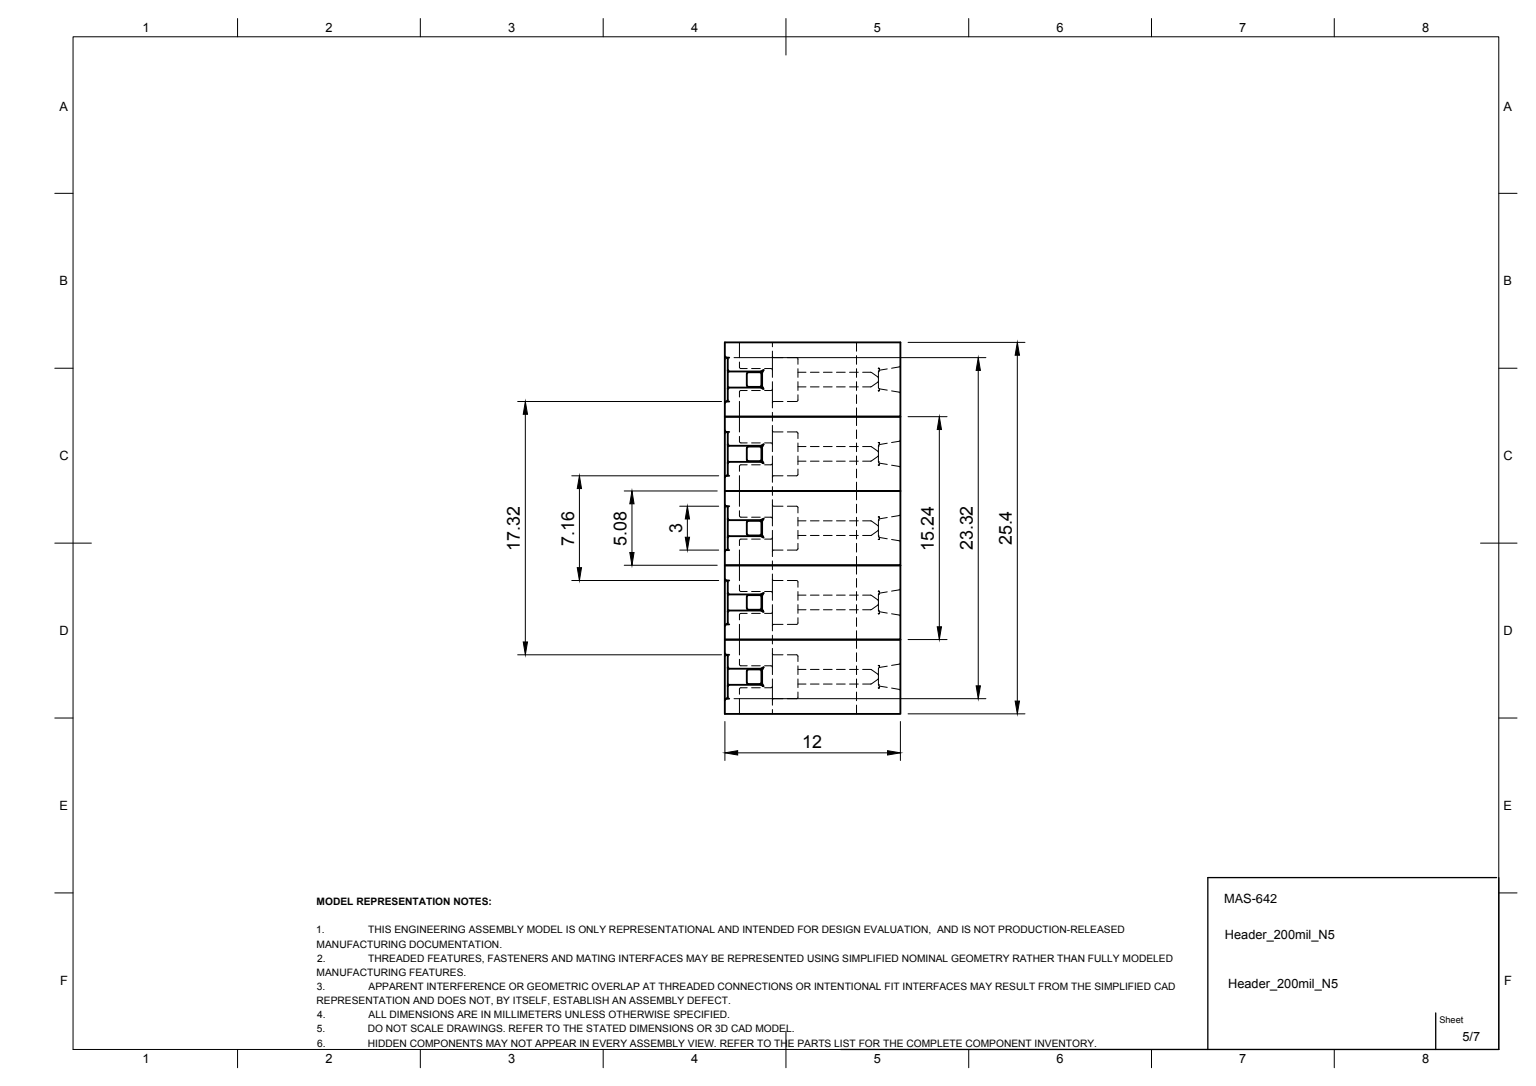
ISO-10303-21;
HEADER;
FILE_DESCRIPTION((''),'2;1');
FILE_NAME('Header_200mil_N5.step','2026-10-09T09:51:33-07:00',(''),(''),'','','');
FILE_SCHEMA (('AUTOMOTIVE_DESIGN { 1 0 10303 214 3 1 1 }'));
ENDSEC;
DATA;
#10=MECHANICAL_DESIGN_GEOMETRIC_PRESENTATION_REPRESENTATION('',(#482,#483,#484,#485,#486,#487,#488,#489,#490,#491,#492,#493,#494,#495,#496,#497,#498,#499,#500,#501,#502,#503,#504,#505,#506,#507,#508,#509,#510,#511,#512,#513,#514,#515,#516,#517,#518,#519,#520,#521,#522,#523,#524,#525,#526,#527,#528,#529,#530,#531,#532,#533,#534,#535,#536,#537,#538,#539,#540,#541,#542,#543,#544,#545,#546,#547,#548,#549,#550,#551,#552,#553,#554,#555,#556,#557,#558,#559,#560,#561,#562,#563,#564,#565,#566,#567,#568,#569,#570,#571,#572,#573,#574,#575,#576,#577,#578,#579,#580,#581,#582,#583,#584,#585,#586,#587,#588,#589,#590,#591,#592,#593,#594,#595,#596,#597,#598,#599,#600,#601,#602,#603,#604,#605,#606,#607,#608,#609,#610,#611,#612,#613,#614,#615,#616,#617,#618,#619,#620,#621,#622,#623,#624,#625,#626,#627,#628,#629,#630,#631,#632,#633,#634,#635,#636,#637,#638,#639,#640,#641,#642,#643,#644,#645,#646,#647,#648,#649,#650,#651,#652,#653,#654,#655,#656,#657,#658,#659,#660,#661,#662,#663,#664,#665,#666,#667,#668,#669,#670,#671,#672,#673,#674,#675,#676,#677,#678,#679,#680,#681,#682,#683,#684,#685,#686,#687,#688,#689,#690,#691,#692,#693,#694,#695,#696,#697,#698,#699,#700,#701,#702,#703,#704,#705,#706,#707,#708,#709,#710,#711,#712,#713,#714,#715,#716,#717,#718,#719,#720,#721,#722,#723,#724,#725,#726,#727,#728,#729,#730,#731,#732,#733,#734,#735,#736,#737,#738,#739,#740,#741,#742,#743,#744,#745,#746,#747,#748,#749,#750,#751,#752,#753,#754,#755,#756,#757,#758,#759,#760,#761,#762,#763,#764,#765,#766,#767,#768,#769,#770,#771,#772,#773,#774,#775,#776,#777,#778,#779,#780,#781,#782,#783,#784,#785,#786,#787,#788,#789,#790,#791,#792,#793,#794,#795,#796,#797,#798,#799,#800,#801,#802,#803,#804,#805,#806,#807,#808,#809,#810,#811,#812,#813,#814,#815,#816,#817,#818,#819,#820,#821,#822,#823,#824,#825,#826,#827,#828,#829,#830,#831,#832,#833,#834,#835,#836,#837,#838,#839,#840,#841,#842,#843,#844,#845,#846,#847,#848,#849,#850,#851,#852,#853,#854,#855,#856,#857,#858,#859,#860,#861,#862,#863,#864,#865,#866,#867,#868,#869,#870,#871,#872,#873,#874,#875,#876,#877,#878,#879,#880,#881,#882,#883,#884,#885,#886,#887,#888,#889,#890,#891,#892,#893,#894,#895,#896,#897,#898,#899,#900,#901,#902,#903,#904,#905,#906,#907,#908,#909,#910,#911,#912,#913,#914,#915,#916,#917,#918,#919,#920,#921,#922,#923,#924,#925,#926,#927,#928,#929,#930,#931,#932,#933,#934,#935,#936,#937,#938,#939,#940,#941,#942,#943,#944,#945,#946,#947,#948,#949,#950,#951,#952,#953,#954,#955,#956,#957,#958,#959,#960,#961,#962,#963,#964,#965,#966,#967,#968,#969,#970,#971,#972,#973,#974,#975,#976,#977,#978,#979,#980,#981,#982,#983,#984,#985,#986,#987,#988,#989,#990,#991,#992,#993,#994,#995,#996,#997,#998,#999,#1000,#1001,#1002,#1003,#1004,#1005,#1006,#1007,#1008,#1009,#1010,#1011,#1012,#1013,#1014,#1015,#1016,#1017,#1018,#1019,#1020,#1021,#1022,#1023,#1024,#1025,#1026,#1027,#1028,#1029,#1030,#1031,#1032,#1033,#1034,#1035,#1036,#1037,#1038,#1039,#1040,#1041,#1042,#1043,#1044,#1045,#1046,#1047,#1048,#1049,#1050,#1051,#1052,#1053,#1054,#1055,#1056,#1057,#1058,#1059,#1060,#1061,#1062,#1063,#1064,#1065,#1066,#1067,#1068,#1069,#1070,#1071,#1072,#1073,#1074,#1075,#1076,#1077,#1078,#1079,#1080,#1081,#1082,#1083,#1084,#1085,#1086,#1087,#1088,#1089,#1090,#1091,#1092,#1093,#1094,#1095,#1096,#1097,#1098,#1099,#1100,#1101,#1102,#1103,#1104,#1105,#1106,#1107,#1108,#1109,#1110,#1111,#1112,#1113,#1114,#1115,#1116,#1117,#1118,#1119,#1120,#1121,#1122,#1123,#1124,#1125,#1126,#1127,#1128,#1129,#1130,#1131,#1132,#1133,#1134,#1135,#1136,#1137,#1138,#1139,#1140,#1141,#1142,#1143,#1144,#1145,#1146,#1147,#1148,#1149,#1150,#1151,#1152,#1153,#1154,#1155,#1156,#1157,#1158,#1159,#1160,#1161,#1162,#1163,#1164,#1165,#1166,#1167,#1168,#1169,#1170,#1171,#1172,#1173,#1174,#1175,#1176,#1177,#1178,#1179,#1180,#1181,#1182,#1183,#1184,#1185,#1186,#1187,#1188,#1189,#1190,#1191,#1192,#1193,#1194,#1195,#1196,#1197,#1198,#1199,#1200,#1201,#1202,#1203,#1204,#1205,#1206,#1207,#1208,#1209,#1210,#1211,#1212,#1213,#1214,#1215,#1216,#1217,#1218,#1219,#1220,#1221,#1222,#1223,#1224,#1225,#1226,#1227,#1228,#1229,#1230,#1231,#1232,#1233,#1234,#1235,#1236,#1237,#1238,#1239,#1240,#1241,#1242,#1243,#1244,#1245,#1246,#1247,#1248,#1249,#1250,#1251,#1252,#1253,#1254,#1255,#1256,#1257,#1258,#1259,#1260,#1261,#1262,#1263,#1264,#1265,#1266,#1267,#1268,#1269,#1270,#1271,#1272,#1273,#1274,#1275,#1276,#1277,#1278,#1279,#1280,#1281,#1282,#1283,#1284,#1285,#1286,#1287,#1288,#1289,#1290,#1291,#1292,#1293,#1294,#1295,#1296,#1297,#1298,#1299,#1300,#1301,#1302,#1303,#1304,#1305,#1306,#1307,#1308,#1309,#1310,#1311,#1312,#1313,#1314,#1315,#1316,#1317,#1318,#1319,#1320,#1321,#1322,#1323,#1324,#1325,#1326,#1327,#1328,#1329,#1330,#1331,#1332,#1333,#1334,#1335,#1336,#1337,#1338,#1339,#1340,#1341,#1342,#1343,#1344,#1345,#1346,#1347,#1348,#1349,#1350,#1351,#1352,#1353,#1354,#1355,#1356,#1357,#1358,#1359,#1360,#1361,#1362,#1363,#1364,#1365,#1366,#1367,#1368,#1369,#1370,#1371,#1372,#1373,#1374,#1375,#1376,#1377,#1378,#1379,#1380,#1381,#1382,#1383,#1384,#1385,#1386,#1387,#1388,#1389,#1390,#1391,#1392,#1393,#1394,#1395,#1396,#1397,#1398,#1399,#1400,#1401,#1402,#1403,#1404,#1405,#1406,#1407,#1408,#1409,#1410,#1411,#1412,#1413,#1414,#1415,#1416,#1417,#1418,#1419,#1420,#1421,#1422,#1423,#1424,#1425,#1426,#1427,#1428,#1429,#1430,#1431,#1432,#1433,#1434,#1435,#1436,#1437,#1438,#1439,#1440,#1441,#1442,#1443,#1444,#1445,#1446,#1447,#1448,#1449,#1450,#1451,#1452,#1453,#1454,#1455,#1456,#1457,#1458,#1459,#1460,#1461,#1462,#1463,#1464,#1465,#1466,#1467,#1468,#1469,#1470,#1471,#1472,#1473,#1474,#1475,#1476,#1477,#1478,#1479,#1480,#1481,#1482,#1483,#1484,#1485,#1486,#1487,#1488,#1489,#1490,#1491,#1492,#1493,#1494,#1495,#1496,#1497,#1498,#1499,#1500,#1501,#1502,#1503,#1504,#1505,#1506,#1507,#1508,#1509,#1510,#1511,#1512,#1513,#1514,#1515,#1516,#1517,#1518,#1519,#1520,#1521,#1522,#1523,#1524,#1525,#1526,#1527,#1528,#1529,#1530,#1531,#1532,#1533,#1534,#1535,#1536,#1537,#1538,#1539,#1540,#1541,#1542,#1543,#1544,#1545,#1546,#1547,#1548,#1549,#1550,#1551,#1552,#1553,#1554,#1555,#1556,#1557,#1558,#1559,#1560,#1561,#1562,#1563,#1564,#1565,#1566,#1567,#1568,#1569,#1570,#1571,#1572,#1573,#1574,#1575,#1576,#1577,#1578,#1579,#1580,#1581,#1582,#1583,#1584,#1585,#1586,#1587,#1588,#1589,#1590,#1591,#1592,#1593,#1594,#1595,#1596,#1597,#1598,#1599,#1600,#1601,#1602,#1603,#1604,#1605,#1606,#1607,#1608,#1609,#1610,#1611,#1612,#1613,#1614,#1615,#1616,#1617,#1618,#1619,#1620,#1621,#1622,#1623,#1624,#1625,#1626,#1627,#1628,#1629,#1630,#1631,#1632,#1633,#1634,#1635,#1636,#1637,#1638,#1639,#1640,#1641,#1642,#1643,#1644,#1645,#1646,#1647,#1648,#1649,#1650,#1651,#1652,#1653,#1654,#1655,#1656,#1657,#1658,#1659,#1660,#1661,#1662,#1663,#1664,#1665,#1666,#1667,#1668,#1669,#1670,#1671,#1672,#1673,#1674,#1675,#1676,#1677,#1678,#1679,#1680,#1681,#1682,#1683,#1684,#1685,#1686,#1687,#1688,#1689,#1690,#1691,#1692,#1693,#1694,#1695,#1696,#1697,#1698,#1699,#1700,#1701,#1702,#1703,#1704,#1705,#1706,#1707,#1708,#1709,#1710,#1711,#1712,#1713,#1714,#1715,#1716,#1717,#1718,#1719,#1720,#1721,#1722,#1723,#1724,#1725,#1726,#1727,#1728,#1729,#1730,#1731,#1732,#1733,#1734,#1735,#1736,#1737,#1738,#1739,#1740,#1741,#1742,#1743,#1744,#1745,#1746,#1747,#1748,#1749,#1750,#1751,#1752,#1753,#1754,#1755,#1756,#1757,#1758,#1759,#1760,#1761,#1762,#1763,#1764,#1765,#1766,#1767,#1768,#1769,#1770,#1771,#1772,#1773,#1774,#1775,#1776,#1777,#1778,#1779,#1780,#1781,#1782,#1783,#1784,#1785,#1786,#1787,#1788,#1789,#1790,#1791,#1792,#1793,#1794,#1795,#1796,#1797,#1798,#1799,#1800,#1801,#1802,#1803,#1804,#1805,#1806,#1807,#1808,#1809,#1810,#1811,#1812,#1813,#1814,#1815,#1816,#1817,#1818,#1819,#1820,#1821,#1822,#1823,#1824,#1825,#1826,#1827,#1828,#1829,#1830,#1831,#1832,#1833,#1834,#1835,#1836,#1837,#1838,#1839,#1840,#1841,#1842,#1843,#1844,#1845,#1846,#1847,#1848,#1849,#1850,#1851,#1852,#1853,#1854,#1855,#1856,#1857,#1858,#1859,#1860,#1861,#1862,#1863,#1864,#1865,#1866,#1867,#1868,#1869,#1870,#1871,#1872,#1873,#1874,#1875,#1876,#1877,#1878,#1879,#1880,#1881,#1882,#1883,#1884,#1885,#1886,#1887,#1888,#1889,#1890,#1891,#1892,#1893,#1894,#1895,#1896,#1897,#1898,#1899,#1900,#1901,#1902,#1903,#1904,#1905,#1906,#1907,#1908,#1909,#1910,#1911,#1912,#1913,#1914,#1915,#1916,#1917,#1918,#1919,#1920,#1921,#1922,#1923,#1924,#1925,#1926,#1927,#1928,#1929,#1930,#1931),#126571);
#75=B_SPLINE_CURVE_WITH_KNOTS('',3,(#101199,#101200,#101201,#101202,#101203,
#101204,#101205,#101206,#101207,#101208),.UNSPECIFIED.,.F.,.F.,(4,3,3,4),
(3.9738238267564E-15,3.94729529730257E-5,7.90727202189652E-5,0.000103003463696664),
 .UNSPECIFIED.) ;
#76=B_SPLINE_CURVE_WITH_KNOTS('',3,(#101215,#101216,#101217,#101218,#101219,
#101220,#101221),.UNSPECIFIED.,.F.,.F.,(4,3,4),(0.000158223357507089,0.000179871364136711,
0.000191820073778124),.UNSPECIFIED.) ;
#77=B_SPLINE_CURVE_WITH_KNOTS('',3,(#101236,#101237,#101238,#101239,#101240,
#101241,#101242,#101243,#101244,#101245,#101246,#101247,#101248,#101249,
#101250,#101251),.UNSPECIFIED.,.F.,.F.,(4,3,3,3,3,4),(2.2541451328491E-8,
3.71181381094363E-5,7.40234349159883E-5,0.000126639028433409,0.000171180683285943,
0.000173579731706481),.UNSPECIFIED.) ;
#78=B_SPLINE_CURVE_WITH_KNOTS('',3,(#101307,#101308,#101309,#101310,#101311,
#101312),.UNSPECIFIED.,.F.,.F.,(4,2,4),(0.,0.000162685424844482,0.000325370849688964),
 .UNSPECIFIED.) ;
#79=B_SPLINE_CURVE_WITH_KNOTS('',3,(#101315,#101316,#101317,#101318,#101319,
#101320),.UNSPECIFIED.,.F.,.F.,(4,2,4),(0.,0.000163438694679258,0.000326877389358517),
 .UNSPECIFIED.) ;
#80=B_SPLINE_CURVE_WITH_KNOTS('',3,(#101331,#101332,#101333,#101334,#101335,
#101336),.UNSPECIFIED.,.F.,.F.,(4,2,4),(-0.00501427184001373,-0.00354643693242479,
0.),.UNSPECIFIED.) ;
#81=B_SPLINE_CURVE_WITH_KNOTS('',3,(#101349,#101350,#101351,#101352,#101353,
#101354,#101355,#101356,#101357,#101358,#101359,#101360,#101361,#101362,
#101363,#101364,#101365,#101366,#101367,#101368,#101369,#101370,#101371,
#101372,#101373,#101374,#101375,#101376),.UNSPECIFIED.,.F.,.F.,(4,3,3,3,
3,3,3,3,3,4),(5.23810621123106E-9,5.84794260518929E-6,8.4966204178186E-6,
1.21937803558207E-5,1.76033670138093E-5,1.93092034273016E-5,2.55871453405733E-5,
3.03154216363468E-5,3.6851966035102E-5,3.92146766969322E-5),
 .UNSPECIFIED.) ;
#82=B_SPLINE_CURVE_WITH_KNOTS('',3,(#101378,#101379,#101380,#101381,#101382,
#101383,#101384,#101385,#101386,#101387),.UNSPECIFIED.,.F.,.F.,(4,3,3,4),
(0.000144469795965456,0.000165397602015579,0.000173816468562374,0.000175865847906018),
 .UNSPECIFIED.) ;
#83=B_SPLINE_CURVE_WITH_KNOTS('',3,(#101405,#101406,#101407,#101408,#101409,
#101410,#101411),.UNSPECIFIED.,.F.,.F.,(4,3,4),(-2.05331166616804E-6,2.04386714305399E-5,
3.16299855932264E-5),.UNSPECIFIED.) ;
#84=B_SPLINE_CURVE_WITH_KNOTS('',3,(#101413,#101414,#101415,#101416,#101417,
#101418,#101419,#101420,#101421,#101422,#101423,#101424),.UNSPECIFIED.,
 .F.,.F.,(4,2,2,2,2,4),(9.00279448284787E-9,0.00183032786992351,0.0060774656661988,
0.0169681634641076,0.0216775195638031,0.0254454420779839),.UNSPECIFIED.) ;
#85=B_SPLINE_CURVE_WITH_KNOTS('',3,(#101583,#101584,#101585,#101586,#101587,
#101588,#101589,#101590,#101591,#101592,#101593,#101594,#101595,#101596,
#101597,#101598,#101599,#101600,#101601,#101602,#101603,#101604,#101605,
#101606,#101607,#101608,#101609,#101610,#101611,#101612,#101613,#101614,
#101615,#101616,#101617,#101618,#101619,#101620,#101621,#101622),
 .UNSPECIFIED.,.F.,.F.,(4,3,3,3,3,3,3,3,3,3,3,3,3,4),(3.25260651745651E-19,
5.07173230207635E-5,0.000104017413485144,0.000124506719166644,0.000125249568192437,
0.000156566023859648,0.000186760078749966,0.000187880030991792,0.000203537318084802,
0.000211366035547456,0.000217886758541627,0.000219194644848635,0.000234851354133261,
0.000249013438333288),.UNSPECIFIED.) ;
#86=B_SPLINE_CURVE_WITH_KNOTS('',3,(#101628,#101629,#101630,#101631,#101632,
#101633,#101634,#101635,#101636,#101637,#101638,#101639,#101640,#101641,
#101642,#101643,#101644,#101645,#101646,#101647,#101648,#101649,#101650,
#101651,#101652,#101653,#101654,#101655,#101656,#101657,#101658,#101659,
#101660,#101661,#101662,#101663,#101664,#101665,#101666,#101667),
 .UNSPECIFIED.,.F.,.F.,(4,3,3,3,3,3,3,3,3,3,3,3,3,4),(0.,1.43115567092604E-5,
3.01335133960367E-5,3.14552036774737E-5,3.8044751729729E-5,4.5956122251847E-5,
6.17788922892814E-5,6.29104073549473E-5,9.3421096696511E-5,0.000125066393795497,
0.000125820814709898,0.000179837268175291,0.000231469985683482,0.0002516416294198),
 .UNSPECIFIED.) ;
#87=B_SPLINE_CURVE_WITH_KNOTS('',3,(#101672,#101673,#101674,#101675,#101676,
#101677,#101678),.UNSPECIFIED.,.F.,.F.,(4,3,4),(-2.04939766627081E-6,0.,
2.93835791072158E-5),.UNSPECIFIED.) ;
#88=B_SPLINE_CURVE_WITH_KNOTS('',3,(#101693,#101694,#101695,#101696,#101697,
#101698,#101699,#101700,#101701,#101702,#101703,#101704,#101705,#101706),
 .UNSPECIFIED.,.F.,.F.,(4,2,2,2,2,2,4),(1.44901762830932E-6,0.00056162152378578,
0.00112173034328052,0.00210338619166554,0.00384452539466144,0.00473112295119629,
0.00541108585516142),.UNSPECIFIED.) ;
#89=B_SPLINE_CURVE_WITH_KNOTS('',3,(#101715,#101716,#101717,#101718,#101719,
#101720,#101721,#101722,#101723,#101724,#101725,#101726,#101727,#101728,
#101729,#101730,#101731,#101732,#101733,#101734,#101735,#101736,#101737,
#101738,#101739,#101740,#101741,#101742,#101743,#101744,#101745,#101746,
#101747,#101748),.UNSPECIFIED.,.F.,.F.,(4,2,2,2,2,2,2,2,2,2,2,2,2,2,2,2,
4),(0.,1.67528894171223E-5,3.36326639087882E-5,3.53285003632596E-5,3.67766442981684E-5,
4.45936877500603E-5,5.25629171992643E-5,5.37833548713901E-5,5.51649664472508E-5,
7.22376444474067E-5,7.35532885963332E-5,0.000109240736296583,0.000146228640920627,
0.000147106577192663,0.000203359192947108,0.000258123601946057,0.000294213154385318),
 .UNSPECIFIED.) ;
#90=B_SPLINE_CURVE_WITH_KNOTS('',3,(#101752,#101753,#101754,#101755,#101756,
#101757,#101758,#101759,#101760,#101761,#101762,#101763,#101764,#101765,
#101766,#101767,#101768,#101769,#101770,#101771,#101772,#101773,#101774,
#101775,#101776,#101777,#101778,#101779,#101780,#101781,#101782,#101783,
#101784,#101785,#101786,#101787,#101788,#101789,#101790,#101791,#101792,
#101793,#101794,#101795,#101796,#101797,#101798,#101799,#101800,#101801,
#101802,#101803),.UNSPECIFIED.,.F.,.F.,(4,3,3,3,3,3,3,3,3,3,3,3,3,3,3,3,
3,4),(0.,5.28180786082966E-5,0.000107888430275573,0.000143209193858987,
0.000144078242180707,0.000180086811859616,0.000214813790788481,0.00021545817026355,
0.000216102549738619,0.000232714940020855,0.000234106492510809,0.000238605983992194,
0.000240855729732887,0.00024310547547358,0.00025061608925323,0.000252108710851783,
0.000270124214172477,0.000286418387717979),.UNSPECIFIED.) ;
#91=B_SPLINE_CURVE_WITH_KNOTS('',3,(#101948,#101949,#101950,#101951,#101952,
#101953,#101954,#101955),.UNSPECIFIED.,.F.,.F.,(4,2,2,4),(-0.0473604779370388,
-0.0461995546884435,-0.0447198409510953,-0.0410407833884838),
 .UNSPECIFIED.) ;
#92=B_SPLINE_CURVE_WITH_KNOTS('',3,(#101963,#101964,#101965,#101966,#101967,
#101968,#101969,#101970),.UNSPECIFIED.,.F.,.F.,(4,2,2,4),(-0.0536801724855785,
-0.0500011149229822,-0.048521401185634,-0.0473604779370388),
 .UNSPECIFIED.) ;
#93=B_SPLINE_CURVE_WITH_KNOTS('',3,(#102424,#102425,#102426,#102427,#102428,
#102429,#102430,#102431,#102432,#102433,#102434,#102435,#102436,#102437),
 .UNSPECIFIED.,.F.,.F.,(4,2,2,2,2,2,4),(4.71238898038469,4.8817580624518,
5.06763701998932,5.24337922965563,5.26451333208247,5.44874090582915,5.49822830854824),
 .UNSPECIFIED.) ;
#94=B_SPLINE_CURVE_WITH_KNOTS('',3,(#102442,#102443,#102444,#102445,#102446,
#102447,#102448,#102449,#102450,#102451,#102452,#102453,#102454,#102455),
 .UNSPECIFIED.,.F.,.F.,(4,2,2,2,2,2,4),(0.784956998631334,0.96694169431193,
1.1431172121296,1.16348181627596,1.34745079132871,1.51752882030683,1.5707963267949),
 .UNSPECIFIED.) ;
#95=B_SPLINE_CURVE_WITH_KNOTS('',3,(#102461,#102462,#102463,#102464,#102465,
#102466,#102467,#102468,#102469,#102470,#102471,#102472,#102473,#102474),
 .UNSPECIFIED.,.F.,.F.,(4,2,2,2,2,2,4),(0.784956998631337,0.966941694311871,
1.14311721213079,1.16348181627588,1.34745079132852,1.51752882030658,1.5707963267949),
 .UNSPECIFIED.) ;
#96=B_SPLINE_CURVE_WITH_KNOTS('',3,(#102476,#102477,#102478,#102479,#102480,
#102481,#102482,#102483,#102484,#102485,#102486,#102487,#102488,#102489),
 .UNSPECIFIED.,.F.,.F.,(4,2,2,2,2,2,4),(4.71238898038469,4.88175806245191,
5.06763701998937,5.24337922965534,5.2645133320825,5.44874090582923,5.49822830854825),
 .UNSPECIFIED.) ;
#97=B_SPLINE_CURVE_WITH_KNOTS('',3,(#102493,#102494,#102495,#102496,#102497,
#102498,#102499,#102500,#102501,#102502,#102503,#102504,#102505,#102506),
 .UNSPECIFIED.,.F.,.F.,(4,2,2,2,2,2,4),(4.71238898038469,4.88175806245175,
5.06763701998915,5.24337922965918,5.26451333208223,5.44874090582892,5.49822830854824),
 .UNSPECIFIED.) ;
#98=B_SPLINE_CURVE_WITH_KNOTS('',3,(#102510,#102511,#102512,#102513,#102514,
#102515,#102516,#102517,#102518,#102519,#102520,#102521,#102522,#102523),
 .UNSPECIFIED.,.F.,.F.,(4,2,2,2,2,2,4),(0.784956998631348,0.96694169431196,
1.14311721213076,1.16348181627594,1.34745079132846,1.51752882030657,1.5707963267949),
 .UNSPECIFIED.) ;
#99=B_SPLINE_CURVE_WITH_KNOTS('',3,(#102538,#102539,#102540,#102541,#102542,
#102543,#102544,#102545,#102546,#102547,#102548,#102549,#102550,#102551),
 .UNSPECIFIED.,.F.,.F.,(4,2,2,2,2,2,4),(0.784956998631344,0.966941694311673,
1.14311721213023,1.16348181627565,1.34745079132822,1.51752882030641,1.5707963267949),
 .UNSPECIFIED.) ;
#100=B_SPLINE_CURVE_WITH_KNOTS('',3,(#102555,#102556,#102557,#102558,#102559,
#102560,#102561,#102562,#102563,#102564,#102565,#102566,#102567,#102568),
 .UNSPECIFIED.,.F.,.F.,(4,2,2,2,2,2,4),(4.71238898038469,4.88175806245189,
5.06763701998948,5.24337922965067,5.26451333208267,5.44874090582925,5.49822830854823),
 .UNSPECIFIED.) ;
#101=B_SPLINE_CURVE_WITH_KNOTS('',3,(#102673,#102674,#102675,#102676,#102677,
#102678,#102679,#102680,#102681,#102682,#102683,#102684,#102685,#102686,
#102687,#102688),.UNSPECIFIED.,.F.,.F.,(4,3,3,3,3,4),(0.,3.26760986414936E-5,
6.60604127813368E-5,0.00010113572426573,0.000138237800333083,0.000166242991827322),
 .UNSPECIFIED.) ;
#102=B_SPLINE_CURVE_WITH_KNOTS('',3,(#102750,#102751,#102752,#102753,#102754,
#102755,#102756,#102757,#102758,#102759,#102760,#102761,#102762,#102763,
#102764,#102765),.UNSPECIFIED.,.F.,.F.,(4,3,3,3,3,4),(0.,1.86901632150157E-5,
5.38940239621533E-5,9.13255451816924E-5,0.000129775966053829,0.000168373497604197),
 .UNSPECIFIED.) ;
#103=B_SPLINE_CURVE_WITH_KNOTS('',3,(#102770,#102771,#102772,#102773,#102774,
#102775,#102776,#102777,#102778,#102779),.UNSPECIFIED.,.F.,.F.,(4,2,2,2,
4),(0.0288531015810606,0.0296205843579712,0.0328031056820271,0.0376042554622301,
0.0407130021445681),.UNSPECIFIED.) ;
#104=B_SPLINE_CURVE_WITH_KNOTS('',3,(#102784,#102785,#102786,#102787,#102788,
#102789),.UNSPECIFIED.,.F.,.F.,(4,2,4),(0.0637474840427468,0.0675088661505087,
0.0720284409664136),.UNSPECIFIED.) ;
#105=B_SPLINE_CURVE_WITH_KNOTS('',3,(#102795,#102796,#102797,#102798,#102799,
#102800,#102801,#102802,#102803,#102804),.UNSPECIFIED.,.F.,.F.,(4,2,2,2,
4),(0.0767275662247105,0.0771734766312244,0.0818220866843324,0.0868722195343171,
0.0892832637334449),.UNSPECIFIED.) ;
#106=B_SPLINE_CURVE_WITH_KNOTS('',3,(#102839,#102840,#102841,#102842,#102843,
#102844),.UNSPECIFIED.,.F.,.F.,(4,2,4),(0.171679973604307,0.178707475947415,
0.186889989698882),.UNSPECIFIED.) ;
#107=B_SPLINE_CURVE_WITH_KNOTS('',3,(#102884,#102885,#102886,#102887,#102888,
#102889,#102890,#102891,#102892,#102893,#102894,#102895,#102896,#102897,
#102898,#102899,#102900,#102901,#102902,#102903,#102904,#102905,#102906,
#102907,#102908,#102909,#102910,#102911,#102912,#102913),.UNSPECIFIED.,
 .F.,.F.,(4,2,2,2,2,2,2,2,2,2,2,2,2,2,4),(2.36970964942748,2.55498029688293,
2.73514427897862,2.74569929646372,2.92071305421519,2.93943382978511,3.11857096683926,
3.13197658032397,3.25399179664489,3.45054278261474,3.62794535800311,3.64606212534864,
3.82474099483969,3.83698255062518,3.9134742131524),.UNSPECIFIED.) ;
#108=B_SPLINE_CURVE_WITH_KNOTS('',3,(#102924,#102925,#102926,#102927,#102928,
#102929,#102930,#102931,#102932,#102933,#102934,#102935,#102936,#102937,
#102938,#102939,#102940,#102941,#102942,#102943,#102944,#102945,#102946,
#102947,#102948,#102949),.UNSPECIFIED.,.F.,.F.,(4,2,2,2,2,2,2,2,2,2,2,2,
4),(2.70344464881052,2.89144352771273,3.06851986332525,3.0808108907457,
3.26996664970825,3.35940092938491,3.54587543017999,3.72254345721242,3.73903833379419,
3.91570024693591,3.93052100184837,4.1173551198632,4.22222897897866),
 .UNSPECIFIED.) ;
#109=B_SPLINE_CURVE_WITH_KNOTS('',3,(#103107,#103108,#103109,#103110,#103111,
#103112,#103113,#103114,#103115,#103116,#103117,#103118,#103119,#103120,
#103121,#103122,#103123,#103124,#103125),.UNSPECIFIED.,.F.,.F.,(4,3,3,3,
3,3,4),(2.81004151652491E-8,3.99307614181575E-5,8.00540716903473E-5,0.000126830846822484,
0.000175618195186419,0.00021519314047228,0.000245220898756747),
 .UNSPECIFIED.) ;
#110=B_SPLINE_CURVE_WITH_KNOTS('',3,(#103148,#103149,#103150,#103151,#103152,
#103153,#103154,#103155,#103156,#103157,#103158,#103159,#103160,#103161,
#103162,#103163,#103164,#103165,#103166,#103167,#103168,#103169,#103170,
#103171,#103172,#103173,#103174,#103175,#103176,#103177,#103178,#103179,
#103180,#103181,#103182,#103183,#103184,#103185,#103186,#103187,#103188,
#103189,#103190,#103191,#103192,#103193,#103194,#103195,#103196,#103197,
#103198,#103199,#103200,#103201,#103202,#103203,#103204,#103205,#103206,
#103207,#103208,#103209,#103210,#103211,#103212,#103213,#103214,#103215,
#103216,#103217,#103218,#103219,#103220,#103221,#103222,#103223,#103224,
#103225,#103226),.UNSPECIFIED.,.F.,.F.,(4,3,3,3,3,3,3,3,3,3,3,3,3,3,3,3,
3,3,3,3,3,3,3,3,3,3,4),(0.000152038190190966,0.00015489284140843,0.000155160464960067,
0.000160456565729287,0.000163456795060822,0.000166580092246913,0.000167751328691697,
0.000168007536663994,0.000168255738137156,0.000169267315291243,0.000175949983805187,
0.000178959298271468,0.000180334649023636,0.000187987241670312,0.000191981216408558,
0.000193065528939082,0.000193839174265184,0.000198143816207852,0.000212206269476803,
0.000226582370019584,0.000228143757087806,0.000228729277238389,0.000232827918292472,
0.000249109432819239,0.000250176797440921,0.000265881325829883,0.00026752567658937),
 .UNSPECIFIED.) ;
#111=B_SPLINE_CURVE_WITH_KNOTS('',3,(#103228,#103229,#103230,#103231,#103232,
#103233,#103234,#103235,#103236,#103237),.UNSPECIFIED.,.F.,.F.,(4,3,3,4),
(0.000130631741230592,0.000139067346352972,0.000143554831048516,0.000152038189371529),
 .UNSPECIFIED.) ;
#112=B_SPLINE_CURVE_WITH_KNOTS('',3,(#103239,#103240,#103241,#103242,#103243,
#103244,#103245,#103246,#103247,#103248,#103249,#103250,#103251,#103252,
#103253,#103254,#103255,#103256,#103257),.UNSPECIFIED.,.F.,.F.,(4,3,3,3,
3,3,4),(0.000104137230127885,0.000110259474166351,0.000116844366893157,
0.000120664217590229,0.000125429508057305,0.000130430624030388,0.000130630877722849),
 .UNSPECIFIED.) ;
#113=B_SPLINE_CURVE_WITH_KNOTS('',3,(#103258,#103259,#103260,#103261,#103262,
#103263,#103264,#103265,#103266,#103267,#103268,#103269,#103270,#103271,
#103272,#103273,#103274,#103275,#103276,#103277,#103278,#103279,#103280,
#103281,#103282,#103283,#103284,#103285,#103286,#103287,#103288,#103289,
#103290,#103291,#103292,#103293,#103294,#103295,#103296,#103297,#103298,
#103299,#103300),.UNSPECIFIED.,.F.,.F.,(4,3,3,3,3,3,3,3,3,3,3,3,3,3,4),
(0.,4.7842153196409E-6,1.59977421330766E-5,1.7596526576931E-5,2.63603667654262E-5,
3.75047088104424E-5,4.29655082836412E-5,5.34507806651091E-5,6.17416442239024E-5,
6.3936053046577E-5,7.32944438956243E-5,8.49065978095127E-5,9.46209320477897E-5,
9.66050857869699E-5,0.000104137229466899),.UNSPECIFIED.) ;
#114=B_SPLINE_CURVE_WITH_KNOTS('',3,(#103370,#103371,#103372,#103373,#103374,
#103375,#103376,#103377,#103378,#103379,#103380,#103381,#103382,#103383,
#103384,#103385,#103386,#103387,#103388,#103389,#103390,#103391,#103392,
#103393,#103394,#103395,#103396,#103397,#103398,#103399,#103400,#103401,
#103402,#103403),.UNSPECIFIED.,.F.,.F.,(4,3,3,3,3,3,3,3,3,3,3,4),(0.000173579735006479,
0.000179152672590571,0.000187122196212527,0.000190349677855674,0.000201571576239331,
0.000207505544696437,0.000209082158340111,0.000218112358783822,0.000219837174422831,
0.000228512621317844,0.000240802935331578,0.000245138123631296),
 .UNSPECIFIED.) ;
#115=B_SPLINE_CURVE_WITH_KNOTS('',3,(#103465,#103466,#103467,#103468,#103469,
#103470,#103471,#103472,#103473,#103474,#103475,#103476,#103477,#103478,
#103479,#103480),.UNSPECIFIED.,.F.,.F.,(4,3,3,3,3,4),(0.00014982626823882,
0.000156541783273878,0.000187447062839771,0.000218157419331145,0.000251253590119498,
0.000263630362845943),.UNSPECIFIED.) ;
#116=B_SPLINE_CURVE_WITH_KNOTS('',3,(#103482,#103483,#103484,#103485),
 .UNSPECIFIED.,.F.,.F.,(4,4),(0.000128945525003041,0.00014982626823882),
 .UNSPECIFIED.) ;
#117=B_SPLINE_CURVE_WITH_KNOTS('',3,(#103486,#103487,#103488,#103489,#103490,
#103491,#103492,#103493,#103494,#103495,#103496,#103497,#103498,#103499,
#103500,#103501),.UNSPECIFIED.,.F.,.F.,(4,3,3,3,3,4),(0.000107977862661221,
0.000113849696954279,0.000116758640899991,0.000123355930725603,0.00012864932133829,
0.000128945525003041),.UNSPECIFIED.) ;
#118=B_SPLINE_CURVE_WITH_KNOTS('',3,(#103711,#103712,#103713,#103714,#103715,
#103716,#103717,#103718,#103719,#103720),.UNSPECIFIED.,.F.,.F.,(4,3,3,4),
(3.97263228028543E-15,3.94729529730253E-5,7.90727202189645E-5,0.000103003463696544),
 .UNSPECIFIED.) ;
#119=B_SPLINE_CURVE_WITH_KNOTS('',3,(#103727,#103728,#103729,#103730,#103731,
#103732,#103733),.UNSPECIFIED.,.F.,.F.,(4,3,4),(0.000158223357507079,0.000179871364137041,
0.000191820073778125),.UNSPECIFIED.) ;
#120=B_SPLINE_CURVE_WITH_KNOTS('',3,(#103748,#103749,#103750,#103751,#103752,
#103753,#103754,#103755,#103756,#103757,#103758,#103759,#103760,#103761,
#103762,#103763),.UNSPECIFIED.,.F.,.F.,(4,3,3,3,3,4),(2.25414513312457E-8,
3.71181381094367E-5,7.40234349159884E-5,0.00012663902843341,0.000171180683285944,
0.000173579731706483),.UNSPECIFIED.) ;
#121=B_SPLINE_CURVE_WITH_KNOTS('',3,(#103819,#103820,#103821,#103822,#103823,
#103824),.UNSPECIFIED.,.F.,.F.,(4,2,4),(0.,0.000162685424844482,0.000325370849688964),
 .UNSPECIFIED.) ;
#122=B_SPLINE_CURVE_WITH_KNOTS('',3,(#103827,#103828,#103829,#103830,#103831,
#103832),.UNSPECIFIED.,.F.,.F.,(4,2,4),(0.,0.000163438694679258,0.000326877389358517),
 .UNSPECIFIED.) ;
#123=B_SPLINE_CURVE_WITH_KNOTS('',3,(#103843,#103844,#103845,#103846,#103847,
#103848),.UNSPECIFIED.,.F.,.F.,(4,2,4),(-0.00501427184001364,-0.00354643693242477,
0.),.UNSPECIFIED.) ;
#124=B_SPLINE_CURVE_WITH_KNOTS('',3,(#103861,#103862,#103863,#103864,#103865,
#103866,#103867,#103868,#103869,#103870,#103871,#103872,#103873,#103874,
#103875,#103876,#103877,#103878,#103879,#103880,#103881,#103882,#103883,
#103884,#103885,#103886,#103887,#103888),.UNSPECIFIED.,.F.,.F.,(4,3,3,3,
3,3,3,3,3,4),(5.23810620682237E-9,5.84794260519337E-6,8.49662041781855E-6,
1.2193780355802E-5,1.76033670137239E-5,1.93092034273018E-5,2.55871453405539E-5,
3.03154216363478E-5,3.68519660351436E-5,3.92146766969337E-5),
 .UNSPECIFIED.) ;
#125=B_SPLINE_CURVE_WITH_KNOTS('',3,(#103890,#103891,#103892,#103893,#103894,
#103895,#103896,#103897,#103898,#103899),.UNSPECIFIED.,.F.,.F.,(4,3,3,4),
(0.000144469795965455,0.000165397602015561,0.000173816468562373,0.000175865847906015),
 .UNSPECIFIED.) ;
#126=B_SPLINE_CURVE_WITH_KNOTS('',3,(#103917,#103918,#103919,#103920,#103921,
#103922,#103923),.UNSPECIFIED.,.F.,.F.,(4,3,4),(-2.05331166616703E-6,2.04386714305792E-5,
3.1629985593224E-5),.UNSPECIFIED.) ;
#127=B_SPLINE_CURVE_WITH_KNOTS('',3,(#103925,#103926,#103927,#103928,#103929,
#103930,#103931,#103932,#103933,#103934,#103935,#103936),.UNSPECIFIED.,
 .F.,.F.,(4,2,2,2,2,4),(9.00279511935952E-9,0.00183032787015945,0.00607746566495241,
0.016968163415124,0.0216775194921712,0.025445441987748),.UNSPECIFIED.) ;
#128=B_SPLINE_CURVE_WITH_KNOTS('',3,(#104095,#104096,#104097,#104098,#104099,
#104100,#104101,#104102,#104103,#104104,#104105,#104106,#104107,#104108,
#104109,#104110,#104111,#104112,#104113,#104114,#104115,#104116,#104117,
#104118,#104119,#104120,#104121,#104122,#104123,#104124,#104125,#104126,
#104127,#104128,#104129,#104130,#104131,#104132,#104133,#104134),
 .UNSPECIFIED.,.F.,.F.,(4,3,3,3,3,3,3,3,3,3,3,3,3,4),(0.,5.0717323021306E-5,
0.000104017413486267,0.000124506719166654,0.000125249568192443,0.000156566023859662,
0.000186760078749982,0.000187880030991811,0.000203537318084821,0.000211366035547473,
0.000217886758541643,0.000219194644848652,0.000234851354133276,0.000249013438333305),
 .UNSPECIFIED.) ;
#129=B_SPLINE_CURVE_WITH_KNOTS('',3,(#104140,#104141,#104142,#104143,#104144,
#104145,#104146,#104147,#104148,#104149,#104150,#104151,#104152,#104153,
#104154,#104155,#104156,#104157,#104158,#104159,#104160,#104161,#104162,
#104163,#104164,#104165,#104166,#104167,#104168,#104169,#104170,#104171,
#104172,#104173,#104174,#104175,#104176,#104177,#104178,#104179),
 .UNSPECIFIED.,.F.,.F.,(4,3,3,3,3,3,3,3,3,3,3,3,3,4),(0.,1.43115567092614E-5,
3.01335133960405E-5,3.14552036774747E-5,3.80447517297348E-5,4.59561222518546E-5,
6.17788922892857E-5,6.29104073549493E-5,9.34210966965139E-5,0.000125066393795497,
0.000125820814709899,0.00017983726817215,0.000231469985677585,0.0002516416294198),
 .UNSPECIFIED.) ;
#130=B_SPLINE_CURVE_WITH_KNOTS('',3,(#104184,#104185,#104186,#104187,#104188,
#104189,#104190),.UNSPECIFIED.,.F.,.F.,(4,3,4),(-2.04939766627066E-6,0.,
2.9383579107217E-5),.UNSPECIFIED.) ;
#131=B_SPLINE_CURVE_WITH_KNOTS('',3,(#104205,#104206,#104207,#104208,#104209,
#104210,#104211,#104212,#104213,#104214,#104215,#104216,#104217,#104218),
 .UNSPECIFIED.,.F.,.F.,(4,2,2,2,2,2,4),(1.44901762819747E-6,0.000561621523735244,
0.00112173034317294,0.00210338619144832,0.00384452539459816,0.00473112295166382,
0.00541108585598296),.UNSPECIFIED.) ;
#132=B_SPLINE_CURVE_WITH_KNOTS('',3,(#104227,#104228,#104229,#104230,#104231,
#104232,#104233,#104234,#104235,#104236,#104237,#104238,#104239,#104240,
#104241,#104242,#104243,#104244,#104245,#104246,#104247,#104248,#104249,
#104250,#104251,#104252,#104253,#104254,#104255,#104256,#104257,#104258,
#104259,#104260),.UNSPECIFIED.,.F.,.F.,(4,2,2,2,2,2,2,2,2,2,2,2,2,2,2,2,
4),(0.,1.67528894171568E-5,3.36326639087595E-5,3.532850036333E-5,3.67766442982351E-5,
4.45936877501458E-5,5.2562917199235E-5,5.37833548714877E-5,5.51649664473517E-5,
7.22376444475302E-5,7.35532885964682E-5,0.000109240736296779,0.000146228640920914,
0.000147106577192946,0.0002033591929484,0.000258123601948835,0.000294213154385907),
 .UNSPECIFIED.) ;
#133=B_SPLINE_CURVE_WITH_KNOTS('',3,(#104264,#104265,#104266,#104267,#104268,
#104269,#104270,#104271,#104272,#104273,#104274,#104275,#104276,#104277,
#104278,#104279,#104280,#104281,#104282,#104283,#104284,#104285,#104286,
#104287,#104288,#104289,#104290,#104291,#104292,#104293,#104294,#104295,
#104296,#104297,#104298,#104299,#104300,#104301,#104302,#104303,#104304,
#104305,#104306,#104307,#104308,#104309,#104310,#104311,#104312,#104313,
#104314,#104315),.UNSPECIFIED.,.F.,.F.,(4,3,3,3,3,3,3,3,3,3,3,3,3,3,3,3,
3,4),(0.,5.28180786102637E-5,0.00010788843028001,0.000143209193858987,0.000144078242180701,
0.000180086811859617,0.000214813790788482,0.000215458170263551,0.00021610254973862,
0.000232714940020857,0.00023410649251081,0.000238605983992196,0.000240855729732889,
0.000243105475473582,0.000250616089253232,0.000252108710851784,0.000270124214172475,
0.00028641838771798),.UNSPECIFIED.) ;
#134=B_SPLINE_CURVE_WITH_KNOTS('',3,(#104460,#104461,#104462,#104463,#104464,
#104465,#104466,#104467),.UNSPECIFIED.,.F.,.F.,(4,2,2,4),(-0.0473604779370388,
-0.0461995546884436,-0.0447198409510954,-0.0410407833884838),
 .UNSPECIFIED.) ;
#135=B_SPLINE_CURVE_WITH_KNOTS('',3,(#104475,#104476,#104477,#104478,#104479,
#104480,#104481,#104482),.UNSPECIFIED.,.F.,.F.,(4,2,2,4),(-0.0536801724855784,
-0.0500011149229823,-0.048521401185634,-0.0473604779370388),
 .UNSPECIFIED.) ;
#136=B_SPLINE_CURVE_WITH_KNOTS('',3,(#104936,#104937,#104938,#104939,#104940,
#104941,#104942,#104943,#104944,#104945,#104946,#104947,#104948,#104949),
 .UNSPECIFIED.,.F.,.F.,(4,2,2,2,2,2,4),(4.71238898038469,4.88175806245194,
5.06763701998947,5.24337922965538,5.26451333208261,5.4487409058292,5.49822830854821),
 .UNSPECIFIED.) ;
#137=B_SPLINE_CURVE_WITH_KNOTS('',3,(#104954,#104955,#104956,#104957,#104958,
#104959,#104960,#104961,#104962,#104963,#104964,#104965,#104966,#104967),
 .UNSPECIFIED.,.F.,.F.,(4,2,2,2,2,2,4),(0.78495699863134,0.966941694312354,
1.14311721213096,1.16348181627614,1.34745079132807,1.51752882030578,1.5707963267949),
 .UNSPECIFIED.) ;
#138=B_SPLINE_CURVE_WITH_KNOTS('',3,(#104973,#104974,#104975,#104976,#104977,
#104978,#104979,#104980,#104981,#104982,#104983,#104984,#104985,#104986),
 .UNSPECIFIED.,.F.,.F.,(4,2,2,2,2,2,4),(0.784956998631338,0.966941694312111,
1.14311721213157,1.16348181627597,1.34745079132821,1.51752882030615,1.5707963267949),
 .UNSPECIFIED.) ;
#139=B_SPLINE_CURVE_WITH_KNOTS('',3,(#104988,#104989,#104990,#104991,#104992,
#104993,#104994,#104995,#104996,#104997,#104998,#104999,#105000,#105001),
 .UNSPECIFIED.,.F.,.F.,(4,2,2,2,2,2,4),(4.71238898038469,4.88175806245166,
5.06763701998869,5.24337922965497,5.26451333208185,5.44874090582888,5.49822830854824),
 .UNSPECIFIED.) ;
#140=B_SPLINE_CURVE_WITH_KNOTS('',3,(#105005,#105006,#105007,#105008,#105009,
#105010,#105011,#105012,#105013,#105014,#105015,#105016,#105017,#105018),
 .UNSPECIFIED.,.F.,.F.,(4,2,2,2,2,2,4),(4.71238898038469,4.88175806245182,
5.06763701998925,5.24337922964886,5.26451333208237,5.44874090582905,5.49822830854823),
 .UNSPECIFIED.) ;
#141=B_SPLINE_CURVE_WITH_KNOTS('',3,(#105022,#105023,#105024,#105025,#105026,
#105027,#105028,#105029,#105030,#105031,#105032,#105033,#105034,#105035),
 .UNSPECIFIED.,.F.,.F.,(4,2,2,2,2,2,4),(0.784956998631348,0.966941694311913,
1.14311721213295,1.16348181627588,1.34745079132843,1.51752882030647,1.5707963267949),
 .UNSPECIFIED.) ;
#142=B_SPLINE_CURVE_WITH_KNOTS('',3,(#105050,#105051,#105052,#105053,#105054,
#105055,#105056,#105057,#105058,#105059,#105060,#105061,#105062,#105063),
 .UNSPECIFIED.,.F.,.F.,(4,2,2,2,2,2,4),(0.784956998631365,0.966941694311873,
1.14311721213002,1.16348181627585,1.34745079132852,1.51752882030655,1.5707963267949),
 .UNSPECIFIED.) ;
#143=B_SPLINE_CURVE_WITH_KNOTS('',3,(#105067,#105068,#105069,#105070,#105071,
#105072,#105073,#105074,#105075,#105076,#105077,#105078,#105079,#105080),
 .UNSPECIFIED.,.F.,.F.,(4,2,2,2,2,2,4),(4.71238898038469,4.88175806245151,
5.06763701998819,5.24337922965584,5.26451333208124,5.4487409058285,5.49822830854824),
 .UNSPECIFIED.) ;
#144=B_SPLINE_CURVE_WITH_KNOTS('',3,(#105185,#105186,#105187,#105188,#105189,
#105190,#105191,#105192,#105193,#105194,#105195,#105196,#105197,#105198,
#105199,#105200),.UNSPECIFIED.,.F.,.F.,(4,3,3,3,3,4),(0.,3.26760986414935E-5,
6.60604127813367E-5,0.00010113572426573,0.000138237800333083,0.000166242991827323),
 .UNSPECIFIED.) ;
#145=B_SPLINE_CURVE_WITH_KNOTS('',3,(#105262,#105263,#105264,#105265,#105266,
#105267,#105268,#105269,#105270,#105271,#105272,#105273,#105274,#105275,
#105276,#105277),.UNSPECIFIED.,.F.,.F.,(4,3,3,3,3,4),(0.,1.86901632150157E-5,
5.38940239621529E-5,9.13255451816918E-5,0.000129775966053829,0.000168373497604196),
 .UNSPECIFIED.) ;
#146=B_SPLINE_CURVE_WITH_KNOTS('',3,(#105282,#105283,#105284,#105285,#105286,
#105287,#105288,#105289,#105290,#105291),.UNSPECIFIED.,.F.,.F.,(4,2,2,2,
4),(0.0288531015801791,0.0296205843570608,0.0328031056810013,0.0376042554610398,
0.0407130021432729),.UNSPECIFIED.) ;
#147=B_SPLINE_CURVE_WITH_KNOTS('',3,(#105296,#105297,#105298,#105299,#105300,
#105301),.UNSPECIFIED.,.F.,.F.,(4,2,4),(0.063747484019213,0.0675088661241108,
0.0720284409363993),.UNSPECIFIED.) ;
#148=B_SPLINE_CURVE_WITH_KNOTS('',3,(#105307,#105308,#105309,#105310,#105311,
#105312,#105313,#105314,#105315,#105316),.UNSPECIFIED.,.F.,.F.,(4,2,2,2,
4),(0.0767275662235905,0.0771734766300911,0.0818220866830681,0.0868722195329092,
0.0892832637319672),.UNSPECIFIED.) ;
#149=B_SPLINE_CURVE_WITH_KNOTS('',3,(#105351,#105352,#105353,#105354,#105355,
#105356),.UNSPECIFIED.,.F.,.F.,(4,2,4),(0.171679973604201,0.178707475947309,
0.186889989698777),.UNSPECIFIED.) ;
#150=B_SPLINE_CURVE_WITH_KNOTS('',3,(#105396,#105397,#105398,#105399,#105400,
#105401,#105402,#105403,#105404,#105405,#105406,#105407,#105408,#105409,
#105410,#105411,#105412,#105413,#105414,#105415,#105416,#105417,#105418,
#105419,#105420,#105421,#105422,#105423,#105424,#105425),.UNSPECIFIED.,
 .F.,.F.,(4,2,2,2,2,2,2,2,2,2,2,2,2,2,4),(2.36970964942748,2.55498029688299,
2.73514427896706,2.74569929646378,2.92071305421126,2.93943382978513,3.11857096684179,
3.13197658032393,3.25399179664495,3.45054278261475,3.62794535799811,3.64606212534864,
3.82474099483732,3.83698255062522,3.91347421315246),.UNSPECIFIED.) ;
#151=B_SPLINE_CURVE_WITH_KNOTS('',3,(#105436,#105437,#105438,#105439,#105440,
#105441,#105442,#105443,#105444,#105445,#105446,#105447,#105448,#105449,
#105450,#105451,#105452,#105453,#105454,#105455,#105456,#105457,#105458,
#105459,#105460,#105461),.UNSPECIFIED.,.F.,.F.,(4,2,2,2,2,2,2,2,2,2,2,2,
4),(2.70344464881055,2.89144352771225,3.06851986332573,3.08081089074492,
3.26996664970766,3.35940092938473,3.5458754301802,3.72254345721718,3.73903833379462,
3.91570024693468,3.93052100184901,4.11735511986399,4.22222897897866),
 .UNSPECIFIED.) ;
#152=B_SPLINE_CURVE_WITH_KNOTS('',3,(#105619,#105620,#105621,#105622,#105623,
#105624,#105625,#105626,#105627,#105628,#105629,#105630,#105631,#105632,
#105633,#105634,#105635,#105636,#105637),.UNSPECIFIED.,.F.,.F.,(4,3,3,3,
3,3,4),(2.81004151703333E-8,3.99307614181576E-5,8.00540716903473E-5,0.000126830846822484,
0.00017561819518642,0.00021519314047228,0.000245220898756746),
 .UNSPECIFIED.) ;
#153=B_SPLINE_CURVE_WITH_KNOTS('',3,(#105660,#105661,#105662,#105663,#105664,
#105665,#105666,#105667,#105668,#105669,#105670,#105671,#105672,#105673,
#105674,#105675,#105676,#105677,#105678,#105679,#105680,#105681,#105682,
#105683,#105684,#105685,#105686,#105687,#105688,#105689,#105690,#105691,
#105692,#105693,#105694,#105695,#105696,#105697,#105698,#105699,#105700,
#105701,#105702,#105703,#105704,#105705,#105706,#105707,#105708,#105709,
#105710,#105711,#105712,#105713,#105714,#105715,#105716,#105717,#105718,
#105719,#105720,#105721,#105722,#105723,#105724,#105725,#105726,#105727,
#105728,#105729,#105730,#105731,#105732,#105733,#105734,#105735,#105736,
#105737,#105738),.UNSPECIFIED.,.F.,.F.,(4,3,3,3,3,3,3,3,3,3,3,3,3,3,3,3,
3,3,3,3,3,3,3,3,3,3,4),(0.000152038190191021,0.000154892841408471,0.000155160464960107,
0.000160456565729371,0.000163456795060821,0.000166580092246908,0.00016775132869169,
0.000168007536663986,0.000168255738137148,0.000169267315291303,0.000175949983805168,
0.000178959298271447,0.000180334649023613,0.000187987241670282,0.00019198121640859,
0.000193065528939067,0.00019383917426517,0.000198143816207851,0.000212206269476815,
0.000226582370019607,0.000228143757087823,0.000228729277238404,0.000232827918292471,
0.00024910943281953,0.00025017679744092,0.000265881325830107,0.000267525676589369),
 .UNSPECIFIED.) ;
#154=B_SPLINE_CURVE_WITH_KNOTS('',3,(#105740,#105741,#105742,#105743,#105744,
#105745,#105746,#105747,#105748,#105749),.UNSPECIFIED.,.F.,.F.,(4,3,3,4),
(0.000130631741230759,0.000139067346352796,0.000143554831048674,0.000152038189371587),
 .UNSPECIFIED.) ;
#155=B_SPLINE_CURVE_WITH_KNOTS('',3,(#105751,#105752,#105753,#105754,#105755,
#105756,#105757,#105758,#105759,#105760,#105761,#105762,#105763,#105764,
#105765,#105766,#105767,#105768,#105769),.UNSPECIFIED.,.F.,.F.,(4,3,3,3,
3,3,4),(0.000104137230127934,0.000110259474166471,0.000116844366893148,
0.000120664217590266,0.000125429508057305,0.000130430624030549,0.000130630877723017),
 .UNSPECIFIED.) ;
#156=B_SPLINE_CURVE_WITH_KNOTS('',3,(#105770,#105771,#105772,#105773,#105774,
#105775,#105776,#105777,#105778,#105779,#105780,#105781,#105782,#105783,
#105784,#105785,#105786,#105787,#105788,#105789,#105790,#105791,#105792,
#105793,#105794,#105795,#105796,#105797,#105798,#105799,#105800,#105801,
#105802,#105803,#105804,#105805,#105806,#105807,#105808,#105809,#105810,
#105811,#105812),.UNSPECIFIED.,.F.,.F.,(4,3,3,3,3,3,3,3,3,3,3,3,3,3,4),
(0.,4.78421531964037E-6,1.59977421331184E-5,1.75965265774506E-5,2.6360366765448E-5,
3.75047088104788E-5,4.29655082836413E-5,5.3450780665109E-5,6.17416442237089E-5,
6.39360530465768E-5,7.32944438958948E-5,8.49065978095123E-5,9.46209320474951E-5,
9.66050857869684E-5,0.000104137229466949),.UNSPECIFIED.) ;
#157=B_SPLINE_CURVE_WITH_KNOTS('',3,(#105882,#105883,#105884,#105885,#105886,
#105887,#105888,#105889,#105890,#105891,#105892,#105893,#105894,#105895,
#105896,#105897,#105898,#105899,#105900,#105901,#105902,#105903,#105904,
#105905,#105906,#105907,#105908,#105909,#105910,#105911,#105912,#105913,
#105914,#105915),.UNSPECIFIED.,.F.,.F.,(4,3,3,3,3,3,3,3,3,3,3,4),(0.000173579735006482,
0.000179152672590559,0.000187122196212438,0.000190349677855741,0.000201571576239487,
0.000207505544696553,0.000209082158340111,0.000218112358783938,0.000219837174422809,
0.000228512621317814,0.000240802935332003,0.000245138123631297),
 .UNSPECIFIED.) ;
#158=B_SPLINE_CURVE_WITH_KNOTS('',3,(#105977,#105978,#105979,#105980,#105981,
#105982,#105983,#105984,#105985,#105986,#105987,#105988,#105989,#105990,
#105991,#105992),.UNSPECIFIED.,.F.,.F.,(4,3,3,3,3,4),(0.000149826268238821,
0.000156541783273878,0.000187447062839771,0.000218157419331144,0.000251253590119497,
0.000263630362845938),.UNSPECIFIED.) ;
#159=B_SPLINE_CURVE_WITH_KNOTS('',3,(#105994,#105995,#105996,#105997),
 .UNSPECIFIED.,.F.,.F.,(4,4),(0.000128945525003057,0.000149826268238821),
 .UNSPECIFIED.) ;
#160=B_SPLINE_CURVE_WITH_KNOTS('',3,(#105998,#105999,#106000,#106001,#106002,
#106003,#106004,#106005,#106006,#106007,#106008,#106009,#106010,#106011,
#106012,#106013),.UNSPECIFIED.,.F.,.F.,(4,3,3,3,3,4),(0.000107977862661221,
0.000113849696954291,0.00011675864089999,0.000123355930725607,0.000128649321338309,
0.000128945525003057),.UNSPECIFIED.) ;
#161=B_SPLINE_CURVE_WITH_KNOTS('',3,(#106223,#106224,#106225,#106226,#106227,
#106228,#106229,#106230,#106231,#106232),.UNSPECIFIED.,.F.,.F.,(4,3,3,4),
(3.97436543900202E-15,3.94729529730262E-5,7.90727202189655E-5,0.000103003463696588),
 .UNSPECIFIED.) ;
#162=B_SPLINE_CURVE_WITH_KNOTS('',3,(#106239,#106240,#106241,#106242,#106243,
#106244,#106245),.UNSPECIFIED.,.F.,.F.,(4,3,4),(0.000158223357507084,0.000179871364136752,
0.000191820073778124),.UNSPECIFIED.) ;
#163=B_SPLINE_CURVE_WITH_KNOTS('',3,(#106260,#106261,#106262,#106263,#106264,
#106265,#106266,#106267,#106268,#106269,#106270,#106271,#106272,#106273,
#106274,#106275),.UNSPECIFIED.,.F.,.F.,(4,3,3,3,3,4),(2.25414513257385E-8,
3.7118138109435E-5,7.40234349159874E-5,0.000126639028433408,0.000171180683285943,
0.000173579731706481),.UNSPECIFIED.) ;
#164=B_SPLINE_CURVE_WITH_KNOTS('',3,(#106331,#106332,#106333,#106334,#106335,
#106336),.UNSPECIFIED.,.F.,.F.,(4,2,4),(0.,0.000162685424844482,0.000325370849688964),
 .UNSPECIFIED.) ;
#165=B_SPLINE_CURVE_WITH_KNOTS('',3,(#106339,#106340,#106341,#106342,#106343,
#106344),.UNSPECIFIED.,.F.,.F.,(4,2,4),(0.,0.000163438694679259,0.000326877389358518),
 .UNSPECIFIED.) ;
#166=B_SPLINE_CURVE_WITH_KNOTS('',3,(#106355,#106356,#106357,#106358,#106359,
#106360),.UNSPECIFIED.,.F.,.F.,(4,2,4),(-0.00501427184001376,-0.00354643693242498,
0.),.UNSPECIFIED.) ;
#167=B_SPLINE_CURVE_WITH_KNOTS('',3,(#106373,#106374,#106375,#106376,#106377,
#106378,#106379,#106380,#106381,#106382,#106383,#106384,#106385,#106386,
#106387,#106388,#106389,#106390,#106391,#106392,#106393,#106394,#106395,
#106396,#106397,#106398,#106399,#106400),.UNSPECIFIED.,.F.,.F.,(4,3,3,3,
3,3,3,3,3,4),(5.2381062129225E-9,5.84794260519105E-6,8.49662041781866E-6,
1.21937803558578E-5,1.76033670137842E-5,1.93092034273014E-5,2.55871453405162E-5,
3.0315421636347E-5,3.68519660350372E-5,3.92146766969318E-5),
 .UNSPECIFIED.) ;
#168=B_SPLINE_CURVE_WITH_KNOTS('',3,(#106402,#106403,#106404,#106405,#106406,
#106407,#106408,#106409,#106410,#106411),.UNSPECIFIED.,.F.,.F.,(4,3,3,4),
(0.000144469795965457,0.000165397602015722,0.000173816468562375,0.000175865847906017),
 .UNSPECIFIED.) ;
#169=B_SPLINE_CURVE_WITH_KNOTS('',3,(#106429,#106430,#106431,#106432,#106433,
#106434,#106435),.UNSPECIFIED.,.F.,.F.,(4,3,4),(-2.05331166617142E-6,2.04386714309068E-5,
3.1629985593225E-5),.UNSPECIFIED.) ;
#170=B_SPLINE_CURVE_WITH_KNOTS('',3,(#106437,#106438,#106439,#106440,#106441,
#106442,#106443,#106444,#106445,#106446,#106447,#106448),.UNSPECIFIED.,
 .F.,.F.,(4,2,2,2,2,4),(9.00279624299152E-9,0.00183032786957268,0.006077465667517,
0.0169681635237984,0.0216775196496615,0.0254454421850849),.UNSPECIFIED.) ;
#171=B_SPLINE_CURVE_WITH_KNOTS('',3,(#106607,#106608,#106609,#106610,#106611,
#106612,#106613,#106614,#106615,#106616,#106617,#106618,#106619,#106620,
#106621,#106622,#106623,#106624,#106625,#106626,#106627,#106628,#106629,
#106630,#106631,#106632,#106633,#106634,#106635,#106636,#106637,#106638,
#106639,#106640,#106641,#106642,#106643,#106644,#106645,#106646),
 .UNSPECIFIED.,.F.,.F.,(4,3,3,3,3,3,3,3,3,3,3,3,3,4),(0.,5.07173230218452E-5,
0.00010401741348744,0.000124506719166651,0.000125249568192438,0.000156566023859653,
0.000186760078749975,0.000187880030991798,0.000203537318084809,0.000211366035547463,
0.000217886758541637,0.000219194644848643,0.000234851354133269,0.000249013438333299),
 .UNSPECIFIED.) ;
#172=B_SPLINE_CURVE_WITH_KNOTS('',3,(#106652,#106653,#106654,#106655,#106656,
#106657,#106658,#106659,#106660,#106661,#106662,#106663,#106664,#106665,
#106666,#106667,#106668,#106669,#106670,#106671,#106672,#106673,#106674,
#106675,#106676,#106677,#106678,#106679,#106680,#106681,#106682,#106683,
#106684,#106685,#106686,#106687,#106688,#106689,#106690,#106691),
 .UNSPECIFIED.,.F.,.F.,(4,3,3,3,3,3,3,3,3,3,3,3,3,4),(0.,1.4311556709258E-5,
3.01335133960352E-5,3.14552036774726E-5,3.80447517297281E-5,4.59561222518464E-5,
6.17788922892798E-5,6.29104073549452E-5,9.34210966965093E-5,0.000125066393795483,
0.000125820814709883,0.000179837268173055,0.000231469985679291,0.000251641629419759),
 .UNSPECIFIED.) ;
#173=B_SPLINE_CURVE_WITH_KNOTS('',3,(#106696,#106697,#106698,#106699,#106700,
#106701,#106702),.UNSPECIFIED.,.F.,.F.,(4,3,4),(-2.04939766627128E-6,0.,
2.93835791072157E-5),.UNSPECIFIED.) ;
#174=B_SPLINE_CURVE_WITH_KNOTS('',3,(#106717,#106718,#106719,#106720,#106721,
#106722,#106723,#106724,#106725,#106726,#106727,#106728,#106729,#106730),
 .UNSPECIFIED.,.F.,.F.,(4,2,2,2,2,2,4),(1.44901762686856E-6,0.000561621523786212,
0.00112173034325288,0.00210338619152427,0.00384452539434926,0.00473112295079285,
0.00541108585487423),.UNSPECIFIED.) ;
#175=B_SPLINE_CURVE_WITH_KNOTS('',3,(#106739,#106740,#106741,#106742,#106743,
#106744,#106745,#106746,#106747,#106748,#106749,#106750,#106751,#106752,
#106753,#106754,#106755,#106756,#106757,#106758,#106759,#106760,#106761,
#106762,#106763,#106764,#106765,#106766,#106767,#106768,#106769,#106770,
#106771,#106772),.UNSPECIFIED.,.F.,.F.,(4,2,2,2,2,2,2,2,2,2,2,2,2,2,2,2,
4),(0.,1.6752889417125E-5,3.36326639084849E-5,3.53285003632986E-5,3.67766442982582E-5,
4.4593687750131E-5,5.25629171995868E-5,5.37833548715131E-5,5.51649664473856E-5,
7.22376444476005E-5,7.35532885965131E-5,0.000109240736296885,0.000146228640921016,
0.000147106577193024,0.000203359192940443,0.000258123601934358,0.000294213154386043),
 .UNSPECIFIED.) ;
#176=B_SPLINE_CURVE_WITH_KNOTS('',3,(#106776,#106777,#106778,#106779,#106780,
#106781,#106782,#106783,#106784,#106785,#106786,#106787,#106788,#106789,
#106790,#106791,#106792,#106793,#106794,#106795,#106796,#106797,#106798,
#106799,#106800,#106801,#106802,#106803,#106804,#106805,#106806,#106807,
#106808,#106809,#106810,#106811,#106812,#106813,#106814,#106815,#106816,
#106817,#106818,#106819,#106820,#106821,#106822,#106823,#106824,#106825,
#106826,#106827),.UNSPECIFIED.,.F.,.F.,(4,3,3,3,3,3,3,3,3,3,3,3,3,3,3,3,
3,4),(0.,5.28180786064093E-5,0.000107888430271973,0.000143209193858987,
0.00014407824218072,0.000180086811859619,0.00021481379078848,0.00021545817026355,
0.00021610254973862,0.000232714940020853,0.000234106492510808,0.000238605983992193,
0.000240855729732885,0.000243105475473578,0.000250616089253225,0.000252108710851782,
0.000270124214172477,0.000286418387717971),.UNSPECIFIED.) ;
#177=B_SPLINE_CURVE_WITH_KNOTS('',3,(#106972,#106973,#106974,#106975,#106976,
#106977,#106978,#106979),.UNSPECIFIED.,.F.,.F.,(4,2,2,4),(-0.0473604779370388,
-0.0461995546884437,-0.0447198409510955,-0.0410407833884838),
 .UNSPECIFIED.) ;
#178=B_SPLINE_CURVE_WITH_KNOTS('',3,(#106987,#106988,#106989,#106990,#106991,
#106992,#106993,#106994),.UNSPECIFIED.,.F.,.F.,(4,2,2,4),(-0.0536801724855783,
-0.0500011149229821,-0.0485214011856339,-0.0473604779370387),
 .UNSPECIFIED.) ;
#179=B_SPLINE_CURVE_WITH_KNOTS('',3,(#107448,#107449,#107450,#107451,#107452,
#107453,#107454,#107455,#107456,#107457,#107458,#107459,#107460,#107461),
 .UNSPECIFIED.,.F.,.F.,(4,2,2,2,2,2,4),(4.71238898038469,4.88175806245169,
5.06763701998897,5.24337922960769,5.26451333208202,5.44874090582883,5.49822830854825),
 .UNSPECIFIED.) ;
#180=B_SPLINE_CURVE_WITH_KNOTS('',3,(#107466,#107467,#107468,#107469,#107470,
#107471,#107472,#107473,#107474,#107475,#107476,#107477,#107478,#107479),
 .UNSPECIFIED.,.F.,.F.,(4,2,2,2,2,2,4),(0.784956998631304,0.966941694312144,
1.14311721221009,1.16348181627612,1.34745079132841,1.51752882030647,1.5707963267949),
 .UNSPECIFIED.) ;
#181=B_SPLINE_CURVE_WITH_KNOTS('',3,(#107485,#107486,#107487,#107488,#107489,
#107490,#107491,#107492,#107493,#107494,#107495,#107496,#107497,#107498),
 .UNSPECIFIED.,.F.,.F.,(4,2,2,2,2,2,4),(0.784956998631347,0.966941694312202,
1.1431172121312,1.16348181627609,1.34745079132826,1.51752882030624,1.5707963267949),
 .UNSPECIFIED.) ;
#182=B_SPLINE_CURVE_WITH_KNOTS('',3,(#107500,#107501,#107502,#107503,#107504,
#107505,#107506,#107507,#107508,#107509,#107510,#107511,#107512,#107513),
 .UNSPECIFIED.,.F.,.F.,(4,2,2,2,2,2,4),(4.71238898038469,4.88175806245171,
5.06763701998877,5.24337922965479,5.26451333208194,5.44874090582893,5.49822830854826),
 .UNSPECIFIED.) ;
#183=B_SPLINE_CURVE_WITH_KNOTS('',3,(#107517,#107518,#107519,#107520,#107521,
#107522,#107523,#107524,#107525,#107526,#107527,#107528,#107529,#107530),
 .UNSPECIFIED.,.F.,.F.,(4,2,2,2,2,2,4),(4.71238898038469,4.88175806245169,
5.06763701998911,5.2433792296566,5.26451333208232,5.44874090582905,5.49822830854824),
 .UNSPECIFIED.) ;
#184=B_SPLINE_CURVE_WITH_KNOTS('',3,(#107534,#107535,#107536,#107537,#107538,
#107539,#107540,#107541,#107542,#107543,#107544,#107545,#107546,#107547),
 .UNSPECIFIED.,.F.,.F.,(4,2,2,2,2,2,4),(0.784956998631345,0.966941694311759,
1.14311721212769,1.16348181627571,1.34745079132821,1.5175288203063,1.5707963267949),
 .UNSPECIFIED.) ;
#185=B_SPLINE_CURVE_WITH_KNOTS('',3,(#107562,#107563,#107564,#107565,#107566,
#107567,#107568,#107569,#107570,#107571,#107572,#107573,#107574,#107575),
 .UNSPECIFIED.,.F.,.F.,(4,2,2,2,2,2,4),(0.784956998631335,0.966941694312017,
1.14311721212471,1.16348181627591,1.34745079132842,1.5175288203063,1.5707963267949),
 .UNSPECIFIED.) ;
#186=B_SPLINE_CURVE_WITH_KNOTS('',3,(#107579,#107580,#107581,#107582,#107583,
#107584,#107585,#107586,#107587,#107588,#107589,#107590,#107591,#107592),
 .UNSPECIFIED.,.F.,.F.,(4,2,2,2,2,2,4),(4.71238898038469,4.88175806245169,
5.06763701998889,5.24337922965042,5.26451333208206,5.44874090582913,5.49822830854829),
 .UNSPECIFIED.) ;
#187=B_SPLINE_CURVE_WITH_KNOTS('',3,(#107697,#107698,#107699,#107700,#107701,
#107702,#107703,#107704,#107705,#107706,#107707,#107708,#107709,#107710,
#107711,#107712),.UNSPECIFIED.,.F.,.F.,(4,3,3,3,3,4),(0.,3.26760986414935E-5,
6.60604127813372E-5,0.00010113572426573,0.000138237800333083,0.000166242991827321),
 .UNSPECIFIED.) ;
#188=B_SPLINE_CURVE_WITH_KNOTS('',3,(#107774,#107775,#107776,#107777,#107778,
#107779,#107780,#107781,#107782,#107783,#107784,#107785,#107786,#107787,
#107788,#107789),.UNSPECIFIED.,.F.,.F.,(4,3,3,3,3,4),(0.,1.86901632150156E-5,
5.38940239621536E-5,9.1325545181693E-5,0.00012977596605383,0.000168373497604197),
 .UNSPECIFIED.) ;
#189=B_SPLINE_CURVE_WITH_KNOTS('',3,(#107794,#107795,#107796,#107797,#107798,
#107799,#107800,#107801,#107802,#107803),.UNSPECIFIED.,.F.,.F.,(4,2,2,2,
4),(0.0288531015833118,0.0296205843603292,0.0328031056847702,0.0376042554655217,
0.0407130021481444),.UNSPECIFIED.) ;
#190=B_SPLINE_CURVE_WITH_KNOTS('',3,(#107808,#107809,#107810,#107811,#107812,
#107813),.UNSPECIFIED.,.F.,.F.,(4,2,4),(0.0637474840407795,0.0675088661482764,
0.0720284409638634),.UNSPECIFIED.) ;
#191=B_SPLINE_CURVE_WITH_KNOTS('',3,(#107819,#107820,#107821,#107822,#107823,
#107824,#107825,#107826,#107827,#107828),.UNSPECIFIED.,.F.,.F.,(4,2,2,2,
4),(0.0767275662236361,0.0771734766301334,0.0818220866832597,0.0868722195332896,
0.0892832637324438),.UNSPECIFIED.) ;
#192=B_SPLINE_CURVE_WITH_KNOTS('',3,(#107863,#107864,#107865,#107866,#107867,
#107868),.UNSPECIFIED.,.F.,.F.,(4,2,4),(0.171679973605268,0.17870747594849,
0.186889989700107),.UNSPECIFIED.) ;
#193=B_SPLINE_CURVE_WITH_KNOTS('',3,(#107908,#107909,#107910,#107911,#107912,
#107913,#107914,#107915,#107916,#107917,#107918,#107919,#107920,#107921,
#107922,#107923,#107924,#107925,#107926,#107927,#107928,#107929,#107930,
#107931,#107932,#107933,#107934,#107935,#107936,#107937),.UNSPECIFIED.,
 .F.,.F.,(4,2,2,2,2,2,2,2,2,2,2,2,2,2,4),(2.36970964942748,2.55498029688296,
2.73514427897508,2.74569929646384,2.92071305423067,2.9394338297853,3.11857096686515,
3.13197658032419,3.25399179664505,3.450542782615,3.62794535799348,3.64606212534887,
3.82474099482299,3.83698255062533,3.9134742131517),.UNSPECIFIED.) ;
#194=B_SPLINE_CURVE_WITH_KNOTS('',3,(#107948,#107949,#107950,#107951,#107952,
#107953,#107954,#107955,#107956,#107957,#107958,#107959,#107960,#107961,
#107962,#107963,#107964,#107965,#107966,#107967,#107968,#107969,#107970,
#107971,#107972,#107973),.UNSPECIFIED.,.F.,.F.,(4,2,2,2,2,2,2,2,2,2,2,2,
4),(2.70344464881042,2.89144352771213,3.06851986339517,3.0808108907447,
3.26996664970742,3.35940092938473,3.54587543017995,3.72254345721779,3.73903833379426,
3.91570024691714,3.93052100184844,4.11735511986315,4.22222897897866),
 .UNSPECIFIED.) ;
#195=B_SPLINE_CURVE_WITH_KNOTS('',3,(#108131,#108132,#108133,#108134,#108135,
#108136,#108137,#108138,#108139,#108140,#108141,#108142,#108143,#108144,
#108145,#108146,#108147,#108148,#108149),.UNSPECIFIED.,.F.,.F.,(4,3,3,3,
3,3,4),(2.81004151523444E-8,3.99307614181576E-5,8.00540716903464E-5,0.000126830846822483,
0.000175618195186419,0.000215193140472279,0.00024522089875675),
 .UNSPECIFIED.) ;
#196=B_SPLINE_CURVE_WITH_KNOTS('',3,(#108172,#108173,#108174,#108175,#108176,
#108177,#108178,#108179,#108180,#108181,#108182,#108183,#108184,#108185,
#108186,#108187,#108188,#108189,#108190,#108191,#108192,#108193,#108194,
#108195,#108196,#108197,#108198,#108199,#108200,#108201,#108202,#108203,
#108204,#108205,#108206,#108207,#108208,#108209,#108210,#108211,#108212,
#108213,#108214,#108215,#108216,#108217,#108218,#108219,#108220,#108221,
#108222,#108223,#108224,#108225,#108226,#108227,#108228,#108229,#108230,
#108231,#108232,#108233,#108234,#108235,#108236,#108237,#108238,#108239,
#108240,#108241,#108242,#108243,#108244,#108245,#108246,#108247,#108248,
#108249,#108250),.UNSPECIFIED.,.F.,.F.,(4,3,3,3,3,3,3,3,3,3,3,3,3,3,3,3,
3,3,3,3,3,3,3,3,3,3,4),(0.000152038190191199,0.000154892841408555,0.000155160464960188,
0.000160456565729593,0.000163456795060823,0.000166580092246912,0.000167751328691695,
0.000168007536663992,0.000168255738137154,0.000169267315291292,0.000175949983805179,
0.000178959298271457,0.000180334649023622,0.000187987241670289,0.000191981216408587,
0.000193065528939071,0.000193839174265175,0.000198143816207854,0.000212206269476809,
0.000226582370019589,0.00022814375708781,0.000228729277238393,0.000232827918292474,
0.000249109432810095,0.000250176797440924,0.000265881325831287,0.000267525676589373),
 .UNSPECIFIED.) ;
#197=B_SPLINE_CURVE_WITH_KNOTS('',3,(#108252,#108253,#108254,#108255,#108256,
#108257,#108258,#108259,#108260,#108261),.UNSPECIFIED.,.F.,.F.,(4,3,3,4),
(0.000130631741230765,0.000139067346353096,0.000143554831048713,0.000152038189371763),
 .UNSPECIFIED.) ;
#198=B_SPLINE_CURVE_WITH_KNOTS('',3,(#108263,#108264,#108265,#108266,#108267,
#108268,#108269,#108270,#108271,#108272,#108273,#108274,#108275,#108276,
#108277,#108278,#108279,#108280,#108281),.UNSPECIFIED.,.F.,.F.,(4,3,3,3,
3,3,4),(0.000104137230128489,0.000110259474166938,0.000116844366893606,
0.00012066421759078,0.000125429508057306,0.000130430624030732,0.000130630877723054),
 .UNSPECIFIED.) ;
#199=B_SPLINE_CURVE_WITH_KNOTS('',3,(#108282,#108283,#108284,#108285,#108286,
#108287,#108288,#108289,#108290,#108291,#108292,#108293,#108294,#108295,
#108296,#108297,#108298,#108299,#108300,#108301,#108302,#108303,#108304,
#108305,#108306,#108307,#108308,#108309,#108310,#108311,#108312,#108313,
#108314,#108315,#108316,#108317,#108318,#108319,#108320,#108321,#108322,
#108323,#108324),.UNSPECIFIED.,.F.,.F.,(4,3,3,3,3,3,3,3,3,3,3,3,3,3,4),
(0.,4.78421531964207E-6,1.5997742133728E-5,1.75965265776594E-5,2.63603667652772E-5,
3.75047088100453E-5,4.29655082836422E-5,5.34507806651101E-5,6.17416442235669E-5,
6.39360530465779E-5,7.32944438965259E-5,8.49065978095135E-5,9.46209320476381E-5,
9.66050857869696E-5,0.000104137229467517),.UNSPECIFIED.) ;
#200=B_SPLINE_CURVE_WITH_KNOTS('',3,(#108394,#108395,#108396,#108397,#108398,
#108399,#108400,#108401,#108402,#108403,#108404,#108405,#108406,#108407,
#108408,#108409,#108410,#108411,#108412,#108413,#108414,#108415,#108416,
#108417,#108418,#108419,#108420,#108421,#108422,#108423,#108424,#108425,
#108426,#108427),.UNSPECIFIED.,.F.,.F.,(4,3,3,3,3,3,3,3,3,3,3,4),(0.00017357973500648,
0.000179152672590604,0.000187122196212524,0.000190349677855844,0.000201571576239683,
0.000207505544696743,0.00020908215834011,0.000218112358783795,0.000219837174422841,
0.000228512621317681,0.00024080293533128,0.000245138123631291),
 .UNSPECIFIED.) ;
#201=B_SPLINE_CURVE_WITH_KNOTS('',3,(#108489,#108490,#108491,#108492,#108493,
#108494,#108495,#108496,#108497,#108498,#108499,#108500,#108501,#108502,
#108503,#108504),.UNSPECIFIED.,.F.,.F.,(4,3,3,3,3,4),(0.000149826268238863,
0.000156541783273878,0.000187447062839773,0.000218157419331147,0.0002512535901195,
0.000263630362845944),.UNSPECIFIED.) ;
#202=B_SPLINE_CURVE_WITH_KNOTS('',3,(#108506,#108507,#108508,#108509),
 .UNSPECIFIED.,.F.,.F.,(4,4),(0.00012894552500308,0.000149826268238863),
 .UNSPECIFIED.) ;
#203=B_SPLINE_CURVE_WITH_KNOTS('',3,(#108510,#108511,#108512,#108513,#108514,
#108515,#108516,#108517,#108518,#108519,#108520,#108521,#108522,#108523,
#108524,#108525),.UNSPECIFIED.,.F.,.F.,(4,3,3,3,3,4),(0.000107977862661225,
0.000113849696954203,0.00011675864089999,0.000123355930725642,0.000128649321338296,
0.00012894552500308),.UNSPECIFIED.) ;
#204=B_SPLINE_CURVE_WITH_KNOTS('',3,(#108735,#108736,#108737,#108738,#108739,
#108740,#108741,#108742,#108743,#108744),.UNSPECIFIED.,.F.,.F.,(4,3,3,4),
(3.97436543900202E-15,3.94729529730262E-5,7.90727202189655E-5,0.000103003463696568),
 .UNSPECIFIED.) ;
#205=B_SPLINE_CURVE_WITH_KNOTS('',3,(#108751,#108752,#108753,#108754,#108755,
#108756,#108757),.UNSPECIFIED.,.F.,.F.,(4,3,4),(0.000158223357507064,0.000179871364136604,
0.000191820073778122),.UNSPECIFIED.) ;
#206=B_SPLINE_CURVE_WITH_KNOTS('',3,(#108772,#108773,#108774,#108775,#108776,
#108777,#108778,#108779,#108780,#108781,#108782,#108783,#108784,#108785,
#108786,#108787),.UNSPECIFIED.,.F.,.F.,(4,3,3,3,3,4),(2.25414513247713E-8,
3.7118138109435E-5,7.40234349159874E-5,0.000126639028433408,0.000171180683285943,
0.000173579731706481),.UNSPECIFIED.) ;
#207=B_SPLINE_CURVE_WITH_KNOTS('',3,(#108843,#108844,#108845,#108846,#108847,
#108848),.UNSPECIFIED.,.F.,.F.,(4,2,4),(0.,0.000162685424844483,0.000325370849688965),
 .UNSPECIFIED.) ;
#208=B_SPLINE_CURVE_WITH_KNOTS('',3,(#108851,#108852,#108853,#108854,#108855,
#108856),.UNSPECIFIED.,.F.,.F.,(4,2,4),(0.,0.000163438694679259,0.000326877389358518),
 .UNSPECIFIED.) ;
#209=B_SPLINE_CURVE_WITH_KNOTS('',3,(#108867,#108868,#108869,#108870,#108871,
#108872),.UNSPECIFIED.,.F.,.F.,(4,2,4),(-0.00501427184001376,-0.00354643693242498,
0.),.UNSPECIFIED.) ;
#210=B_SPLINE_CURVE_WITH_KNOTS('',3,(#108885,#108886,#108887,#108888,#108889,
#108890,#108891,#108892,#108893,#108894,#108895,#108896,#108897,#108898,
#108899,#108900,#108901,#108902,#108903,#108904,#108905,#108906,#108907,
#108908,#108909,#108910,#108911,#108912),.UNSPECIFIED.,.F.,.F.,(4,3,3,3,
3,3,3,3,3,4),(5.23810621265401E-9,5.84794260519711E-6,8.49662041781891E-6,
1.21937803558104E-5,1.76033670136906E-5,1.93092034273021E-5,2.55871453406251E-5,
3.0315421636348E-5,3.68519660352467E-5,3.92146766969314E-5),
 .UNSPECIFIED.) ;
#211=B_SPLINE_CURVE_WITH_KNOTS('',3,(#108914,#108915,#108916,#108917,#108918,
#108919,#108920,#108921,#108922,#108923),.UNSPECIFIED.,.F.,.F.,(4,3,3,4),
(0.000144469795965455,0.000165397602015376,0.000173816468562374,0.000175865847906018),
 .UNSPECIFIED.) ;
#212=B_SPLINE_CURVE_WITH_KNOTS('',3,(#108941,#108942,#108943,#108944,#108945,
#108946,#108947),.UNSPECIFIED.,.F.,.F.,(4,3,4),(-2.05331166616594E-6,2.04386714314149E-5,
3.16299855932266E-5),.UNSPECIFIED.) ;
#213=B_SPLINE_CURVE_WITH_KNOTS('',3,(#108949,#108950,#108951,#108952,#108953,
#108954,#108955,#108956,#108957,#108958,#108959,#108960),.UNSPECIFIED.,
 .F.,.F.,(4,2,2,2,2,4),(9.00279528345874E-9,0.00183032786964776,0.00607746566718187,
0.0169681635075991,0.0216775196267783,0.0254454421566977),.UNSPECIFIED.) ;
#214=B_SPLINE_CURVE_WITH_KNOTS('',3,(#109119,#109120,#109121,#109122,#109123,
#109124,#109125,#109126,#109127,#109128,#109129,#109130,#109131,#109132,
#109133,#109134,#109135,#109136,#109137,#109138,#109139,#109140,#109141,
#109142,#109143,#109144,#109145,#109146,#109147,#109148,#109149,#109150,
#109151,#109152,#109153,#109154,#109155,#109156,#109157,#109158),
 .UNSPECIFIED.,.F.,.F.,(4,3,3,3,3,3,3,3,3,3,3,3,3,4),(0.,5.0717323028302E-5,
0.00010401741350107,0.00012450671916665,0.000125249568192411,0.000156566023859649,
0.000186760078749971,0.000187880030991799,0.000203537318084808,0.000211366035547462,
0.000217886758541633,0.000219194644848641,0.000234851354133266,0.000249013438333296),
 .UNSPECIFIED.) ;
#215=B_SPLINE_CURVE_WITH_KNOTS('',3,(#109164,#109165,#109166,#109167,#109168,
#109169,#109170,#109171,#109172,#109173,#109174,#109175,#109176,#109177,
#109178,#109179,#109180,#109181,#109182,#109183,#109184,#109185,#109186,
#109187,#109188,#109189,#109190,#109191,#109192,#109193,#109194,#109195,
#109196,#109197,#109198,#109199,#109200,#109201,#109202,#109203),
 .UNSPECIFIED.,.F.,.F.,(4,3,3,3,3,3,3,3,3,3,3,3,3,4),(0.,1.43115567092591E-5,
3.01335133960395E-5,3.14552036774756E-5,3.80447517297363E-5,4.59561222518582E-5,
6.17788922892867E-5,6.29104073549512E-5,9.34210966965043E-5,0.00012506639379551,
0.00012582081470991,0.000179837268177068,0.000231469985686737,0.00025164162941983),
 .UNSPECIFIED.) ;
#216=B_SPLINE_CURVE_WITH_KNOTS('',3,(#109208,#109209,#109210,#109211,#109212,
#109213,#109214),.UNSPECIFIED.,.F.,.F.,(4,3,4),(-2.04939766627128E-6,0.,
2.93835791072157E-5),.UNSPECIFIED.) ;
#217=B_SPLINE_CURVE_WITH_KNOTS('',3,(#109229,#109230,#109231,#109232,#109233,
#109234,#109235,#109236,#109237,#109238,#109239,#109240,#109241,#109242),
 .UNSPECIFIED.,.F.,.F.,(4,2,2,2,2,2,4),(1.44901763072086E-6,0.000561621523748031,
0.00112173034319911,0.00210338619150003,0.00384452539461507,0.00473112295159275,
0.00541108585601945),.UNSPECIFIED.) ;
#218=B_SPLINE_CURVE_WITH_KNOTS('',3,(#109251,#109252,#109253,#109254,#109255,
#109256,#109257,#109258,#109259,#109260,#109261,#109262,#109263,#109264,
#109265,#109266,#109267,#109268,#109269,#109270,#109271,#109272,#109273,
#109274,#109275,#109276,#109277,#109278,#109279,#109280,#109281,#109282,
#109283,#109284),.UNSPECIFIED.,.F.,.F.,(4,2,2,2,2,2,2,2,2,2,2,2,2,2,2,2,
4),(0.,1.67528894171495E-5,3.36326639089867E-5,3.5328500363345E-5,3.67766442982523E-5,
4.45936877501694E-5,5.25629171990832E-5,5.37833548715101E-5,5.51649664473801E-5,
7.22376444475638E-5,7.35532885965079E-5,0.00010924073629687,0.000146228640921011,
0.000147106577193012,0.000203359192943554,0.000258123601940488,0.00029421315438602),
 .UNSPECIFIED.) ;
#219=B_SPLINE_CURVE_WITH_KNOTS('',3,(#109288,#109289,#109290,#109291,#109292,
#109293,#109294,#109295,#109296,#109297,#109298,#109299,#109300,#109301,
#109302,#109303,#109304,#109305,#109306,#109307,#109308,#109309,#109310,
#109311,#109312,#109313,#109314,#109315,#109316,#109317,#109318,#109319,
#109320,#109321,#109322,#109323,#109324,#109325,#109326,#109327,#109328,
#109329,#109330,#109331,#109332,#109333,#109334,#109335,#109336,#109337,
#109338,#109339),.UNSPECIFIED.,.F.,.F.,(4,3,3,3,3,3,3,3,3,3,3,3,3,3,3,3,
3,4),(0.,5.28180786069338E-5,0.00010788843027313,0.000143209193858996,0.000144078242180727,
0.000180086811859628,0.000214813790788495,0.000215458170263561,0.000216102549738628,
0.000232714940020866,0.000234106492510818,0.000238605983992203,0.000240855729732896,
0.000243105475473589,0.000250616089253237,0.000252108710851791,0.000270124214172479,
0.000286418387717971),.UNSPECIFIED.) ;
#220=B_SPLINE_CURVE_WITH_KNOTS('',3,(#109484,#109485,#109486,#109487,#109488,
#109489,#109490,#109491),.UNSPECIFIED.,.F.,.F.,(4,2,2,4),(-0.0473604779370388,
-0.0461995546884437,-0.0447198409510955,-0.0410407833884838),
 .UNSPECIFIED.) ;
#221=B_SPLINE_CURVE_WITH_KNOTS('',3,(#109499,#109500,#109501,#109502,#109503,
#109504,#109505,#109506),.UNSPECIFIED.,.F.,.F.,(4,2,2,4),(-0.0536801724855779,
-0.0500011149229821,-0.048521401185634,-0.0473604779370388),
 .UNSPECIFIED.) ;
#222=B_SPLINE_CURVE_WITH_KNOTS('',3,(#109960,#109961,#109962,#109963,#109964,
#109965,#109966,#109967,#109968,#109969,#109970,#109971,#109972,#109973),
 .UNSPECIFIED.,.F.,.F.,(4,2,2,2,2,2,4),(4.71238898038469,4.88175806245107,
5.06763701998695,5.2433792296077,5.26451333207962,5.44874090582719,5.49822830854814),
 .UNSPECIFIED.) ;
#223=B_SPLINE_CURVE_WITH_KNOTS('',3,(#109978,#109979,#109980,#109981,#109982,
#109983,#109984,#109985,#109986,#109987,#109988,#109989,#109990,#109991),
 .UNSPECIFIED.,.F.,.F.,(4,2,2,2,2,2,4),(0.784956998631454,0.966941694311884,
1.1431172121161,1.16348181627568,1.34745079132797,1.51752882030577,1.5707963267949),
 .UNSPECIFIED.) ;
#224=B_SPLINE_CURVE_WITH_KNOTS('',3,(#109997,#109998,#109999,#110000,#110001,
#110002,#110003,#110004,#110005,#110006,#110007,#110008,#110009,#110010),
 .UNSPECIFIED.,.F.,.F.,(4,2,2,2,2,2,4),(0.78495699863135,0.966941694311801,
1.14311721212949,1.16348181627581,1.34745079132849,1.51752882030664,1.5707963267949),
 .UNSPECIFIED.) ;
#225=B_SPLINE_CURVE_WITH_KNOTS('',3,(#110012,#110013,#110014,#110015,#110016,
#110017,#110018,#110019,#110020,#110021,#110022,#110023,#110024,#110025),
 .UNSPECIFIED.,.F.,.F.,(4,2,2,2,2,2,4),(4.71238898038469,4.8817580624516,
5.06763701998866,5.24337922965485,5.26451333208181,5.44874090582897,5.49822830854826),
 .UNSPECIFIED.) ;
#226=B_SPLINE_CURVE_WITH_KNOTS('',3,(#110029,#110030,#110031,#110032,#110033,
#110034,#110035,#110036,#110037,#110038,#110039,#110040,#110041,#110042),
 .UNSPECIFIED.,.F.,.F.,(4,2,2,2,2,2,4),(4.71238898038469,4.88175806245179,
5.06763701998917,5.24337922965321,5.26451333208237,5.44874090582905,5.49822830854822),
 .UNSPECIFIED.) ;
#227=B_SPLINE_CURVE_WITH_KNOTS('',3,(#110046,#110047,#110048,#110049,#110050,
#110051,#110052,#110053,#110054,#110055,#110056,#110057,#110058,#110059),
 .UNSPECIFIED.,.F.,.F.,(4,2,2,2,2,2,4),(0.784956998631211,0.966941694311843,
1.14311721213428,1.16348181627569,1.3474507913286,1.51752882030718,1.5707963267949),
 .UNSPECIFIED.) ;
#228=B_SPLINE_CURVE_WITH_KNOTS('',3,(#110074,#110075,#110076,#110077,#110078,
#110079,#110080,#110081,#110082,#110083,#110084,#110085,#110086,#110087),
 .UNSPECIFIED.,.F.,.F.,(4,2,2,2,2,2,4),(0.784956998631298,0.966941694311769,
1.14311721211431,1.1634818162758,1.3474507913284,1.51752882030656,1.5707963267949),
 .UNSPECIFIED.) ;
#229=B_SPLINE_CURVE_WITH_KNOTS('',3,(#110091,#110092,#110093,#110094,#110095,
#110096,#110097,#110098,#110099,#110100,#110101,#110102,#110103,#110104),
 .UNSPECIFIED.,.F.,.F.,(4,2,2,2,2,2,4),(4.71238898038469,4.88175806245195,
5.06763701998927,5.24337922961088,5.26451333208257,5.44874090582964,5.49822830854831),
 .UNSPECIFIED.) ;
#230=B_SPLINE_CURVE_WITH_KNOTS('',3,(#110209,#110210,#110211,#110212,#110213,
#110214,#110215,#110216,#110217,#110218,#110219,#110220,#110221,#110222,
#110223,#110224),.UNSPECIFIED.,.F.,.F.,(4,3,3,3,3,4),(0.,3.26760986414938E-5,
6.60604127813367E-5,0.000101135724265729,0.00013823780033308,0.00016624299182732),
 .UNSPECIFIED.) ;
#231=B_SPLINE_CURVE_WITH_KNOTS('',3,(#110286,#110287,#110288,#110289,#110290,
#110291,#110292,#110293,#110294,#110295,#110296,#110297,#110298,#110299,
#110300,#110301),.UNSPECIFIED.,.F.,.F.,(4,3,3,3,3,4),(0.,1.86901632150156E-5,
5.38940239621536E-5,9.1325545181693E-5,0.00012977596605383,0.000168373497604197),
 .UNSPECIFIED.) ;
#232=B_SPLINE_CURVE_WITH_KNOTS('',3,(#110306,#110307,#110308,#110309,#110310,
#110311,#110312,#110313,#110314,#110315),.UNSPECIFIED.,.F.,.F.,(4,2,2,2,
4),(0.0288531015809221,0.0296205843578462,0.0328031056819848,0.0376042554623528,
0.0407130021448623),.UNSPECIFIED.) ;
#233=B_SPLINE_CURVE_WITH_KNOTS('',3,(#110320,#110321,#110322,#110323,#110324,
#110325),.UNSPECIFIED.,.F.,.F.,(4,2,4),(0.0637474840407795,0.0675088661482764,
0.0720284409638635),.UNSPECIFIED.) ;
#234=B_SPLINE_CURVE_WITH_KNOTS('',3,(#110331,#110332,#110333,#110334,#110335,
#110336,#110337,#110338,#110339,#110340),.UNSPECIFIED.,.F.,.F.,(4,2,2,2,
4),(0.0767275662269652,0.0771734766335448,0.0818220866869972,0.0868722195372896,
0.0892832637365362),.UNSPECIFIED.) ;
#235=B_SPLINE_CURVE_WITH_KNOTS('',3,(#110375,#110376,#110377,#110378,#110379,
#110380),.UNSPECIFIED.,.F.,.F.,(4,2,4),(0.171679973605596,0.178707475948804,
0.186889989700405),.UNSPECIFIED.) ;
#236=B_SPLINE_CURVE_WITH_KNOTS('',3,(#110420,#110421,#110422,#110423,#110424,
#110425,#110426,#110427,#110428,#110429,#110430,#110431,#110432,#110433,
#110434,#110435,#110436,#110437,#110438,#110439,#110440,#110441,#110442,
#110443,#110444,#110445,#110446,#110447,#110448,#110449),.UNSPECIFIED.,
 .F.,.F.,(4,2,2,2,2,2,2,2,2,2,2,2,2,2,4),(2.36970964942748,2.55498029688329,
2.73514427898821,2.74569929646429,2.92071305420847,2.93943382978577,3.11857096685307,
3.13197658032462,3.25399179664507,3.45054278261492,3.62794535799599,3.64606212534882,
3.82474099482791,3.83698255062549,3.91347421315166),.UNSPECIFIED.) ;
#237=B_SPLINE_CURVE_WITH_KNOTS('',3,(#110460,#110461,#110462,#110463,#110464,
#110465,#110466,#110467,#110468,#110469,#110470,#110471,#110472,#110473,
#110474,#110475,#110476,#110477,#110478,#110479,#110480,#110481,#110482,
#110483,#110484,#110485),.UNSPECIFIED.,.F.,.F.,(4,2,2,2,2,2,2,2,2,2,2,2,
4),(2.70344464880683,2.89144352771223,3.06851986340401,3.08081089074483,
3.26996664970738,3.35940092938476,3.54587543017967,3.72254345722124,3.73903833379381,
3.9157002469173,3.93052100184786,4.11735511986238,4.22222897897867),
 .UNSPECIFIED.) ;
#238=B_SPLINE_CURVE_WITH_KNOTS('',3,(#110643,#110644,#110645,#110646,#110647,
#110648,#110649,#110650,#110651,#110652,#110653,#110654,#110655,#110656,
#110657,#110658,#110659,#110660,#110661),.UNSPECIFIED.,.F.,.F.,(4,3,3,3,
3,3,4),(2.81004151507315E-8,3.99307614181576E-5,8.00540716903477E-5,0.000126830846822483,
0.000175618195186418,0.000215193140472276,0.00024522089875673),
 .UNSPECIFIED.) ;
#239=B_SPLINE_CURVE_WITH_KNOTS('',3,(#110684,#110685,#110686,#110687,#110688,
#110689,#110690,#110691,#110692,#110693,#110694,#110695,#110696,#110697,
#110698,#110699,#110700,#110701,#110702,#110703,#110704,#110705,#110706,
#110707,#110708,#110709,#110710,#110711,#110712,#110713,#110714,#110715,
#110716,#110717,#110718,#110719,#110720,#110721,#110722,#110723,#110724,
#110725,#110726,#110727,#110728,#110729,#110730,#110731,#110732,#110733,
#110734,#110735,#110736,#110737,#110738,#110739,#110740,#110741,#110742,
#110743,#110744,#110745,#110746,#110747,#110748,#110749,#110750,#110751,
#110752,#110753,#110754,#110755,#110756,#110757,#110758,#110759,#110760,
#110761,#110762),.UNSPECIFIED.,.F.,.F.,(4,3,3,3,3,3,3,3,3,3,3,3,3,3,3,3,
3,3,3,3,3,3,3,3,3,3,4),(0.000152038190190988,0.000154892841408446,0.000155160464960082,
0.000160456565729206,0.000163456795060818,0.0001665800922469,0.000167751328691681,
0.000168007536663977,0.000168255738137138,0.000169267315291294,0.000175949983805147,
0.000178959298271426,0.000180334649023592,0.000187987241670261,0.000191981216408588,
0.000193065528939054,0.000193839174265159,0.000198143816207847,0.000212206269476804,
0.000226582370019588,0.000228143757087808,0.000228729277238391,0.000232827918292468,
0.000249109432820284,0.000250176797440916,0.000265881325831968,0.000267525676589363),
 .UNSPECIFIED.) ;
#240=B_SPLINE_CURVE_WITH_KNOTS('',3,(#110764,#110765,#110766,#110767,#110768,
#110769,#110770,#110771,#110772,#110773),.UNSPECIFIED.,.F.,.F.,(4,3,3,4),
(0.00013063174123083,0.000139067346351189,0.000143554831048705,0.00015203818937155),
 .UNSPECIFIED.) ;
#241=B_SPLINE_CURVE_WITH_KNOTS('',3,(#110775,#110776,#110777,#110778,#110779,
#110780,#110781,#110782,#110783,#110784,#110785,#110786,#110787,#110788,
#110789,#110790,#110791,#110792,#110793),.UNSPECIFIED.,.F.,.F.,(4,3,3,3,
3,3,4),(0.000104137230128263,0.000110259474166881,0.000116844366893684,
0.000120664217590594,0.000125429508057303,0.000130430624030584,0.000130630877723054),
 .UNSPECIFIED.) ;
#242=B_SPLINE_CURVE_WITH_KNOTS('',3,(#110794,#110795,#110796,#110797,#110798,
#110799,#110800,#110801,#110802,#110803,#110804,#110805,#110806,#110807,
#110808,#110809,#110810,#110811,#110812,#110813,#110814,#110815,#110816,
#110817,#110818,#110819,#110820,#110821,#110822,#110823,#110824,#110825,
#110826,#110827,#110828,#110829,#110830,#110831,#110832,#110833,#110834,
#110835,#110836),.UNSPECIFIED.,.F.,.F.,(4,3,3,3,3,3,3,3,3,3,3,3,3,3,4),
(0.,4.78421531964037E-6,1.59977421339088E-5,1.75965265776683E-5,2.63603667652888E-5,
3.75047088100213E-5,4.29655082836385E-5,5.3450780665107E-5,6.17416442233874E-5,
6.39360530465754E-5,7.32944438965348E-5,8.49065978095124E-5,9.46209320470023E-5,
9.66050857869651E-5,0.00010413722946728),.UNSPECIFIED.) ;
#243=B_SPLINE_CURVE_WITH_KNOTS('',3,(#110906,#110907,#110908,#110909,#110910,
#110911,#110912,#110913,#110914,#110915,#110916,#110917,#110918,#110919,
#110920,#110921,#110922,#110923,#110924,#110925,#110926,#110927,#110928,
#110929,#110930,#110931,#110932,#110933,#110934,#110935,#110936,#110937,
#110938,#110939),.UNSPECIFIED.,.F.,.F.,(4,3,3,3,3,3,3,3,3,3,3,4),(0.000173579735006458,
0.000179152672590563,0.00018712219621297,0.000190349677855919,0.000201571576238784,
0.000207505544696865,0.00020908215834011,0.000218112358783792,0.000219837174422847,
0.000228512621317669,0.00024080293533235,0.000245138123631364),
 .UNSPECIFIED.) ;
#244=B_SPLINE_CURVE_WITH_KNOTS('',3,(#111001,#111002,#111003,#111004,#111005,
#111006,#111007,#111008,#111009,#111010,#111011,#111012,#111013,#111014,
#111015,#111016),.UNSPECIFIED.,.F.,.F.,(4,3,3,3,3,4),(0.000149826268238874,
0.000156541783273878,0.000187447062839771,0.000218157419331147,0.0002512535901195,
0.000263630362845938),.UNSPECIFIED.) ;
#245=B_SPLINE_CURVE_WITH_KNOTS('',3,(#111018,#111019,#111020,#111021),
 .UNSPECIFIED.,.F.,.F.,(4,4),(0.00012894552500308,0.000149826268238874),
 .UNSPECIFIED.) ;
#246=B_SPLINE_CURVE_WITH_KNOTS('',3,(#111022,#111023,#111024,#111025,#111026,
#111027,#111028,#111029,#111030,#111031,#111032,#111033,#111034,#111035,
#111036,#111037),.UNSPECIFIED.,.F.,.F.,(4,3,3,3,3,4),(0.000107977862661226,
0.000113849696954328,0.00011675864089999,0.000123355930725867,0.000128649321338313,
0.00012894552500308),.UNSPECIFIED.) ;
#247=B_SPLINE_CURVE_WITH_KNOTS('',3,(#111247,#111248,#111249,#111250,#111251,
#111252,#111253,#111254,#111255,#111256),.UNSPECIFIED.,.F.,.F.,(4,3,3,4),
(3.97263228028543E-15,3.94729529730244E-5,7.90727202189635E-5,0.00010300346369627),
 .UNSPECIFIED.) ;
#248=B_SPLINE_CURVE_WITH_KNOTS('',3,(#111263,#111264,#111265,#111266,#111267,
#111268,#111269),.UNSPECIFIED.,.F.,.F.,(4,3,4),(0.00015822335750707,0.000179871364136697,
0.000191820073778123),.UNSPECIFIED.) ;
#249=B_SPLINE_CURVE_WITH_KNOTS('',3,(#111284,#111285,#111286,#111287,#111288,
#111289,#111290,#111291,#111292,#111293,#111294,#111295,#111296,#111297,
#111298,#111299),.UNSPECIFIED.,.F.,.F.,(4,3,3,3,3,4),(2.25414513468041E-8,
3.71181381094367E-5,7.40234349159894E-5,0.000126639028433412,0.000171180683285944,
0.000173579731706482),.UNSPECIFIED.) ;
#250=B_SPLINE_CURVE_WITH_KNOTS('',3,(#111355,#111356,#111357,#111358,#111359,
#111360),.UNSPECIFIED.,.F.,.F.,(4,2,4),(0.,0.000162685424844483,0.000325370849688965),
 .UNSPECIFIED.) ;
#251=B_SPLINE_CURVE_WITH_KNOTS('',3,(#111363,#111364,#111365,#111366,#111367,
#111368),.UNSPECIFIED.,.F.,.F.,(4,2,4),(0.,0.000163438694679257,0.000326877389358514),
 .UNSPECIFIED.) ;
#252=B_SPLINE_CURVE_WITH_KNOTS('',3,(#111379,#111380,#111381,#111382,#111383,
#111384),.UNSPECIFIED.,.F.,.F.,(4,2,4),(-0.00501427184001352,-0.00354643693242498,
0.),.UNSPECIFIED.) ;
#253=B_SPLINE_CURVE_WITH_KNOTS('',3,(#111397,#111398,#111399,#111400,#111401,
#111402,#111403,#111404,#111405,#111406,#111407,#111408,#111409,#111410,
#111411,#111412,#111413,#111414,#111415,#111416,#111417,#111418,#111419,
#111420,#111421,#111422,#111423,#111424),.UNSPECIFIED.,.F.,.F.,(4,3,3,3,
3,3,3,3,3,4),(5.2381062116969E-9,5.84794260526809E-6,8.49662041781891E-6,
1.21937803558058E-5,1.7603367013667E-5,1.93092034273021E-5,2.55871453405969E-5,
3.0315421636348E-5,3.68519660351865E-5,3.92146766969307E-5),
 .UNSPECIFIED.) ;
#254=B_SPLINE_CURVE_WITH_KNOTS('',3,(#111426,#111427,#111428,#111429,#111430,
#111431,#111432,#111433,#111434,#111435),.UNSPECIFIED.,.F.,.F.,(4,3,3,4),
(0.000144469795965455,0.000165397602015043,0.000173816468562374,0.000175865847906018),
 .UNSPECIFIED.) ;
#255=B_SPLINE_CURVE_WITH_KNOTS('',3,(#111453,#111454,#111455,#111456,#111457,
#111458,#111459),.UNSPECIFIED.,.F.,.F.,(4,3,4),(-2.05331166616455E-6,2.04386714311757E-5,
3.16299855932218E-5),.UNSPECIFIED.) ;
#256=B_SPLINE_CURVE_WITH_KNOTS('',3,(#111461,#111462,#111463,#111464,#111465,
#111466,#111467,#111468,#111469,#111470,#111471,#111472),.UNSPECIFIED.,
 .F.,.F.,(4,2,2,2,2,4),(9.00279523814192E-9,0.00183032786984177,0.0060774656662359,
0.0169681634717373,0.0216775195756215,0.0254454420933995),.UNSPECIFIED.) ;
#257=B_SPLINE_CURVE_WITH_KNOTS('',3,(#111631,#111632,#111633,#111634,#111635,
#111636,#111637,#111638,#111639,#111640,#111641,#111642,#111643,#111644,
#111645,#111646,#111647,#111648,#111649,#111650,#111651,#111652,#111653,
#111654,#111655,#111656,#111657,#111658,#111659,#111660,#111661,#111662,
#111663,#111664,#111665,#111666,#111667,#111668,#111669,#111670),
 .UNSPECIFIED.,.F.,.F.,(4,3,3,3,3,3,3,3,3,3,3,3,3,4),(0.,5.0717323028292E-5,
0.000104017413501046,0.00012450671916665,0.00012524956819241,0.000156566023859647,
0.000186760078749971,0.000187880030991795,0.000203537318084806,0.00021136603554746,
0.000217886758541633,0.00021919464484864,0.000234851354133265,0.000249013438333296),
 .UNSPECIFIED.) ;
#258=B_SPLINE_CURVE_WITH_KNOTS('',3,(#111676,#111677,#111678,#111679,#111680,
#111681,#111682,#111683,#111684,#111685,#111686,#111687,#111688,#111689,
#111690,#111691,#111692,#111693,#111694,#111695,#111696,#111697,#111698,
#111699,#111700,#111701,#111702,#111703,#111704,#111705,#111706,#111707,
#111708,#111709,#111710,#111711,#111712,#111713,#111714,#111715),
 .UNSPECIFIED.,.F.,.F.,(4,3,3,3,3,3,3,3,3,3,3,3,3,4),(0.,1.43115567092639E-5,
3.01335133960425E-5,3.14552036774813E-5,3.80447517297347E-5,4.59561222518525E-5,
6.17788922892923E-5,6.29104073549626E-5,9.34210966965285E-5,0.000125066393795525,
0.000125820814709921,0.000179837268182647,0.000231469985696588,0.000251641629419827),
 .UNSPECIFIED.) ;
#259=B_SPLINE_CURVE_WITH_KNOTS('',3,(#111720,#111721,#111722,#111723,#111724,
#111725,#111726),.UNSPECIFIED.,.F.,.F.,(4,3,4),(-2.04939766627003E-6,0.,
2.93835791072157E-5),.UNSPECIFIED.) ;
#260=B_SPLINE_CURVE_WITH_KNOTS('',3,(#111741,#111742,#111743,#111744,#111745,
#111746,#111747,#111748,#111749,#111750,#111751,#111752,#111753,#111754),
 .UNSPECIFIED.,.F.,.F.,(4,2,2,2,2,2,4),(1.44901763004144E-6,0.000561621523804037,
0.00112173034329354,0.00210338619163598,0.00384452539442495,0.00473112295062459,
0.00541108585437911),.UNSPECIFIED.) ;
#261=B_SPLINE_CURVE_WITH_KNOTS('',3,(#111763,#111764,#111765,#111766,#111767,
#111768,#111769,#111770,#111771,#111772,#111773,#111774,#111775,#111776,
#111777,#111778,#111779,#111780,#111781,#111782,#111783,#111784,#111785,
#111786,#111787,#111788,#111789,#111790,#111791,#111792,#111793,#111794,
#111795,#111796),.UNSPECIFIED.,.F.,.F.,(4,2,2,2,2,2,2,2,2,2,2,2,2,2,2,2,
4),(0.,1.67528894171673E-5,3.36326639087995E-5,3.53285003633486E-5,3.67766442982523E-5,
4.45936877501694E-5,5.25629171991637E-5,5.37833548715111E-5,5.51649664473801E-5,
7.22376444475639E-5,7.35532885965079E-5,0.000109240736296815,0.000146228640920945,
0.000147106577193012,0.000203359192945594,0.000258123601943362,0.00029421315438602),
 .UNSPECIFIED.) ;
#262=B_SPLINE_CURVE_WITH_KNOTS('',3,(#111800,#111801,#111802,#111803,#111804,
#111805,#111806,#111807,#111808,#111809,#111810,#111811,#111812,#111813,
#111814,#111815,#111816,#111817,#111818,#111819,#111820,#111821,#111822,
#111823,#111824,#111825,#111826,#111827,#111828,#111829,#111830,#111831,
#111832,#111833,#111834,#111835,#111836,#111837,#111838,#111839,#111840,
#111841,#111842,#111843,#111844,#111845,#111846,#111847,#111848,#111849,
#111850,#111851),.UNSPECIFIED.,.F.,.F.,(4,3,3,3,3,3,3,3,3,3,3,3,3,3,3,3,
3,4),(0.,5.28180786157377E-5,0.000107888430292485,0.000143209193859038,
0.000144078242180733,0.000180086811859676,0.000214813790788553,0.000215458170263625,
0.000216102549738696,0.000232714940020933,0.000234106492510888,0.000238605983992275,
0.000240855729732968,0.000243105475473661,0.000250616089253313,0.000252108710851866,
0.000270124214172563,0.000286418387718064),.UNSPECIFIED.) ;
#263=B_SPLINE_CURVE_WITH_KNOTS('',3,(#111996,#111997,#111998,#111999,#112000,
#112001,#112002,#112003),.UNSPECIFIED.,.F.,.F.,(4,2,2,4),(-0.0473604779370388,
-0.0461995546884436,-0.0447198409510952,-0.0410407833884837),
 .UNSPECIFIED.) ;
#264=B_SPLINE_CURVE_WITH_KNOTS('',3,(#112011,#112012,#112013,#112014,#112015,
#112016,#112017,#112018),.UNSPECIFIED.,.F.,.F.,(4,2,2,4),(-0.0536801724855783,
-0.0500011149229823,-0.0485214011856339,-0.0473604779370388),
 .UNSPECIFIED.) ;
#265=B_SPLINE_CURVE_WITH_KNOTS('',3,(#112472,#112473,#112474,#112475,#112476,
#112477,#112478,#112479,#112480,#112481,#112482,#112483,#112484,#112485),
 .UNSPECIFIED.,.F.,.F.,(4,2,2,2,2,2,4),(4.71238898038469,4.88175806245101,
5.06763701998682,5.24337922961327,5.2645133320796,5.44874090582723,5.49822830854813),
 .UNSPECIFIED.) ;
#266=B_SPLINE_CURVE_WITH_KNOTS('',3,(#112490,#112491,#112492,#112493,#112494,
#112495,#112496,#112497,#112498,#112499,#112500,#112501,#112502,#112503),
 .UNSPECIFIED.,.F.,.F.,(4,2,2,2,2,2,4),(0.78495699863145,0.966941694311798,
1.1431172121153,1.16348181627562,1.34745079132799,1.51752882030591,1.5707963267949),
 .UNSPECIFIED.) ;
#267=B_SPLINE_CURVE_WITH_KNOTS('',3,(#112509,#112510,#112511,#112512,#112513,
#112514,#112515,#112516,#112517,#112518,#112519,#112520,#112521,#112522),
 .UNSPECIFIED.,.F.,.F.,(4,2,2,2,2,2,4),(0.784956998631343,0.966941694311655,
1.14311721212998,1.16348181627563,1.34745079132838,1.51752882030652,1.5707963267949),
 .UNSPECIFIED.) ;
#268=B_SPLINE_CURVE_WITH_KNOTS('',3,(#112524,#112525,#112526,#112527,#112528,
#112529,#112530,#112531,#112532,#112533,#112534,#112535,#112536,#112537),
 .UNSPECIFIED.,.F.,.F.,(4,2,2,2,2,2,4),(4.71238898038469,4.88175806245179,
5.06763701998934,5.2433792296541,5.26451333208252,5.44874090582906,5.49822830854823),
 .UNSPECIFIED.) ;
#269=B_SPLINE_CURVE_WITH_KNOTS('',3,(#112541,#112542,#112543,#112544,#112545,
#112546,#112547,#112548,#112549,#112550,#112551,#112552,#112553,#112554),
 .UNSPECIFIED.,.F.,.F.,(4,2,2,2,2,2,4),(4.71238898038469,4.88175806245174,
5.06763701998914,5.24337922964868,5.26451333208227,5.44874090582901,5.49822830854825),
 .UNSPECIFIED.) ;
#270=B_SPLINE_CURVE_WITH_KNOTS('',3,(#112558,#112559,#112560,#112561,#112562,
#112563,#112564,#112565,#112566,#112567,#112568,#112569,#112570,#112571),
 .UNSPECIFIED.,.F.,.F.,(4,2,2,2,2,2,4),(0.784956998631379,0.966941694311961,
1.14311721212408,1.1634818162759,1.34745079132852,1.5175288203065,1.5707963267949),
 .UNSPECIFIED.) ;
#271=B_SPLINE_CURVE_WITH_KNOTS('',3,(#112586,#112587,#112588,#112589,#112590,
#112591,#112592,#112593,#112594,#112595,#112596,#112597,#112598,#112599),
 .UNSPECIFIED.,.F.,.F.,(4,2,2,2,2,2,4),(0.784956998631469,0.966941694312593,
1.14311721209935,1.16348181627602,1.34745079132695,1.51752882030426,1.5707963267949),
 .UNSPECIFIED.) ;
#272=B_SPLINE_CURVE_WITH_KNOTS('',3,(#112603,#112604,#112605,#112606,#112607,
#112608,#112609,#112610,#112611,#112612,#112613,#112614,#112615,#112616),
 .UNSPECIFIED.,.F.,.F.,(4,2,2,2,2,2,4),(4.71238898038469,4.88175806245153,
5.06763701998872,5.24337922961216,5.2645133320817,5.44874090582829,5.49822830854814),
 .UNSPECIFIED.) ;
#273=B_SPLINE_CURVE_WITH_KNOTS('',3,(#112721,#112722,#112723,#112724,#112725,
#112726,#112727,#112728,#112729,#112730,#112731,#112732,#112733,#112734,
#112735,#112736),.UNSPECIFIED.,.F.,.F.,(4,3,3,3,3,4),(0.,3.26760986414938E-5,
6.60604127813367E-5,0.000101135724265729,0.00013823780033308,0.00016624299182732),
 .UNSPECIFIED.) ;
#274=B_SPLINE_CURVE_WITH_KNOTS('',3,(#112798,#112799,#112800,#112801,#112802,
#112803,#112804,#112805,#112806,#112807,#112808,#112809,#112810,#112811,
#112812,#112813),.UNSPECIFIED.,.F.,.F.,(4,3,3,3,3,4),(0.,1.86901632150156E-5,
5.38940239621527E-5,9.13255451816914E-5,0.000129775966053829,0.000168373497604197),
 .UNSPECIFIED.) ;
#275=B_SPLINE_CURVE_WITH_KNOTS('',3,(#112818,#112819,#112820,#112821,#112822,
#112823,#112824,#112825,#112826,#112827),.UNSPECIFIED.,.F.,.F.,(4,2,2,2,
4),(0.0288531015839766,0.0296205843610201,0.032803105685514,0.0376042554662768,
0.0407130021489537),.UNSPECIFIED.) ;
#276=B_SPLINE_CURVE_WITH_KNOTS('',3,(#112832,#112833,#112834,#112835,#112836,
#112837),.UNSPECIFIED.,.F.,.F.,(4,2,4),(0.0637474840140125,0.0675088661184123,
0.0720284409301188),.UNSPECIFIED.) ;
#277=B_SPLINE_CURVE_WITH_KNOTS('',3,(#112843,#112844,#112845,#112846,#112847,
#112848,#112849,#112850,#112851,#112852),.UNSPECIFIED.,.F.,.F.,(4,2,2,2,
4),(0.0767275662203977,0.0771734766269397,0.0818220866796455,0.0868722195290685,
0.0892832637278774),.UNSPECIFIED.) ;
#278=B_SPLINE_CURVE_WITH_KNOTS('',3,(#112887,#112888,#112889,#112890,#112891,
#112892),.UNSPECIFIED.,.F.,.F.,(4,2,4),(0.171679973607292,0.178707475950603,
0.186889989702311),.UNSPECIFIED.) ;
#279=B_SPLINE_CURVE_WITH_KNOTS('',3,(#112932,#112933,#112934,#112935,#112936,
#112937,#112938,#112939,#112940,#112941,#112942,#112943,#112944,#112945,
#112946,#112947,#112948,#112949,#112950,#112951,#112952,#112953,#112954,
#112955,#112956,#112957,#112958,#112959,#112960,#112961),.UNSPECIFIED.,
 .F.,.F.,(4,2,2,2,2,2,2,2,2,2,2,2,2,2,4),(2.36970964942748,2.55498029688324,
2.73514427898934,2.74569929646418,2.92071305420845,2.93943382978562,3.11857096684871,
3.13197658032441,3.25399179664502,3.4505427826148,3.6279453579965,3.64606212534862,
3.82474099481916,3.83698255062526,3.91347421315172),.UNSPECIFIED.) ;
#280=B_SPLINE_CURVE_WITH_KNOTS('',3,(#112972,#112973,#112974,#112975,#112976,
#112977,#112978,#112979,#112980,#112981,#112982,#112983,#112984,#112985,
#112986,#112987,#112988,#112989,#112990,#112991,#112992,#112993,#112994,
#112995,#112996,#112997),.UNSPECIFIED.,.F.,.F.,(4,2,2,2,2,2,2,2,2,2,2,2,
4),(2.70344464881048,2.89144352771225,3.06851986339127,3.08081089074493,
3.2699666497075,3.35940092938474,3.54587543017978,3.72254345722052,3.73903833379394,
3.91570024691754,3.93052100184793,4.11735511986242,4.22222897897867),
 .UNSPECIFIED.) ;
#281=B_SPLINE_CURVE_WITH_KNOTS('',3,(#113155,#113156,#113157,#113158,#113159,
#113160,#113161,#113162,#113163,#113164,#113165,#113166,#113167,#113168,
#113169,#113170,#113171,#113172,#113173),.UNSPECIFIED.,.F.,.F.,(4,3,3,3,
3,3,4),(2.8100415148163E-8,3.99307614181576E-5,8.00540716903477E-5,0.000126830846822483,
0.000175618195186418,0.000215193140472276,0.00024522089875673),
 .UNSPECIFIED.) ;
#282=B_SPLINE_CURVE_WITH_KNOTS('',3,(#113196,#113197,#113198,#113199,#113200,
#113201,#113202,#113203,#113204,#113205,#113206,#113207,#113208,#113209,
#113210,#113211,#113212,#113213,#113214,#113215,#113216,#113217,#113218,
#113219,#113220,#113221,#113222,#113223,#113224,#113225,#113226,#113227,
#113228,#113229,#113230,#113231,#113232,#113233,#113234,#113235,#113236,
#113237,#113238,#113239,#113240,#113241,#113242,#113243,#113244,#113245,
#113246,#113247,#113248,#113249,#113250,#113251,#113252,#113253,#113254,
#113255,#113256,#113257,#113258,#113259,#113260,#113261,#113262,#113263,
#113264,#113265,#113266,#113267,#113268,#113269,#113270,#113271,#113272,
#113273,#113274),.UNSPECIFIED.,.F.,.F.,(4,3,3,3,3,3,3,3,3,3,3,3,3,3,3,3,
3,3,3,3,3,3,3,3,3,3,4),(0.000152038190190979,0.000154892841408439,0.000155160464960076,
0.00016045656572911,0.000163456795060818,0.000166580092246901,0.000167751328691683,
0.000168007536663979,0.00016825573813714,0.0001692673152913,0.000175949983805152,
0.000178959298271428,0.000180334649023594,0.000187987241670257,0.000191981216408588,
0.000193065528939052,0.000193839174265157,0.000198143816207847,0.000212206269476822,
0.000226582370019626,0.000228143757087837,0.000228729277238415,0.000232827918292468,
0.000249109432822923,0.000250176797440916,0.000265881325831446,0.000267525676589363),
 .UNSPECIFIED.) ;
#283=B_SPLINE_CURVE_WITH_KNOTS('',3,(#113276,#113277,#113278,#113279,#113280,
#113281,#113282,#113283,#113284,#113285),.UNSPECIFIED.,.F.,.F.,(4,3,3,4),
(0.000130631741230824,0.000139067346351537,0.000143554831048706,0.000152038189371535),
 .UNSPECIFIED.) ;
#284=B_SPLINE_CURVE_WITH_KNOTS('',3,(#113287,#113288,#113289,#113290,#113291,
#113292,#113293,#113294,#113295,#113296,#113297,#113298,#113299,#113300,
#113301,#113302,#113303,#113304,#113305),.UNSPECIFIED.,.F.,.F.,(4,3,3,3,
3,3,4),(0.000104137230128253,0.00011025947416687,0.000116844366893704,0.000120664217590573,
0.000125429508057303,0.00013043062403061,0.000130630877723054),
 .UNSPECIFIED.) ;
#285=B_SPLINE_CURVE_WITH_KNOTS('',3,(#113306,#113307,#113308,#113309,#113310,
#113311,#113312,#113313,#113314,#113315,#113316,#113317,#113318,#113319,
#113320,#113321,#113322,#113323,#113324,#113325,#113326,#113327,#113328,
#113329,#113330,#113331,#113332,#113333,#113334,#113335,#113336,#113337,
#113338,#113339,#113340,#113341,#113342,#113343,#113344,#113345,#113346,
#113347,#113348),.UNSPECIFIED.,.F.,.F.,(4,3,3,3,3,3,3,3,3,3,3,3,3,3,4),
(0.,4.78421531964037E-6,1.5997742133367E-5,1.75965265776407E-5,2.63603667654138E-5,
3.75047088105756E-5,4.29655082836385E-5,5.3450780665107E-5,6.17416442233547E-5,
6.39360530465754E-5,7.32944438965254E-5,8.49065978095124E-5,9.4620932046832E-5,
9.6605085786969E-5,0.000104137229467266),.UNSPECIFIED.) ;
#286=B_SPLINE_CURVE_WITH_KNOTS('',3,(#113418,#113419,#113420,#113421,#113422,
#113423,#113424,#113425,#113426,#113427,#113428,#113429,#113430,#113431,
#113432,#113433,#113434,#113435,#113436,#113437,#113438,#113439,#113440,
#113441,#113442,#113443,#113444,#113445,#113446,#113447,#113448,#113449,
#113450,#113451),.UNSPECIFIED.,.F.,.F.,(4,3,3,3,3,3,3,3,3,3,3,4),(0.00017357973500646,
0.000179152672590516,0.000187122196212348,0.000190349677855926,0.00020157157623905,
0.000207505544696952,0.000209082158340111,0.000218112358784159,0.00021983717442272,
0.000228512621317903,0.000240802935335257,0.000245138123631368),
 .UNSPECIFIED.) ;
#287=B_SPLINE_CURVE_WITH_KNOTS('',3,(#113513,#113514,#113515,#113516,#113517,
#113518,#113519,#113520,#113521,#113522,#113523,#113524,#113525,#113526,
#113527,#113528),.UNSPECIFIED.,.F.,.F.,(4,3,3,3,3,4),(0.00014982626823866,
0.000156541783273877,0.000187447062839769,0.000218157419331144,0.000251253590119498,
0.000263630362845952),.UNSPECIFIED.) ;
#288=B_SPLINE_CURVE_WITH_KNOTS('',3,(#113530,#113531,#113532,#113533),
 .UNSPECIFIED.,.F.,.F.,(4,4),(0.000128945525002973,0.00014982626823866),
 .UNSPECIFIED.) ;
#289=B_SPLINE_CURVE_WITH_KNOTS('',3,(#113534,#113535,#113536,#113537,#113538,
#113539,#113540,#113541,#113542,#113543,#113544,#113545,#113546,#113547,
#113548,#113549),.UNSPECIFIED.,.F.,.F.,(4,3,3,3,3,4),(0.000107977862661223,
0.000113849696953733,0.000116758640899989,0.000123355930725824,0.000128649321338145,
0.000128945525002973),.UNSPECIFIED.) ;
#377=(
BOUNDED_SURFACE()
B_SPLINE_SURFACE(3,2,((#101185,#101186,#101187),(#101188,#101189,#101190),
(#101191,#101192,#101193),(#101194,#101195,#101196)),.UNSPECIFIED.,.F.,
 .F.,.F.)
B_SPLINE_SURFACE_WITH_KNOTS((4,4),(3,3),(-8.88178419700125E-16,1.00173611575494),
(0.800638603120404,1.),.UNSPECIFIED.)
GEOMETRIC_REPRESENTATION_ITEM()
RATIONAL_B_SPLINE_SURFACE(((0.931056261594764,0.956944532691445,1.),(0.931106613485821,
0.956975977522396,1.),(0.926966069646249,0.954390201728277,1.),(0.920044734228405,
0.950067817452233,1.)))
REPRESENTATION_ITEM('')
SURFACE()
) ;
#378=(
BOUNDED_SURFACE()
B_SPLINE_SURFACE(3,2,((#101222,#101223,#101224),(#101225,#101226,#101227),
(#101228,#101229,#101230),(#101231,#101232,#101233)),.UNSPECIFIED.,.F.,
 .F.,.F.)
B_SPLINE_SURFACE_WITH_KNOTS((4,4),(3,3),(1.8295911660693E-15,1.08063632538888),
(0.,1.),.UNSPECIFIED.)
GEOMETRIC_REPRESENTATION_ITEM()
RATIONAL_B_SPLINE_SURFACE(((1.,0.821344978643199,1.),(1.,0.821618737292292,
1.),(1.,0.799663084581839,1.),(1.,0.763019982472727,1.)))
REPRESENTATION_ITEM('')
SURFACE()
) ;
#379=(
BOUNDED_SURFACE()
B_SPLINE_SURFACE(3,2,((#102700,#102701,#102702),(#102703,#102704,#102705),
(#102706,#102707,#102708),(#102709,#102710,#102711),(#102712,#102713,#102714),
(#102715,#102716,#102717)),.UNSPECIFIED.,.F.,.F.,.F.)
B_SPLINE_SURFACE_WITH_KNOTS((4,2,4),(3,3),(9.07204043127161E-5,0.000289236237441534,
0.000487752070570359),(-0.000844756555527479,1.00064307855265),
 .UNSPECIFIED.)
GEOMETRIC_REPRESENTATION_ITEM()
RATIONAL_B_SPLINE_SURFACE(((1.0006785336953,0.598126578821808,1.00051643581316),
(1.00070177595156,0.584360946986066,1.00053412562517),(1.00066498743049,
0.606149590529446,1.00050612567481),(1.00056632625581,0.664583392836326,
1.00043103409964),(1.00050548323107,0.700618735924288,1.0003847261312),
(1.00047271456519,0.720026550084155,1.00035978571524)))
REPRESENTATION_ITEM('')
SURFACE()
) ;
#380=(
BOUNDED_SURFACE()
B_SPLINE_SURFACE(3,2,((#102732,#102733,#102734),(#102735,#102736,#102737),
(#102738,#102739,#102740),(#102741,#102742,#102743),(#102744,#102745,#102746),
(#102747,#102748,#102749)),.UNSPECIFIED.,.F.,.F.,.F.)
B_SPLINE_SURFACE_WITH_KNOTS((4,2,4),(3,3),(0.000107162911540598,0.000298022515767418,
0.000488882119994237),(-0.000759939855646165,1.00062534339576),
 .UNSPECIFIED.)
GEOMETRIC_REPRESENTATION_ITEM()
RATIONAL_B_SPLINE_SURFACE(((1.000428625731,0.717810580914592,1.00035266240945),
(1.00045905072597,0.697780025035142,1.00037769532571),(1.00051114946329,
0.663480375353458,1.00042056084894),(1.00059665225219,0.607188882365371,
1.00049091038087),(1.00062840114513,0.586286726926422,1.0005170325669),
(1.00061268510755,0.596633514797481,1.00050410180871)))
REPRESENTATION_ITEM('')
SURFACE()
) ;
#381=(
BOUNDED_SURFACE()
B_SPLINE_SURFACE(3,2,((#102979,#102980,#102981),(#102982,#102983,#102984),
(#102985,#102986,#102987),(#102988,#102989,#102990),(#102991,#102992,#102993),
(#102994,#102995,#102996),(#102997,#102998,#102999),(#103000,#103001,#103002)),
 .UNSPECIFIED.,.F.,.F.,.F.)
B_SPLINE_SURFACE_WITH_KNOTS((4,2,2,4),(3,3),(6.28318530717959,6.67588438887831,
7.06858347057703,7.85398163397448),(0.,1.),.UNSPECIFIED.)
GEOMETRIC_REPRESENTATION_ITEM()
RATIONAL_B_SPLINE_SURFACE(((1.,0.707106781186548,1.),(1.,0.706675310150437,
1.),(1.,0.726552333979981,1.),(1.,0.787677905717223,1.),(1.,0.828238301901761,
1.),(1.,0.941599607549792,1.),(1.,1.00267605951746,1.),(1.,1.,1.)))
REPRESENTATION_ITEM('')
SURFACE()
) ;
#382=(
BOUNDED_SURFACE()
B_SPLINE_SURFACE(3,2,((#103010,#103011,#103012),(#103013,#103014,#103015),
(#103016,#103017,#103018),(#103019,#103020,#103021),(#103022,#103023,#103024),
(#103025,#103026,#103027),(#103028,#103029,#103030),(#103031,#103032,#103033)),
 .UNSPECIFIED.,.F.,.F.,.F.)
B_SPLINE_SURFACE_WITH_KNOTS((4,2,2,4),(3,3),(4.71238898038469,5.49778714378214,
5.89048622548086,6.28318530717959),(0.,1.),.UNSPECIFIED.)
GEOMETRIC_REPRESENTATION_ITEM()
RATIONAL_B_SPLINE_SURFACE(((1.,1.,1.),(1.,1.00267605951745,1.),(1.,0.941599607549811,
1.),(1.,0.828238301901754,1.),(1.,0.787677905717215,1.),(1.,0.72655233397999,
1.),(1.,0.706675310150431,1.),(1.,0.707106781186547,1.)))
REPRESENTATION_ITEM('')
SURFACE()
) ;
#383=(
BOUNDED_SURFACE()
B_SPLINE_SURFACE(3,2,((#103034,#103035,#103036),(#103037,#103038,#103039),
(#103040,#103041,#103042),(#103043,#103044,#103045),(#103046,#103047,#103048),
(#103049,#103050,#103051),(#103052,#103053,#103054),(#103055,#103056,#103057)),
 .UNSPECIFIED.,.F.,.F.,.F.)
B_SPLINE_SURFACE_WITH_KNOTS((4,2,2,4),(3,3),(4.71238898038469,5.49778714378214,
5.89048622548086,6.28318530717959),(0.,1.),.UNSPECIFIED.)
GEOMETRIC_REPRESENTATION_ITEM()
RATIONAL_B_SPLINE_SURFACE(((1.,1.,1.),(1.,1.00267605951745,1.),(1.,0.941599607549811,
1.),(1.,0.828238301901754,1.),(1.,0.787677905717212,1.),(1.,0.726552333979993,
1.),(1.,0.706675310150429,1.),(1.,0.707106781186548,1.)))
REPRESENTATION_ITEM('')
SURFACE()
) ;
#384=(
BOUNDED_SURFACE()
B_SPLINE_SURFACE(3,2,((#103065,#103066,#103067),(#103068,#103069,#103070),
(#103071,#103072,#103073),(#103074,#103075,#103076),(#103077,#103078,#103079),
(#103080,#103081,#103082),(#103083,#103084,#103085),(#103086,#103087,#103088)),
 .UNSPECIFIED.,.F.,.F.,.F.)
B_SPLINE_SURFACE_WITH_KNOTS((4,2,2,4),(3,3),(6.28318530717959,6.67588438887831,
7.06858347057703,7.85398163397448),(0.,1.),.UNSPECIFIED.)
GEOMETRIC_REPRESENTATION_ITEM()
RATIONAL_B_SPLINE_SURFACE(((1.,0.707106781186548,1.),(1.,0.70667531015044,
1.),(1.,0.726552333979978,1.),(1.,0.787677905717225,1.),(1.,0.828238301901761,
1.),(1.,0.941599607549792,1.),(1.,1.00267605951746,1.),(1.,1.,1.)))
REPRESENTATION_ITEM('')
SURFACE()
) ;
#385=(
BOUNDED_SURFACE()
B_SPLINE_SURFACE(3,2,((#103089,#103090,#103091),(#103092,#103093,#103094),
(#103095,#103096,#103097),(#103098,#103099,#103100),(#103101,#103102,#103103),
(#103104,#103105,#103106)),.UNSPECIFIED.,.F.,.F.,.F.)
B_SPLINE_SURFACE_WITH_KNOTS((4,2,4),(3,3),(2.06095632820092,2.9281173096476,
3.79527829109429),(0.,1.),.UNSPECIFIED.)
GEOMETRIC_REPRESENTATION_ITEM()
RATIONAL_B_SPLINE_SURFACE(((1.,0.763019982472727,1.),(1.,0.792403856906193,
1.),(1.,0.812400188579439,1.),(1.,0.825457041220947,1.),(1.,0.818529518851321,
1.),(1.,0.799131938862213,1.)))
REPRESENTATION_ITEM('')
SURFACE()
) ;
#386=(
BOUNDED_SURFACE()
B_SPLINE_SURFACE(3,2,((#103129,#103130,#103131),(#103132,#103133,#103134),
(#103135,#103136,#103137),(#103138,#103139,#103140),(#103141,#103142,#103143),
(#103144,#103145,#103146)),.UNSPECIFIED.,.F.,.F.,.F.)
B_SPLINE_SURFACE_WITH_KNOTS((4,2,4),(3,3),(2.13522523980987,3.02435044878099,
3.9134756577521),(0.,1.),.UNSPECIFIED.)
GEOMETRIC_REPRESENTATION_ITEM()
RATIONAL_B_SPLINE_SURFACE(((1.,0.749240327740277,1.),(1.,0.768579562596357,
1.),(1.,0.780993049743008,1.),(1.,0.78606840104594,1.),(1.,0.778729916329032,
1.),(1.,0.763019982472727,1.)))
REPRESENTATION_ITEM('')
SURFACE()
) ;
#387=(
BOUNDED_SURFACE()
B_SPLINE_SURFACE(3,2,((#103303,#103304,#103305),(#103306,#103307,#103308),
(#103309,#103310,#103311),(#103312,#103313,#103314),(#103315,#103316,#103317),
(#103318,#103319,#103320),(#103321,#103322,#103323),(#103324,#103325,#103326),
(#103327,#103328,#103329),(#103330,#103331,#103332),(#103333,#103334,#103335),
(#103336,#103337,#103338),(#103339,#103340,#103341),(#103342,#103343,#103344),
(#103345,#103346,#103347),(#103348,#103349,#103350),(#103351,#103352,#103353),
(#103354,#103355,#103356)),.UNSPECIFIED.,.F.,.F.,.F.)
B_SPLINE_SURFACE_WITH_KNOTS((4,2,2,2,2,2,2,2,4),(3,3),(-2.88136898045006E-5,
0.000144068449022501,0.000180085561278126,0.000216102673533752,0.000234111229661564,
0.000243115507725471,0.000252119785789377,0.00027012834191719,0.000315232069289129),
(-0.00230043332376221,1.00649231299482),.UNSPECIFIED.)
GEOMETRIC_REPRESENTATION_ITEM()
RATIONAL_B_SPLINE_SURFACE(((1.00137797387137,0.698547958833496,1.00390520040674),
(1.00130996746141,0.713425360736485,1.00371246913268),(1.0013392130407,
0.707027460342999,1.00379535158098),(1.00112343332548,0.754232445100877,
1.00318382835174),(1.00107694244916,0.76440300773299,1.00305207245063),
(1.00092854904644,0.796866246024035,1.00263152312912),(1.00083723042777,
0.816843536281347,1.00237272467569),(1.0005249519753,0.885159038384459,
1.00148772245255),(1.0003623858312,0.920722772198159,1.00102700735102),
(1.00013066612431,0.97141486445937,1.00037030992561),(1.00008161134638,
0.982146318257361,1.00023128788558),(1.00010185218186,0.977718337948078,
1.00028865074315),(1.00015066464696,0.967039893643917,1.00042698606469),
(1.00027150756266,0.94060372939002,1.00076945685705),(1.00035349548867,
0.922667665317858,1.00100181197542),(1.00060974665136,0.866608956479207,
1.0017280319463),(1.00075148156369,0.8356023608425,1.00212971099755),(1.00085165739564,
0.813687424976079,1.00241361093774)))
REPRESENTATION_ITEM('')
SURFACE()
) ;
#388=(
BOUNDED_SURFACE()
B_SPLINE_SURFACE(3,2,((#103358,#103359,#103360),(#103361,#103362,#103363),
(#103364,#103365,#103366),(#103367,#103368,#103369)),.UNSPECIFIED.,.F.,
 .F.,.F.)
B_SPLINE_SURFACE_WITH_KNOTS((4,4),(3,3),(5.63598348762742,6.28318530717959),
(0.792338840560963,1.),.UNSPECIFIED.)
GEOMETRIC_REPRESENTATION_ITEM()
RATIONAL_B_SPLINE_SURFACE(((0.934040253948343,0.958376553896462,1.),(0.938725627259265,
0.961333226642434,1.),(0.941220250254381,0.962907441402214,1.),(0.941208919370365,
0.962900291125441,1.)))
REPRESENTATION_ITEM('')
SURFACE()
) ;
#389=(
BOUNDED_SURFACE()
B_SPLINE_SURFACE(3,2,((#103410,#103411,#103412),(#103413,#103414,#103415),
(#103416,#103417,#103418),(#103419,#103420,#103421),(#103422,#103423,#103424),
(#103425,#103426,#103427),(#103428,#103429,#103430),(#103431,#103432,#103433),
(#103434,#103435,#103436),(#103437,#103438,#103439),(#103440,#103441,#103442),
(#103443,#103444,#103445),(#103446,#103447,#103448),(#103449,#103450,#103451),
(#103452,#103453,#103454),(#103455,#103456,#103457),(#103458,#103459,#103460),
(#103461,#103462,#103463)),.UNSPECIFIED.,.F.,.F.,.F.)
B_SPLINE_SURFACE_WITH_KNOTS((4,2,2,2,2,2,2,2,4),(3,3),(-3.19743590576754E-5,
0.000144068449022546,0.000180085561278183,0.000216102673533819,0.000234111229661638,
0.000243115507725547,0.000252119785789456,0.000270128341917274,0.000288136898045092),
(-0.00668341897260021,1.00019683226132),.UNSPECIFIED.)
GEOMETRIC_REPRESENTATION_ITEM()
RATIONAL_B_SPLINE_SURFACE(((1.00403209003396,0.698291475893957,1.00011798325541),
(1.00381915098312,0.714225030505444,1.00011175243164),(1.00391733895236,
0.706877935813784,1.00011462551636),(1.00327816898458,0.754704999695385,
1.0000959227213),(1.00314250899891,0.764856006670135,1.00009195316541),
(1.00270949829923,0.797256825605574,1.00007928281045),(1.00244303133882,
0.817195704120572,1.00007148570295),(1.0015318054439,0.885379851192721,
1.00004482226126),(1.0010574388042,0.920875204110099,1.00003094178738),
(1.00038128265054,0.971469827113991,1.00001115673707),(1.00023814122158,
0.98218064678933,1.00000696826617),(1.00029720380908,0.97776118046934,1.00000869650048),
(1.00043963817124,0.967103268362387,1.00001286428185),(1.0007922567818,
0.940717934784036,1.00002318227853),(1.00103149685957,0.922816357646008,
1.00003018269841),(1.00145821870303,0.890886113898632,1.00004266903473),
(1.00165232267982,0.87636192821199,1.00004834872414),(1.00182713963607,
0.863280929173223,1.00005346405476)))
REPRESENTATION_ITEM('')
SURFACE()
) ;
#390=(
BOUNDED_SURFACE()
B_SPLINE_SURFACE(3,2,((#103502,#103503,#103504),(#103505,#103506,#103507),
(#103508,#103509,#103510),(#103511,#103512,#103513)),.UNSPECIFIED.,.F.,
 .F.,.F.)
B_SPLINE_SURFACE_WITH_KNOTS((4,4),(3,3),(5.51130230301728,6.28318530717959),
(0.,1.),.UNSPECIFIED.)
GEOMETRIC_REPRESENTATION_ITEM()
RATIONAL_B_SPLINE_SURFACE(((1.,0.763019982472727,1.),(1.,0.776565014072566,
1.),(1.,0.78408875836913,1.),(1.,0.784033077704815,1.)))
REPRESENTATION_ITEM('')
SURFACE()
) ;
#391=(
BOUNDED_SURFACE()
B_SPLINE_SURFACE(3,2,((#103518,#103519,#103520),(#103521,#103522,#103523),
(#103524,#103525,#103526),(#103527,#103528,#103529)),.UNSPECIFIED.,.F.,
 .F.,.F.)
B_SPLINE_SURFACE_WITH_KNOTS((4,4),(3,3),(0.0051446850272488,0.00657473287039649),
(0.,1.),.UNSPECIFIED.)
GEOMETRIC_REPRESENTATION_ITEM()
RATIONAL_B_SPLINE_SURFACE(((1.,0.943476662524758,1.),(1.,0.944945702024752,
1.),(1.,0.946300916277096,1.),(1.,0.947565352018496,1.)))
REPRESENTATION_ITEM('')
SURFACE()
) ;
#392=(
BOUNDED_SURFACE()
B_SPLINE_SURFACE(3,2,((#103568,#103569,#103570),(#103571,#103572,#103573),
(#103574,#103575,#103576),(#103577,#103578,#103579)),.UNSPECIFIED.,.F.,
 .F.,.F.)
B_SPLINE_SURFACE_WITH_KNOTS((4,4),(3,3),(0.0051446850272488,0.00657473287039648),
(0.,1.),.UNSPECIFIED.)
GEOMETRIC_REPRESENTATION_ITEM()
RATIONAL_B_SPLINE_SURFACE(((1.,0.943476662524758,1.),(1.,0.944945702024752,
1.),(1.,0.946300916277096,1.),(1.,0.947565352018496,1.)))
REPRESENTATION_ITEM('')
SURFACE()
) ;
#393=(
BOUNDED_SURFACE()
B_SPLINE_SURFACE(3,2,((#103584,#103585,#103586),(#103587,#103588,#103589),
(#103590,#103591,#103592),(#103593,#103594,#103595),(#103596,#103597,#103598),
(#103599,#103600,#103601),(#103602,#103603,#103604),(#103605,#103606,#103607),
(#103608,#103609,#103610),(#103611,#103612,#103613),(#103614,#103615,#103616),
(#103617,#103618,#103619),(#103620,#103621,#103622),(#103623,#103624,#103625),
(#103626,#103627,#103628),(#103629,#103630,#103631),(#103632,#103633,#103634),
(#103635,#103636,#103637)),.UNSPECIFIED.,.F.,.F.,.F.)
B_SPLINE_SURFACE_WITH_KNOTS((4,2,2,2,2,2,2,2,4),(3,3),(-2.77591379149742E-5,
0.000125253167969377,0.000156566459961721,0.000187879751954065,0.000203536397950237,
0.000211364720948323,0.000219193043946409,0.000234849689942581,0.000250506335938753),
(0.,1.00287807885248),.UNSPECIFIED.)
GEOMETRIC_REPRESENTATION_ITEM()
RATIONAL_B_SPLINE_SURFACE(((1.,0.698587265144072,1.00173497923611),(1.,
0.713937574732587,1.0016466204333),(1.,0.719549163949171,1.00161431924079),
(1.,0.771808112009009,1.00131350849427),(1.,0.782482243723509,1.00125206650876),
(1.,0.810804881627976,1.00108903693836),(1.,0.827824808964379,1.00099106755248),
(1.,0.868687526094284,1.00075585530843),(1.,0.885097717150239,1.00066139566074),
(1.,0.918597380148661,1.00046856631746),(1.,0.931968622959475,1.00039159933513),
(1.,0.95574199467466,1.00025475605836),(1.,0.963776461019218,1.00020850840301),
(1.,0.96542172890934,1.00019903798156),(1.,0.949947468785993,1.0002881102632),
(1.,0.927474619202833,1.00041746752948),(1.,0.916335140210118,1.00048158812731),
(1.,0.906010523700252,1.00054101824819)))
REPRESENTATION_ITEM('')
SURFACE()
) ;
#394=(
BOUNDED_SURFACE()
B_SPLINE_SURFACE(3,2,((#103641,#103642,#103643),(#103644,#103645,#103646),
(#103647,#103648,#103649),(#103650,#103651,#103652),(#103653,#103654,#103655),
(#103656,#103657,#103658),(#103659,#103660,#103661),(#103662,#103663,#103664),
(#103665,#103666,#103667),(#103668,#103669,#103670),(#103671,#103672,#103673),
(#103674,#103675,#103676),(#103677,#103678,#103679),(#103680,#103681,#103682),
(#103683,#103684,#103685),(#103686,#103687,#103688),(#103689,#103690,#103691),
(#103692,#103693,#103694)),.UNSPECIFIED.,.F.,.F.,.F.)
B_SPLINE_SURFACE_WITH_KNOTS((4,2,2,2,2,2,2,2,4),(3,3),(-2.79610875103897E-5,
0.000125253167969368,0.00015656645996171,0.000187879751954052,0.000203536397950223,
0.000211364720948308,0.000219193043946394,0.000234849689942565,0.000253195388096685),
(-0.00314610977262661,1.),.UNSPECIFIED.)
GEOMETRIC_REPRESENTATION_ITEM()
RATIONAL_B_SPLINE_SURFACE(((1.00189744483735,0.698445862592737,1.),(1.00180054146108,
0.713846370407001,1.),(1.0017654902188,0.719416939270283,1.),(1.001436217201,
0.771747125052562,1.),(1.00136903527044,0.782424109553829,1.),(1.00119077538533,
0.810754317015262,1.),(1.00108365364399,0.82777879312693,1.),(1.00082646773902,
0.868652431296543,1.),(1.0007231836176,0.885067008168521,1.),(1.00051234004796,
0.918575624344433,1.),(1.00042818276659,0.931950440776527,1.),(1.00027855551348,
0.955730166204014,1.),(1.00022798737599,0.963766779853875,1.),(1.00021763222242,
0.965412487461153,1.),(1.00031502568701,0.949934091660457,1.),(1.00046861400988,
0.92552484754986,1.),(1.00055064362451,0.912488173602249,1.),(1.00062456604608,
0.900739946914071,0.999999999999999)))
REPRESENTATION_ITEM('')
SURFACE()
) ;
#395=(
BOUNDED_SURFACE()
B_SPLINE_SURFACE(3,2,((#103697,#103698,#103699),(#103700,#103701,#103702),
(#103703,#103704,#103705),(#103706,#103707,#103708)),.UNSPECIFIED.,.F.,
 .F.,.F.)
B_SPLINE_SURFACE_WITH_KNOTS((4,4),(3,3),(-1.77635683940025E-15,1.00173611575493),
(0.800638603120394,1.),.UNSPECIFIED.)
GEOMETRIC_REPRESENTATION_ITEM()
RATIONAL_B_SPLINE_SURFACE(((0.931056261594762,0.956944532691443,1.),(0.931106613485818,
0.956975977522394,1.),(0.926966069646246,0.954390201728275,1.),(0.920044734228402,
0.95006781745223,1.)))
REPRESENTATION_ITEM('')
SURFACE()
) ;
#396=(
BOUNDED_SURFACE()
B_SPLINE_SURFACE(3,2,((#103734,#103735,#103736),(#103737,#103738,#103739),
(#103740,#103741,#103742),(#103743,#103744,#103745)),.UNSPECIFIED.,.F.,
 .F.,.F.)
B_SPLINE_SURFACE_WITH_KNOTS((4,4),(3,3),(3.32036915323687E-15,1.08063632538888),
(0.,1.),.UNSPECIFIED.)
GEOMETRIC_REPRESENTATION_ITEM()
RATIONAL_B_SPLINE_SURFACE(((1.,0.821344978643199,1.),(1.,0.821618737292291,
1.),(1.,0.79966308458184,1.),(1.,0.763019982472727,1.)))
REPRESENTATION_ITEM('')
SURFACE()
) ;
#397=(
BOUNDED_SURFACE()
B_SPLINE_SURFACE(3,2,((#105212,#105213,#105214),(#105215,#105216,#105217),
(#105218,#105219,#105220),(#105221,#105222,#105223),(#105224,#105225,#105226),
(#105227,#105228,#105229)),.UNSPECIFIED.,.F.,.F.,.F.)
B_SPLINE_SURFACE_WITH_KNOTS((4,2,4),(3,3),(9.07204043127111E-5,0.000289236237441535,
0.000487752070570357),(-0.000844756555506173,1.00064307855256),
 .UNSPECIFIED.)
GEOMETRIC_REPRESENTATION_ITEM()
RATIONAL_B_SPLINE_SURFACE(((1.00067853369529,0.598126578821862,1.00051643581309),
(1.00070177595154,0.5843609469861,1.00053412562509),(1.00066498743048,0.606149590529492,
1.00050612567475),(1.0005663262558,0.664583392836358,1.00043103409958),
(1.00050548323105,0.700618735924326,1.00038472613115),(1.00047271456518,
0.720026550084179,1.00035978571519)))
REPRESENTATION_ITEM('')
SURFACE()
) ;
#398=(
BOUNDED_SURFACE()
B_SPLINE_SURFACE(3,2,((#105244,#105245,#105246),(#105247,#105248,#105249),
(#105250,#105251,#105252),(#105253,#105254,#105255),(#105256,#105257,#105258),
(#105259,#105260,#105261)),.UNSPECIFIED.,.F.,.F.,.F.)
B_SPLINE_SURFACE_WITH_KNOTS((4,2,4),(3,3),(0.000107162911540596,0.000298022515767417,
0.000488882119994237),(-0.00075993985561925,1.00062534339583),
 .UNSPECIFIED.)
GEOMETRIC_REPRESENTATION_ITEM()
RATIONAL_B_SPLINE_SURFACE(((1.00042862573099,0.717810580914598,1.00035266240949),
(1.00045905072595,0.697780025035093,1.00037769532575),(1.00051114946327,
0.663480375353471,1.00042056084899),(1.00059665225217,0.607188882365325,
1.00049091038093),(1.0006284011451,0.586286726926441,1.00051703256696),
(1.00061268510753,0.596633514797444,1.00050410180877)))
REPRESENTATION_ITEM('')
SURFACE()
) ;
#399=(
BOUNDED_SURFACE()
B_SPLINE_SURFACE(3,2,((#105491,#105492,#105493),(#105494,#105495,#105496),
(#105497,#105498,#105499),(#105500,#105501,#105502),(#105503,#105504,#105505),
(#105506,#105507,#105508),(#105509,#105510,#105511),(#105512,#105513,#105514)),
 .UNSPECIFIED.,.F.,.F.,.F.)
B_SPLINE_SURFACE_WITH_KNOTS((4,2,2,4),(3,3),(6.28318530717959,6.67588438887831,
7.06858347057703,7.85398163397448),(0.,1.),.UNSPECIFIED.)
GEOMETRIC_REPRESENTATION_ITEM()
RATIONAL_B_SPLINE_SURFACE(((1.,0.707106781186548,1.),(1.,0.706675310150414,
1.),(1.,0.726552333980012,1.),(1.,0.787677905717191,1.),(1.,0.828238301901766,
1.),(1.,0.941599607549786,1.),(1.,1.00267605951747,1.),(1.,1.,1.)))
REPRESENTATION_ITEM('')
SURFACE()
) ;
#400=(
BOUNDED_SURFACE()
B_SPLINE_SURFACE(3,2,((#105522,#105523,#105524),(#105525,#105526,#105527),
(#105528,#105529,#105530),(#105531,#105532,#105533),(#105534,#105535,#105536),
(#105537,#105538,#105539),(#105540,#105541,#105542),(#105543,#105544,#105545)),
 .UNSPECIFIED.,.F.,.F.,.F.)
B_SPLINE_SURFACE_WITH_KNOTS((4,2,2,4),(3,3),(4.71238898038469,5.49778714378214,
5.89048622548086,6.28318530717959),(0.,1.),.UNSPECIFIED.)
GEOMETRIC_REPRESENTATION_ITEM()
RATIONAL_B_SPLINE_SURFACE(((1.,1.,1.),(1.,1.00267605951742,1.),(1.,0.941599607549841,
1.),(1.,0.82823830190174,1.),(1.,0.787677905717214,1.),(1.,0.726552333979992,
1.),(1.,0.706675310150431,1.),(1.,0.707106781186548,1.)))
REPRESENTATION_ITEM('')
SURFACE()
) ;
#401=(
BOUNDED_SURFACE()
B_SPLINE_SURFACE(3,2,((#105546,#105547,#105548),(#105549,#105550,#105551),
(#105552,#105553,#105554),(#105555,#105556,#105557),(#105558,#105559,#105560),
(#105561,#105562,#105563),(#105564,#105565,#105566),(#105567,#105568,#105569)),
 .UNSPECIFIED.,.F.,.F.,.F.)
B_SPLINE_SURFACE_WITH_KNOTS((4,2,2,4),(3,3),(4.71238898038469,5.49778714378214,
5.89048622548086,6.28318530717959),(0.,1.),.UNSPECIFIED.)
GEOMETRIC_REPRESENTATION_ITEM()
RATIONAL_B_SPLINE_SURFACE(((1.,1.,1.),(1.,1.00267605951742,1.),(1.,0.94159960754984,
1.),(1.,0.828238301901739,1.),(1.,0.787677905717214,1.),(1.,0.726552333979992,
1.),(1.,0.70667531015043,1.),(1.,0.707106781186548,1.)))
REPRESENTATION_ITEM('')
SURFACE()
) ;
#402=(
BOUNDED_SURFACE()
B_SPLINE_SURFACE(3,2,((#105577,#105578,#105579),(#105580,#105581,#105582),
(#105583,#105584,#105585),(#105586,#105587,#105588),(#105589,#105590,#105591),
(#105592,#105593,#105594),(#105595,#105596,#105597),(#105598,#105599,#105600)),
 .UNSPECIFIED.,.F.,.F.,.F.)
B_SPLINE_SURFACE_WITH_KNOTS((4,2,2,4),(3,3),(6.28318530717959,6.67588438887831,
7.06858347057703,7.85398163397448),(0.,1.),.UNSPECIFIED.)
GEOMETRIC_REPRESENTATION_ITEM()
RATIONAL_B_SPLINE_SURFACE(((1.,0.707106781186548,1.),(1.,0.706675310150437,
1.),(1.,0.726552333979981,1.),(1.,0.787677905717222,1.),(1.,0.828238301901765,
1.),(1.,0.941599607549785,1.),(1.,1.00267605951747,1.),(1.,1.,1.)))
REPRESENTATION_ITEM('')
SURFACE()
) ;
#403=(
BOUNDED_SURFACE()
B_SPLINE_SURFACE(3,2,((#105601,#105602,#105603),(#105604,#105605,#105606),
(#105607,#105608,#105609),(#105610,#105611,#105612),(#105613,#105614,#105615),
(#105616,#105617,#105618)),.UNSPECIFIED.,.F.,.F.,.F.)
B_SPLINE_SURFACE_WITH_KNOTS((4,2,4),(3,3),(2.06095632820092,2.9281173096476,
3.79527829109429),(0.,1.),.UNSPECIFIED.)
GEOMETRIC_REPRESENTATION_ITEM()
RATIONAL_B_SPLINE_SURFACE(((1.,0.763019982472727,1.),(1.,0.792403856906172,
1.),(1.,0.812400188579468,1.),(1.,0.825457041220918,1.),(1.,0.818529518851342,
1.),(1.,0.799131938862213,1.)))
REPRESENTATION_ITEM('')
SURFACE()
) ;
#404=(
BOUNDED_SURFACE()
B_SPLINE_SURFACE(3,2,((#105641,#105642,#105643),(#105644,#105645,#105646),
(#105647,#105648,#105649),(#105650,#105651,#105652),(#105653,#105654,#105655),
(#105656,#105657,#105658)),.UNSPECIFIED.,.F.,.F.,.F.)
B_SPLINE_SURFACE_WITH_KNOTS((4,2,4),(3,3),(2.13522523980988,3.02435044878099,
3.9134756577521),(0.,1.),.UNSPECIFIED.)
GEOMETRIC_REPRESENTATION_ITEM()
RATIONAL_B_SPLINE_SURFACE(((1.,0.749240327740277,1.),(1.,0.76857956259632,
1.),(1.,0.780993049743057,1.),(1.,0.786068401045891,1.),(1.,0.778729916329069,
1.),(1.,0.763019982472727,1.)))
REPRESENTATION_ITEM('')
SURFACE()
) ;
#405=(
BOUNDED_SURFACE()
B_SPLINE_SURFACE(3,2,((#105815,#105816,#105817),(#105818,#105819,#105820),
(#105821,#105822,#105823),(#105824,#105825,#105826),(#105827,#105828,#105829),
(#105830,#105831,#105832),(#105833,#105834,#105835),(#105836,#105837,#105838),
(#105839,#105840,#105841),(#105842,#105843,#105844),(#105845,#105846,#105847),
(#105848,#105849,#105850),(#105851,#105852,#105853),(#105854,#105855,#105856),
(#105857,#105858,#105859),(#105860,#105861,#105862),(#105863,#105864,#105865),
(#105866,#105867,#105868)),.UNSPECIFIED.,.F.,.F.,.F.)
B_SPLINE_SURFACE_WITH_KNOTS((4,2,2,2,2,2,2,2,4),(3,3),(-2.88136898044879E-5,
0.000144068449022439,0.000180085561278049,0.000216102673533659,0.000234111229661463,
0.000243115507725366,0.000252119785789268,0.000270128341917073,0.000315232069288994),
(-0.00230043332309208,1.00649231299495),.UNSPECIFIED.)
GEOMETRIC_REPRESENTATION_ITEM()
RATIONAL_B_SPLINE_SURFACE(((1.00137797387097,0.698547958833687,1.00390520040681),
(1.00130996746102,0.71342536073659,1.00371246913275),(1.00133921304031,
0.707027460343199,1.00379535158106),(1.00112343332516,0.754232445100949,
1.0031838283518),(1.00107694244884,0.764403007733067,1.00305207245068),
(1.00092854904617,0.796866246023982,1.00263152312917),(1.00083723042752,
0.81684353628167,1.00237272467573),(1.00052495197515,0.885159038383876,
1.00148772245259),(1.0003623858311,0.920722772198335,1.00102700735104),
(1.00013066612427,0.971414864458886,1.00037030992563),(1.00008161134636,
0.98214631825728,1.00023128788558),(1.00010185218183,0.977718337948346,
1.00028865074315),(1.00015066464691,0.967039893644153,1.00042698606469),
(1.00027150756258,0.940603729390226,1.00076945685706),(1.00035349548857,
0.922667665318029,1.00100181197544),(1.00060974665118,0.866608956479267,
1.00172803194633),(1.00075148156347,0.835602360842649,1.00212971099759),
(1.0008516573954,0.813687424975539,1.0024136109378)))
REPRESENTATION_ITEM('')
SURFACE()
) ;
#406=(
BOUNDED_SURFACE()
B_SPLINE_SURFACE(3,2,((#105870,#105871,#105872),(#105873,#105874,#105875),
(#105876,#105877,#105878),(#105879,#105880,#105881)),.UNSPECIFIED.,.F.,
 .F.,.F.)
B_SPLINE_SURFACE_WITH_KNOTS((4,4),(3,3),(5.63598348762742,6.28318530717959),
(0.792338840560958,1.),.UNSPECIFIED.)
GEOMETRIC_REPRESENTATION_ITEM()
RATIONAL_B_SPLINE_SURFACE(((0.934040253948341,0.958376553896461,1.),(0.938725627259263,
0.961333226642432,1.),(0.94122025025438,0.962907441402213,1.),(0.941208919370364,
0.96290029112544,1.)))
REPRESENTATION_ITEM('')
SURFACE()
) ;
#407=(
BOUNDED_SURFACE()
B_SPLINE_SURFACE(3,2,((#105922,#105923,#105924),(#105925,#105926,#105927),
(#105928,#105929,#105930),(#105931,#105932,#105933),(#105934,#105935,#105936),
(#105937,#105938,#105939),(#105940,#105941,#105942),(#105943,#105944,#105945),
(#105946,#105947,#105948),(#105949,#105950,#105951),(#105952,#105953,#105954),
(#105955,#105956,#105957),(#105958,#105959,#105960),(#105961,#105962,#105963),
(#105964,#105965,#105966),(#105967,#105968,#105969),(#105970,#105971,#105972),
(#105973,#105974,#105975)),.UNSPECIFIED.,.F.,.F.,.F.)
B_SPLINE_SURFACE_WITH_KNOTS((4,2,2,2,2,2,2,2,4),(3,3),(-3.19743590576624E-5,
0.000144068449022547,0.000180085561278184,0.000216102673533821,0.000234111229661639,
0.000243115507725548,0.000252119785789458,0.000270128341917276,0.000288136898045094),
(-0.0066834189723838,1.00019683226129),.UNSPECIFIED.)
GEOMETRIC_REPRESENTATION_ITEM()
RATIONAL_B_SPLINE_SURFACE(((1.00403209003383,0.698291475894096,1.00011798325539),
(1.003819150983,0.714225030505405,1.00011175243162),(1.00391733895223,0.706877935813939,
1.00011462551634),(1.00327816898448,0.75470499969543,1.00009592272129),
(1.00314250899881,0.764856006670175,1.0000919531654),(1.00270949829915,
0.797256825605654,1.00007928281044),(1.00244303133874,0.817195704120573,
1.00007148570294),(1.00153180544385,0.885379851192701,1.00004482226125),
(1.00105743880416,0.920875204110361,1.00003094178737),(1.00038128265052,
0.971469827114154,1.00001115673707),(1.00023814122157,0.982180646789333,
1.00000696826617),(1.00029720380907,0.977761180469344,1.00000869650048),
(1.00043963817123,0.967103268362389,1.00001286428185),(1.00079225678177,
0.940717934784047,1.00002318227853),(1.00103149685954,0.922816357646006,
1.0000301826984),(1.00145821870299,0.890886113898669,1.00004266903472),
(1.00165232267976,0.876361928212014,1.00004834872413),(1.00182713963601,
0.863280929173256,1.00005346405475)))
REPRESENTATION_ITEM('')
SURFACE()
) ;
#408=(
BOUNDED_SURFACE()
B_SPLINE_SURFACE(3,2,((#106014,#106015,#106016),(#106017,#106018,#106019),
(#106020,#106021,#106022),(#106023,#106024,#106025)),.UNSPECIFIED.,.F.,
 .F.,.F.)
B_SPLINE_SURFACE_WITH_KNOTS((4,4),(3,3),(5.51130230301728,6.28318530717958),
(0.,1.),.UNSPECIFIED.)
GEOMETRIC_REPRESENTATION_ITEM()
RATIONAL_B_SPLINE_SURFACE(((1.,0.763019982472727,1.),(1.,0.776565014072565,
1.),(1.,0.784088758369132,1.),(1.,0.784033077704815,1.)))
REPRESENTATION_ITEM('')
SURFACE()
) ;
#409=(
BOUNDED_SURFACE()
B_SPLINE_SURFACE(3,2,((#106030,#106031,#106032),(#106033,#106034,#106035),
(#106036,#106037,#106038),(#106039,#106040,#106041)),.UNSPECIFIED.,.F.,
 .F.,.F.)
B_SPLINE_SURFACE_WITH_KNOTS((4,4),(3,3),(0.0051446850272488,0.00657473287039649),
(0.,1.),.UNSPECIFIED.)
GEOMETRIC_REPRESENTATION_ITEM()
RATIONAL_B_SPLINE_SURFACE(((1.,0.943476662524758,1.),(1.,0.944945702024752,
1.),(1.,0.946300916277095,1.),(1.,0.947565352018496,1.)))
REPRESENTATION_ITEM('')
SURFACE()
) ;
#410=(
BOUNDED_SURFACE()
B_SPLINE_SURFACE(3,2,((#106080,#106081,#106082),(#106083,#106084,#106085),
(#106086,#106087,#106088),(#106089,#106090,#106091)),.UNSPECIFIED.,.F.,
 .F.,.F.)
B_SPLINE_SURFACE_WITH_KNOTS((4,4),(3,3),(0.0051446850272488,0.00657473287039648),
(0.,1.),.UNSPECIFIED.)
GEOMETRIC_REPRESENTATION_ITEM()
RATIONAL_B_SPLINE_SURFACE(((1.,0.943476662524758,1.),(1.,0.944945702024752,
1.),(1.,0.946300916277093,1.),(1.,0.947565352018496,1.)))
REPRESENTATION_ITEM('')
SURFACE()
) ;
#411=(
BOUNDED_SURFACE()
B_SPLINE_SURFACE(3,2,((#106096,#106097,#106098),(#106099,#106100,#106101),
(#106102,#106103,#106104),(#106105,#106106,#106107),(#106108,#106109,#106110),
(#106111,#106112,#106113),(#106114,#106115,#106116),(#106117,#106118,#106119),
(#106120,#106121,#106122),(#106123,#106124,#106125),(#106126,#106127,#106128),
(#106129,#106130,#106131),(#106132,#106133,#106134),(#106135,#106136,#106137),
(#106138,#106139,#106140),(#106141,#106142,#106143),(#106144,#106145,#106146),
(#106147,#106148,#106149)),.UNSPECIFIED.,.F.,.F.,.F.)
B_SPLINE_SURFACE_WITH_KNOTS((4,2,2,2,2,2,2,2,4),(3,3),(-2.77591379149735E-5,
0.000125253167969377,0.000156566459961721,0.000187879751954065,0.000203536397950237,
0.000211364720948323,0.000219193043946409,0.000234849689942581,0.000250506335938753),
(0.,1.00287807885233),.UNSPECIFIED.)
GEOMETRIC_REPRESENTATION_ITEM()
RATIONAL_B_SPLINE_SURFACE(((1.,0.698587265144123,1.00173497923602),(1.,
0.713937574732621,1.00164662043321),(1.,0.719549163949218,1.00161431924071),
(1.,0.771808112009042,1.0013135084942),(1.,0.782482243723491,1.00125206650869),
(1.,0.810804881628056,1.0010890369383),(1.,0.82782480896442,1.00099106755243),
(1.,0.868687526094324,1.00075585530839),(1.,0.885097717150333,1.00066139566071),
(1.,0.918597380148702,1.00046856631744),(1.,0.931968622959456,1.00039159933511),
(1.,0.955741994674696,1.00025475605835),(1.,0.963776461019225,1.00020850840299),
(1.,0.965421728909339,1.00019903798155),(1.,0.949947468785964,1.00028811026319),
(1.,0.927474619202864,1.00041746752946),(1.,0.91633514021013,1.00048158812729),
(1.,0.906010523700257,1.00054101824816)))
REPRESENTATION_ITEM('')
SURFACE()
) ;
#412=(
BOUNDED_SURFACE()
B_SPLINE_SURFACE(3,2,((#106153,#106154,#106155),(#106156,#106157,#106158),
(#106159,#106160,#106161),(#106162,#106163,#106164),(#106165,#106166,#106167),
(#106168,#106169,#106170),(#106171,#106172,#106173),(#106174,#106175,#106176),
(#106177,#106178,#106179),(#106180,#106181,#106182),(#106183,#106184,#106185),
(#106186,#106187,#106188),(#106189,#106190,#106191),(#106192,#106193,#106194),
(#106195,#106196,#106197),(#106198,#106199,#106200),(#106201,#106202,#106203),
(#106204,#106205,#106206)),.UNSPECIFIED.,.F.,.F.,.F.)
B_SPLINE_SURFACE_WITH_KNOTS((4,2,2,2,2,2,2,2,4),(3,3),(-2.79610875103821E-5,
0.000125253167969377,0.000156566459961721,0.000187879751954065,0.000203536397950237,
0.000211364720948323,0.000219193043946409,0.000234849689942581,0.00025319538809668),
(-0.00314610977277591,1.),.UNSPECIFIED.)
GEOMETRIC_REPRESENTATION_ITEM()
RATIONAL_B_SPLINE_SURFACE(((1.00189744483744,0.698445862592552,0.999999999999999),
(1.00180054146116,0.713846370407211,1.),(1.00176549021887,0.719416939270069,
1.),(1.00143621720107,0.771747125052571,1.),(1.00136903527051,0.782424109553791,
1.),(1.00119077538539,0.810754317015272,1.),(1.00108365364405,0.827778793126799,
1.),(1.00082646773906,0.868652431296628,1.),(1.00072318361763,0.885067008168634,
1.),(1.00051234004798,0.918575624344512,1.),(1.00042818276661,0.931950440776572,
1.),(1.00027855551349,0.955730166204094,1.),(1.000227987376,0.96376677985388,
1.),(1.00021763222243,0.965412487461141,1.),(1.00031502568702,0.949934091660348,
1.),(1.0004686140099,0.925524847549937,1.),(1.00055064362453,0.912488173602174,
1.),(1.00062456604613,0.90073994691414,1.)))
REPRESENTATION_ITEM('')
SURFACE()
) ;
#413=(
BOUNDED_SURFACE()
B_SPLINE_SURFACE(3,2,((#106209,#106210,#106211),(#106212,#106213,#106214),
(#106215,#106216,#106217),(#106218,#106219,#106220)),.UNSPECIFIED.,.F.,
 .F.,.F.)
B_SPLINE_SURFACE_WITH_KNOTS((4,4),(3,3),(-1.77635683940025E-15,1.00173611575494),
(0.800638603120415,1.),.UNSPECIFIED.)
GEOMETRIC_REPRESENTATION_ITEM()
RATIONAL_B_SPLINE_SURFACE(((0.931056261594767,0.956944532691447,1.),(0.931106613485823,
0.956975977522398,1.),(0.926966069646252,0.95439020172828,1.),(0.920044734228408,
0.950067817452235,1.)))
REPRESENTATION_ITEM('')
SURFACE()
) ;
#414=(
BOUNDED_SURFACE()
B_SPLINE_SURFACE(3,2,((#106246,#106247,#106248),(#106249,#106250,#106251),
(#106252,#106253,#106254),(#106255,#106256,#106257)),.UNSPECIFIED.,.F.,
 .F.,.F.)
B_SPLINE_SURFACE_WITH_KNOTS((4,4),(3,3),(-8.88178419700125E-16,1.08063632538888),
(0.,1.),.UNSPECIFIED.)
GEOMETRIC_REPRESENTATION_ITEM()
RATIONAL_B_SPLINE_SURFACE(((1.,0.821344978643199,1.),(1.,0.821618737292292,
1.),(1.,0.799663084581839,1.),(1.,0.763019982472728,1.)))
REPRESENTATION_ITEM('')
SURFACE()
) ;
#415=(
BOUNDED_SURFACE()
B_SPLINE_SURFACE(3,2,((#107724,#107725,#107726),(#107727,#107728,#107729),
(#107730,#107731,#107732),(#107733,#107734,#107735),(#107736,#107737,#107738),
(#107739,#107740,#107741)),.UNSPECIFIED.,.F.,.F.,.F.)
B_SPLINE_SURFACE_WITH_KNOTS((4,2,4),(3,3),(9.07204043127126E-5,0.000289236237441534,
0.000487752070570335),(-0.000844756556539755,1.00064307855249),
 .UNSPECIFIED.)
GEOMETRIC_REPRESENTATION_ITEM()
RATIONAL_B_SPLINE_SURFACE(((1.00067853369612,0.598126578821559,1.00051643581304),
(1.0007017759524,0.584360946985556,1.00053412562504),(1.00066498743129,
0.60614959052921,1.00050612567469),(1.00056632625649,0.664583392835936,
1.00043103409954),(1.00050548323167,0.700618735924161,1.00038472613111),
(1.00047271456577,0.720026550083823,1.00035978571515)))
REPRESENTATION_ITEM('')
SURFACE()
) ;
#416=(
BOUNDED_SURFACE()
B_SPLINE_SURFACE(3,2,((#107756,#107757,#107758),(#107759,#107760,#107761),
(#107762,#107763,#107764),(#107765,#107766,#107767),(#107768,#107769,#107770),
(#107771,#107772,#107773)),.UNSPECIFIED.,.F.,.F.,.F.)
B_SPLINE_SURFACE_WITH_KNOTS((4,2,4),(3,3),(0.000107162911540598,0.000298022515767418,
0.000488882119994237),(-0.000759939855667643,1.00062534339582),
 .UNSPECIFIED.)
GEOMETRIC_REPRESENTATION_ITEM()
RATIONAL_B_SPLINE_SURFACE(((1.00042862573101,0.717810580914495,1.00035266240948),
(1.00045905072598,0.697780025035261,1.00037769532575),(1.0005111494633,
0.663480375353317,1.00042056084899),(1.00059665225221,0.607188882365452,
1.00049091038093),(1.00062840114514,0.586286726926244,1.00051703256695),
(1.00061268510756,0.596633514797517,1.00050410180877)))
REPRESENTATION_ITEM('')
SURFACE()
) ;
#417=(
BOUNDED_SURFACE()
B_SPLINE_SURFACE(3,2,((#108003,#108004,#108005),(#108006,#108007,#108008),
(#108009,#108010,#108011),(#108012,#108013,#108014),(#108015,#108016,#108017),
(#108018,#108019,#108020),(#108021,#108022,#108023),(#108024,#108025,#108026)),
 .UNSPECIFIED.,.F.,.F.,.F.)
B_SPLINE_SURFACE_WITH_KNOTS((4,2,2,4),(3,3),(6.28318530717959,6.67588438887831,
7.06858347057703,7.85398163397448),(0.,1.),.UNSPECIFIED.)
GEOMETRIC_REPRESENTATION_ITEM()
RATIONAL_B_SPLINE_SURFACE(((1.,0.707106781186548,1.),(1.,0.706675310150441,
1.),(1.,0.726552333979978,1.),(1.,0.787677905717226,1.),(1.,0.828238301901708,
1.),(1.,0.941599607549899,1.),(1.,1.00267605951738,1.),(1.,1.,1.)))
REPRESENTATION_ITEM('')
SURFACE()
) ;
#418=(
BOUNDED_SURFACE()
B_SPLINE_SURFACE(3,2,((#108034,#108035,#108036),(#108037,#108038,#108039),
(#108040,#108041,#108042),(#108043,#108044,#108045),(#108046,#108047,#108048),
(#108049,#108050,#108051),(#108052,#108053,#108054),(#108055,#108056,#108057)),
 .UNSPECIFIED.,.F.,.F.,.F.)
B_SPLINE_SURFACE_WITH_KNOTS((4,2,2,4),(3,3),(4.71238898038469,5.49778714378214,
5.89048622548086,6.28318530717959),(0.,1.),.UNSPECIFIED.)
GEOMETRIC_REPRESENTATION_ITEM()
RATIONAL_B_SPLINE_SURFACE(((1.,1.,1.),(1.,1.0026760595174,1.),(1.,0.94159960754987,
1.),(1.,0.828238301901727,1.),(1.,0.787677905717214,1.),(1.,0.726552333979982,
1.),(1.,0.706675310150449,1.),(1.,0.707106781186548,1.)))
REPRESENTATION_ITEM('')
SURFACE()
) ;
#419=(
BOUNDED_SURFACE()
B_SPLINE_SURFACE(3,2,((#108058,#108059,#108060),(#108061,#108062,#108063),
(#108064,#108065,#108066),(#108067,#108068,#108069),(#108070,#108071,#108072),
(#108073,#108074,#108075),(#108076,#108077,#108078),(#108079,#108080,#108081)),
 .UNSPECIFIED.,.F.,.F.,.F.)
B_SPLINE_SURFACE_WITH_KNOTS((4,2,2,4),(3,3),(4.71238898038469,5.49778714378214,
5.89048622548086,6.28318530717959),(0.,1.),.UNSPECIFIED.)
GEOMETRIC_REPRESENTATION_ITEM()
RATIONAL_B_SPLINE_SURFACE(((1.,1.,1.),(1.,1.00267605951745,1.),(1.,0.941599607549811,
1.),(1.,0.828238301901754,1.),(1.,0.787677905717219,1.),(1.,0.726552333979987,
1.),(1.,0.706675310150434,1.),(1.,0.707106781186548,1.)))
REPRESENTATION_ITEM('')
SURFACE()
) ;
#420=(
BOUNDED_SURFACE()
B_SPLINE_SURFACE(3,2,((#108089,#108090,#108091),(#108092,#108093,#108094),
(#108095,#108096,#108097),(#108098,#108099,#108100),(#108101,#108102,#108103),
(#108104,#108105,#108106),(#108107,#108108,#108109),(#108110,#108111,#108112)),
 .UNSPECIFIED.,.F.,.F.,.F.)
B_SPLINE_SURFACE_WITH_KNOTS((4,2,2,4),(3,3),(6.28318530717959,6.67588438887831,
7.06858347057703,7.85398163397448),(0.,1.),.UNSPECIFIED.)
GEOMETRIC_REPRESENTATION_ITEM()
RATIONAL_B_SPLINE_SURFACE(((1.,0.707106781186548,1.),(1.,0.70667531015044,
1.),(1.,0.726552333979978,1.),(1.,0.787677905717226,1.),(1.,0.828238301901736,
1.),(1.,0.941599607549842,1.),(1.,1.00267605951742,1.),(1.,1.,1.)))
REPRESENTATION_ITEM('')
SURFACE()
) ;
#421=(
BOUNDED_SURFACE()
B_SPLINE_SURFACE(3,2,((#108113,#108114,#108115),(#108116,#108117,#108118),
(#108119,#108120,#108121),(#108122,#108123,#108124),(#108125,#108126,#108127),
(#108128,#108129,#108130)),.UNSPECIFIED.,.F.,.F.,.F.)
B_SPLINE_SURFACE_WITH_KNOTS((4,2,4),(3,3),(2.06095632820092,2.9281173096476,
3.79527829109429),(0.,1.),.UNSPECIFIED.)
GEOMETRIC_REPRESENTATION_ITEM()
RATIONAL_B_SPLINE_SURFACE(((1.,0.763019982472728,1.),(1.,0.792403856906196,
1.),(1.,0.812400188579439,1.),(1.,0.825457041220947,1.),(1.,0.818529518851322,
1.),(1.,0.799131938862213,1.)))
REPRESENTATION_ITEM('')
SURFACE()
) ;
#422=(
BOUNDED_SURFACE()
B_SPLINE_SURFACE(3,2,((#108153,#108154,#108155),(#108156,#108157,#108158),
(#108159,#108160,#108161),(#108162,#108163,#108164),(#108165,#108166,#108167),
(#108168,#108169,#108170)),.UNSPECIFIED.,.F.,.F.,.F.)
B_SPLINE_SURFACE_WITH_KNOTS((4,2,4),(3,3),(2.13522523980986,3.02435044878098,
3.91347565775211),(0.,1.),.UNSPECIFIED.)
GEOMETRIC_REPRESENTATION_ITEM()
RATIONAL_B_SPLINE_SURFACE(((1.,0.749240327740271,1.),(1.,0.768579562596362,
1.),(1.,0.780993049743008,1.),(1.,0.78606840104594,1.),(1.,0.778729916329028,
1.),(1.,0.763019982472728,1.)))
REPRESENTATION_ITEM('')
SURFACE()
) ;
#423=(
BOUNDED_SURFACE()
B_SPLINE_SURFACE(3,2,((#108327,#108328,#108329),(#108330,#108331,#108332),
(#108333,#108334,#108335),(#108336,#108337,#108338),(#108339,#108340,#108341),
(#108342,#108343,#108344),(#108345,#108346,#108347),(#108348,#108349,#108350),
(#108351,#108352,#108353),(#108354,#108355,#108356),(#108357,#108358,#108359),
(#108360,#108361,#108362),(#108363,#108364,#108365),(#108366,#108367,#108368),
(#108369,#108370,#108371),(#108372,#108373,#108374),(#108375,#108376,#108377),
(#108378,#108379,#108380)),.UNSPECIFIED.,.F.,.F.,.F.)
B_SPLINE_SURFACE_WITH_KNOTS((4,2,2,2,2,2,2,2,4),(3,3),(-2.88136898044851E-5,
0.000144068449022425,0.000180085561278031,0.000216102673533637,0.00023411122966144,
0.000243115507725342,0.000252119785789243,0.000270128341917046,0.000315232069288961),
(-0.00230043332275091,1.00649231299441),.UNSPECIFIED.)
GEOMETRIC_REPRESENTATION_ITEM()
RATIONAL_B_SPLINE_SURFACE(((1.00137797387076,0.698547958833899,1.00390520040649),
(1.00130996746083,0.713425360736938,1.00371246913244),(1.00133921304011,
0.70702746034338,1.00379535158075),(1.00112343332499,0.754232445101169,
1.00318382835154),(1.00107694244868,0.764403007733155,1.00305207245044),
(1.00092854904603,0.796866246024235,1.00263152312896),(1.0008372304274,
0.816843536281796,1.00237272467553),(1.00052495197507,0.885159038383831,
1.00148772245247),(1.00036238583105,0.920722772197686,1.00102700735096),
(1.00013066612426,0.97141486445809,1.0003703099256),(1.00008161134635,0.982146318257279,
1.00023128788556),(1.00010185218181,0.977718337948419,1.00028865074314),
(1.00015066464689,0.967039893644228,1.00042698606465),(1.00027150756254,
0.940603729390326,1.00076945685699),(1.00035349548852,0.922667665318131,
1.00100181197535),(1.00060974665109,0.866608956479371,1.00172803194619),
(1.00075148156336,0.835602360842761,1.00212971099741),(1.00085165739527,
0.813687424975854,1.00241361093759)))
REPRESENTATION_ITEM('')
SURFACE()
) ;
#424=(
BOUNDED_SURFACE()
B_SPLINE_SURFACE(3,2,((#108382,#108383,#108384),(#108385,#108386,#108387),
(#108388,#108389,#108390),(#108391,#108392,#108393)),.UNSPECIFIED.,.F.,
 .F.,.F.)
B_SPLINE_SURFACE_WITH_KNOTS((4,4),(3,3),(5.63598348762741,6.28318530717959),
(0.792338840560947,1.),.UNSPECIFIED.)
GEOMETRIC_REPRESENTATION_ITEM()
RATIONAL_B_SPLINE_SURFACE(((0.934040253948337,0.958376553896458,1.),(0.938725627259263,
0.961333226642432,1.),(0.941220250254377,0.96290744140221,1.),(0.941208919370362,
0.962900291125438,1.)))
REPRESENTATION_ITEM('')
SURFACE()
) ;
#425=(
BOUNDED_SURFACE()
B_SPLINE_SURFACE(3,2,((#108434,#108435,#108436),(#108437,#108438,#108439),
(#108440,#108441,#108442),(#108443,#108444,#108445),(#108446,#108447,#108448),
(#108449,#108450,#108451),(#108452,#108453,#108454),(#108455,#108456,#108457),
(#108458,#108459,#108460),(#108461,#108462,#108463),(#108464,#108465,#108466),
(#108467,#108468,#108469),(#108470,#108471,#108472),(#108473,#108474,#108475),
(#108476,#108477,#108478),(#108479,#108480,#108481),(#108482,#108483,#108484),
(#108485,#108486,#108487)),.UNSPECIFIED.,.F.,.F.,.F.)
B_SPLINE_SURFACE_WITH_KNOTS((4,2,2,2,2,2,2,2,4),(3,3),(-3.19743590576725E-5,
0.000144068449022543,0.000180085561278178,0.000216102673533814,0.000234111229661632,
0.000243115507725541,0.00025211978578945,0.000270128341917267,0.000288136898045085),
(-0.0066834189729316,1.00019683226125),.UNSPECIFIED.)
GEOMETRIC_REPRESENTATION_ITEM()
RATIONAL_B_SPLINE_SURFACE(((1.00403209003416,0.69829147589393,1.00011798325537),
(1.00381915098331,0.714225030505279,1.0001117524316),(1.00391733895256,
0.706877935813777,1.00011462551633),(1.00327816898475,0.754704999695305,
1.00009592272127),(1.00314250899907,0.764856006670041,1.00009195316538),
(1.00270949829937,0.797256825605557,1.00007928281042),(1.00244303133896,
0.817195704119684,1.00007148570292),(1.00153180544397,0.885379851193009,
1.00004482226124),(1.00105743880425,0.920875204110236,1.00003094178737),
(1.00038128265055,0.971469827114243,1.00001115673706),(1.00023814122159,
0.982180646789321,1.00000696826617),(1.0002972038091,0.977761180469343,
1.00000869650048),(1.00043963817126,0.967103268362385,1.00001286428185),
(1.00079225678184,0.940717934784041,1.00002318227853),(1.00103149685962,
0.922816357645972,1.0000301826984),(1.00145821870311,0.890886113898623,
1.00004266903471),(1.0016523226799,0.876361928211943,1.00004834872412),
(1.00182713963616,0.863280929173184,1.00005346405474)))
REPRESENTATION_ITEM('')
SURFACE()
) ;
#426=(
BOUNDED_SURFACE()
B_SPLINE_SURFACE(3,2,((#108526,#108527,#108528),(#108529,#108530,#108531),
(#108532,#108533,#108534),(#108535,#108536,#108537)),.UNSPECIFIED.,.F.,
 .F.,.F.)
B_SPLINE_SURFACE_WITH_KNOTS((4,4),(3,3),(5.51130230301727,6.28318530717958),
(0.,1.),.UNSPECIFIED.)
GEOMETRIC_REPRESENTATION_ITEM()
RATIONAL_B_SPLINE_SURFACE(((1.,0.763019982472728,1.),(1.,0.776565014072567,
1.),(1.,0.78408875836913,1.),(1.,0.784033077704815,1.)))
REPRESENTATION_ITEM('')
SURFACE()
) ;
#427=(
BOUNDED_SURFACE()
B_SPLINE_SURFACE(3,2,((#108542,#108543,#108544),(#108545,#108546,#108547),
(#108548,#108549,#108550),(#108551,#108552,#108553)),.UNSPECIFIED.,.F.,
 .F.,.F.)
B_SPLINE_SURFACE_WITH_KNOTS((4,4),(3,3),(0.0051446850272488,0.00657473287039649),
(0.,1.),.UNSPECIFIED.)
GEOMETRIC_REPRESENTATION_ITEM()
RATIONAL_B_SPLINE_SURFACE(((1.,0.943476662524758,1.),(1.,0.94494570202475,
1.),(1.,0.946300916277098,1.),(1.,0.947565352018496,1.)))
REPRESENTATION_ITEM('')
SURFACE()
) ;
#428=(
BOUNDED_SURFACE()
B_SPLINE_SURFACE(3,2,((#108592,#108593,#108594),(#108595,#108596,#108597),
(#108598,#108599,#108600),(#108601,#108602,#108603)),.UNSPECIFIED.,.F.,
 .F.,.F.)
B_SPLINE_SURFACE_WITH_KNOTS((4,4),(3,3),(0.0051446850272488,0.00657473287039648),
(0.,1.),.UNSPECIFIED.)
GEOMETRIC_REPRESENTATION_ITEM()
RATIONAL_B_SPLINE_SURFACE(((1.,0.943476662524758,1.),(1.,0.944945702024751,
1.),(1.,0.946300916277097,1.),(1.,0.947565352018496,1.)))
REPRESENTATION_ITEM('')
SURFACE()
) ;
#429=(
BOUNDED_SURFACE()
B_SPLINE_SURFACE(3,2,((#108608,#108609,#108610),(#108611,#108612,#108613),
(#108614,#108615,#108616),(#108617,#108618,#108619),(#108620,#108621,#108622),
(#108623,#108624,#108625),(#108626,#108627,#108628),(#108629,#108630,#108631),
(#108632,#108633,#108634),(#108635,#108636,#108637),(#108638,#108639,#108640),
(#108641,#108642,#108643),(#108644,#108645,#108646),(#108647,#108648,#108649),
(#108650,#108651,#108652),(#108653,#108654,#108655),(#108656,#108657,#108658),
(#108659,#108660,#108661)),.UNSPECIFIED.,.F.,.F.,.F.)
B_SPLINE_SURFACE_WITH_KNOTS((4,2,2,2,2,2,2,2,4),(3,3),(-2.77591379149846E-5,
0.00012525316796938,0.000156566459961724,0.000187879751954069,0.000203536397950241,
0.000211364720948327,0.000219193043946413,0.000234849689942586,0.000250506335938758),
(0.,1.00287807885244),.UNSPECIFIED.)
GEOMETRIC_REPRESENTATION_ITEM()
RATIONAL_B_SPLINE_SURFACE(((1.,0.6985872651442,1.00173497923609),(1.,0.713937574732387,
1.00164662043327),(1.,0.719549163949333,1.00161431924077),(1.,0.771808112008987,
1.00131350849425),(1.,0.78248224372348,1.00125206650874),(1.,0.810804881628055,
1.00108903693834),(1.,0.82782480896445,1.00099106755247),(1.,0.868687526094294,
1.00075585530842),(1.,0.885097717150226,1.00066139566073),(1.,0.918597380148776,
1.00046856631745),(1.,0.931968622959474,1.00039159933513),(1.,0.955741994674726,
1.00025475605836),(1.,0.963776461019231,1.000208508403),(1.,0.965421728909319,
1.00019903798156),(1.,0.949947468785985,1.0002881102632),(1.,0.92747461920283,
1.00041746752947),(1.,0.916335140210132,1.00048158812731),(1.,0.906010523700246,
1.00054101824818)))
REPRESENTATION_ITEM('')
SURFACE()
) ;
#430=(
BOUNDED_SURFACE()
B_SPLINE_SURFACE(3,2,((#108665,#108666,#108667),(#108668,#108669,#108670),
(#108671,#108672,#108673),(#108674,#108675,#108676),(#108677,#108678,#108679),
(#108680,#108681,#108682),(#108683,#108684,#108685),(#108686,#108687,#108688),
(#108689,#108690,#108691),(#108692,#108693,#108694),(#108695,#108696,#108697),
(#108698,#108699,#108700),(#108701,#108702,#108703),(#108704,#108705,#108706),
(#108707,#108708,#108709),(#108710,#108711,#108712),(#108713,#108714,#108715),
(#108716,#108717,#108718)),.UNSPECIFIED.,.F.,.F.,.F.)
B_SPLINE_SURFACE_WITH_KNOTS((4,2,2,2,2,2,2,2,4),(3,3),(-2.79610875103729E-5,
0.000125253167969372,0.000156566459961715,0.000187879751954059,0.00020353639795023,
0.000211364720948316,0.000219193043946402,0.000234849689942574,0.000253195388096673),
(-0.00314610977265889,1.),.UNSPECIFIED.)
GEOMETRIC_REPRESENTATION_ITEM()
RATIONAL_B_SPLINE_SURFACE(((1.00189744483737,0.698445862592838,0.999999999999999),
(1.00180054146109,0.713846370406803,1.),(1.0017654902188,0.719416939270416,
1.),(1.00143621720102,0.771747125052534,1.),(1.00136903527045,0.782424109553835,
1.),(1.00119077538534,0.810754317015274,1.),(1.00108365364401,0.827778793126865,
1.),(1.00082646773903,0.868652431296584,1.),(1.0007231836176,0.885067008168485,
1.),(1.00051234004796,0.91857562434451,1.),(1.0004281827666,0.931950440776612,
1.),(1.00027855551348,0.955730166203988,1.),(1.00022798737599,0.963766779853886,
1.),(1.00021763222242,0.965412487461145,1.),(1.00031502568701,0.949934091660368,
1.),(1.00046861400989,0.925524847549974,1.),(1.00055064362451,0.912488173602136,
1.),(1.00062456604611,0.900739946914172,1.)))
REPRESENTATION_ITEM('')
SURFACE()
) ;
#431=(
BOUNDED_SURFACE()
B_SPLINE_SURFACE(3,2,((#108721,#108722,#108723),(#108724,#108725,#108726),
(#108727,#108728,#108729),(#108730,#108731,#108732)),.UNSPECIFIED.,.F.,
 .F.,.F.)
B_SPLINE_SURFACE_WITH_KNOTS((4,4),(3,3),(-1.77635683940025E-15,1.00173611575494),
(0.800638603120396,1.),.UNSPECIFIED.)
GEOMETRIC_REPRESENTATION_ITEM()
RATIONAL_B_SPLINE_SURFACE(((0.931056261594762,0.956944532691443,1.),(0.931106613485818,
0.956975977522394,1.),(0.926966069646247,0.954390201728275,1.),(0.920044734228403,
0.950067817452231,1.)))
REPRESENTATION_ITEM('')
SURFACE()
) ;
#432=(
BOUNDED_SURFACE()
B_SPLINE_SURFACE(3,2,((#108758,#108759,#108760),(#108761,#108762,#108763),
(#108764,#108765,#108766),(#108767,#108768,#108769)),.UNSPECIFIED.,.F.,
 .F.,.F.)
B_SPLINE_SURFACE_WITH_KNOTS((4,4),(3,3),(-8.88178419700125E-16,1.08063632538888),
(0.,1.),.UNSPECIFIED.)
GEOMETRIC_REPRESENTATION_ITEM()
RATIONAL_B_SPLINE_SURFACE(((1.,0.8213449786432,1.),(1.,0.821618737292288,
1.),(1.,0.799663084581846,1.),(1.,0.763019982472728,1.)))
REPRESENTATION_ITEM('')
SURFACE()
) ;
#433=(
BOUNDED_SURFACE()
B_SPLINE_SURFACE(3,2,((#110236,#110237,#110238),(#110239,#110240,#110241),
(#110242,#110243,#110244),(#110245,#110246,#110247),(#110248,#110249,#110250),
(#110251,#110252,#110253)),.UNSPECIFIED.,.F.,.F.,.F.)
B_SPLINE_SURFACE_WITH_KNOTS((4,2,4),(3,3),(9.07204043127176E-5,0.000289236237441533,
0.000487752070570311),(-0.000844756555347329,1.00064307855269),
 .UNSPECIFIED.)
GEOMETRIC_REPRESENTATION_ITEM()
RATIONAL_B_SPLINE_SURFACE(((1.00067853369516,0.598126578821866,1.0005164358132),
(1.00070177595141,0.584360946986094,1.0005341256252),(1.00066498743035,
0.606149590529527,1.00050612567485),(1.00056632625569,0.66458339283634,
1.00043103409967),(1.00050548323096,0.700618735924348,1.00038472613123),
(1.00047271456509,0.720026550084158,1.00035978571527)))
REPRESENTATION_ITEM('')
SURFACE()
) ;
#434=(
BOUNDED_SURFACE()
B_SPLINE_SURFACE(3,2,((#110268,#110269,#110270),(#110271,#110272,#110273),
(#110274,#110275,#110276),(#110277,#110278,#110279),(#110280,#110281,#110282),
(#110283,#110284,#110285)),.UNSPECIFIED.,.F.,.F.,.F.)
B_SPLINE_SURFACE_WITH_KNOTS((4,2,4),(3,3),(0.000107162911540598,0.000298022515767418,
0.000488882119994237),(-0.00075993985566105,1.00062534339582),
 .UNSPECIFIED.)
GEOMETRIC_REPRESENTATION_ITEM()
RATIONAL_B_SPLINE_SURFACE(((1.00042862573101,0.717810580914573,1.00035266240948),
(1.00045905072598,0.697780025035115,1.00037769532575),(1.0005111494633,
0.663480375353433,1.00042056084899),(1.0005966522522,0.607188882365342,
1.00049091038092),(1.00062840114514,0.586286726926399,1.00051703256695),
(1.00061268510756,0.596633514797443,1.00050410180877)))
REPRESENTATION_ITEM('')
SURFACE()
) ;
#435=(
BOUNDED_SURFACE()
B_SPLINE_SURFACE(3,2,((#110515,#110516,#110517),(#110518,#110519,#110520),
(#110521,#110522,#110523),(#110524,#110525,#110526),(#110527,#110528,#110529),
(#110530,#110531,#110532),(#110533,#110534,#110535),(#110536,#110537,#110538)),
 .UNSPECIFIED.,.F.,.F.,.F.)
B_SPLINE_SURFACE_WITH_KNOTS((4,2,2,4),(3,3),(6.28318530717959,6.67588438887831,
7.06858347057703,7.85398163397448),(0.,1.),.UNSPECIFIED.)
GEOMETRIC_REPRESENTATION_ITEM()
RATIONAL_B_SPLINE_SURFACE(((1.,0.707106781186548,1.),(1.,0.706675310150436,
1.),(1.,0.726552333979984,1.),(1.,0.787677905717219,1.),(1.,0.828238301901734,
1.),(1.,0.94159960754984,1.),(1.,1.00267605951742,1.),(1.,1.,1.)))
REPRESENTATION_ITEM('')
SURFACE()
) ;
#436=(
BOUNDED_SURFACE()
B_SPLINE_SURFACE(3,2,((#110546,#110547,#110548),(#110549,#110550,#110551),
(#110552,#110553,#110554),(#110555,#110556,#110557),(#110558,#110559,#110560),
(#110561,#110562,#110563),(#110564,#110565,#110566),(#110567,#110568,#110569)),
 .UNSPECIFIED.,.F.,.F.,.F.)
B_SPLINE_SURFACE_WITH_KNOTS((4,2,2,4),(3,3),(4.71238898038469,5.49778714378214,
5.89048622548086,6.28318530717959),(0.,1.),.UNSPECIFIED.)
GEOMETRIC_REPRESENTATION_ITEM()
RATIONAL_B_SPLINE_SURFACE(((1.,1.,1.),(1.,1.0026760595174,1.),(1.,0.94159960754987,
1.),(1.,0.828238301901727,1.),(1.,0.787677905717213,1.),(1.,0.726552333979991,
1.),(1.,0.706675310150431,1.),(1.,0.707106781186548,1.)))
REPRESENTATION_ITEM('')
SURFACE()
) ;
#437=(
BOUNDED_SURFACE()
B_SPLINE_SURFACE(3,2,((#110570,#110571,#110572),(#110573,#110574,#110575),
(#110576,#110577,#110578),(#110579,#110580,#110581),(#110582,#110583,#110584),
(#110585,#110586,#110587),(#110588,#110589,#110590),(#110591,#110592,#110593)),
 .UNSPECIFIED.,.F.,.F.,.F.)
B_SPLINE_SURFACE_WITH_KNOTS((4,2,2,4),(3,3),(4.71238898038469,5.49778714378214,
5.89048622548086,6.28318530717959),(0.,1.),.UNSPECIFIED.)
GEOMETRIC_REPRESENTATION_ITEM()
RATIONAL_B_SPLINE_SURFACE(((1.,1.,1.),(1.,1.00267605951744,1.),(1.,0.941599607549825,
1.),(1.,0.828238301901746,1.),(1.,0.787677905717283,1.),(1.,0.726552333979923,
1.),(1.,0.706675310150477,1.),(1.,0.707106781186554,1.)))
REPRESENTATION_ITEM('')
SURFACE()
) ;
#438=(
BOUNDED_SURFACE()
B_SPLINE_SURFACE(3,2,((#110601,#110602,#110603),(#110604,#110605,#110606),
(#110607,#110608,#110609),(#110610,#110611,#110612),(#110613,#110614,#110615),
(#110616,#110617,#110618),(#110619,#110620,#110621),(#110622,#110623,#110624)),
 .UNSPECIFIED.,.F.,.F.,.F.)
B_SPLINE_SURFACE_WITH_KNOTS((4,2,2,4),(3,3),(6.28318530717959,6.67588438887831,
7.06858347057703,7.85398163397448),(0.,1.),.UNSPECIFIED.)
GEOMETRIC_REPRESENTATION_ITEM()
RATIONAL_B_SPLINE_SURFACE(((1.,0.707106781186548,1.),(1.,0.706675310150428,
1.),(1.,0.726552333979983,1.),(1.,0.78767790571723,1.),(1.,0.828238301901763,
1.),(1.,0.941599607549783,1.),(1.,1.00267605951747,1.),(1.,1.,1.)))
REPRESENTATION_ITEM('')
SURFACE()
) ;
#439=(
BOUNDED_SURFACE()
B_SPLINE_SURFACE(3,2,((#110625,#110626,#110627),(#110628,#110629,#110630),
(#110631,#110632,#110633),(#110634,#110635,#110636),(#110637,#110638,#110639),
(#110640,#110641,#110642)),.UNSPECIFIED.,.F.,.F.,.F.)
B_SPLINE_SURFACE_WITH_KNOTS((4,2,4),(3,3),(2.06095632820092,2.92811730964759,
3.79527829109427),(0.,1.),.UNSPECIFIED.)
GEOMETRIC_REPRESENTATION_ITEM()
RATIONAL_B_SPLINE_SURFACE(((1.,0.763019982472728,1.),(1.,0.792403856906218,
1.),(1.,0.812400188579406,1.),(1.,0.825457041220978,1.),(1.,0.818529518851298,
1.),(1.,0.799131938862213,1.)))
REPRESENTATION_ITEM('')
SURFACE()
) ;
#440=(
BOUNDED_SURFACE()
B_SPLINE_SURFACE(3,2,((#110665,#110666,#110667),(#110668,#110669,#110670),
(#110671,#110672,#110673),(#110674,#110675,#110676),(#110677,#110678,#110679),
(#110680,#110681,#110682)),.UNSPECIFIED.,.F.,.F.,.F.)
B_SPLINE_SURFACE_WITH_KNOTS((4,2,4),(3,3),(2.13522523980989,3.02435044878099,
3.9134756577521),(0.,1.),.UNSPECIFIED.)
GEOMETRIC_REPRESENTATION_ITEM()
RATIONAL_B_SPLINE_SURFACE(((1.,0.749240327740279,1.),(1.,0.768579562596332,
1.),(1.,0.780993049743038,1.),(1.,0.78606840104591,1.),(1.,0.778729916329054,
1.),(1.,0.763019982472728,1.)))
REPRESENTATION_ITEM('')
SURFACE()
) ;
#441=(
BOUNDED_SURFACE()
B_SPLINE_SURFACE(3,2,((#110839,#110840,#110841),(#110842,#110843,#110844),
(#110845,#110846,#110847),(#110848,#110849,#110850),(#110851,#110852,#110853),
(#110854,#110855,#110856),(#110857,#110858,#110859),(#110860,#110861,#110862),
(#110863,#110864,#110865),(#110866,#110867,#110868),(#110869,#110870,#110871),
(#110872,#110873,#110874),(#110875,#110876,#110877),(#110878,#110879,#110880),
(#110881,#110882,#110883),(#110884,#110885,#110886),(#110887,#110888,#110889),
(#110890,#110891,#110892)),.UNSPECIFIED.,.F.,.F.,.F.)
B_SPLINE_SURFACE_WITH_KNOTS((4,2,2,2,2,2,2,2,4),(3,3),(-2.88136898044833E-5,
0.000144068449022426,0.000180085561278032,0.000216102673533639,0.000234111229661442,
0.000243115507725343,0.000252119785789245,0.000270128341917048,0.000315232069288965),
(-0.00230043332394133,1.00649231299454),.UNSPECIFIED.)
GEOMETRIC_REPRESENTATION_ITEM()
RATIONAL_B_SPLINE_SURFACE(((1.00137797387148,0.69854795883355,1.00390520040657),
(1.00130996746151,0.71342536073646,1.00371246913252),(1.00133921304081,
0.707027460343067,1.00379535158082),(1.00112343332557,0.754232445100828,
1.0031838283516),(1.00107694244924,0.764403007732966,1.0030520724505),(1.00092854904651,
0.796866246023831,1.00263152312901),(1.00083723042783,0.816843536281475,
1.00237272467558),(1.00052495197535,0.885159038383718,1.0014877224525),
(1.00036238583123,0.920722772198033,1.00102700735098),(1.00013066612433,
0.971414864457831,1.00037030992562),(1.00008161134639,0.982146318257256,
1.00023128788557),(1.00010185218186,0.977718337948391,1.00028865074313),
(1.00015066464697,0.96703989364419,1.00042698606466),(1.00027150756269,
0.940603729390218,1.00076945685701),(1.0003534954887,0.922667665318,1.00100181197537),
(1.00060974665141,0.866608956479275,1.00172803194623),(1.00075148156375,
0.835602360842203,1.00212971099746),(1.00085165739571,0.813687424976644,
1.00241361093764)))
REPRESENTATION_ITEM('')
SURFACE()
) ;
#442=(
BOUNDED_SURFACE()
B_SPLINE_SURFACE(3,2,((#110894,#110895,#110896),(#110897,#110898,#110899),
(#110900,#110901,#110902),(#110903,#110904,#110905)),.UNSPECIFIED.,.F.,
 .F.,.F.)
B_SPLINE_SURFACE_WITH_KNOTS((4,4),(3,3),(5.63598348762741,6.28318530717959),
(0.792338840560962,1.),.UNSPECIFIED.)
GEOMETRIC_REPRESENTATION_ITEM()
RATIONAL_B_SPLINE_SURFACE(((0.934040253948341,0.958376553896461,1.),(0.938725627259267,
0.961333226642435,1.),(0.941220250254379,0.962907441402212,1.),(0.941208919370365,
0.962900291125441,1.)))
REPRESENTATION_ITEM('')
SURFACE()
) ;
#443=(
BOUNDED_SURFACE()
B_SPLINE_SURFACE(3,2,((#110946,#110947,#110948),(#110949,#110950,#110951),
(#110952,#110953,#110954),(#110955,#110956,#110957),(#110958,#110959,#110960),
(#110961,#110962,#110963),(#110964,#110965,#110966),(#110967,#110968,#110969),
(#110970,#110971,#110972),(#110973,#110974,#110975),(#110976,#110977,#110978),
(#110979,#110980,#110981),(#110982,#110983,#110984),(#110985,#110986,#110987),
(#110988,#110989,#110990),(#110991,#110992,#110993),(#110994,#110995,#110996),
(#110997,#110998,#110999)),.UNSPECIFIED.,.F.,.F.,.F.)
B_SPLINE_SURFACE_WITH_KNOTS((4,2,2,2,2,2,2,2,4),(3,3),(-3.1974359057668E-5,
0.000144068449022543,0.000180085561278178,0.000216102673533814,0.000234111229661632,
0.000243115507725541,0.00025211978578945,0.000270128341917267,0.000288136898045085),
(-0.00668341897303802,1.00019683226125),.UNSPECIFIED.)
GEOMETRIC_REPRESENTATION_ITEM()
RATIONAL_B_SPLINE_SURFACE(((1.00403209003423,0.698291475893822,1.00011798325538),
(1.00381915098337,0.714225030505383,1.00011175243161),(1.00391733895262,
0.706877935813645,1.00011462551632),(1.0032781689848,0.754704999695298,
1.00009592272127),(1.00314250899912,0.764856006669979,1.00009195316538),
(1.00270949829941,0.79725682560557,1.00007928281042),(1.00244303133899,
0.817195704119653,1.00007148570293),(1.001531805444,0.885379851193002,1.00004482226125),
(1.00105743880427,0.920875204110228,1.00003094178737),(1.00038128265056,
0.971469827114239,1.00001115673706),(1.0002381412216,0.982180646789319,
1.00000696826617),(1.0002972038091,0.97776118046934,1.00000869650048),(1.00043963817127,
0.967103268362382,1.00001286428185),(1.00079225678185,0.940717934784034,
1.00002318227853),(1.00103149685964,0.922816357645954,1.0000301826984),
(1.00145821870313,0.890886113898608,1.00004266903471),(1.00165232267993,
0.876361928211933,1.00004834872412),(1.00182713963619,0.863280929173169,
1.00005346405474)))
REPRESENTATION_ITEM('')
SURFACE()
) ;
#444=(
BOUNDED_SURFACE()
B_SPLINE_SURFACE(3,2,((#111038,#111039,#111040),(#111041,#111042,#111043),
(#111044,#111045,#111046),(#111047,#111048,#111049)),.UNSPECIFIED.,.F.,
 .F.,.F.)
B_SPLINE_SURFACE_WITH_KNOTS((4,4),(3,3),(5.51130230301728,6.28318530717958),
(0.,1.),.UNSPECIFIED.)
GEOMETRIC_REPRESENTATION_ITEM()
RATIONAL_B_SPLINE_SURFACE(((1.,0.763019982472728,1.),(1.,0.776565014072563,
1.),(1.,0.78408875836913,1.),(1.,0.784033077704815,1.)))
REPRESENTATION_ITEM('')
SURFACE()
) ;
#445=(
BOUNDED_SURFACE()
B_SPLINE_SURFACE(3,2,((#111054,#111055,#111056),(#111057,#111058,#111059),
(#111060,#111061,#111062),(#111063,#111064,#111065)),.UNSPECIFIED.,.F.,
 .F.,.F.)
B_SPLINE_SURFACE_WITH_KNOTS((4,4),(3,3),(0.0051446850272488,0.00657473287039649),
(0.,1.),.UNSPECIFIED.)
GEOMETRIC_REPRESENTATION_ITEM()
RATIONAL_B_SPLINE_SURFACE(((1.,0.943476662524758,1.),(1.,0.944945702024748,
1.),(1.,0.946300916277099,1.),(1.,0.947565352018495,1.)))
REPRESENTATION_ITEM('')
SURFACE()
) ;
#446=(
BOUNDED_SURFACE()
B_SPLINE_SURFACE(3,2,((#111104,#111105,#111106),(#111107,#111108,#111109),
(#111110,#111111,#111112),(#111113,#111114,#111115)),.UNSPECIFIED.,.F.,
 .F.,.F.)
B_SPLINE_SURFACE_WITH_KNOTS((4,4),(3,3),(0.0051446850272488,0.00657473287039648),
(0.,1.),.UNSPECIFIED.)
GEOMETRIC_REPRESENTATION_ITEM()
RATIONAL_B_SPLINE_SURFACE(((1.,0.943476662524758,1.),(1.,0.944945702024752,
1.),(1.,0.946300916277091,1.),(1.,0.947565352018496,1.)))
REPRESENTATION_ITEM('')
SURFACE()
) ;
#447=(
BOUNDED_SURFACE()
B_SPLINE_SURFACE(3,2,((#111120,#111121,#111122),(#111123,#111124,#111125),
(#111126,#111127,#111128),(#111129,#111130,#111131),(#111132,#111133,#111134),
(#111135,#111136,#111137),(#111138,#111139,#111140),(#111141,#111142,#111143),
(#111144,#111145,#111146),(#111147,#111148,#111149),(#111150,#111151,#111152),
(#111153,#111154,#111155),(#111156,#111157,#111158),(#111159,#111160,#111161),
(#111162,#111163,#111164),(#111165,#111166,#111167),(#111168,#111169,#111170),
(#111171,#111172,#111173)),.UNSPECIFIED.,.F.,.F.,.F.)
B_SPLINE_SURFACE_WITH_KNOTS((4,2,2,2,2,2,2,2,4),(3,3),(-2.77591379148802E-5,
0.000125253167969374,0.000156566459961717,0.000187879751954061,0.000203536397950232,
0.000211364720948318,0.000219193043946404,0.000234849689942576,0.000250506335938747),
(0.,1.00287807885236),.UNSPECIFIED.)
GEOMETRIC_REPRESENTATION_ITEM()
RATIONAL_B_SPLINE_SURFACE(((1.,0.698587265144137,1.00173497923604),(1.,
0.713937574732619,1.00164662043323),(1.,0.719549163949235,1.00161431924073),
(1.,0.771808112009033,1.00131350849422),(1.,0.782482243723513,1.00125206650871),
(1.,0.810804881628019,1.00108903693831),(1.,0.827824808964515,1.00099106755244),
(1.,0.868687526094263,1.0007558553084),(1.,0.885097717150305,1.00066139566072),
(1.,0.918597380148718,1.00046856631744),(1.,0.931968622959399,1.00039159933512),
(1.,0.955741994674697,1.00025475605835),(1.,0.963776461019228,1.000208508403),
(1.,0.965421728909335,1.00019903798155),(1.,0.949947468785963,1.00028811026319),
(1.,0.927474619202861,1.00041746752946),(1.,0.916335140210129,1.00048158812729),
(1.,0.906010523700251,1.00054101824817)))
REPRESENTATION_ITEM('')
SURFACE()
) ;
#448=(
BOUNDED_SURFACE()
B_SPLINE_SURFACE(3,2,((#111177,#111178,#111179),(#111180,#111181,#111182),
(#111183,#111184,#111185),(#111186,#111187,#111188),(#111189,#111190,#111191),
(#111192,#111193,#111194),(#111195,#111196,#111197),(#111198,#111199,#111200),
(#111201,#111202,#111203),(#111204,#111205,#111206),(#111207,#111208,#111209),
(#111210,#111211,#111212),(#111213,#111214,#111215),(#111216,#111217,#111218),
(#111219,#111220,#111221),(#111222,#111223,#111224),(#111225,#111226,#111227),
(#111228,#111229,#111230)),.UNSPECIFIED.,.F.,.F.,.F.)
B_SPLINE_SURFACE_WITH_KNOTS((4,2,2,2,2,2,2,2,4),(3,3),(-2.7961087510372E-5,
0.000125253167969371,0.000156566459961714,0.000187879751954057,0.000203536397950228,
0.000211364720948314,0.000219193043946399,0.000234849689942571,0.000253195388096718),
(-0.00314610977256982,1.),.UNSPECIFIED.)
GEOMETRIC_REPRESENTATION_ITEM()
RATIONAL_B_SPLINE_SURFACE(((1.00189744483732,0.698445862592752,0.999999999999999),
(1.00180054146104,0.713846370407033,1.),(1.00176549021876,0.71941693927029,
1.),(1.00143621720098,0.771747125052584,1.),(1.00136903527042,0.78242410955385,
1.),(1.00119077538531,0.810754317015277,1.),(1.00108365364397,0.827778793126865,
1.),(1.000826467739,0.868652431296581,1.),(1.00072318361758,0.885067008168526,
1.),(1.00051234004795,0.9185756243445,1.),(1.00042818276658,0.931950440776531,
1.),(1.00027855551347,0.95573016620407,1.),(1.00022798737599,0.963766779853886,
1.),(1.00021763222241,0.965412487461147,1.),(1.000315025687,0.949934091660343,
1.),(1.00046861400987,0.925524847549985,1.),(1.0005506436245,0.912488173602062,
1.),(1.00062456604607,0.900739946914099,1.)))
REPRESENTATION_ITEM('')
SURFACE()
) ;
#449=(
BOUNDED_SURFACE()
B_SPLINE_SURFACE(3,2,((#111233,#111234,#111235),(#111236,#111237,#111238),
(#111239,#111240,#111241),(#111242,#111243,#111244)),.UNSPECIFIED.,.F.,
 .F.,.F.)
B_SPLINE_SURFACE_WITH_KNOTS((4,4),(3,3),(-1.77635683940025E-15,1.00173611575493),
(0.800638603120408,1.),.UNSPECIFIED.)
GEOMETRIC_REPRESENTATION_ITEM()
RATIONAL_B_SPLINE_SURFACE(((0.931056261594765,0.956944532691446,1.),(0.931106613485821,
0.956975977522397,1.),(0.92696606964625,0.954390201728278,1.),(0.920044734228406,
0.950067817452234,1.)))
REPRESENTATION_ITEM('')
SURFACE()
) ;
#450=(
BOUNDED_SURFACE()
B_SPLINE_SURFACE(3,2,((#111270,#111271,#111272),(#111273,#111274,#111275),
(#111276,#111277,#111278),(#111279,#111280,#111281)),.UNSPECIFIED.,.F.,
 .F.,.F.)
B_SPLINE_SURFACE_WITH_KNOTS((4,4),(3,3),(7.18283939271647E-15,1.08063632538888),
(0.,1.),.UNSPECIFIED.)
GEOMETRIC_REPRESENTATION_ITEM()
RATIONAL_B_SPLINE_SURFACE(((1.,0.821344978643199,1.),(1.,0.821618737292293,
1.),(1.,0.799663084581839,1.),(1.,0.763019982472728,1.)))
REPRESENTATION_ITEM('')
SURFACE()
) ;
#451=(
BOUNDED_SURFACE()
B_SPLINE_SURFACE(3,2,((#112748,#112749,#112750),(#112751,#112752,#112753),
(#112754,#112755,#112756),(#112757,#112758,#112759),(#112760,#112761,#112762),
(#112763,#112764,#112765)),.UNSPECIFIED.,.F.,.F.,.F.)
B_SPLINE_SURFACE_WITH_KNOTS((4,2,4),(3,3),(9.07204043127144E-5,0.000289236237441533,
0.000487752070570316),(-0.000844756555295823,1.00064307855252),
 .UNSPECIFIED.)
GEOMETRIC_REPRESENTATION_ITEM()
RATIONAL_B_SPLINE_SURFACE(((1.00067853369511,0.598126578822019,1.00051643581306),
(1.00070177595137,0.58436094698614,1.00053412562506),(1.0006649874303,0.606149590529623,
1.00050612567471),(1.00056632625566,0.664583392836423,1.00043103409956),
(1.00050548323092,0.700618735924398,1.00038472613112),(1.00047271456507,
0.720026550084235,1.00035978571517)))
REPRESENTATION_ITEM('')
SURFACE()
) ;
#452=(
BOUNDED_SURFACE()
B_SPLINE_SURFACE(3,2,((#112780,#112781,#112782),(#112783,#112784,#112785),
(#112786,#112787,#112788),(#112789,#112790,#112791),(#112792,#112793,#112794),
(#112795,#112796,#112797)),.UNSPECIFIED.,.F.,.F.,.F.)
B_SPLINE_SURFACE_WITH_KNOTS((4,2,4),(3,3),(0.000107162911540599,0.000298022515767417,
0.000488882119994238),(-0.000759939855676642,1.00062534339577),
 .UNSPECIFIED.)
GEOMETRIC_REPRESENTATION_ITEM()
RATIONAL_B_SPLINE_SURFACE(((1.00042862573102,0.717810580914605,1.00035266240945),
(1.00045905072599,0.697780025035077,1.00037769532572),(1.00051114946331,
0.663480375353483,1.00042056084895),(1.00059665225221,0.607188882365318,
1.00049091038088),(1.00062840114515,0.586286726926443,1.00051703256691),
(1.00061268510757,0.596633514797456,1.00050410180872)))
REPRESENTATION_ITEM('')
SURFACE()
) ;
#453=(
BOUNDED_SURFACE()
B_SPLINE_SURFACE(3,2,((#113027,#113028,#113029),(#113030,#113031,#113032),
(#113033,#113034,#113035),(#113036,#113037,#113038),(#113039,#113040,#113041),
(#113042,#113043,#113044),(#113045,#113046,#113047),(#113048,#113049,#113050)),
 .UNSPECIFIED.,.F.,.F.,.F.)
B_SPLINE_SURFACE_WITH_KNOTS((4,2,2,4),(3,3),(6.28318530717959,6.67588438887831,
7.06858347057703,7.85398163397448),(0.,1.),.UNSPECIFIED.)
GEOMETRIC_REPRESENTATION_ITEM()
RATIONAL_B_SPLINE_SURFACE(((1.,0.707106781186548,1.),(1.,0.706675310150436,
1.),(1.,0.726552333979984,1.),(1.,0.787677905717219,1.),(1.,0.828238301901734,
1.),(1.,0.94159960754984,1.),(1.,1.00267605951742,1.),(1.,1.,1.)))
REPRESENTATION_ITEM('')
SURFACE()
) ;
#454=(
BOUNDED_SURFACE()
B_SPLINE_SURFACE(3,2,((#113058,#113059,#113060),(#113061,#113062,#113063),
(#113064,#113065,#113066),(#113067,#113068,#113069),(#113070,#113071,#113072),
(#113073,#113074,#113075),(#113076,#113077,#113078),(#113079,#113080,#113081)),
 .UNSPECIFIED.,.F.,.F.,.F.)
B_SPLINE_SURFACE_WITH_KNOTS((4,2,2,4),(3,3),(4.71238898038469,5.49778714378214,
5.89048622548086,6.28318530717959),(0.,1.),.UNSPECIFIED.)
GEOMETRIC_REPRESENTATION_ITEM()
RATIONAL_B_SPLINE_SURFACE(((1.,1.,1.),(1.,1.0026760595174,1.),(1.,0.94159960754987,
1.),(1.,0.828238301901727,1.),(1.,0.787677905717213,1.),(1.,0.726552333979991,
1.),(1.,0.706675310150431,1.),(1.,0.707106781186548,1.)))
REPRESENTATION_ITEM('')
SURFACE()
) ;
#455=(
BOUNDED_SURFACE()
B_SPLINE_SURFACE(3,2,((#113082,#113083,#113084),(#113085,#113086,#113087),
(#113088,#113089,#113090),(#113091,#113092,#113093),(#113094,#113095,#113096),
(#113097,#113098,#113099),(#113100,#113101,#113102),(#113103,#113104,#113105)),
 .UNSPECIFIED.,.F.,.F.,.F.)
B_SPLINE_SURFACE_WITH_KNOTS((4,2,2,4),(3,3),(4.71238898038469,5.49778714378214,
5.89048622548086,6.28318530717959),(0.,1.),.UNSPECIFIED.)
GEOMETRIC_REPRESENTATION_ITEM()
RATIONAL_B_SPLINE_SURFACE(((1.,1.,1.),(1.,1.0026760595174,1.),(1.,0.94159960754987,
1.),(1.,0.828238301901727,1.),(1.,0.787677905717213,1.),(1.,0.726552333979991,
1.),(1.,0.706675310150431,1.),(1.,0.707106781186548,1.)))
REPRESENTATION_ITEM('')
SURFACE()
) ;
#456=(
BOUNDED_SURFACE()
B_SPLINE_SURFACE(3,2,((#113113,#113114,#113115),(#113116,#113117,#113118),
(#113119,#113120,#113121),(#113122,#113123,#113124),(#113125,#113126,#113127),
(#113128,#113129,#113130),(#113131,#113132,#113133),(#113134,#113135,#113136)),
 .UNSPECIFIED.,.F.,.F.,.F.)
B_SPLINE_SURFACE_WITH_KNOTS((4,2,2,4),(3,3),(6.28318530717959,6.67588438887831,
7.06858347057703,7.85398163397448),(0.,1.),.UNSPECIFIED.)
GEOMETRIC_REPRESENTATION_ITEM()
RATIONAL_B_SPLINE_SURFACE(((1.,0.707106781186548,1.),(1.,0.706675310150436,
1.),(1.,0.726552333979984,1.),(1.,0.787677905717219,1.),(1.,0.828238301901734,
1.),(1.,0.94159960754984,1.),(1.,1.00267605951742,1.),(1.,1.,1.)))
REPRESENTATION_ITEM('')
SURFACE()
) ;
#457=(
BOUNDED_SURFACE()
B_SPLINE_SURFACE(3,2,((#113137,#113138,#113139),(#113140,#113141,#113142),
(#113143,#113144,#113145),(#113146,#113147,#113148),(#113149,#113150,#113151),
(#113152,#113153,#113154)),.UNSPECIFIED.,.F.,.F.,.F.)
B_SPLINE_SURFACE_WITH_KNOTS((4,2,4),(3,3),(2.06095632820092,2.92811730964759,
3.79527829109427),(0.,1.),.UNSPECIFIED.)
GEOMETRIC_REPRESENTATION_ITEM()
RATIONAL_B_SPLINE_SURFACE(((1.,0.763019982472728,1.),(1.,0.792403856906318,
1.),(1.,0.812400188579283,1.),(1.,0.825457041221101,1.),(1.,0.818529518851208,
1.),(1.,0.799131938862211,1.)))
REPRESENTATION_ITEM('')
SURFACE()
) ;
#458=(
BOUNDED_SURFACE()
B_SPLINE_SURFACE(3,2,((#113177,#113178,#113179),(#113180,#113181,#113182),
(#113183,#113184,#113185),(#113186,#113187,#113188),(#113189,#113190,#113191),
(#113192,#113193,#113194)),.UNSPECIFIED.,.F.,.F.,.F.)
B_SPLINE_SURFACE_WITH_KNOTS((4,2,4),(3,3),(2.13522523980989,3.02435044878099,
3.9134756577521),(0.,1.),.UNSPECIFIED.)
GEOMETRIC_REPRESENTATION_ITEM()
RATIONAL_B_SPLINE_SURFACE(((1.,0.749240327740277,1.),(1.,0.768579562596332,
1.),(1.,0.780993049743038,1.),(1.,0.78606840104591,1.),(1.,0.778729916329044,
1.),(1.,0.763019982472728,1.)))
REPRESENTATION_ITEM('')
SURFACE()
) ;
#459=(
BOUNDED_SURFACE()
B_SPLINE_SURFACE(3,2,((#113351,#113352,#113353),(#113354,#113355,#113356),
(#113357,#113358,#113359),(#113360,#113361,#113362),(#113363,#113364,#113365),
(#113366,#113367,#113368),(#113369,#113370,#113371),(#113372,#113373,#113374),
(#113375,#113376,#113377),(#113378,#113379,#113380),(#113381,#113382,#113383),
(#113384,#113385,#113386),(#113387,#113388,#113389),(#113390,#113391,#113392),
(#113393,#113394,#113395),(#113396,#113397,#113398),(#113399,#113400,#113401),
(#113402,#113403,#113404)),.UNSPECIFIED.,.F.,.F.,.F.)
B_SPLINE_SURFACE_WITH_KNOTS((4,2,2,2,2,2,2,2,4),(3,3),(-2.88136898044833E-5,
0.000144068449022426,0.000180085561278032,0.000216102673533639,0.000234111229661442,
0.000243115507725343,0.000252119785789245,0.000270128341917048,0.000315232069288961),
(-0.00230043332395591,1.00649231299463),.UNSPECIFIED.)
GEOMETRIC_REPRESENTATION_ITEM()
RATIONAL_B_SPLINE_SURFACE(((1.00137797387149,0.698547958833521,1.00390520040663),
(1.00130996746152,0.713425360736431,1.00371246913257),(1.00133921304082,
0.707027460343038,1.00379535158087),(1.00112343332558,0.754232445100804,
1.00318382835165),(1.00107694244925,0.764403007732903,1.00305207245053),
(1.00092854904652,0.79686624602385,1.00263152312904),(1.00083723042784,
0.816843536281434,1.00237272467562),(1.00052495197535,0.885159038383718,
1.00148772245252),(1.00036238583123,0.920722772198024,1.00102700735099),
(1.00013066612433,0.971414864457828,1.00037030992562),(1.00008161134639,
0.982146318257254,1.00023128788557),(1.00010185218186,0.977718337948389,
1.00028865074314),(1.00015066464697,0.967039893644187,1.00042698606467),
(1.00027150756269,0.940603729390212,1.00076945685701),(1.0003534954887,
0.922667665317993,1.00100181197539),(1.00060974665141,0.866608956479265,
1.00172803194625),(1.00075148156376,0.835602360842176,1.00212971099749),
(1.00085165739571,0.813687424976746,1.00241361093766)))
REPRESENTATION_ITEM('')
SURFACE()
) ;
#460=(
BOUNDED_SURFACE()
B_SPLINE_SURFACE(3,2,((#113406,#113407,#113408),(#113409,#113410,#113411),
(#113412,#113413,#113414),(#113415,#113416,#113417)),.UNSPECIFIED.,.F.,
 .F.,.F.)
B_SPLINE_SURFACE_WITH_KNOTS((4,4),(3,3),(5.63598348762743,6.28318530717959),
(0.792338840560947,1.),.UNSPECIFIED.)
GEOMETRIC_REPRESENTATION_ITEM()
RATIONAL_B_SPLINE_SURFACE(((0.934040253948338,0.958376553896459,1.),(0.938725627259262,
0.961333226642431,1.),(0.941220250254377,0.962907441402211,1.),(0.941208919370362,
0.962900291125438,1.)))
REPRESENTATION_ITEM('')
SURFACE()
) ;
#461=(
BOUNDED_SURFACE()
B_SPLINE_SURFACE(3,2,((#113458,#113459,#113460),(#113461,#113462,#113463),
(#113464,#113465,#113466),(#113467,#113468,#113469),(#113470,#113471,#113472),
(#113473,#113474,#113475),(#113476,#113477,#113478),(#113479,#113480,#113481),
(#113482,#113483,#113484),(#113485,#113486,#113487),(#113488,#113489,#113490),
(#113491,#113492,#113493),(#113494,#113495,#113496),(#113497,#113498,#113499),
(#113500,#113501,#113502),(#113503,#113504,#113505),(#113506,#113507,#113508),
(#113509,#113510,#113511)),.UNSPECIFIED.,.F.,.F.,.F.)
B_SPLINE_SURFACE_WITH_KNOTS((4,2,2,2,2,2,2,2,4),(3,3),(-3.19743590575723E-5,
0.000144068449022591,0.000180085561278238,0.000216102673533885,0.000234111229661708,
0.00024311550772562,0.000252119785789532,0.000270128341917355,0.000288136898045179),
(-0.0066834189728382,1.00019683226058),.UNSPECIFIED.)
GEOMETRIC_REPRESENTATION_ITEM()
RATIONAL_B_SPLINE_SURFACE(((1.00403209003411,0.69829147589406,1.00011798325497),
(1.00381915098325,0.714225030505723,1.00011175243122),(1.0039173389525,
0.706877935813847,1.00011462551593),(1.0032781689847,0.754704999695571,
1.00009592272094),(1.00314250899902,0.764856006670268,1.00009195316507),
(1.00270949829933,0.797256825605796,1.00007928281015),(1.00244303133891,
0.817195704120733,1.00007148570268),(1.00153180544395,0.885379851192955,
1.00004482226109),(1.00105743880421,0.920875204111829,1.00003094178726),
(1.00038128265055,0.971469827113733,1.00001115673703),(1.00023814122159,
0.982180646789395,1.00000696826614),(1.00029720380909,0.977761180469183,
1.00000869650045),(1.00043963817126,0.967103268362262,1.0000128642818),
(1.00079225678183,0.940717934783944,1.00002318227845),(1.00103149685961,
0.922816357645932,1.00003018269829),(1.00145821870309,0.890886113898687,
1.00004266903457),(1.00165232267988,0.876361928212012,1.00004834872396),
(1.00182713963613,0.863280929173305,1.00005346405456)))
REPRESENTATION_ITEM('')
SURFACE()
) ;
#462=(
BOUNDED_SURFACE()
B_SPLINE_SURFACE(3,2,((#113550,#113551,#113552),(#113553,#113554,#113555),
(#113556,#113557,#113558),(#113559,#113560,#113561)),.UNSPECIFIED.,.F.,
 .F.,.F.)
B_SPLINE_SURFACE_WITH_KNOTS((4,4),(3,3),(5.51130230301728,6.28318530717958),
(0.,1.),.UNSPECIFIED.)
GEOMETRIC_REPRESENTATION_ITEM()
RATIONAL_B_SPLINE_SURFACE(((1.,0.763019982472728,1.),(1.,0.776565014072567,
1.),(1.,0.784088758369131,1.),(1.,0.784033077704815,1.)))
REPRESENTATION_ITEM('')
SURFACE()
) ;
#463=(
BOUNDED_SURFACE()
B_SPLINE_SURFACE(3,2,((#113566,#113567,#113568),(#113569,#113570,#113571),
(#113572,#113573,#113574),(#113575,#113576,#113577)),.UNSPECIFIED.,.F.,
 .F.,.F.)
B_SPLINE_SURFACE_WITH_KNOTS((4,4),(3,3),(0.0051446850272488,0.00657473287039649),
(0.,1.),.UNSPECIFIED.)
GEOMETRIC_REPRESENTATION_ITEM()
RATIONAL_B_SPLINE_SURFACE(((1.,0.943476662524759,1.),(1.,0.944945702024751,
1.),(1.,0.946300916277093,1.),(1.,0.947565352018496,1.)))
REPRESENTATION_ITEM('')
SURFACE()
) ;
#464=(
BOUNDED_SURFACE()
B_SPLINE_SURFACE(3,2,((#113616,#113617,#113618),(#113619,#113620,#113621),
(#113622,#113623,#113624),(#113625,#113626,#113627)),.UNSPECIFIED.,.F.,
 .F.,.F.)
B_SPLINE_SURFACE_WITH_KNOTS((4,4),(3,3),(0.0051446850272488,0.00657473287039648),
(0.,1.),.UNSPECIFIED.)
GEOMETRIC_REPRESENTATION_ITEM()
RATIONAL_B_SPLINE_SURFACE(((1.,0.94347666252476,1.),(1.,0.94494570202475,
1.),(1.,0.946300916277093,1.),(1.,0.947565352018496,1.)))
REPRESENTATION_ITEM('')
SURFACE()
) ;
#465=(
BOUNDED_SURFACE()
B_SPLINE_SURFACE(3,2,((#113632,#113633,#113634),(#113635,#113636,#113637),
(#113638,#113639,#113640),(#113641,#113642,#113643),(#113644,#113645,#113646),
(#113647,#113648,#113649),(#113650,#113651,#113652),(#113653,#113654,#113655),
(#113656,#113657,#113658),(#113659,#113660,#113661),(#113662,#113663,#113664),
(#113665,#113666,#113667),(#113668,#113669,#113670),(#113671,#113672,#113673),
(#113674,#113675,#113676),(#113677,#113678,#113679),(#113680,#113681,#113682),
(#113683,#113684,#113685)),.UNSPECIFIED.,.F.,.F.,.F.)
B_SPLINE_SURFACE_WITH_KNOTS((4,2,2,2,2,2,2,2,4),(3,3),(-2.77591379149701E-5,
0.000125253167969375,0.000156566459961718,0.000187879751954062,0.000203536397950234,
0.00021136472094832,0.000219193043946406,0.000234849689942578,0.00025050633593875),
(0.,1.00287807885242),.UNSPECIFIED.)
GEOMETRIC_REPRESENTATION_ITEM()
RATIONAL_B_SPLINE_SURFACE(((1.,0.698587265143979,1.00173497923608),(1.,
0.713937574732811,1.00164662043326),(1.,0.719549163949031,1.00161431924076),
(1.,0.771808112009055,1.00131350849424),(1.,0.782482243723506,1.00125206650873),
(1.,0.810804881628005,1.00108903693833),(1.,0.827824808964385,1.00099106755246),
(1.,0.868687526094324,1.00075585530841),(1.,0.885097717150309,1.00066139566073),
(1.,0.91859738014868,1.00046856631745),(1.,0.931968622959436,1.00039159933512),
(1.,0.955741994674629,1.00025475605835),(1.,0.963776461019212,1.000208508403),
(1.,0.965421728909353,1.00019903798156),(1.,0.949947468785925,1.00028811026319),
(1.,0.927474619202907,1.00041746752947),(1.,0.916335140210081,1.0004815881273),
(1.,0.906010523700247,1.00054101824818)))
REPRESENTATION_ITEM('')
SURFACE()
) ;
#466=(
BOUNDED_SURFACE()
B_SPLINE_SURFACE(3,2,((#113689,#113690,#113691),(#113692,#113693,#113694),
(#113695,#113696,#113697),(#113698,#113699,#113700),(#113701,#113702,#113703),
(#113704,#113705,#113706),(#113707,#113708,#113709),(#113710,#113711,#113712),
(#113713,#113714,#113715),(#113716,#113717,#113718),(#113719,#113720,#113721),
(#113722,#113723,#113724),(#113725,#113726,#113727),(#113728,#113729,#113730),
(#113731,#113732,#113733),(#113734,#113735,#113736),(#113737,#113738,#113739),
(#113740,#113741,#113742)),.UNSPECIFIED.,.F.,.F.,.F.)
B_SPLINE_SURFACE_WITH_KNOTS((4,2,2,2,2,2,2,2,4),(3,3),(-2.79610875104704E-5,
0.000125253167969371,0.000156566459961714,0.000187879751954057,0.000203536397950228,
0.000211364720948314,0.000219193043946399,0.000234849689942571,0.000253195388096719),
(-0.00314610977255892,1.),.UNSPECIFIED.)
GEOMETRIC_REPRESENTATION_ITEM()
RATIONAL_B_SPLINE_SURFACE(((1.00189744483731,0.698445862592619,1.),(1.00180054146103,
0.713846370407217,1.),(1.00176549021876,0.719416939270132,1.),(1.00143621720097,
0.771747125052614,1.),(1.00136903527041,0.782424109553879,1.),(1.00119077538531,
0.810754317015252,1.),(1.00108365364397,0.827778793126867,1.),(1.000826467739,
0.868652431296582,1.),(1.00072318361758,0.885067008168527,1.),(1.00051234004795,
0.918575624344501,1.),(1.00042818276658,0.931950440776532,1.),(1.00027855551347,
0.955730166204071,1.),(1.00022798737599,0.963766779853886,1.),(1.00021763222241,
0.965412487461148,1.),(1.000315025687,0.949934091660343,1.),(1.00046861400987,
0.925524847549986,1.),(1.0005506436245,0.912488173602064,1.),(1.00062456604607,
0.900739946914099,1.)))
REPRESENTATION_ITEM('')
SURFACE()
) ;
#470=SHAPE_REPRESENTATION_RELATIONSHIP('SRR','None',#126600,#476) ;
#476=ADVANCED_BREP_SHAPE_REPRESENTATION('',(#4173,#4174,#4175,#4176,#4177),
#126566) ;
#482=STYLED_ITEM('',(#126640),#63895) ;
#483=STYLED_ITEM('',(#126640),#63896) ;
#484=STYLED_ITEM('',(#126640),#63897) ;
#485=STYLED_ITEM('',(#126640),#63898) ;
#486=STYLED_ITEM('',(#126640),#63899) ;
#487=STYLED_ITEM('',(#126640),#63900) ;
#488=STYLED_ITEM('',(#126640),#63901) ;
#489=STYLED_ITEM('',(#126640),#63902) ;
#490=STYLED_ITEM('',(#126640),#63903) ;
#491=STYLED_ITEM('',(#126640),#63904) ;
#492=STYLED_ITEM('',(#126640),#63905) ;
#493=STYLED_ITEM('',(#126640),#63906) ;
#494=STYLED_ITEM('',(#126640),#63907) ;
#495=STYLED_ITEM('',(#126640),#63908) ;
#496=STYLED_ITEM('',(#126640),#63909) ;
#497=STYLED_ITEM('',(#126640),#63910) ;
#498=STYLED_ITEM('',(#126640),#63911) ;
#499=STYLED_ITEM('',(#126640),#63912) ;
#500=STYLED_ITEM('',(#126640),#63913) ;
#501=STYLED_ITEM('',(#126640),#63914) ;
#502=STYLED_ITEM('',(#126640),#63915) ;
#503=STYLED_ITEM('',(#126640),#63916) ;
#504=STYLED_ITEM('',(#126640),#63917) ;
#505=STYLED_ITEM('',(#126640),#63918) ;
#506=STYLED_ITEM('',(#126640),#63919) ;
#507=STYLED_ITEM('',(#126640),#63920) ;
#508=STYLED_ITEM('',(#126640),#63921) ;
#509=STYLED_ITEM('',(#126640),#63922) ;
#510=STYLED_ITEM('',(#126640),#63923) ;
#511=STYLED_ITEM('',(#126640),#63924) ;
#512=STYLED_ITEM('',(#126640),#63925) ;
#513=STYLED_ITEM('',(#126640),#63926) ;
#514=STYLED_ITEM('',(#126640),#63927) ;
#515=STYLED_ITEM('',(#126640),#63928) ;
#516=STYLED_ITEM('',(#126640),#63929) ;
#517=STYLED_ITEM('',(#126640),#63930) ;
#518=STYLED_ITEM('',(#126640),#63931) ;
#519=STYLED_ITEM('',(#126640),#63932) ;
#520=STYLED_ITEM('',(#126640),#63933) ;
#521=STYLED_ITEM('',(#126640),#63934) ;
#522=STYLED_ITEM('',(#126640),#63935) ;
#523=STYLED_ITEM('',(#126640),#63936) ;
#524=STYLED_ITEM('',(#126640),#63937) ;
#525=STYLED_ITEM('',(#126640),#63938) ;
#526=STYLED_ITEM('',(#126640),#63939) ;
#527=STYLED_ITEM('',(#126640),#63940) ;
#528=STYLED_ITEM('',(#126640),#63941) ;
#529=STYLED_ITEM('',(#126640),#63942) ;
#530=STYLED_ITEM('',(#126640),#63943) ;
#531=STYLED_ITEM('',(#126640),#63944) ;
#532=STYLED_ITEM('',(#126640),#63945) ;
#533=STYLED_ITEM('',(#126640),#63946) ;
#534=STYLED_ITEM('',(#126640),#63947) ;
#535=STYLED_ITEM('',(#126640),#63948) ;
#536=STYLED_ITEM('',(#126640),#63949) ;
#537=STYLED_ITEM('',(#126640),#63950) ;
#538=STYLED_ITEM('',(#126641),#63951) ;
#539=STYLED_ITEM('',(#126641),#63952) ;
#540=STYLED_ITEM('',(#126641),#63953) ;
#541=STYLED_ITEM('',(#126641),#63954) ;
#542=STYLED_ITEM('',(#126641),#63955) ;
#543=STYLED_ITEM('',(#126641),#63956) ;
#544=STYLED_ITEM('',(#126641),#63957) ;
#545=STYLED_ITEM('',(#126641),#63958) ;
#546=STYLED_ITEM('',(#126641),#63959) ;
#547=STYLED_ITEM('',(#126641),#63960) ;
#548=STYLED_ITEM('',(#126641),#63961) ;
#549=STYLED_ITEM('',(#126641),#63962) ;
#550=STYLED_ITEM('',(#126641),#63963) ;
#551=STYLED_ITEM('',(#126641),#63964) ;
#552=STYLED_ITEM('',(#126641),#63965) ;
#553=STYLED_ITEM('',(#126641),#63966) ;
#554=STYLED_ITEM('',(#126641),#63967) ;
#555=STYLED_ITEM('',(#126641),#63968) ;
#556=STYLED_ITEM('',(#126641),#63969) ;
#557=STYLED_ITEM('',(#126641),#63970) ;
#558=STYLED_ITEM('',(#126640),#63971) ;
#559=STYLED_ITEM('',(#126640),#63972) ;
#560=STYLED_ITEM('',(#126640),#63973) ;
#561=STYLED_ITEM('',(#126640),#63974) ;
#562=STYLED_ITEM('',(#126640),#63975) ;
#563=STYLED_ITEM('',(#126640),#63976) ;
#564=STYLED_ITEM('',(#126640),#63977) ;
#565=STYLED_ITEM('',(#126640),#63978) ;
#566=STYLED_ITEM('',(#126640),#63979) ;
#567=STYLED_ITEM('',(#126640),#63980) ;
#568=STYLED_ITEM('',(#126640),#63981) ;
#569=STYLED_ITEM('',(#126640),#63982) ;
#570=STYLED_ITEM('',(#126640),#63983) ;
#571=STYLED_ITEM('',(#126640),#63984) ;
#572=STYLED_ITEM('',(#126640),#63985) ;
#573=STYLED_ITEM('',(#126640),#63986) ;
#574=STYLED_ITEM('',(#126640),#63987) ;
#575=STYLED_ITEM('',(#126640),#63988) ;
#576=STYLED_ITEM('',(#126640),#63989) ;
#577=STYLED_ITEM('',(#126640),#63990) ;
#578=STYLED_ITEM('',(#126640),#63991) ;
#579=STYLED_ITEM('',(#126640),#63992) ;
#580=STYLED_ITEM('',(#126640),#63993) ;
#581=STYLED_ITEM('',(#126640),#63994) ;
#582=STYLED_ITEM('',(#126640),#63995) ;
#583=STYLED_ITEM('',(#126640),#63996) ;
#584=STYLED_ITEM('',(#126640),#63997) ;
#585=STYLED_ITEM('',(#126640),#63998) ;
#586=STYLED_ITEM('',(#126640),#63999) ;
#587=STYLED_ITEM('',(#126640),#64000) ;
#588=STYLED_ITEM('',(#126640),#64001) ;
#589=STYLED_ITEM('',(#126640),#64002) ;
#590=STYLED_ITEM('',(#126640),#64003) ;
#591=STYLED_ITEM('',(#126640),#64004) ;
#592=STYLED_ITEM('',(#126640),#64005) ;
#593=STYLED_ITEM('',(#126640),#64006) ;
#594=STYLED_ITEM('',(#126640),#64007) ;
#595=STYLED_ITEM('',(#126640),#64008) ;
#596=STYLED_ITEM('',(#126640),#64009) ;
#597=STYLED_ITEM('',(#126640),#64010) ;
#598=STYLED_ITEM('',(#126640),#64011) ;
#599=STYLED_ITEM('',(#126640),#64012) ;
#600=STYLED_ITEM('',(#126640),#64013) ;
#601=STYLED_ITEM('',(#126640),#64014) ;
#602=STYLED_ITEM('',(#126640),#64015) ;
#603=STYLED_ITEM('',(#126640),#64016) ;
#604=STYLED_ITEM('',(#126640),#64017) ;
#605=STYLED_ITEM('',(#126640),#64018) ;
#606=STYLED_ITEM('',(#126640),#64019) ;
#607=STYLED_ITEM('',(#126640),#64020) ;
#608=STYLED_ITEM('',(#126640),#64021) ;
#609=STYLED_ITEM('',(#126640),#64022) ;
#610=STYLED_ITEM('',(#126640),#64023) ;
#611=STYLED_ITEM('',(#126640),#64024) ;
#612=STYLED_ITEM('',(#126640),#64025) ;
#613=STYLED_ITEM('',(#126640),#64026) ;
#614=STYLED_ITEM('',(#126640),#64027) ;
#615=STYLED_ITEM('',(#126640),#64028) ;
#616=STYLED_ITEM('',(#126640),#64029) ;
#617=STYLED_ITEM('',(#126640),#64030) ;
#618=STYLED_ITEM('',(#126640),#64031) ;
#619=STYLED_ITEM('',(#126640),#64032) ;
#620=STYLED_ITEM('',(#126640),#64033) ;
#621=STYLED_ITEM('',(#126640),#64034) ;
#622=STYLED_ITEM('',(#126640),#64035) ;
#623=STYLED_ITEM('',(#126640),#64036) ;
#624=STYLED_ITEM('',(#126640),#64037) ;
#625=STYLED_ITEM('',(#126640),#64038) ;
#626=STYLED_ITEM('',(#126640),#64039) ;
#627=STYLED_ITEM('',(#126640),#64040) ;
#628=STYLED_ITEM('',(#126640),#64041) ;
#629=STYLED_ITEM('',(#126640),#64042) ;
#630=STYLED_ITEM('',(#126640),#64043) ;
#631=STYLED_ITEM('',(#126640),#64044) ;
#632=STYLED_ITEM('',(#126640),#64045) ;
#633=STYLED_ITEM('',(#126640),#64046) ;
#634=STYLED_ITEM('',(#126640),#64047) ;
#635=STYLED_ITEM('',(#126640),#64048) ;
#636=STYLED_ITEM('',(#126640),#64049) ;
#637=STYLED_ITEM('',(#126640),#64050) ;
#638=STYLED_ITEM('',(#126640),#64051) ;
#639=STYLED_ITEM('',(#126640),#64052) ;
#640=STYLED_ITEM('',(#126640),#64053) ;
#641=STYLED_ITEM('',(#126640),#64054) ;
#642=STYLED_ITEM('',(#126640),#64055) ;
#643=STYLED_ITEM('',(#126640),#64056) ;
#644=STYLED_ITEM('',(#126640),#64057) ;
#645=STYLED_ITEM('',(#126640),#64058) ;
#646=STYLED_ITEM('',(#126640),#64059) ;
#647=STYLED_ITEM('',(#126640),#64060) ;
#648=STYLED_ITEM('',(#126640),#64061) ;
#649=STYLED_ITEM('',(#126640),#64062) ;
#650=STYLED_ITEM('',(#126640),#64063) ;
#651=STYLED_ITEM('',(#126640),#64064) ;
#652=STYLED_ITEM('',(#126640),#64065) ;
#653=STYLED_ITEM('',(#126640),#64066) ;
#654=STYLED_ITEM('',(#126640),#64067) ;
#655=STYLED_ITEM('',(#126640),#64068) ;
#656=STYLED_ITEM('',(#126640),#64069) ;
#657=STYLED_ITEM('',(#126640),#64070) ;
#658=STYLED_ITEM('',(#126640),#64071) ;
#659=STYLED_ITEM('',(#126640),#64072) ;
#660=STYLED_ITEM('',(#126640),#64073) ;
#661=STYLED_ITEM('',(#126640),#64074) ;
#662=STYLED_ITEM('',(#126640),#64075) ;
#663=STYLED_ITEM('',(#126641),#64076) ;
#664=STYLED_ITEM('',(#126641),#64077) ;
#665=STYLED_ITEM('',(#126641),#64078) ;
#666=STYLED_ITEM('',(#126641),#64079) ;
#667=STYLED_ITEM('',(#126641),#64080) ;
#668=STYLED_ITEM('',(#126641),#64081) ;
#669=STYLED_ITEM('',(#126641),#64082) ;
#670=STYLED_ITEM('',(#126641),#64083) ;
#671=STYLED_ITEM('',(#126641),#64084) ;
#672=STYLED_ITEM('',(#126641),#64085) ;
#673=STYLED_ITEM('',(#126641),#64086) ;
#674=STYLED_ITEM('',(#126641),#64087) ;
#675=STYLED_ITEM('',(#126641),#64088) ;
#676=STYLED_ITEM('',(#126641),#64089) ;
#677=STYLED_ITEM('',(#126641),#64090) ;
#678=STYLED_ITEM('',(#126641),#64091) ;
#679=STYLED_ITEM('',(#126641),#64092) ;
#680=STYLED_ITEM('',(#126641),#64093) ;
#681=STYLED_ITEM('',(#126641),#64094) ;
#682=STYLED_ITEM('',(#126641),#64095) ;
#683=STYLED_ITEM('',(#126641),#64096) ;
#684=STYLED_ITEM('',(#126641),#64097) ;
#685=STYLED_ITEM('',(#126641),#64098) ;
#686=STYLED_ITEM('',(#126641),#64099) ;
#687=STYLED_ITEM('',(#126641),#64100) ;
#688=STYLED_ITEM('',(#126641),#64101) ;
#689=STYLED_ITEM('',(#126641),#64102) ;
#690=STYLED_ITEM('',(#126641),#64103) ;
#691=STYLED_ITEM('',(#126641),#64104) ;
#692=STYLED_ITEM('',(#126641),#64105) ;
#693=STYLED_ITEM('',(#126641),#64106) ;
#694=STYLED_ITEM('',(#126641),#64107) ;
#695=STYLED_ITEM('',(#126641),#64108) ;
#696=STYLED_ITEM('',(#126641),#64109) ;
#697=STYLED_ITEM('',(#126641),#64110) ;
#698=STYLED_ITEM('',(#126641),#64111) ;
#699=STYLED_ITEM('',(#126640),#64112) ;
#700=STYLED_ITEM('',(#126640),#64113) ;
#701=STYLED_ITEM('',(#126640),#64114) ;
#702=STYLED_ITEM('',(#126640),#64115) ;
#703=STYLED_ITEM('',(#126640),#64116) ;
#704=STYLED_ITEM('',(#126640),#64117) ;
#705=STYLED_ITEM('',(#126640),#64118) ;
#706=STYLED_ITEM('',(#126640),#64119) ;
#707=STYLED_ITEM('',(#126640),#64120) ;
#708=STYLED_ITEM('',(#126640),#64121) ;
#709=STYLED_ITEM('',(#126640),#64122) ;
#710=STYLED_ITEM('',(#126640),#64123) ;
#711=STYLED_ITEM('',(#126640),#64124) ;
#712=STYLED_ITEM('',(#126640),#64125) ;
#713=STYLED_ITEM('',(#126640),#64126) ;
#714=STYLED_ITEM('',(#126640),#64127) ;
#715=STYLED_ITEM('',(#126640),#64128) ;
#716=STYLED_ITEM('',(#126640),#64129) ;
#717=STYLED_ITEM('',(#126640),#64130) ;
#718=STYLED_ITEM('',(#126640),#64131) ;
#719=STYLED_ITEM('',(#126640),#64132) ;
#720=STYLED_ITEM('',(#126640),#64133) ;
#721=STYLED_ITEM('',(#126640),#64134) ;
#722=STYLED_ITEM('',(#126640),#64135) ;
#723=STYLED_ITEM('',(#126640),#64136) ;
#724=STYLED_ITEM('',(#126640),#64137) ;
#725=STYLED_ITEM('',(#126640),#64138) ;
#726=STYLED_ITEM('',(#126640),#64139) ;
#727=STYLED_ITEM('',(#126640),#64140) ;
#728=STYLED_ITEM('',(#126640),#64141) ;
#729=STYLED_ITEM('',(#126640),#64142) ;
#730=STYLED_ITEM('',(#126640),#64143) ;
#731=STYLED_ITEM('',(#126640),#64144) ;
#732=STYLED_ITEM('',(#126640),#64145) ;
#733=STYLED_ITEM('',(#126640),#64146) ;
#734=STYLED_ITEM('',(#126640),#64147) ;
#735=STYLED_ITEM('',(#126640),#64148) ;
#736=STYLED_ITEM('',(#126640),#64149) ;
#737=STYLED_ITEM('',(#126640),#64150) ;
#738=STYLED_ITEM('',(#126640),#64151) ;
#739=STYLED_ITEM('',(#126640),#64152) ;
#740=STYLED_ITEM('',(#126640),#64153) ;
#741=STYLED_ITEM('',(#126640),#64154) ;
#742=STYLED_ITEM('',(#126640),#64155) ;
#743=STYLED_ITEM('',(#126640),#64156) ;
#744=STYLED_ITEM('',(#126640),#64157) ;
#745=STYLED_ITEM('',(#126640),#64158) ;
#746=STYLED_ITEM('',(#126641),#64159) ;
#747=STYLED_ITEM('',(#126641),#64160) ;
#748=STYLED_ITEM('',(#126641),#64161) ;
#749=STYLED_ITEM('',(#126641),#64162) ;
#750=STYLED_ITEM('',(#126641),#64163) ;
#751=STYLED_ITEM('',(#126641),#64164) ;
#752=STYLED_ITEM('',(#126641),#64165) ;
#753=STYLED_ITEM('',(#126641),#64166) ;
#754=STYLED_ITEM('',(#126641),#64167) ;
#755=STYLED_ITEM('',(#126641),#64168) ;
#756=STYLED_ITEM('',(#126641),#64169) ;
#757=STYLED_ITEM('',(#126641),#64170) ;
#758=STYLED_ITEM('',(#126641),#64171) ;
#759=STYLED_ITEM('',(#126641),#64172) ;
#760=STYLED_ITEM('',(#126641),#64173) ;
#761=STYLED_ITEM('',(#126641),#64174) ;
#762=STYLED_ITEM('',(#126640),#64175) ;
#763=STYLED_ITEM('',(#126640),#64176) ;
#764=STYLED_ITEM('',(#126640),#64177) ;
#765=STYLED_ITEM('',(#126640),#64178) ;
#766=STYLED_ITEM('',(#126640),#64179) ;
#767=STYLED_ITEM('',(#126640),#64180) ;
#768=STYLED_ITEM('',(#126640),#64181) ;
#769=STYLED_ITEM('',(#126640),#64182) ;
#770=STYLED_ITEM('',(#126640),#64183) ;
#771=STYLED_ITEM('',(#126639),#4173) ;
#772=STYLED_ITEM('',(#126640),#64184) ;
#773=STYLED_ITEM('',(#126640),#64185) ;
#774=STYLED_ITEM('',(#126640),#64186) ;
#775=STYLED_ITEM('',(#126640),#64187) ;
#776=STYLED_ITEM('',(#126640),#64188) ;
#777=STYLED_ITEM('',(#126640),#64189) ;
#778=STYLED_ITEM('',(#126640),#64190) ;
#779=STYLED_ITEM('',(#126640),#64191) ;
#780=STYLED_ITEM('',(#126640),#64192) ;
#781=STYLED_ITEM('',(#126640),#64193) ;
#782=STYLED_ITEM('',(#126640),#64194) ;
#783=STYLED_ITEM('',(#126640),#64195) ;
#784=STYLED_ITEM('',(#126640),#64196) ;
#785=STYLED_ITEM('',(#126640),#64197) ;
#786=STYLED_ITEM('',(#126640),#64198) ;
#787=STYLED_ITEM('',(#126640),#64199) ;
#788=STYLED_ITEM('',(#126640),#64200) ;
#789=STYLED_ITEM('',(#126640),#64201) ;
#790=STYLED_ITEM('',(#126640),#64202) ;
#791=STYLED_ITEM('',(#126640),#64203) ;
#792=STYLED_ITEM('',(#126640),#64204) ;
#793=STYLED_ITEM('',(#126640),#64205) ;
#794=STYLED_ITEM('',(#126640),#64206) ;
#795=STYLED_ITEM('',(#126640),#64207) ;
#796=STYLED_ITEM('',(#126640),#64208) ;
#797=STYLED_ITEM('',(#126640),#64209) ;
#798=STYLED_ITEM('',(#126640),#64210) ;
#799=STYLED_ITEM('',(#126640),#64211) ;
#800=STYLED_ITEM('',(#126640),#64212) ;
#801=STYLED_ITEM('',(#126640),#64213) ;
#802=STYLED_ITEM('',(#126640),#64214) ;
#803=STYLED_ITEM('',(#126640),#64215) ;
#804=STYLED_ITEM('',(#126640),#64216) ;
#805=STYLED_ITEM('',(#126640),#64217) ;
#806=STYLED_ITEM('',(#126640),#64218) ;
#807=STYLED_ITEM('',(#126640),#64219) ;
#808=STYLED_ITEM('',(#126640),#64220) ;
#809=STYLED_ITEM('',(#126640),#64221) ;
#810=STYLED_ITEM('',(#126640),#64222) ;
#811=STYLED_ITEM('',(#126640),#64223) ;
#812=STYLED_ITEM('',(#126640),#64224) ;
#813=STYLED_ITEM('',(#126640),#64225) ;
#814=STYLED_ITEM('',(#126640),#64226) ;
#815=STYLED_ITEM('',(#126640),#64227) ;
#816=STYLED_ITEM('',(#126640),#64228) ;
#817=STYLED_ITEM('',(#126640),#64229) ;
#818=STYLED_ITEM('',(#126640),#64230) ;
#819=STYLED_ITEM('',(#126640),#64231) ;
#820=STYLED_ITEM('',(#126640),#64232) ;
#821=STYLED_ITEM('',(#126640),#64233) ;
#822=STYLED_ITEM('',(#126640),#64234) ;
#823=STYLED_ITEM('',(#126640),#64235) ;
#824=STYLED_ITEM('',(#126640),#64236) ;
#825=STYLED_ITEM('',(#126640),#64237) ;
#826=STYLED_ITEM('',(#126640),#64238) ;
#827=STYLED_ITEM('',(#126640),#64239) ;
#828=STYLED_ITEM('',(#126641),#64240) ;
#829=STYLED_ITEM('',(#126641),#64241) ;
#830=STYLED_ITEM('',(#126641),#64242) ;
#831=STYLED_ITEM('',(#126641),#64243) ;
#832=STYLED_ITEM('',(#126641),#64244) ;
#833=STYLED_ITEM('',(#126641),#64245) ;
#834=STYLED_ITEM('',(#126641),#64246) ;
#835=STYLED_ITEM('',(#126641),#64247) ;
#836=STYLED_ITEM('',(#126641),#64248) ;
#837=STYLED_ITEM('',(#126641),#64249) ;
#838=STYLED_ITEM('',(#126641),#64250) ;
#839=STYLED_ITEM('',(#126641),#64251) ;
#840=STYLED_ITEM('',(#126641),#64252) ;
#841=STYLED_ITEM('',(#126641),#64253) ;
#842=STYLED_ITEM('',(#126641),#64254) ;
#843=STYLED_ITEM('',(#126641),#64255) ;
#844=STYLED_ITEM('',(#126641),#64256) ;
#845=STYLED_ITEM('',(#126641),#64257) ;
#846=STYLED_ITEM('',(#126641),#64258) ;
#847=STYLED_ITEM('',(#126641),#64259) ;
#848=STYLED_ITEM('',(#126640),#64260) ;
#849=STYLED_ITEM('',(#126640),#64261) ;
#850=STYLED_ITEM('',(#126640),#64262) ;
#851=STYLED_ITEM('',(#126640),#64263) ;
#852=STYLED_ITEM('',(#126640),#64264) ;
#853=STYLED_ITEM('',(#126640),#64265) ;
#854=STYLED_ITEM('',(#126640),#64266) ;
#855=STYLED_ITEM('',(#126640),#64267) ;
#856=STYLED_ITEM('',(#126640),#64268) ;
#857=STYLED_ITEM('',(#126640),#64269) ;
#858=STYLED_ITEM('',(#126640),#64270) ;
#859=STYLED_ITEM('',(#126640),#64271) ;
#860=STYLED_ITEM('',(#126640),#64272) ;
#861=STYLED_ITEM('',(#126640),#64273) ;
#862=STYLED_ITEM('',(#126640),#64274) ;
#863=STYLED_ITEM('',(#126640),#64275) ;
#864=STYLED_ITEM('',(#126640),#64276) ;
#865=STYLED_ITEM('',(#126640),#64277) ;
#866=STYLED_ITEM('',(#126640),#64278) ;
#867=STYLED_ITEM('',(#126640),#64279) ;
#868=STYLED_ITEM('',(#126640),#64280) ;
#869=STYLED_ITEM('',(#126640),#64281) ;
#870=STYLED_ITEM('',(#126640),#64282) ;
#871=STYLED_ITEM('',(#126640),#64283) ;
#872=STYLED_ITEM('',(#126640),#64284) ;
#873=STYLED_ITEM('',(#126640),#64285) ;
#874=STYLED_ITEM('',(#126640),#64286) ;
#875=STYLED_ITEM('',(#126640),#64287) ;
#876=STYLED_ITEM('',(#126640),#64288) ;
#877=STYLED_ITEM('',(#126640),#64289) ;
#878=STYLED_ITEM('',(#126640),#64290) ;
#879=STYLED_ITEM('',(#126640),#64291) ;
#880=STYLED_ITEM('',(#126640),#64292) ;
#881=STYLED_ITEM('',(#126640),#64293) ;
#882=STYLED_ITEM('',(#126640),#64294) ;
#883=STYLED_ITEM('',(#126640),#64295) ;
#884=STYLED_ITEM('',(#126640),#64296) ;
#885=STYLED_ITEM('',(#126640),#64297) ;
#886=STYLED_ITEM('',(#126640),#64298) ;
#887=STYLED_ITEM('',(#126640),#64299) ;
#888=STYLED_ITEM('',(#126640),#64300) ;
#889=STYLED_ITEM('',(#126640),#64301) ;
#890=STYLED_ITEM('',(#126640),#64302) ;
#891=STYLED_ITEM('',(#126640),#64303) ;
#892=STYLED_ITEM('',(#126640),#64304) ;
#893=STYLED_ITEM('',(#126640),#64305) ;
#894=STYLED_ITEM('',(#126640),#64306) ;
#895=STYLED_ITEM('',(#126640),#64307) ;
#896=STYLED_ITEM('',(#126640),#64308) ;
#897=STYLED_ITEM('',(#126640),#64309) ;
#898=STYLED_ITEM('',(#126640),#64310) ;
#899=STYLED_ITEM('',(#126640),#64311) ;
#900=STYLED_ITEM('',(#126640),#64312) ;
#901=STYLED_ITEM('',(#126640),#64313) ;
#902=STYLED_ITEM('',(#126640),#64314) ;
#903=STYLED_ITEM('',(#126640),#64315) ;
#904=STYLED_ITEM('',(#126640),#64316) ;
#905=STYLED_ITEM('',(#126640),#64317) ;
#906=STYLED_ITEM('',(#126640),#64318) ;
#907=STYLED_ITEM('',(#126640),#64319) ;
#908=STYLED_ITEM('',(#126640),#64320) ;
#909=STYLED_ITEM('',(#126640),#64321) ;
#910=STYLED_ITEM('',(#126640),#64322) ;
#911=STYLED_ITEM('',(#126640),#64323) ;
#912=STYLED_ITEM('',(#126640),#64324) ;
#913=STYLED_ITEM('',(#126640),#64325) ;
#914=STYLED_ITEM('',(#126640),#64326) ;
#915=STYLED_ITEM('',(#126640),#64327) ;
#916=STYLED_ITEM('',(#126640),#64328) ;
#917=STYLED_ITEM('',(#126640),#64329) ;
#918=STYLED_ITEM('',(#126640),#64330) ;
#919=STYLED_ITEM('',(#126640),#64331) ;
#920=STYLED_ITEM('',(#126640),#64332) ;
#921=STYLED_ITEM('',(#126640),#64333) ;
#922=STYLED_ITEM('',(#126640),#64334) ;
#923=STYLED_ITEM('',(#126640),#64335) ;
#924=STYLED_ITEM('',(#126640),#64336) ;
#925=STYLED_ITEM('',(#126640),#64337) ;
#926=STYLED_ITEM('',(#126640),#64338) ;
#927=STYLED_ITEM('',(#126640),#64339) ;
#928=STYLED_ITEM('',(#126640),#64340) ;
#929=STYLED_ITEM('',(#126640),#64341) ;
#930=STYLED_ITEM('',(#126640),#64342) ;
#931=STYLED_ITEM('',(#126640),#64343) ;
#932=STYLED_ITEM('',(#126640),#64344) ;
#933=STYLED_ITEM('',(#126640),#64345) ;
#934=STYLED_ITEM('',(#126640),#64346) ;
#935=STYLED_ITEM('',(#126640),#64347) ;
#936=STYLED_ITEM('',(#126640),#64348) ;
#937=STYLED_ITEM('',(#126640),#64349) ;
#938=STYLED_ITEM('',(#126640),#64350) ;
#939=STYLED_ITEM('',(#126640),#64351) ;
#940=STYLED_ITEM('',(#126640),#64352) ;
#941=STYLED_ITEM('',(#126640),#64353) ;
#942=STYLED_ITEM('',(#126640),#64354) ;
#943=STYLED_ITEM('',(#126640),#64355) ;
#944=STYLED_ITEM('',(#126640),#64356) ;
#945=STYLED_ITEM('',(#126640),#64357) ;
#946=STYLED_ITEM('',(#126640),#64358) ;
#947=STYLED_ITEM('',(#126640),#64359) ;
#948=STYLED_ITEM('',(#126640),#64360) ;
#949=STYLED_ITEM('',(#126640),#64361) ;
#950=STYLED_ITEM('',(#126640),#64362) ;
#951=STYLED_ITEM('',(#126640),#64363) ;
#952=STYLED_ITEM('',(#126640),#64364) ;
#953=STYLED_ITEM('',(#126641),#64365) ;
#954=STYLED_ITEM('',(#126641),#64366) ;
#955=STYLED_ITEM('',(#126641),#64367) ;
#956=STYLED_ITEM('',(#126641),#64368) ;
#957=STYLED_ITEM('',(#126641),#64369) ;
#958=STYLED_ITEM('',(#126641),#64370) ;
#959=STYLED_ITEM('',(#126640),#64371) ;
#960=STYLED_ITEM('',(#126641),#64372) ;
#961=STYLED_ITEM('',(#126641),#64373) ;
#962=STYLED_ITEM('',(#126641),#64374) ;
#963=STYLED_ITEM('',(#126641),#64375) ;
#964=STYLED_ITEM('',(#126641),#64376) ;
#965=STYLED_ITEM('',(#126640),#64377) ;
#966=STYLED_ITEM('',(#126640),#64378) ;
#967=STYLED_ITEM('',(#126641),#64379) ;
#968=STYLED_ITEM('',(#126641),#64380) ;
#969=STYLED_ITEM('',(#126640),#64381) ;
#970=STYLED_ITEM('',(#126641),#64382) ;
#971=STYLED_ITEM('',(#126641),#64383) ;
#972=STYLED_ITEM('',(#126641),#64384) ;
#973=STYLED_ITEM('',(#126641),#64385) ;
#974=STYLED_ITEM('',(#126641),#64386) ;
#975=STYLED_ITEM('',(#126641),#64387) ;
#976=STYLED_ITEM('',(#126641),#64388) ;
#977=STYLED_ITEM('',(#126641),#64389) ;
#978=STYLED_ITEM('',(#126640),#64390) ;
#979=STYLED_ITEM('',(#126641),#64391) ;
#980=STYLED_ITEM('',(#126641),#64392) ;
#981=STYLED_ITEM('',(#126640),#64393) ;
#982=STYLED_ITEM('',(#126641),#64394) ;
#983=STYLED_ITEM('',(#126641),#64395) ;
#984=STYLED_ITEM('',(#126641),#64396) ;
#985=STYLED_ITEM('',(#126641),#64397) ;
#986=STYLED_ITEM('',(#126640),#64398) ;
#987=STYLED_ITEM('',(#126640),#64399) ;
#988=STYLED_ITEM('',(#126641),#64400) ;
#989=STYLED_ITEM('',(#126640),#64401) ;
#990=STYLED_ITEM('',(#126640),#64402) ;
#991=STYLED_ITEM('',(#126640),#64403) ;
#992=STYLED_ITEM('',(#126640),#64404) ;
#993=STYLED_ITEM('',(#126640),#64405) ;
#994=STYLED_ITEM('',(#126640),#64406) ;
#995=STYLED_ITEM('',(#126640),#64407) ;
#996=STYLED_ITEM('',(#126640),#64408) ;
#997=STYLED_ITEM('',(#126640),#64409) ;
#998=STYLED_ITEM('',(#126640),#64410) ;
#999=STYLED_ITEM('',(#126640),#64411) ;
#1000=STYLED_ITEM('',(#126640),#64412) ;
#1001=STYLED_ITEM('',(#126640),#64413) ;
#1002=STYLED_ITEM('',(#126640),#64414) ;
#1003=STYLED_ITEM('',(#126640),#64415) ;
#1004=STYLED_ITEM('',(#126640),#64416) ;
#1005=STYLED_ITEM('',(#126640),#64417) ;
#1006=STYLED_ITEM('',(#126640),#64418) ;
#1007=STYLED_ITEM('',(#126640),#64419) ;
#1008=STYLED_ITEM('',(#126640),#64420) ;
#1009=STYLED_ITEM('',(#126640),#64421) ;
#1010=STYLED_ITEM('',(#126640),#64422) ;
#1011=STYLED_ITEM('',(#126640),#64423) ;
#1012=STYLED_ITEM('',(#126640),#64424) ;
#1013=STYLED_ITEM('',(#126640),#64425) ;
#1014=STYLED_ITEM('',(#126640),#64426) ;
#1015=STYLED_ITEM('',(#126640),#64427) ;
#1016=STYLED_ITEM('',(#126640),#64428) ;
#1017=STYLED_ITEM('',(#126640),#64429) ;
#1018=STYLED_ITEM('',(#126640),#64430) ;
#1019=STYLED_ITEM('',(#126640),#64431) ;
#1020=STYLED_ITEM('',(#126640),#64432) ;
#1021=STYLED_ITEM('',(#126640),#64433) ;
#1022=STYLED_ITEM('',(#126640),#64434) ;
#1023=STYLED_ITEM('',(#126640),#64435) ;
#1024=STYLED_ITEM('',(#126640),#64436) ;
#1025=STYLED_ITEM('',(#126640),#64437) ;
#1026=STYLED_ITEM('',(#126640),#64438) ;
#1027=STYLED_ITEM('',(#126640),#64439) ;
#1028=STYLED_ITEM('',(#126640),#64440) ;
#1029=STYLED_ITEM('',(#126640),#64441) ;
#1030=STYLED_ITEM('',(#126640),#64442) ;
#1031=STYLED_ITEM('',(#126640),#64443) ;
#1032=STYLED_ITEM('',(#126640),#64444) ;
#1033=STYLED_ITEM('',(#126640),#64445) ;
#1034=STYLED_ITEM('',(#126640),#64446) ;
#1035=STYLED_ITEM('',(#126640),#64447) ;
#1036=STYLED_ITEM('',(#126641),#64448) ;
#1037=STYLED_ITEM('',(#126641),#64449) ;
#1038=STYLED_ITEM('',(#126641),#64450) ;
#1039=STYLED_ITEM('',(#126641),#64451) ;
#1040=STYLED_ITEM('',(#126641),#64452) ;
#1041=STYLED_ITEM('',(#126641),#64453) ;
#1042=STYLED_ITEM('',(#126641),#64454) ;
#1043=STYLED_ITEM('',(#126641),#64455) ;
#1044=STYLED_ITEM('',(#126641),#64456) ;
#1045=STYLED_ITEM('',(#126641),#64457) ;
#1046=STYLED_ITEM('',(#126641),#64458) ;
#1047=STYLED_ITEM('',(#126641),#64459) ;
#1048=STYLED_ITEM('',(#126641),#64460) ;
#1049=STYLED_ITEM('',(#126641),#64461) ;
#1050=STYLED_ITEM('',(#126641),#64462) ;
#1051=STYLED_ITEM('',(#126641),#64463) ;
#1052=STYLED_ITEM('',(#126640),#64464) ;
#1053=STYLED_ITEM('',(#126640),#64465) ;
#1054=STYLED_ITEM('',(#126640),#64466) ;
#1055=STYLED_ITEM('',(#126640),#64467) ;
#1056=STYLED_ITEM('',(#126640),#64468) ;
#1057=STYLED_ITEM('',(#126640),#64469) ;
#1058=STYLED_ITEM('',(#126640),#64470) ;
#1059=STYLED_ITEM('',(#126640),#64471) ;
#1060=STYLED_ITEM('',(#126640),#64472) ;
#1061=STYLED_ITEM('',(#126639),#4174) ;
#1062=STYLED_ITEM('',(#126640),#64473) ;
#1063=STYLED_ITEM('',(#126640),#64474) ;
#1064=STYLED_ITEM('',(#126640),#64475) ;
#1065=STYLED_ITEM('',(#126640),#64476) ;
#1066=STYLED_ITEM('',(#126640),#64477) ;
#1067=STYLED_ITEM('',(#126640),#64478) ;
#1068=STYLED_ITEM('',(#126640),#64479) ;
#1069=STYLED_ITEM('',(#126640),#64480) ;
#1070=STYLED_ITEM('',(#126640),#64481) ;
#1071=STYLED_ITEM('',(#126640),#64482) ;
#1072=STYLED_ITEM('',(#126640),#64483) ;
#1073=STYLED_ITEM('',(#126640),#64484) ;
#1074=STYLED_ITEM('',(#126640),#64485) ;
#1075=STYLED_ITEM('',(#126640),#64486) ;
#1076=STYLED_ITEM('',(#126640),#64487) ;
#1077=STYLED_ITEM('',(#126640),#64488) ;
#1078=STYLED_ITEM('',(#126640),#64489) ;
#1079=STYLED_ITEM('',(#126640),#64490) ;
#1080=STYLED_ITEM('',(#126640),#64491) ;
#1081=STYLED_ITEM('',(#126640),#64492) ;
#1082=STYLED_ITEM('',(#126640),#64493) ;
#1083=STYLED_ITEM('',(#126640),#64494) ;
#1084=STYLED_ITEM('',(#126640),#64495) ;
#1085=STYLED_ITEM('',(#126640),#64496) ;
#1086=STYLED_ITEM('',(#126640),#64497) ;
#1087=STYLED_ITEM('',(#126640),#64498) ;
#1088=STYLED_ITEM('',(#126640),#64499) ;
#1089=STYLED_ITEM('',(#126640),#64500) ;
#1090=STYLED_ITEM('',(#126640),#64501) ;
#1091=STYLED_ITEM('',(#126640),#64502) ;
#1092=STYLED_ITEM('',(#126640),#64503) ;
#1093=STYLED_ITEM('',(#126640),#64504) ;
#1094=STYLED_ITEM('',(#126640),#64505) ;
#1095=STYLED_ITEM('',(#126640),#64506) ;
#1096=STYLED_ITEM('',(#126640),#64507) ;
#1097=STYLED_ITEM('',(#126640),#64508) ;
#1098=STYLED_ITEM('',(#126640),#64509) ;
#1099=STYLED_ITEM('',(#126640),#64510) ;
#1100=STYLED_ITEM('',(#126640),#64511) ;
#1101=STYLED_ITEM('',(#126640),#64512) ;
#1102=STYLED_ITEM('',(#126640),#64513) ;
#1103=STYLED_ITEM('',(#126640),#64514) ;
#1104=STYLED_ITEM('',(#126640),#64515) ;
#1105=STYLED_ITEM('',(#126640),#64516) ;
#1106=STYLED_ITEM('',(#126640),#64517) ;
#1107=STYLED_ITEM('',(#126640),#64518) ;
#1108=STYLED_ITEM('',(#126640),#64519) ;
#1109=STYLED_ITEM('',(#126640),#64520) ;
#1110=STYLED_ITEM('',(#126640),#64521) ;
#1111=STYLED_ITEM('',(#126640),#64522) ;
#1112=STYLED_ITEM('',(#126640),#64523) ;
#1113=STYLED_ITEM('',(#126640),#64524) ;
#1114=STYLED_ITEM('',(#126640),#64525) ;
#1115=STYLED_ITEM('',(#126640),#64526) ;
#1116=STYLED_ITEM('',(#126640),#64527) ;
#1117=STYLED_ITEM('',(#126640),#64528) ;
#1118=STYLED_ITEM('',(#126641),#64529) ;
#1119=STYLED_ITEM('',(#126641),#64530) ;
#1120=STYLED_ITEM('',(#126641),#64531) ;
#1121=STYLED_ITEM('',(#126641),#64532) ;
#1122=STYLED_ITEM('',(#126641),#64533) ;
#1123=STYLED_ITEM('',(#126641),#64534) ;
#1124=STYLED_ITEM('',(#126641),#64535) ;
#1125=STYLED_ITEM('',(#126641),#64536) ;
#1126=STYLED_ITEM('',(#126641),#64537) ;
#1127=STYLED_ITEM('',(#126641),#64538) ;
#1128=STYLED_ITEM('',(#126641),#64539) ;
#1129=STYLED_ITEM('',(#126641),#64540) ;
#1130=STYLED_ITEM('',(#126641),#64541) ;
#1131=STYLED_ITEM('',(#126641),#64542) ;
#1132=STYLED_ITEM('',(#126641),#64543) ;
#1133=STYLED_ITEM('',(#126641),#64544) ;
#1134=STYLED_ITEM('',(#126641),#64545) ;
#1135=STYLED_ITEM('',(#126641),#64546) ;
#1136=STYLED_ITEM('',(#126641),#64547) ;
#1137=STYLED_ITEM('',(#126641),#64548) ;
#1138=STYLED_ITEM('',(#126640),#64549) ;
#1139=STYLED_ITEM('',(#126640),#64550) ;
#1140=STYLED_ITEM('',(#126640),#64551) ;
#1141=STYLED_ITEM('',(#126640),#64552) ;
#1142=STYLED_ITEM('',(#126640),#64553) ;
#1143=STYLED_ITEM('',(#126640),#64554) ;
#1144=STYLED_ITEM('',(#126640),#64555) ;
#1145=STYLED_ITEM('',(#126640),#64556) ;
#1146=STYLED_ITEM('',(#126640),#64557) ;
#1147=STYLED_ITEM('',(#126640),#64558) ;
#1148=STYLED_ITEM('',(#126640),#64559) ;
#1149=STYLED_ITEM('',(#126640),#64560) ;
#1150=STYLED_ITEM('',(#126640),#64561) ;
#1151=STYLED_ITEM('',(#126640),#64562) ;
#1152=STYLED_ITEM('',(#126640),#64563) ;
#1153=STYLED_ITEM('',(#126640),#64564) ;
#1154=STYLED_ITEM('',(#126640),#64565) ;
#1155=STYLED_ITEM('',(#126640),#64566) ;
#1156=STYLED_ITEM('',(#126640),#64567) ;
#1157=STYLED_ITEM('',(#126640),#64568) ;
#1158=STYLED_ITEM('',(#126640),#64569) ;
#1159=STYLED_ITEM('',(#126640),#64570) ;
#1160=STYLED_ITEM('',(#126640),#64571) ;
#1161=STYLED_ITEM('',(#126640),#64572) ;
#1162=STYLED_ITEM('',(#126640),#64573) ;
#1163=STYLED_ITEM('',(#126640),#64574) ;
#1164=STYLED_ITEM('',(#126640),#64575) ;
#1165=STYLED_ITEM('',(#126640),#64576) ;
#1166=STYLED_ITEM('',(#126640),#64577) ;
#1167=STYLED_ITEM('',(#126640),#64578) ;
#1168=STYLED_ITEM('',(#126640),#64579) ;
#1169=STYLED_ITEM('',(#126640),#64580) ;
#1170=STYLED_ITEM('',(#126640),#64581) ;
#1171=STYLED_ITEM('',(#126640),#64582) ;
#1172=STYLED_ITEM('',(#126640),#64583) ;
#1173=STYLED_ITEM('',(#126640),#64584) ;
#1174=STYLED_ITEM('',(#126640),#64585) ;
#1175=STYLED_ITEM('',(#126640),#64586) ;
#1176=STYLED_ITEM('',(#126640),#64587) ;
#1177=STYLED_ITEM('',(#126640),#64588) ;
#1178=STYLED_ITEM('',(#126640),#64589) ;
#1179=STYLED_ITEM('',(#126640),#64590) ;
#1180=STYLED_ITEM('',(#126640),#64591) ;
#1181=STYLED_ITEM('',(#126640),#64592) ;
#1182=STYLED_ITEM('',(#126640),#64593) ;
#1183=STYLED_ITEM('',(#126640),#64594) ;
#1184=STYLED_ITEM('',(#126640),#64595) ;
#1185=STYLED_ITEM('',(#126640),#64596) ;
#1186=STYLED_ITEM('',(#126640),#64597) ;
#1187=STYLED_ITEM('',(#126640),#64598) ;
#1188=STYLED_ITEM('',(#126640),#64599) ;
#1189=STYLED_ITEM('',(#126640),#64600) ;
#1190=STYLED_ITEM('',(#126640),#64601) ;
#1191=STYLED_ITEM('',(#126640),#64602) ;
#1192=STYLED_ITEM('',(#126640),#64603) ;
#1193=STYLED_ITEM('',(#126640),#64604) ;
#1194=STYLED_ITEM('',(#126640),#64605) ;
#1195=STYLED_ITEM('',(#126640),#64606) ;
#1196=STYLED_ITEM('',(#126640),#64607) ;
#1197=STYLED_ITEM('',(#126640),#64608) ;
#1198=STYLED_ITEM('',(#126640),#64609) ;
#1199=STYLED_ITEM('',(#126640),#64610) ;
#1200=STYLED_ITEM('',(#126640),#64611) ;
#1201=STYLED_ITEM('',(#126640),#64612) ;
#1202=STYLED_ITEM('',(#126640),#64613) ;
#1203=STYLED_ITEM('',(#126640),#64614) ;
#1204=STYLED_ITEM('',(#126640),#64615) ;
#1205=STYLED_ITEM('',(#126640),#64616) ;
#1206=STYLED_ITEM('',(#126640),#64617) ;
#1207=STYLED_ITEM('',(#126640),#64618) ;
#1208=STYLED_ITEM('',(#126640),#64619) ;
#1209=STYLED_ITEM('',(#126640),#64620) ;
#1210=STYLED_ITEM('',(#126640),#64621) ;
#1211=STYLED_ITEM('',(#126640),#64622) ;
#1212=STYLED_ITEM('',(#126640),#64623) ;
#1213=STYLED_ITEM('',(#126640),#64624) ;
#1214=STYLED_ITEM('',(#126640),#64625) ;
#1215=STYLED_ITEM('',(#126640),#64626) ;
#1216=STYLED_ITEM('',(#126640),#64627) ;
#1217=STYLED_ITEM('',(#126640),#64628) ;
#1218=STYLED_ITEM('',(#126640),#64629) ;
#1219=STYLED_ITEM('',(#126640),#64630) ;
#1220=STYLED_ITEM('',(#126640),#64631) ;
#1221=STYLED_ITEM('',(#126640),#64632) ;
#1222=STYLED_ITEM('',(#126640),#64633) ;
#1223=STYLED_ITEM('',(#126640),#64634) ;
#1224=STYLED_ITEM('',(#126640),#64635) ;
#1225=STYLED_ITEM('',(#126640),#64636) ;
#1226=STYLED_ITEM('',(#126640),#64637) ;
#1227=STYLED_ITEM('',(#126640),#64638) ;
#1228=STYLED_ITEM('',(#126640),#64639) ;
#1229=STYLED_ITEM('',(#126640),#64640) ;
#1230=STYLED_ITEM('',(#126640),#64641) ;
#1231=STYLED_ITEM('',(#126640),#64642) ;
#1232=STYLED_ITEM('',(#126640),#64643) ;
#1233=STYLED_ITEM('',(#126640),#64644) ;
#1234=STYLED_ITEM('',(#126640),#64645) ;
#1235=STYLED_ITEM('',(#126640),#64646) ;
#1236=STYLED_ITEM('',(#126640),#64647) ;
#1237=STYLED_ITEM('',(#126640),#64648) ;
#1238=STYLED_ITEM('',(#126640),#64649) ;
#1239=STYLED_ITEM('',(#126640),#64650) ;
#1240=STYLED_ITEM('',(#126640),#64651) ;
#1241=STYLED_ITEM('',(#126640),#64652) ;
#1242=STYLED_ITEM('',(#126640),#64653) ;
#1243=STYLED_ITEM('',(#126641),#64654) ;
#1244=STYLED_ITEM('',(#126641),#64655) ;
#1245=STYLED_ITEM('',(#126641),#64656) ;
#1246=STYLED_ITEM('',(#126641),#64657) ;
#1247=STYLED_ITEM('',(#126641),#64658) ;
#1248=STYLED_ITEM('',(#126641),#64659) ;
#1249=STYLED_ITEM('',(#126640),#64660) ;
#1250=STYLED_ITEM('',(#126641),#64661) ;
#1251=STYLED_ITEM('',(#126641),#64662) ;
#1252=STYLED_ITEM('',(#126641),#64663) ;
#1253=STYLED_ITEM('',(#126641),#64664) ;
#1254=STYLED_ITEM('',(#126641),#64665) ;
#1255=STYLED_ITEM('',(#126640),#64666) ;
#1256=STYLED_ITEM('',(#126640),#64667) ;
#1257=STYLED_ITEM('',(#126641),#64668) ;
#1258=STYLED_ITEM('',(#126641),#64669) ;
#1259=STYLED_ITEM('',(#126640),#64670) ;
#1260=STYLED_ITEM('',(#126641),#64671) ;
#1261=STYLED_ITEM('',(#126641),#64672) ;
#1262=STYLED_ITEM('',(#126641),#64673) ;
#1263=STYLED_ITEM('',(#126641),#64674) ;
#1264=STYLED_ITEM('',(#126641),#64675) ;
#1265=STYLED_ITEM('',(#126641),#64676) ;
#1266=STYLED_ITEM('',(#126641),#64677) ;
#1267=STYLED_ITEM('',(#126641),#64678) ;
#1268=STYLED_ITEM('',(#126640),#64679) ;
#1269=STYLED_ITEM('',(#126641),#64680) ;
#1270=STYLED_ITEM('',(#126641),#64681) ;
#1271=STYLED_ITEM('',(#126640),#64682) ;
#1272=STYLED_ITEM('',(#126641),#64683) ;
#1273=STYLED_ITEM('',(#126641),#64684) ;
#1274=STYLED_ITEM('',(#126641),#64685) ;
#1275=STYLED_ITEM('',(#126641),#64686) ;
#1276=STYLED_ITEM('',(#126640),#64687) ;
#1277=STYLED_ITEM('',(#126640),#64688) ;
#1278=STYLED_ITEM('',(#126641),#64689) ;
#1279=STYLED_ITEM('',(#126640),#64690) ;
#1280=STYLED_ITEM('',(#126640),#64691) ;
#1281=STYLED_ITEM('',(#126640),#64692) ;
#1282=STYLED_ITEM('',(#126640),#64693) ;
#1283=STYLED_ITEM('',(#126640),#64694) ;
#1284=STYLED_ITEM('',(#126640),#64695) ;
#1285=STYLED_ITEM('',(#126640),#64696) ;
#1286=STYLED_ITEM('',(#126640),#64697) ;
#1287=STYLED_ITEM('',(#126640),#64698) ;
#1288=STYLED_ITEM('',(#126640),#64699) ;
#1289=STYLED_ITEM('',(#126640),#64700) ;
#1290=STYLED_ITEM('',(#126640),#64701) ;
#1291=STYLED_ITEM('',(#126640),#64702) ;
#1292=STYLED_ITEM('',(#126640),#64703) ;
#1293=STYLED_ITEM('',(#126640),#64704) ;
#1294=STYLED_ITEM('',(#126640),#64705) ;
#1295=STYLED_ITEM('',(#126640),#64706) ;
#1296=STYLED_ITEM('',(#126640),#64707) ;
#1297=STYLED_ITEM('',(#126640),#64708) ;
#1298=STYLED_ITEM('',(#126640),#64709) ;
#1299=STYLED_ITEM('',(#126640),#64710) ;
#1300=STYLED_ITEM('',(#126640),#64711) ;
#1301=STYLED_ITEM('',(#126640),#64712) ;
#1302=STYLED_ITEM('',(#126640),#64713) ;
#1303=STYLED_ITEM('',(#126640),#64714) ;
#1304=STYLED_ITEM('',(#126640),#64715) ;
#1305=STYLED_ITEM('',(#126640),#64716) ;
#1306=STYLED_ITEM('',(#126640),#64717) ;
#1307=STYLED_ITEM('',(#126640),#64718) ;
#1308=STYLED_ITEM('',(#126640),#64719) ;
#1309=STYLED_ITEM('',(#126640),#64720) ;
#1310=STYLED_ITEM('',(#126640),#64721) ;
#1311=STYLED_ITEM('',(#126640),#64722) ;
#1312=STYLED_ITEM('',(#126640),#64723) ;
#1313=STYLED_ITEM('',(#126640),#64724) ;
#1314=STYLED_ITEM('',(#126640),#64725) ;
#1315=STYLED_ITEM('',(#126640),#64726) ;
#1316=STYLED_ITEM('',(#126640),#64727) ;
#1317=STYLED_ITEM('',(#126640),#64728) ;
#1318=STYLED_ITEM('',(#126640),#64729) ;
#1319=STYLED_ITEM('',(#126640),#64730) ;
#1320=STYLED_ITEM('',(#126640),#64731) ;
#1321=STYLED_ITEM('',(#126640),#64732) ;
#1322=STYLED_ITEM('',(#126640),#64733) ;
#1323=STYLED_ITEM('',(#126640),#64734) ;
#1324=STYLED_ITEM('',(#126640),#64735) ;
#1325=STYLED_ITEM('',(#126640),#64736) ;
#1326=STYLED_ITEM('',(#126641),#64737) ;
#1327=STYLED_ITEM('',(#126641),#64738) ;
#1328=STYLED_ITEM('',(#126641),#64739) ;
#1329=STYLED_ITEM('',(#126641),#64740) ;
#1330=STYLED_ITEM('',(#126641),#64741) ;
#1331=STYLED_ITEM('',(#126641),#64742) ;
#1332=STYLED_ITEM('',(#126641),#64743) ;
#1333=STYLED_ITEM('',(#126641),#64744) ;
#1334=STYLED_ITEM('',(#126641),#64745) ;
#1335=STYLED_ITEM('',(#126641),#64746) ;
#1336=STYLED_ITEM('',(#126641),#64747) ;
#1337=STYLED_ITEM('',(#126641),#64748) ;
#1338=STYLED_ITEM('',(#126641),#64749) ;
#1339=STYLED_ITEM('',(#126641),#64750) ;
#1340=STYLED_ITEM('',(#126641),#64751) ;
#1341=STYLED_ITEM('',(#126641),#64752) ;
#1342=STYLED_ITEM('',(#126640),#64753) ;
#1343=STYLED_ITEM('',(#126640),#64754) ;
#1344=STYLED_ITEM('',(#126640),#64755) ;
#1345=STYLED_ITEM('',(#126640),#64756) ;
#1346=STYLED_ITEM('',(#126640),#64757) ;
#1347=STYLED_ITEM('',(#126640),#64758) ;
#1348=STYLED_ITEM('',(#126640),#64759) ;
#1349=STYLED_ITEM('',(#126640),#64760) ;
#1350=STYLED_ITEM('',(#126640),#64761) ;
#1351=STYLED_ITEM('',(#126639),#4175) ;
#1352=STYLED_ITEM('',(#126640),#64762) ;
#1353=STYLED_ITEM('',(#126640),#64763) ;
#1354=STYLED_ITEM('',(#126640),#64764) ;
#1355=STYLED_ITEM('',(#126640),#64765) ;
#1356=STYLED_ITEM('',(#126640),#64766) ;
#1357=STYLED_ITEM('',(#126640),#64767) ;
#1358=STYLED_ITEM('',(#126640),#64768) ;
#1359=STYLED_ITEM('',(#126640),#64769) ;
#1360=STYLED_ITEM('',(#126640),#64770) ;
#1361=STYLED_ITEM('',(#126640),#64771) ;
#1362=STYLED_ITEM('',(#126640),#64772) ;
#1363=STYLED_ITEM('',(#126640),#64773) ;
#1364=STYLED_ITEM('',(#126640),#64774) ;
#1365=STYLED_ITEM('',(#126640),#64775) ;
#1366=STYLED_ITEM('',(#126640),#64776) ;
#1367=STYLED_ITEM('',(#126640),#64777) ;
#1368=STYLED_ITEM('',(#126640),#64778) ;
#1369=STYLED_ITEM('',(#126640),#64779) ;
#1370=STYLED_ITEM('',(#126640),#64780) ;
#1371=STYLED_ITEM('',(#126640),#64781) ;
#1372=STYLED_ITEM('',(#126640),#64782) ;
#1373=STYLED_ITEM('',(#126640),#64783) ;
#1374=STYLED_ITEM('',(#126640),#64784) ;
#1375=STYLED_ITEM('',(#126640),#64785) ;
#1376=STYLED_ITEM('',(#126640),#64786) ;
#1377=STYLED_ITEM('',(#126640),#64787) ;
#1378=STYLED_ITEM('',(#126640),#64788) ;
#1379=STYLED_ITEM('',(#126640),#64789) ;
#1380=STYLED_ITEM('',(#126640),#64790) ;
#1381=STYLED_ITEM('',(#126640),#64791) ;
#1382=STYLED_ITEM('',(#126640),#64792) ;
#1383=STYLED_ITEM('',(#126640),#64793) ;
#1384=STYLED_ITEM('',(#126640),#64794) ;
#1385=STYLED_ITEM('',(#126640),#64795) ;
#1386=STYLED_ITEM('',(#126640),#64796) ;
#1387=STYLED_ITEM('',(#126640),#64797) ;
#1388=STYLED_ITEM('',(#126640),#64798) ;
#1389=STYLED_ITEM('',(#126640),#64799) ;
#1390=STYLED_ITEM('',(#126640),#64800) ;
#1391=STYLED_ITEM('',(#126640),#64801) ;
#1392=STYLED_ITEM('',(#126640),#64802) ;
#1393=STYLED_ITEM('',(#126640),#64803) ;
#1394=STYLED_ITEM('',(#126640),#64804) ;
#1395=STYLED_ITEM('',(#126640),#64805) ;
#1396=STYLED_ITEM('',(#126640),#64806) ;
#1397=STYLED_ITEM('',(#126640),#64807) ;
#1398=STYLED_ITEM('',(#126640),#64808) ;
#1399=STYLED_ITEM('',(#126640),#64809) ;
#1400=STYLED_ITEM('',(#126640),#64810) ;
#1401=STYLED_ITEM('',(#126640),#64811) ;
#1402=STYLED_ITEM('',(#126640),#64812) ;
#1403=STYLED_ITEM('',(#126640),#64813) ;
#1404=STYLED_ITEM('',(#126640),#64814) ;
#1405=STYLED_ITEM('',(#126640),#64815) ;
#1406=STYLED_ITEM('',(#126640),#64816) ;
#1407=STYLED_ITEM('',(#126640),#64817) ;
#1408=STYLED_ITEM('',(#126641),#64818) ;
#1409=STYLED_ITEM('',(#126641),#64819) ;
#1410=STYLED_ITEM('',(#126641),#64820) ;
#1411=STYLED_ITEM('',(#126641),#64821) ;
#1412=STYLED_ITEM('',(#126641),#64822) ;
#1413=STYLED_ITEM('',(#126641),#64823) ;
#1414=STYLED_ITEM('',(#126641),#64824) ;
#1415=STYLED_ITEM('',(#126641),#64825) ;
#1416=STYLED_ITEM('',(#126641),#64826) ;
#1417=STYLED_ITEM('',(#126641),#64827) ;
#1418=STYLED_ITEM('',(#126641),#64828) ;
#1419=STYLED_ITEM('',(#126641),#64829) ;
#1420=STYLED_ITEM('',(#126641),#64830) ;
#1421=STYLED_ITEM('',(#126641),#64831) ;
#1422=STYLED_ITEM('',(#126641),#64832) ;
#1423=STYLED_ITEM('',(#126641),#64833) ;
#1424=STYLED_ITEM('',(#126641),#64834) ;
#1425=STYLED_ITEM('',(#126641),#64835) ;
#1426=STYLED_ITEM('',(#126641),#64836) ;
#1427=STYLED_ITEM('',(#126641),#64837) ;
#1428=STYLED_ITEM('',(#126640),#64838) ;
#1429=STYLED_ITEM('',(#126640),#64839) ;
#1430=STYLED_ITEM('',(#126640),#64840) ;
#1431=STYLED_ITEM('',(#126640),#64841) ;
#1432=STYLED_ITEM('',(#126640),#64842) ;
#1433=STYLED_ITEM('',(#126640),#64843) ;
#1434=STYLED_ITEM('',(#126640),#64844) ;
#1435=STYLED_ITEM('',(#126640),#64845) ;
#1436=STYLED_ITEM('',(#126640),#64846) ;
#1437=STYLED_ITEM('',(#126640),#64847) ;
#1438=STYLED_ITEM('',(#126640),#64848) ;
#1439=STYLED_ITEM('',(#126640),#64849) ;
#1440=STYLED_ITEM('',(#126640),#64850) ;
#1441=STYLED_ITEM('',(#126640),#64851) ;
#1442=STYLED_ITEM('',(#126640),#64852) ;
#1443=STYLED_ITEM('',(#126640),#64853) ;
#1444=STYLED_ITEM('',(#126640),#64854) ;
#1445=STYLED_ITEM('',(#126640),#64855) ;
#1446=STYLED_ITEM('',(#126640),#64856) ;
#1447=STYLED_ITEM('',(#126640),#64857) ;
#1448=STYLED_ITEM('',(#126640),#64858) ;
#1449=STYLED_ITEM('',(#126640),#64859) ;
#1450=STYLED_ITEM('',(#126640),#64860) ;
#1451=STYLED_ITEM('',(#126640),#64861) ;
#1452=STYLED_ITEM('',(#126640),#64862) ;
#1453=STYLED_ITEM('',(#126640),#64863) ;
#1454=STYLED_ITEM('',(#126640),#64864) ;
#1455=STYLED_ITEM('',(#126640),#64865) ;
#1456=STYLED_ITEM('',(#126640),#64866) ;
#1457=STYLED_ITEM('',(#126640),#64867) ;
#1458=STYLED_ITEM('',(#126640),#64868) ;
#1459=STYLED_ITEM('',(#126640),#64869) ;
#1460=STYLED_ITEM('',(#126640),#64870) ;
#1461=STYLED_ITEM('',(#126640),#64871) ;
#1462=STYLED_ITEM('',(#126640),#64872) ;
#1463=STYLED_ITEM('',(#126640),#64873) ;
#1464=STYLED_ITEM('',(#126640),#64874) ;
#1465=STYLED_ITEM('',(#126640),#64875) ;
#1466=STYLED_ITEM('',(#126640),#64876) ;
#1467=STYLED_ITEM('',(#126640),#64877) ;
#1468=STYLED_ITEM('',(#126640),#64878) ;
#1469=STYLED_ITEM('',(#126640),#64879) ;
#1470=STYLED_ITEM('',(#126640),#64880) ;
#1471=STYLED_ITEM('',(#126640),#64881) ;
#1472=STYLED_ITEM('',(#126640),#64882) ;
#1473=STYLED_ITEM('',(#126640),#64883) ;
#1474=STYLED_ITEM('',(#126640),#64884) ;
#1475=STYLED_ITEM('',(#126640),#64885) ;
#1476=STYLED_ITEM('',(#126640),#64886) ;
#1477=STYLED_ITEM('',(#126640),#64887) ;
#1478=STYLED_ITEM('',(#126640),#64888) ;
#1479=STYLED_ITEM('',(#126640),#64889) ;
#1480=STYLED_ITEM('',(#126640),#64890) ;
#1481=STYLED_ITEM('',(#126640),#64891) ;
#1482=STYLED_ITEM('',(#126640),#64892) ;
#1483=STYLED_ITEM('',(#126640),#64893) ;
#1484=STYLED_ITEM('',(#126640),#64894) ;
#1485=STYLED_ITEM('',(#126640),#64895) ;
#1486=STYLED_ITEM('',(#126640),#64896) ;
#1487=STYLED_ITEM('',(#126640),#64897) ;
#1488=STYLED_ITEM('',(#126640),#64898) ;
#1489=STYLED_ITEM('',(#126640),#64899) ;
#1490=STYLED_ITEM('',(#126640),#64900) ;
#1491=STYLED_ITEM('',(#126640),#64901) ;
#1492=STYLED_ITEM('',(#126640),#64902) ;
#1493=STYLED_ITEM('',(#126640),#64903) ;
#1494=STYLED_ITEM('',(#126640),#64904) ;
#1495=STYLED_ITEM('',(#126640),#64905) ;
#1496=STYLED_ITEM('',(#126640),#64906) ;
#1497=STYLED_ITEM('',(#126640),#64907) ;
#1498=STYLED_ITEM('',(#126640),#64908) ;
#1499=STYLED_ITEM('',(#126640),#64909) ;
#1500=STYLED_ITEM('',(#126640),#64910) ;
#1501=STYLED_ITEM('',(#126640),#64911) ;
#1502=STYLED_ITEM('',(#126640),#64912) ;
#1503=STYLED_ITEM('',(#126640),#64913) ;
#1504=STYLED_ITEM('',(#126640),#64914) ;
#1505=STYLED_ITEM('',(#126640),#64915) ;
#1506=STYLED_ITEM('',(#126640),#64916) ;
#1507=STYLED_ITEM('',(#126640),#64917) ;
#1508=STYLED_ITEM('',(#126640),#64918) ;
#1509=STYLED_ITEM('',(#126640),#64919) ;
#1510=STYLED_ITEM('',(#126640),#64920) ;
#1511=STYLED_ITEM('',(#126640),#64921) ;
#1512=STYLED_ITEM('',(#126640),#64922) ;
#1513=STYLED_ITEM('',(#126640),#64923) ;
#1514=STYLED_ITEM('',(#126640),#64924) ;
#1515=STYLED_ITEM('',(#126640),#64925) ;
#1516=STYLED_ITEM('',(#126640),#64926) ;
#1517=STYLED_ITEM('',(#126640),#64927) ;
#1518=STYLED_ITEM('',(#126640),#64928) ;
#1519=STYLED_ITEM('',(#126640),#64929) ;
#1520=STYLED_ITEM('',(#126640),#64930) ;
#1521=STYLED_ITEM('',(#126640),#64931) ;
#1522=STYLED_ITEM('',(#126640),#64932) ;
#1523=STYLED_ITEM('',(#126640),#64933) ;
#1524=STYLED_ITEM('',(#126640),#64934) ;
#1525=STYLED_ITEM('',(#126640),#64935) ;
#1526=STYLED_ITEM('',(#126640),#64936) ;
#1527=STYLED_ITEM('',(#126640),#64937) ;
#1528=STYLED_ITEM('',(#126640),#64938) ;
#1529=STYLED_ITEM('',(#126640),#64939) ;
#1530=STYLED_ITEM('',(#126640),#64940) ;
#1531=STYLED_ITEM('',(#126640),#64941) ;
#1532=STYLED_ITEM('',(#126640),#64942) ;
#1533=STYLED_ITEM('',(#126641),#64943) ;
#1534=STYLED_ITEM('',(#126641),#64944) ;
#1535=STYLED_ITEM('',(#126641),#64945) ;
#1536=STYLED_ITEM('',(#126641),#64946) ;
#1537=STYLED_ITEM('',(#126641),#64947) ;
#1538=STYLED_ITEM('',(#126641),#64948) ;
#1539=STYLED_ITEM('',(#126640),#64949) ;
#1540=STYLED_ITEM('',(#126641),#64950) ;
#1541=STYLED_ITEM('',(#126641),#64951) ;
#1542=STYLED_ITEM('',(#126641),#64952) ;
#1543=STYLED_ITEM('',(#126641),#64953) ;
#1544=STYLED_ITEM('',(#126641),#64954) ;
#1545=STYLED_ITEM('',(#126640),#64955) ;
#1546=STYLED_ITEM('',(#126640),#64956) ;
#1547=STYLED_ITEM('',(#126641),#64957) ;
#1548=STYLED_ITEM('',(#126641),#64958) ;
#1549=STYLED_ITEM('',(#126640),#64959) ;
#1550=STYLED_ITEM('',(#126641),#64960) ;
#1551=STYLED_ITEM('',(#126641),#64961) ;
#1552=STYLED_ITEM('',(#126641),#64962) ;
#1553=STYLED_ITEM('',(#126641),#64963) ;
#1554=STYLED_ITEM('',(#126641),#64964) ;
#1555=STYLED_ITEM('',(#126641),#64965) ;
#1556=STYLED_ITEM('',(#126641),#64966) ;
#1557=STYLED_ITEM('',(#126641),#64967) ;
#1558=STYLED_ITEM('',(#126640),#64968) ;
#1559=STYLED_ITEM('',(#126641),#64969) ;
#1560=STYLED_ITEM('',(#126641),#64970) ;
#1561=STYLED_ITEM('',(#126640),#64971) ;
#1562=STYLED_ITEM('',(#126641),#64972) ;
#1563=STYLED_ITEM('',(#126641),#64973) ;
#1564=STYLED_ITEM('',(#126641),#64974) ;
#1565=STYLED_ITEM('',(#126641),#64975) ;
#1566=STYLED_ITEM('',(#126640),#64976) ;
#1567=STYLED_ITEM('',(#126640),#64977) ;
#1568=STYLED_ITEM('',(#126641),#64978) ;
#1569=STYLED_ITEM('',(#126640),#64979) ;
#1570=STYLED_ITEM('',(#126640),#64980) ;
#1571=STYLED_ITEM('',(#126640),#64981) ;
#1572=STYLED_ITEM('',(#126640),#64982) ;
#1573=STYLED_ITEM('',(#126640),#64983) ;
#1574=STYLED_ITEM('',(#126640),#64984) ;
#1575=STYLED_ITEM('',(#126640),#64985) ;
#1576=STYLED_ITEM('',(#126640),#64986) ;
#1577=STYLED_ITEM('',(#126640),#64987) ;
#1578=STYLED_ITEM('',(#126640),#64988) ;
#1579=STYLED_ITEM('',(#126640),#64989) ;
#1580=STYLED_ITEM('',(#126640),#64990) ;
#1581=STYLED_ITEM('',(#126640),#64991) ;
#1582=STYLED_ITEM('',(#126640),#64992) ;
#1583=STYLED_ITEM('',(#126640),#64993) ;
#1584=STYLED_ITEM('',(#126640),#64994) ;
#1585=STYLED_ITEM('',(#126640),#64995) ;
#1586=STYLED_ITEM('',(#126640),#64996) ;
#1587=STYLED_ITEM('',(#126640),#64997) ;
#1588=STYLED_ITEM('',(#126640),#64998) ;
#1589=STYLED_ITEM('',(#126640),#64999) ;
#1590=STYLED_ITEM('',(#126640),#65000) ;
#1591=STYLED_ITEM('',(#126640),#65001) ;
#1592=STYLED_ITEM('',(#126640),#65002) ;
#1593=STYLED_ITEM('',(#126640),#65003) ;
#1594=STYLED_ITEM('',(#126640),#65004) ;
#1595=STYLED_ITEM('',(#126640),#65005) ;
#1596=STYLED_ITEM('',(#126640),#65006) ;
#1597=STYLED_ITEM('',(#126640),#65007) ;
#1598=STYLED_ITEM('',(#126640),#65008) ;
#1599=STYLED_ITEM('',(#126640),#65009) ;
#1600=STYLED_ITEM('',(#126640),#65010) ;
#1601=STYLED_ITEM('',(#126640),#65011) ;
#1602=STYLED_ITEM('',(#126640),#65012) ;
#1603=STYLED_ITEM('',(#126640),#65013) ;
#1604=STYLED_ITEM('',(#126640),#65014) ;
#1605=STYLED_ITEM('',(#126640),#65015) ;
#1606=STYLED_ITEM('',(#126640),#65016) ;
#1607=STYLED_ITEM('',(#126640),#65017) ;
#1608=STYLED_ITEM('',(#126640),#65018) ;
#1609=STYLED_ITEM('',(#126640),#65019) ;
#1610=STYLED_ITEM('',(#126640),#65020) ;
#1611=STYLED_ITEM('',(#126640),#65021) ;
#1612=STYLED_ITEM('',(#126640),#65022) ;
#1613=STYLED_ITEM('',(#126640),#65023) ;
#1614=STYLED_ITEM('',(#126640),#65024) ;
#1615=STYLED_ITEM('',(#126640),#65025) ;
#1616=STYLED_ITEM('',(#126641),#65026) ;
#1617=STYLED_ITEM('',(#126641),#65027) ;
#1618=STYLED_ITEM('',(#126641),#65028) ;
#1619=STYLED_ITEM('',(#126641),#65029) ;
#1620=STYLED_ITEM('',(#126641),#65030) ;
#1621=STYLED_ITEM('',(#126641),#65031) ;
#1622=STYLED_ITEM('',(#126641),#65032) ;
#1623=STYLED_ITEM('',(#126641),#65033) ;
#1624=STYLED_ITEM('',(#126641),#65034) ;
#1625=STYLED_ITEM('',(#126641),#65035) ;
#1626=STYLED_ITEM('',(#126641),#65036) ;
#1627=STYLED_ITEM('',(#126641),#65037) ;
#1628=STYLED_ITEM('',(#126641),#65038) ;
#1629=STYLED_ITEM('',(#126641),#65039) ;
#1630=STYLED_ITEM('',(#126641),#65040) ;
#1631=STYLED_ITEM('',(#126641),#65041) ;
#1632=STYLED_ITEM('',(#126640),#65042) ;
#1633=STYLED_ITEM('',(#126640),#65043) ;
#1634=STYLED_ITEM('',(#126640),#65044) ;
#1635=STYLED_ITEM('',(#126640),#65045) ;
#1636=STYLED_ITEM('',(#126640),#65046) ;
#1637=STYLED_ITEM('',(#126640),#65047) ;
#1638=STYLED_ITEM('',(#126640),#65048) ;
#1639=STYLED_ITEM('',(#126640),#65049) ;
#1640=STYLED_ITEM('',(#126640),#65050) ;
#1641=STYLED_ITEM('',(#126639),#4176) ;
#1642=STYLED_ITEM('',(#126640),#65051) ;
#1643=STYLED_ITEM('',(#126640),#65052) ;
#1644=STYLED_ITEM('',(#126640),#65053) ;
#1645=STYLED_ITEM('',(#126640),#65054) ;
#1646=STYLED_ITEM('',(#126640),#65055) ;
#1647=STYLED_ITEM('',(#126640),#65056) ;
#1648=STYLED_ITEM('',(#126640),#65057) ;
#1649=STYLED_ITEM('',(#126640),#65058) ;
#1650=STYLED_ITEM('',(#126640),#65059) ;
#1651=STYLED_ITEM('',(#126640),#65060) ;
#1652=STYLED_ITEM('',(#126640),#65061) ;
#1653=STYLED_ITEM('',(#126640),#65062) ;
#1654=STYLED_ITEM('',(#126640),#65063) ;
#1655=STYLED_ITEM('',(#126640),#65064) ;
#1656=STYLED_ITEM('',(#126640),#65065) ;
#1657=STYLED_ITEM('',(#126640),#65066) ;
#1658=STYLED_ITEM('',(#126640),#65067) ;
#1659=STYLED_ITEM('',(#126640),#65068) ;
#1660=STYLED_ITEM('',(#126640),#65069) ;
#1661=STYLED_ITEM('',(#126640),#65070) ;
#1662=STYLED_ITEM('',(#126640),#65071) ;
#1663=STYLED_ITEM('',(#126640),#65072) ;
#1664=STYLED_ITEM('',(#126640),#65073) ;
#1665=STYLED_ITEM('',(#126640),#65074) ;
#1666=STYLED_ITEM('',(#126640),#65075) ;
#1667=STYLED_ITEM('',(#126640),#65076) ;
#1668=STYLED_ITEM('',(#126640),#65077) ;
#1669=STYLED_ITEM('',(#126640),#65078) ;
#1670=STYLED_ITEM('',(#126640),#65079) ;
#1671=STYLED_ITEM('',(#126640),#65080) ;
#1672=STYLED_ITEM('',(#126640),#65081) ;
#1673=STYLED_ITEM('',(#126640),#65082) ;
#1674=STYLED_ITEM('',(#126640),#65083) ;
#1675=STYLED_ITEM('',(#126640),#65084) ;
#1676=STYLED_ITEM('',(#126640),#65085) ;
#1677=STYLED_ITEM('',(#126640),#65086) ;
#1678=STYLED_ITEM('',(#126640),#65087) ;
#1679=STYLED_ITEM('',(#126640),#65088) ;
#1680=STYLED_ITEM('',(#126640),#65089) ;
#1681=STYLED_ITEM('',(#126640),#65090) ;
#1682=STYLED_ITEM('',(#126640),#65091) ;
#1683=STYLED_ITEM('',(#126640),#65092) ;
#1684=STYLED_ITEM('',(#126640),#65093) ;
#1685=STYLED_ITEM('',(#126640),#65094) ;
#1686=STYLED_ITEM('',(#126640),#65095) ;
#1687=STYLED_ITEM('',(#126640),#65096) ;
#1688=STYLED_ITEM('',(#126640),#65097) ;
#1689=STYLED_ITEM('',(#126640),#65098) ;
#1690=STYLED_ITEM('',(#126640),#65099) ;
#1691=STYLED_ITEM('',(#126640),#65100) ;
#1692=STYLED_ITEM('',(#126640),#65101) ;
#1693=STYLED_ITEM('',(#126640),#65102) ;
#1694=STYLED_ITEM('',(#126640),#65103) ;
#1695=STYLED_ITEM('',(#126640),#65104) ;
#1696=STYLED_ITEM('',(#126640),#65105) ;
#1697=STYLED_ITEM('',(#126640),#65106) ;
#1698=STYLED_ITEM('',(#126641),#65107) ;
#1699=STYLED_ITEM('',(#126641),#65108) ;
#1700=STYLED_ITEM('',(#126641),#65109) ;
#1701=STYLED_ITEM('',(#126641),#65110) ;
#1702=STYLED_ITEM('',(#126641),#65111) ;
#1703=STYLED_ITEM('',(#126641),#65112) ;
#1704=STYLED_ITEM('',(#126641),#65113) ;
#1705=STYLED_ITEM('',(#126641),#65114) ;
#1706=STYLED_ITEM('',(#126641),#65115) ;
#1707=STYLED_ITEM('',(#126641),#65116) ;
#1708=STYLED_ITEM('',(#126641),#65117) ;
#1709=STYLED_ITEM('',(#126641),#65118) ;
#1710=STYLED_ITEM('',(#126641),#65119) ;
#1711=STYLED_ITEM('',(#126641),#65120) ;
#1712=STYLED_ITEM('',(#126641),#65121) ;
#1713=STYLED_ITEM('',(#126641),#65122) ;
#1714=STYLED_ITEM('',(#126641),#65123) ;
#1715=STYLED_ITEM('',(#126641),#65124) ;
#1716=STYLED_ITEM('',(#126641),#65125) ;
#1717=STYLED_ITEM('',(#126641),#65126) ;
#1718=STYLED_ITEM('',(#126640),#65127) ;
#1719=STYLED_ITEM('',(#126640),#65128) ;
#1720=STYLED_ITEM('',(#126640),#65129) ;
#1721=STYLED_ITEM('',(#126640),#65130) ;
#1722=STYLED_ITEM('',(#126640),#65131) ;
#1723=STYLED_ITEM('',(#126640),#65132) ;
#1724=STYLED_ITEM('',(#126640),#65133) ;
#1725=STYLED_ITEM('',(#126640),#65134) ;
#1726=STYLED_ITEM('',(#126640),#65135) ;
#1727=STYLED_ITEM('',(#126640),#65136) ;
#1728=STYLED_ITEM('',(#126640),#65137) ;
#1729=STYLED_ITEM('',(#126640),#65138) ;
#1730=STYLED_ITEM('',(#126640),#65139) ;
#1731=STYLED_ITEM('',(#126640),#65140) ;
#1732=STYLED_ITEM('',(#126640),#65141) ;
#1733=STYLED_ITEM('',(#126640),#65142) ;
#1734=STYLED_ITEM('',(#126640),#65143) ;
#1735=STYLED_ITEM('',(#126640),#65144) ;
#1736=STYLED_ITEM('',(#126640),#65145) ;
#1737=STYLED_ITEM('',(#126640),#65146) ;
#1738=STYLED_ITEM('',(#126640),#65147) ;
#1739=STYLED_ITEM('',(#126640),#65148) ;
#1740=STYLED_ITEM('',(#126640),#65149) ;
#1741=STYLED_ITEM('',(#126640),#65150) ;
#1742=STYLED_ITEM('',(#126640),#65151) ;
#1743=STYLED_ITEM('',(#126640),#65152) ;
#1744=STYLED_ITEM('',(#126640),#65153) ;
#1745=STYLED_ITEM('',(#126640),#65154) ;
#1746=STYLED_ITEM('',(#126640),#65155) ;
#1747=STYLED_ITEM('',(#126640),#65156) ;
#1748=STYLED_ITEM('',(#126640),#65157) ;
#1749=STYLED_ITEM('',(#126640),#65158) ;
#1750=STYLED_ITEM('',(#126640),#65159) ;
#1751=STYLED_ITEM('',(#126640),#65160) ;
#1752=STYLED_ITEM('',(#126640),#65161) ;
#1753=STYLED_ITEM('',(#126640),#65162) ;
#1754=STYLED_ITEM('',(#126640),#65163) ;
#1755=STYLED_ITEM('',(#126640),#65164) ;
#1756=STYLED_ITEM('',(#126640),#65165) ;
#1757=STYLED_ITEM('',(#126640),#65166) ;
#1758=STYLED_ITEM('',(#126640),#65167) ;
#1759=STYLED_ITEM('',(#126640),#65168) ;
#1760=STYLED_ITEM('',(#126640),#65169) ;
#1761=STYLED_ITEM('',(#126640),#65170) ;
#1762=STYLED_ITEM('',(#126640),#65171) ;
#1763=STYLED_ITEM('',(#126640),#65172) ;
#1764=STYLED_ITEM('',(#126640),#65173) ;
#1765=STYLED_ITEM('',(#126640),#65174) ;
#1766=STYLED_ITEM('',(#126640),#65175) ;
#1767=STYLED_ITEM('',(#126640),#65176) ;
#1768=STYLED_ITEM('',(#126640),#65177) ;
#1769=STYLED_ITEM('',(#126640),#65178) ;
#1770=STYLED_ITEM('',(#126640),#65179) ;
#1771=STYLED_ITEM('',(#126640),#65180) ;
#1772=STYLED_ITEM('',(#126640),#65181) ;
#1773=STYLED_ITEM('',(#126640),#65182) ;
#1774=STYLED_ITEM('',(#126640),#65183) ;
#1775=STYLED_ITEM('',(#126640),#65184) ;
#1776=STYLED_ITEM('',(#126640),#65185) ;
#1777=STYLED_ITEM('',(#126640),#65186) ;
#1778=STYLED_ITEM('',(#126640),#65187) ;
#1779=STYLED_ITEM('',(#126640),#65188) ;
#1780=STYLED_ITEM('',(#126640),#65189) ;
#1781=STYLED_ITEM('',(#126640),#65190) ;
#1782=STYLED_ITEM('',(#126640),#65191) ;
#1783=STYLED_ITEM('',(#126640),#65192) ;
#1784=STYLED_ITEM('',(#126640),#65193) ;
#1785=STYLED_ITEM('',(#126640),#65194) ;
#1786=STYLED_ITEM('',(#126640),#65195) ;
#1787=STYLED_ITEM('',(#126640),#65196) ;
#1788=STYLED_ITEM('',(#126640),#65197) ;
#1789=STYLED_ITEM('',(#126640),#65198) ;
#1790=STYLED_ITEM('',(#126640),#65199) ;
#1791=STYLED_ITEM('',(#126640),#65200) ;
#1792=STYLED_ITEM('',(#126640),#65201) ;
#1793=STYLED_ITEM('',(#126640),#65202) ;
#1794=STYLED_ITEM('',(#126640),#65203) ;
#1795=STYLED_ITEM('',(#126640),#65204) ;
#1796=STYLED_ITEM('',(#126640),#65205) ;
#1797=STYLED_ITEM('',(#126640),#65206) ;
#1798=STYLED_ITEM('',(#126640),#65207) ;
#1799=STYLED_ITEM('',(#126640),#65208) ;
#1800=STYLED_ITEM('',(#126640),#65209) ;
#1801=STYLED_ITEM('',(#126640),#65210) ;
#1802=STYLED_ITEM('',(#126640),#65211) ;
#1803=STYLED_ITEM('',(#126640),#65212) ;
#1804=STYLED_ITEM('',(#126640),#65213) ;
#1805=STYLED_ITEM('',(#126640),#65214) ;
#1806=STYLED_ITEM('',(#126640),#65215) ;
#1807=STYLED_ITEM('',(#126640),#65216) ;
#1808=STYLED_ITEM('',(#126640),#65217) ;
#1809=STYLED_ITEM('',(#126640),#65218) ;
#1810=STYLED_ITEM('',(#126640),#65219) ;
#1811=STYLED_ITEM('',(#126640),#65220) ;
#1812=STYLED_ITEM('',(#126640),#65221) ;
#1813=STYLED_ITEM('',(#126640),#65222) ;
#1814=STYLED_ITEM('',(#126640),#65223) ;
#1815=STYLED_ITEM('',(#126640),#65224) ;
#1816=STYLED_ITEM('',(#126640),#65225) ;
#1817=STYLED_ITEM('',(#126640),#65226) ;
#1818=STYLED_ITEM('',(#126640),#65227) ;
#1819=STYLED_ITEM('',(#126640),#65228) ;
#1820=STYLED_ITEM('',(#126640),#65229) ;
#1821=STYLED_ITEM('',(#126640),#65230) ;
#1822=STYLED_ITEM('',(#126640),#65231) ;
#1823=STYLED_ITEM('',(#126641),#65232) ;
#1824=STYLED_ITEM('',(#126641),#65233) ;
#1825=STYLED_ITEM('',(#126641),#65234) ;
#1826=STYLED_ITEM('',(#126641),#65235) ;
#1827=STYLED_ITEM('',(#126641),#65236) ;
#1828=STYLED_ITEM('',(#126641),#65237) ;
#1829=STYLED_ITEM('',(#126640),#65238) ;
#1830=STYLED_ITEM('',(#126641),#65239) ;
#1831=STYLED_ITEM('',(#126641),#65240) ;
#1832=STYLED_ITEM('',(#126641),#65241) ;
#1833=STYLED_ITEM('',(#126641),#65242) ;
#1834=STYLED_ITEM('',(#126641),#65243) ;
#1835=STYLED_ITEM('',(#126640),#65244) ;
#1836=STYLED_ITEM('',(#126640),#65245) ;
#1837=STYLED_ITEM('',(#126641),#65246) ;
#1838=STYLED_ITEM('',(#126641),#65247) ;
#1839=STYLED_ITEM('',(#126640),#65248) ;
#1840=STYLED_ITEM('',(#126641),#65249) ;
#1841=STYLED_ITEM('',(#126641),#65250) ;
#1842=STYLED_ITEM('',(#126641),#65251) ;
#1843=STYLED_ITEM('',(#126641),#65252) ;
#1844=STYLED_ITEM('',(#126641),#65253) ;
#1845=STYLED_ITEM('',(#126641),#65254) ;
#1846=STYLED_ITEM('',(#126641),#65255) ;
#1847=STYLED_ITEM('',(#126641),#65256) ;
#1848=STYLED_ITEM('',(#126640),#65257) ;
#1849=STYLED_ITEM('',(#126641),#65258) ;
#1850=STYLED_ITEM('',(#126641),#65259) ;
#1851=STYLED_ITEM('',(#126640),#65260) ;
#1852=STYLED_ITEM('',(#126641),#65261) ;
#1853=STYLED_ITEM('',(#126641),#65262) ;
#1854=STYLED_ITEM('',(#126641),#65263) ;
#1855=STYLED_ITEM('',(#126641),#65264) ;
#1856=STYLED_ITEM('',(#126640),#65265) ;
#1857=STYLED_ITEM('',(#126640),#65266) ;
#1858=STYLED_ITEM('',(#126641),#65267) ;
#1859=STYLED_ITEM('',(#126640),#65268) ;
#1860=STYLED_ITEM('',(#126640),#65269) ;
#1861=STYLED_ITEM('',(#126640),#65270) ;
#1862=STYLED_ITEM('',(#126640),#65271) ;
#1863=STYLED_ITEM('',(#126640),#65272) ;
#1864=STYLED_ITEM('',(#126640),#65273) ;
#1865=STYLED_ITEM('',(#126640),#65274) ;
#1866=STYLED_ITEM('',(#126640),#65275) ;
#1867=STYLED_ITEM('',(#126640),#65276) ;
#1868=STYLED_ITEM('',(#126640),#65277) ;
#1869=STYLED_ITEM('',(#126640),#65278) ;
#1870=STYLED_ITEM('',(#126640),#65279) ;
#1871=STYLED_ITEM('',(#126640),#65280) ;
#1872=STYLED_ITEM('',(#126640),#65281) ;
#1873=STYLED_ITEM('',(#126640),#65282) ;
#1874=STYLED_ITEM('',(#126640),#65283) ;
#1875=STYLED_ITEM('',(#126640),#65284) ;
#1876=STYLED_ITEM('',(#126640),#65285) ;
#1877=STYLED_ITEM('',(#126640),#65286) ;
#1878=STYLED_ITEM('',(#126640),#65287) ;
#1879=STYLED_ITEM('',(#126640),#65288) ;
#1880=STYLED_ITEM('',(#126640),#65289) ;
#1881=STYLED_ITEM('',(#126640),#65290) ;
#1882=STYLED_ITEM('',(#126640),#65291) ;
#1883=STYLED_ITEM('',(#126640),#65292) ;
#1884=STYLED_ITEM('',(#126640),#65293) ;
#1885=STYLED_ITEM('',(#126640),#65294) ;
#1886=STYLED_ITEM('',(#126640),#65295) ;
#1887=STYLED_ITEM('',(#126640),#65296) ;
#1888=STYLED_ITEM('',(#126640),#65297) ;
#1889=STYLED_ITEM('',(#126640),#65298) ;
#1890=STYLED_ITEM('',(#126640),#65299) ;
#1891=STYLED_ITEM('',(#126640),#65300) ;
#1892=STYLED_ITEM('',(#126640),#65301) ;
#1893=STYLED_ITEM('',(#126640),#65302) ;
#1894=STYLED_ITEM('',(#126640),#65303) ;
#1895=STYLED_ITEM('',(#126640),#65304) ;
#1896=STYLED_ITEM('',(#126640),#65305) ;
#1897=STYLED_ITEM('',(#126640),#65306) ;
#1898=STYLED_ITEM('',(#126640),#65307) ;
#1899=STYLED_ITEM('',(#126640),#65308) ;
#1900=STYLED_ITEM('',(#126640),#65309) ;
#1901=STYLED_ITEM('',(#126640),#65310) ;
#1902=STYLED_ITEM('',(#126640),#65311) ;
#1903=STYLED_ITEM('',(#126640),#65312) ;
#1904=STYLED_ITEM('',(#126640),#65313) ;
#1905=STYLED_ITEM('',(#126640),#65314) ;
#1906=STYLED_ITEM('',(#126641),#65315) ;
#1907=STYLED_ITEM('',(#126641),#65316) ;
#1908=STYLED_ITEM('',(#126641),#65317) ;
#1909=STYLED_ITEM('',(#126641),#65318) ;
#1910=STYLED_ITEM('',(#126641),#65319) ;
#1911=STYLED_ITEM('',(#126641),#65320) ;
#1912=STYLED_ITEM('',(#126641),#65321) ;
#1913=STYLED_ITEM('',(#126641),#65322) ;
#1914=STYLED_ITEM('',(#126641),#65323) ;
#1915=STYLED_ITEM('',(#126641),#65324) ;
#1916=STYLED_ITEM('',(#126641),#65325) ;
#1917=STYLED_ITEM('',(#126641),#65326) ;
#1918=STYLED_ITEM('',(#126641),#65327) ;
#1919=STYLED_ITEM('',(#126641),#65328) ;
#1920=STYLED_ITEM('',(#126641),#65329) ;
#1921=STYLED_ITEM('',(#126641),#65330) ;
#1922=STYLED_ITEM('',(#126640),#65331) ;
#1923=STYLED_ITEM('',(#126640),#65332) ;
#1924=STYLED_ITEM('',(#126640),#65333) ;
#1925=STYLED_ITEM('',(#126640),#65334) ;
#1926=STYLED_ITEM('',(#126640),#65335) ;
#1927=STYLED_ITEM('',(#126640),#65336) ;
#1928=STYLED_ITEM('',(#126640),#65337) ;
#1929=STYLED_ITEM('',(#126640),#65338) ;
#1930=STYLED_ITEM('',(#126640),#65339) ;
#1931=STYLED_ITEM('',(#126639),#4177) ;
#4173=MANIFOLD_SOLID_BREP('Body1',#67687) ;
#4174=MANIFOLD_SOLID_BREP('Body2',#67688) ;
#4175=MANIFOLD_SOLID_BREP('Body3',#67689) ;
#4176=MANIFOLD_SOLID_BREP('Body4',#67690) ;
#4177=MANIFOLD_SOLID_BREP('Body5',#67691) ;
#4206=SPHERICAL_SURFACE('',#68975,0.1) ;
#4207=SPHERICAL_SURFACE('',#68986,0.1) ;
#4208=SPHERICAL_SURFACE('',#69004,0.1) ;
#4209=SPHERICAL_SURFACE('',#69010,0.1) ;
#4210=SPHERICAL_SURFACE('',#69023,0.1) ;
#4211=SPHERICAL_SURFACE('',#69037,0.1) ;
#4212=SPHERICAL_SURFACE('',#69042,0.1) ;
#4213=SPHERICAL_SURFACE('',#69063,0.1) ;
#4214=SPHERICAL_SURFACE('',#69081,0.1) ;
#4215=SPHERICAL_SURFACE('',#69083,0.1) ;
#4216=SPHERICAL_SURFACE('',#69090,0.1) ;
#4217=SPHERICAL_SURFACE('',#69105,0.1) ;
#4218=SPHERICAL_SURFACE('',#69118,0.1) ;
#4219=SPHERICAL_SURFACE('',#69134,0.1) ;
#4220=SPHERICAL_SURFACE('',#69156,0.1) ;
#4221=SPHERICAL_SURFACE('',#69159,0.1) ;
#4222=SPHERICAL_SURFACE('',#69175,0.1) ;
#4223=SPHERICAL_SURFACE('',#69177,0.1) ;
#4224=SPHERICAL_SURFACE('',#69203,0.1) ;
#4225=SPHERICAL_SURFACE('',#69218,0.1) ;
#4226=SPHERICAL_SURFACE('',#69220,0.1) ;
#4227=SPHERICAL_SURFACE('',#69226,0.1) ;
#4228=SPHERICAL_SURFACE('',#69247,0.1) ;
#4229=SPHERICAL_SURFACE('',#69253,0.1) ;
#4230=SPHERICAL_SURFACE('',#69265,0.1) ;
#4231=SPHERICAL_SURFACE('',#69267,0.1) ;
#4232=SPHERICAL_SURFACE('',#69274,0.1) ;
#4233=SPHERICAL_SURFACE('',#69280,0.1) ;
#4234=SPHERICAL_SURFACE('',#69288,0.1) ;
#4235=SPHERICAL_SURFACE('',#69294,0.1) ;
#4236=SPHERICAL_SURFACE('',#69315,0.1) ;
#4237=SPHERICAL_SURFACE('',#69322,0.1) ;
#4238=SPHERICAL_SURFACE('',#69340,0.1) ;
#4239=SPHERICAL_SURFACE('',#69343,0.1) ;
#4240=SPHERICAL_SURFACE('',#69344,0.1) ;
#4241=SPHERICAL_SURFACE('',#69351,0.1) ;
#4242=SPHERICAL_SURFACE('',#69353,0.1) ;
#4243=SPHERICAL_SURFACE('',#69359,0.1) ;
#4244=SPHERICAL_SURFACE('',#69360,0.1) ;
#4245=SPHERICAL_SURFACE('',#69367,0.1) ;
#4246=SPHERICAL_SURFACE('',#69369,0.1) ;
#4247=SPHERICAL_SURFACE('',#69375,0.1) ;
#4248=SPHERICAL_SURFACE('',#69378,0.1) ;
#4249=SPHERICAL_SURFACE('',#69381,0.1) ;
#4250=SPHERICAL_SURFACE('',#69585,0.1) ;
#4251=SPHERICAL_SURFACE('',#69596,0.1) ;
#4252=SPHERICAL_SURFACE('',#69614,0.1) ;
#4253=SPHERICAL_SURFACE('',#69620,0.1) ;
#4254=SPHERICAL_SURFACE('',#69633,0.1) ;
#4255=SPHERICAL_SURFACE('',#69647,0.1) ;
#4256=SPHERICAL_SURFACE('',#69652,0.1) ;
#4257=SPHERICAL_SURFACE('',#69673,0.1) ;
#4258=SPHERICAL_SURFACE('',#69691,0.1) ;
#4259=SPHERICAL_SURFACE('',#69693,0.1) ;
#4260=SPHERICAL_SURFACE('',#69700,0.1) ;
#4261=SPHERICAL_SURFACE('',#69715,0.1) ;
#4262=SPHERICAL_SURFACE('',#69728,0.1) ;
#4263=SPHERICAL_SURFACE('',#69744,0.1) ;
#4264=SPHERICAL_SURFACE('',#69766,0.1) ;
#4265=SPHERICAL_SURFACE('',#69769,0.1) ;
#4266=SPHERICAL_SURFACE('',#69785,0.1) ;
#4267=SPHERICAL_SURFACE('',#69787,0.1) ;
#4268=SPHERICAL_SURFACE('',#69813,0.1) ;
#4269=SPHERICAL_SURFACE('',#69828,0.1) ;
#4270=SPHERICAL_SURFACE('',#69830,0.1) ;
#4271=SPHERICAL_SURFACE('',#69836,0.1) ;
#4272=SPHERICAL_SURFACE('',#69857,0.1) ;
#4273=SPHERICAL_SURFACE('',#69863,0.1) ;
#4274=SPHERICAL_SURFACE('',#69875,0.1) ;
#4275=SPHERICAL_SURFACE('',#69877,0.1) ;
#4276=SPHERICAL_SURFACE('',#69884,0.1) ;
#4277=SPHERICAL_SURFACE('',#69890,0.1) ;
#4278=SPHERICAL_SURFACE('',#69898,0.1) ;
#4279=SPHERICAL_SURFACE('',#69904,0.1) ;
#4280=SPHERICAL_SURFACE('',#69925,0.1) ;
#4281=SPHERICAL_SURFACE('',#69932,0.1) ;
#4282=SPHERICAL_SURFACE('',#69950,0.1) ;
#4283=SPHERICAL_SURFACE('',#69953,0.1) ;
#4284=SPHERICAL_SURFACE('',#69954,0.1) ;
#4285=SPHERICAL_SURFACE('',#69961,0.1) ;
#4286=SPHERICAL_SURFACE('',#69963,0.1) ;
#4287=SPHERICAL_SURFACE('',#69969,0.1) ;
#4288=SPHERICAL_SURFACE('',#69970,0.1) ;
#4289=SPHERICAL_SURFACE('',#69977,0.1) ;
#4290=SPHERICAL_SURFACE('',#69979,0.1) ;
#4291=SPHERICAL_SURFACE('',#69985,0.1) ;
#4292=SPHERICAL_SURFACE('',#69988,0.1) ;
#4293=SPHERICAL_SURFACE('',#69991,0.1) ;
#4294=SPHERICAL_SURFACE('',#70195,0.1) ;
#4295=SPHERICAL_SURFACE('',#70206,0.1) ;
#4296=SPHERICAL_SURFACE('',#70224,0.1) ;
#4297=SPHERICAL_SURFACE('',#70230,0.1) ;
#4298=SPHERICAL_SURFACE('',#70243,0.1) ;
#4299=SPHERICAL_SURFACE('',#70257,0.1) ;
#4300=SPHERICAL_SURFACE('',#70262,0.1) ;
#4301=SPHERICAL_SURFACE('',#70283,0.1) ;
#4302=SPHERICAL_SURFACE('',#70301,0.1) ;
#4303=SPHERICAL_SURFACE('',#70303,0.1) ;
#4304=SPHERICAL_SURFACE('',#70310,0.1) ;
#4305=SPHERICAL_SURFACE('',#70325,0.1) ;
#4306=SPHERICAL_SURFACE('',#70338,0.1) ;
#4307=SPHERICAL_SURFACE('',#70354,0.1) ;
#4308=SPHERICAL_SURFACE('',#70376,0.1) ;
#4309=SPHERICAL_SURFACE('',#70379,0.1) ;
#4310=SPHERICAL_SURFACE('',#70395,0.1) ;
#4311=SPHERICAL_SURFACE('',#70397,0.1) ;
#4312=SPHERICAL_SURFACE('',#70423,0.1) ;
#4313=SPHERICAL_SURFACE('',#70438,0.1) ;
#4314=SPHERICAL_SURFACE('',#70440,0.1) ;
#4315=SPHERICAL_SURFACE('',#70446,0.1) ;
#4316=SPHERICAL_SURFACE('',#70467,0.1) ;
#4317=SPHERICAL_SURFACE('',#70473,0.1) ;
#4318=SPHERICAL_SURFACE('',#70485,0.1) ;
#4319=SPHERICAL_SURFACE('',#70487,0.1) ;
#4320=SPHERICAL_SURFACE('',#70494,0.1) ;
#4321=SPHERICAL_SURFACE('',#70500,0.1) ;
#4322=SPHERICAL_SURFACE('',#70508,0.1) ;
#4323=SPHERICAL_SURFACE('',#70514,0.1) ;
#4324=SPHERICAL_SURFACE('',#70535,0.1) ;
#4325=SPHERICAL_SURFACE('',#70542,0.1) ;
#4326=SPHERICAL_SURFACE('',#70560,0.1) ;
#4327=SPHERICAL_SURFACE('',#70563,0.1) ;
#4328=SPHERICAL_SURFACE('',#70564,0.1) ;
#4329=SPHERICAL_SURFACE('',#70571,0.1) ;
#4330=SPHERICAL_SURFACE('',#70573,0.1) ;
#4331=SPHERICAL_SURFACE('',#70579,0.1) ;
#4332=SPHERICAL_SURFACE('',#70580,0.1) ;
#4333=SPHERICAL_SURFACE('',#70587,0.1) ;
#4334=SPHERICAL_SURFACE('',#70589,0.1) ;
#4335=SPHERICAL_SURFACE('',#70595,0.1) ;
#4336=SPHERICAL_SURFACE('',#70598,0.1) ;
#4337=SPHERICAL_SURFACE('',#70601,0.1) ;
#4338=SPHERICAL_SURFACE('',#70805,0.1) ;
#4339=SPHERICAL_SURFACE('',#70816,0.1) ;
#4340=SPHERICAL_SURFACE('',#70834,0.1) ;
#4341=SPHERICAL_SURFACE('',#70840,0.1) ;
#4342=SPHERICAL_SURFACE('',#70853,0.1) ;
#4343=SPHERICAL_SURFACE('',#70867,0.1) ;
#4344=SPHERICAL_SURFACE('',#70872,0.1) ;
#4345=SPHERICAL_SURFACE('',#70893,0.1) ;
#4346=SPHERICAL_SURFACE('',#70911,0.1) ;
#4347=SPHERICAL_SURFACE('',#70913,0.1) ;
#4348=SPHERICAL_SURFACE('',#70920,0.1) ;
#4349=SPHERICAL_SURFACE('',#70935,0.1) ;
#4350=SPHERICAL_SURFACE('',#70948,0.1) ;
#4351=SPHERICAL_SURFACE('',#70964,0.1) ;
#4352=SPHERICAL_SURFACE('',#70986,0.1) ;
#4353=SPHERICAL_SURFACE('',#70989,0.1) ;
#4354=SPHERICAL_SURFACE('',#71005,0.1) ;
#4355=SPHERICAL_SURFACE('',#71007,0.1) ;
#4356=SPHERICAL_SURFACE('',#71033,0.1) ;
#4357=SPHERICAL_SURFACE('',#71048,0.1) ;
#4358=SPHERICAL_SURFACE('',#71050,0.1) ;
#4359=SPHERICAL_SURFACE('',#71056,0.1) ;
#4360=SPHERICAL_SURFACE('',#71077,0.1) ;
#4361=SPHERICAL_SURFACE('',#71083,0.1) ;
#4362=SPHERICAL_SURFACE('',#71095,0.1) ;
#4363=SPHERICAL_SURFACE('',#71097,0.1) ;
#4364=SPHERICAL_SURFACE('',#71104,0.1) ;
#4365=SPHERICAL_SURFACE('',#71110,0.1) ;
#4366=SPHERICAL_SURFACE('',#71118,0.1) ;
#4367=SPHERICAL_SURFACE('',#71124,0.1) ;
#4368=SPHERICAL_SURFACE('',#71145,0.1) ;
#4369=SPHERICAL_SURFACE('',#71152,0.1) ;
#4370=SPHERICAL_SURFACE('',#71170,0.1) ;
#4371=SPHERICAL_SURFACE('',#71173,0.1) ;
#4372=SPHERICAL_SURFACE('',#71174,0.1) ;
#4373=SPHERICAL_SURFACE('',#71181,0.1) ;
#4374=SPHERICAL_SURFACE('',#71183,0.1) ;
#4375=SPHERICAL_SURFACE('',#71189,0.1) ;
#4376=SPHERICAL_SURFACE('',#71190,0.1) ;
#4377=SPHERICAL_SURFACE('',#71197,0.1) ;
#4378=SPHERICAL_SURFACE('',#71199,0.1) ;
#4379=SPHERICAL_SURFACE('',#71205,0.1) ;
#4380=SPHERICAL_SURFACE('',#71208,0.1) ;
#4381=SPHERICAL_SURFACE('',#71211,0.1) ;
#4382=SPHERICAL_SURFACE('',#71415,0.1) ;
#4383=SPHERICAL_SURFACE('',#71426,0.1) ;
#4384=SPHERICAL_SURFACE('',#71444,0.1) ;
#4385=SPHERICAL_SURFACE('',#71450,0.1) ;
#4386=SPHERICAL_SURFACE('',#71463,0.1) ;
#4387=SPHERICAL_SURFACE('',#71477,0.1) ;
#4388=SPHERICAL_SURFACE('',#71482,0.1) ;
#4389=SPHERICAL_SURFACE('',#71503,0.1) ;
#4390=SPHERICAL_SURFACE('',#71521,0.1) ;
#4391=SPHERICAL_SURFACE('',#71523,0.1) ;
#4392=SPHERICAL_SURFACE('',#71530,0.1) ;
#4393=SPHERICAL_SURFACE('',#71545,0.1) ;
#4394=SPHERICAL_SURFACE('',#71558,0.1) ;
#4395=SPHERICAL_SURFACE('',#71574,0.1) ;
#4396=SPHERICAL_SURFACE('',#71596,0.1) ;
#4397=SPHERICAL_SURFACE('',#71599,0.1) ;
#4398=SPHERICAL_SURFACE('',#71615,0.1) ;
#4399=SPHERICAL_SURFACE('',#71617,0.1) ;
#4400=SPHERICAL_SURFACE('',#71643,0.1) ;
#4401=SPHERICAL_SURFACE('',#71658,0.1) ;
#4402=SPHERICAL_SURFACE('',#71660,0.1) ;
#4403=SPHERICAL_SURFACE('',#71666,0.1) ;
#4404=SPHERICAL_SURFACE('',#71687,0.1) ;
#4405=SPHERICAL_SURFACE('',#71693,0.1) ;
#4406=SPHERICAL_SURFACE('',#71705,0.1) ;
#4407=SPHERICAL_SURFACE('',#71707,0.1) ;
#4408=SPHERICAL_SURFACE('',#71714,0.1) ;
#4409=SPHERICAL_SURFACE('',#71720,0.1) ;
#4410=SPHERICAL_SURFACE('',#71728,0.1) ;
#4411=SPHERICAL_SURFACE('',#71734,0.1) ;
#4412=SPHERICAL_SURFACE('',#71755,0.1) ;
#4413=SPHERICAL_SURFACE('',#71762,0.1) ;
#4414=SPHERICAL_SURFACE('',#71780,0.1) ;
#4415=SPHERICAL_SURFACE('',#71783,0.1) ;
#4416=SPHERICAL_SURFACE('',#71784,0.1) ;
#4417=SPHERICAL_SURFACE('',#71791,0.1) ;
#4418=SPHERICAL_SURFACE('',#71793,0.1) ;
#4419=SPHERICAL_SURFACE('',#71799,0.1) ;
#4420=SPHERICAL_SURFACE('',#71800,0.1) ;
#4421=SPHERICAL_SURFACE('',#71807,0.1) ;
#4422=SPHERICAL_SURFACE('',#71809,0.1) ;
#4423=SPHERICAL_SURFACE('',#71815,0.1) ;
#4424=SPHERICAL_SURFACE('',#71818,0.1) ;
#4425=SPHERICAL_SURFACE('',#71821,0.1) ;
#4848=ELLIPSE('',#68779,0.0809537756926331,0.0568957747646781) ;
#4849=ELLIPSE('',#68781,0.100391322057661,0.0922176205486333) ;
#4850=ELLIPSE('',#68783,0.113377229734873,0.0929834630466229) ;
#4851=ELLIPSE('',#68785,0.223917610441093,0.216142984077905) ;
#4852=ELLIPSE('',#68812,0.121362326126752,0.103679679516972) ;
#4853=ELLIPSE('',#68858,0.0267230623193982,0.018714321485574) ;
#4854=ELLIPSE('',#68933,0.199399949088646,0.187786165419954) ;
#4855=ELLIPSE('',#68934,0.199099081511402,0.194604184805257) ;
#4856=ELLIPSE('',#68935,0.201529676353064,0.190129099365806) ;
#4857=ELLIPSE('',#69047,0.239594752729702,0.10422367698916) ;
#4858=ELLIPSE('',#69049,0.239471272532979,0.104190452488474) ;
#4859=ELLIPSE('',#69053,0.239471272536741,0.104190452489493) ;
#4860=ELLIPSE('',#69054,0.239594752729914,0.104223676989188) ;
#4861=ELLIPSE('',#69056,0.239594752728089,0.104223676988759) ;
#4862=ELLIPSE('',#69057,0.239471272538988,0.104190452490065) ;
#4863=ELLIPSE('',#69067,0.239471272536946,0.10419045248958) ;
#4864=ELLIPSE('',#69070,0.239594752723292,0.104223676987398) ;
#4865=ELLIPSE('',#69075,0.14142135623732,0.100000000000004) ;
#4866=ELLIPSE('',#69111,0.141421356237308,0.0999999999999974) ;
#4867=ELLIPSE('',#69284,0.097021650614293,0.0903313095003513) ;
#4868=ELLIPSE('',#69297,0.0951423444618738,0.0854984019584871) ;
#4869=ELLIPSE('',#69330,0.104054226887004,0.0879291201711123) ;
#4870=ELLIPSE('',#69335,0.104149278807314,0.0880903460854034) ;
#4871=ELLIPSE('',#69383,0.107757087311018,0.0995628413317711) ;
#4872=ELLIPSE('',#69387,0.107757092531729,0.0995628480425321) ;
#4873=ELLIPSE('',#69389,0.0809537320004613,0.0568957137241202) ;
#4874=ELLIPSE('',#69391,0.10039132205649,0.0922176205475765) ;
#4875=ELLIPSE('',#69393,0.113377229735081,0.0929834630467951) ;
#4876=ELLIPSE('',#69395,0.223917611676684,0.216142984782922) ;
#4877=ELLIPSE('',#69422,0.121362326117636,0.10367967951289) ;
#4878=ELLIPSE('',#69468,0.0267230623194912,0.0187143214857259) ;
#4879=ELLIPSE('',#69543,0.19939994910193,0.187786165441026) ;
#4880=ELLIPSE('',#69544,0.199099083267325,0.194604186778209) ;
#4881=ELLIPSE('',#69545,0.201529680428943,0.190129102907909) ;
#4882=ELLIPSE('',#69657,0.23959475272645,0.104223676988348) ;
#4883=ELLIPSE('',#69659,0.23947127252868,0.104190452487282) ;
#4884=ELLIPSE('',#69663,0.239471272523845,0.104190452486007) ;
#4885=ELLIPSE('',#69664,0.239594752719793,0.104223676986401) ;
#4886=ELLIPSE('',#69666,0.239594752718529,0.104223676986274) ;
#4887=ELLIPSE('',#69667,0.239471272528616,0.10419045248741) ;
#4888=ELLIPSE('',#69677,0.239471272535145,0.104190452489145) ;
#4889=ELLIPSE('',#69680,0.239594752726162,0.104223676988029) ;
#4890=ELLIPSE('',#69685,0.141421356237384,0.100000000000052) ;
#4891=ELLIPSE('',#69721,0.141421356237348,0.100000000000022) ;
#4892=ELLIPSE('',#69894,0.0970216506148374,0.0903313095008944) ;
#4893=ELLIPSE('',#69907,0.0951423444627011,0.0854984019587331) ;
#4894=ELLIPSE('',#69940,0.104054227208667,0.0879291207156953) ;
#4895=ELLIPSE('',#69945,0.10414927820719,0.0880903450688493) ;
#4896=ELLIPSE('',#69993,0.107757087370127,0.0995628414091742) ;
#4897=ELLIPSE('',#69997,0.107757092560179,0.0995628480825893) ;
#4898=ELLIPSE('',#69999,0.0809537150131407,0.0568956899993869) ;
#4899=ELLIPSE('',#70001,0.100391322056624,0.0922176205478182) ;
#4900=ELLIPSE('',#70003,0.11337722973501,0.0929834630467645) ;
#4901=ELLIPSE('',#70005,0.223917608546806,0.216142982996952) ;
#4902=ELLIPSE('',#70032,0.121362326128888,0.103679679517888) ;
#4903=ELLIPSE('',#70078,0.0267230623192196,0.018714321485282) ;
#4904=ELLIPSE('',#70153,0.199399948440172,0.187786164286963) ;
#4905=ELLIPSE('',#70154,0.19909908761073,0.194604191600843) ;
#4906=ELLIPSE('',#70155,0.201529663713424,0.190129088416408) ;
#4907=ELLIPSE('',#70267,0.239594752713108,0.104223676985137) ;
#4908=ELLIPSE('',#70269,0.239471272519053,0.10419045248485) ;
#4909=ELLIPSE('',#70273,0.239471272510231,0.104190452482661) ;
#4910=ELLIPSE('',#70274,0.239594752744898,0.104223676993171) ;
#4911=ELLIPSE('',#70276,0.239594752804206,0.104223677008282) ;
#4912=ELLIPSE('',#70277,0.239471272554278,0.104190452494285) ;
#4913=ELLIPSE('',#70287,0.239471272532213,0.10419045248842) ;
#4914=ELLIPSE('',#70290,0.239594752728355,0.104223676988648) ;
#4915=ELLIPSE('',#70295,0.141421356237532,0.100000000000142) ;
#4916=ELLIPSE('',#70331,0.141421356237283,0.0999999999999815) ;
#4917=ELLIPSE('',#70504,0.097021650613777,0.0903313094997654) ;
#4918=ELLIPSE('',#70517,0.0951423444666796,0.0854984019616217) ;
#4919=ELLIPSE('',#70550,0.104054228132819,0.0879291222802139) ;
#4920=ELLIPSE('',#70555,0.104149278173856,0.0880903450126872) ;
#4921=ELLIPSE('',#70603,0.107757087301598,0.0995628413185721) ;
#4922=ELLIPSE('',#70607,0.107757092599453,0.0995628481342478) ;
#4923=ELLIPSE('',#70609,0.0809537387857418,0.0568957231926316) ;
#4924=ELLIPSE('',#70611,0.10039132205777,0.092217620548776) ;
#4925=ELLIPSE('',#70613,0.113377229735182,0.0929834630469383) ;
#4926=ELLIPSE('',#70615,0.223917610559684,0.216142984153567) ;
#4927=ELLIPSE('',#70642,0.121362326124367,0.103679679515825) ;
#4928=ELLIPSE('',#70688,0.026723062320724,0.0187143214878425) ;
#4929=ELLIPSE('',#70763,0.199399948145838,0.187786163779416) ;
#4930=ELLIPSE('',#70764,0.199099054947908,0.194604155307638) ;
#4931=ELLIPSE('',#70765,0.201529689838765,0.190129111016764) ;
#4932=ELLIPSE('',#70877,0.239594752707325,0.104223676983421) ;
#4933=ELLIPSE('',#70879,0.239471272497778,0.104190452479804) ;
#4934=ELLIPSE('',#70883,0.239471272515141,0.104190452483868) ;
#4935=ELLIPSE('',#70884,0.239594752753233,0.10422367699537) ;
#4936=ELLIPSE('',#70886,0.239594752695653,0.104223676980216) ;
#4937=ELLIPSE('',#70887,0.239471272540246,0.10419045249087) ;
#4938=ELLIPSE('',#70897,0.239471272540333,0.104190452490452) ;
#4939=ELLIPSE('',#70900,0.239594752729595,0.10422367698884) ;
#4940=ELLIPSE('',#70905,0.141421356237619,0.100000000000176) ;
#4941=ELLIPSE('',#70941,0.14142135623723,0.0999999999999436) ;
#4942=ELLIPSE('',#71114,0.0970216506126833,0.0903313094987464) ;
#4943=ELLIPSE('',#71127,0.0951423444690284,0.0854984019628288) ;
#4944=ELLIPSE('',#71160,0.104054227520181,0.0879291212428128) ;
#4945=ELLIPSE('',#71165,0.104149278514073,0.0880903455891445) ;
#4946=ELLIPSE('',#71213,0.107757082275427,0.0995628348635113) ;
#4947=ELLIPSE('',#71217,0.107757087537776,0.0995628416311376) ;
#4948=ELLIPSE('',#71219,0.0809537573847507,0.0568957491961901) ;
#4949=ELLIPSE('',#71221,0.100391322057649,0.0922176205486138) ;
#4950=ELLIPSE('',#71223,0.113377229735276,0.0929834630468768) ;
#4951=ELLIPSE('',#71225,0.22391761061454,0.216142984175044) ;
#4952=ELLIPSE('',#71252,0.121362326124309,0.103679679515832) ;
#4953=ELLIPSE('',#71298,0.0267230623209999,0.0187143214882515) ;
#4954=ELLIPSE('',#71373,0.199399950265729,0.187786167479822) ;
#4955=ELLIPSE('',#71374,0.199099063433144,0.194604164642533) ;
#4956=ELLIPSE('',#71375,0.201529637184767,0.190129065311698) ;
#4957=ELLIPSE('',#71487,0.239594752727344,0.104223676988237) ;
#4958=ELLIPSE('',#71489,0.239471272520672,0.104190452485608) ;
#4959=ELLIPSE('',#71493,0.239471272484206,0.104190452475713) ;
#4960=ELLIPSE('',#71494,0.239594752698159,0.104223676980846) ;
#4961=ELLIPSE('',#71496,0.239594752701739,0.104223676981937) ;
#4962=ELLIPSE('',#71497,0.239471272477747,0.104190452474144) ;
#4963=ELLIPSE('',#71507,0.239471272525481,0.104190452486512) ;
#4964=ELLIPSE('',#71510,0.239594752715511,0.104223676985684) ;
#4965=ELLIPSE('',#71515,0.141421356237514,0.100000000000115) ;
#4966=ELLIPSE('',#71551,0.141421356237124,0.0999999999998686) ;
#4967=ELLIPSE('',#71724,0.0970216506112587,0.0903313094971849) ;
#4968=ELLIPSE('',#71737,0.0951423444596952,0.0854984019571455) ;
#4969=ELLIPSE('',#71770,0.104054227648042,0.0879291214596957) ;
#4970=ELLIPSE('',#71775,0.104149278744974,0.0880903459807416) ;
#4971=ELLIPSE('',#71823,0.107757087317353,0.0995628413381732) ;
#4972=ELLIPSE('',#71827,0.107757082308246,0.0995628349076281) ;
#5019=FACE_BOUND('',#20908,.T.) ;
#5020=FACE_BOUND('',#20920,.T.) ;
#5021=FACE_BOUND('',#21199,.T.) ;
#5022=FACE_BOUND('',#21211,.T.) ;
#5023=FACE_BOUND('',#21490,.T.) ;
#5024=FACE_BOUND('',#21502,.T.) ;
#5025=FACE_BOUND('',#21781,.T.) ;
#5026=FACE_BOUND('',#21793,.T.) ;
#5027=FACE_BOUND('',#22072,.T.) ;
#5028=FACE_BOUND('',#22084,.T.) ;
#5153=PLANE('',#68811) ;
#5154=PLANE('',#68813) ;
#5155=PLANE('',#68814) ;
#5156=PLANE('',#68815) ;
#5157=PLANE('',#68816) ;
#5158=PLANE('',#68817) ;
#5159=PLANE('',#68818) ;
#5160=PLANE('',#68820) ;
#5161=PLANE('',#68837) ;
#5162=PLANE('',#68854) ;
#5163=PLANE('',#68855) ;
#5164=PLANE('',#68856) ;
#5165=PLANE('',#68857) ;
#5166=PLANE('',#68859) ;
#5167=PLANE('',#68860) ;
#5168=PLANE('',#68861) ;
#5169=PLANE('',#68864) ;
#5170=PLANE('',#68878) ;
#5171=PLANE('',#68881) ;
#5172=PLANE('',#68884) ;
#5173=PLANE('',#68886) ;
#5174=PLANE('',#68888) ;
#5175=PLANE('',#68889) ;
#5176=PLANE('',#68890) ;
#5177=PLANE('',#68891) ;
#5178=PLANE('',#68892) ;
#5179=PLANE('',#68893) ;
#5180=PLANE('',#68894) ;
#5181=PLANE('',#68899) ;
#5182=PLANE('',#68903) ;
#5183=PLANE('',#68904) ;
#5184=PLANE('',#68911) ;
#5185=PLANE('',#68912) ;
#5186=PLANE('',#68913) ;
#5187=PLANE('',#68917) ;
#5188=PLANE('',#68919) ;
#5189=PLANE('',#68923) ;
#5190=PLANE('',#68927) ;
#5191=PLANE('',#68928) ;
#5192=PLANE('',#68929) ;
#5193=PLANE('',#68931) ;
#5194=PLANE('',#68932) ;
#5195=PLANE('',#68936) ;
#5196=PLANE('',#68937) ;
#5197=PLANE('',#68938) ;
#5198=PLANE('',#68939) ;
#5199=PLANE('',#68940) ;
#5200=PLANE('',#68941) ;
#5201=PLANE('',#68942) ;
#5202=PLANE('',#68943) ;
#5203=PLANE('',#68944) ;
#5204=PLANE('',#68947) ;
#5205=PLANE('',#68953) ;
#5206=PLANE('',#68954) ;
#5207=PLANE('',#68955) ;
#5208=PLANE('',#68956) ;
#5209=PLANE('',#68957) ;
#5210=PLANE('',#68961) ;
#5211=PLANE('',#68962) ;
#5212=PLANE('',#68963) ;
#5213=PLANE('',#68964) ;
#5214=PLANE('',#68965) ;
#5215=PLANE('',#68971) ;
#5216=PLANE('',#69421) ;
#5217=PLANE('',#69423) ;
#5218=PLANE('',#69424) ;
#5219=PLANE('',#69425) ;
#5220=PLANE('',#69426) ;
#5221=PLANE('',#69427) ;
#5222=PLANE('',#69428) ;
#5223=PLANE('',#69430) ;
#5224=PLANE('',#69447) ;
#5225=PLANE('',#69464) ;
#5226=PLANE('',#69465) ;
#5227=PLANE('',#69466) ;
#5228=PLANE('',#69467) ;
#5229=PLANE('',#69469) ;
#5230=PLANE('',#69470) ;
#5231=PLANE('',#69471) ;
#5232=PLANE('',#69474) ;
#5233=PLANE('',#69488) ;
#5234=PLANE('',#69491) ;
#5235=PLANE('',#69494) ;
#5236=PLANE('',#69496) ;
#5237=PLANE('',#69498) ;
#5238=PLANE('',#69499) ;
#5239=PLANE('',#69500) ;
#5240=PLANE('',#69501) ;
#5241=PLANE('',#69502) ;
#5242=PLANE('',#69503) ;
#5243=PLANE('',#69504) ;
#5244=PLANE('',#69509) ;
#5245=PLANE('',#69513) ;
#5246=PLANE('',#69514) ;
#5247=PLANE('',#69521) ;
#5248=PLANE('',#69522) ;
#5249=PLANE('',#69523) ;
#5250=PLANE('',#69527) ;
#5251=PLANE('',#69529) ;
#5252=PLANE('',#69533) ;
#5253=PLANE('',#69537) ;
#5254=PLANE('',#69538) ;
#5255=PLANE('',#69539) ;
#5256=PLANE('',#69541) ;
#5257=PLANE('',#69542) ;
#5258=PLANE('',#69546) ;
#5259=PLANE('',#69547) ;
#5260=PLANE('',#69548) ;
#5261=PLANE('',#69549) ;
#5262=PLANE('',#69550) ;
#5263=PLANE('',#69551) ;
#5264=PLANE('',#69552) ;
#5265=PLANE('',#69553) ;
#5266=PLANE('',#69554) ;
#5267=PLANE('',#69557) ;
#5268=PLANE('',#69563) ;
#5269=PLANE('',#69564) ;
#5270=PLANE('',#69565) ;
#5271=PLANE('',#69566) ;
#5272=PLANE('',#69567) ;
#5273=PLANE('',#69571) ;
#5274=PLANE('',#69572) ;
#5275=PLANE('',#69573) ;
#5276=PLANE('',#69574) ;
#5277=PLANE('',#69575) ;
#5278=PLANE('',#69581) ;
#5279=PLANE('',#70031) ;
#5280=PLANE('',#70033) ;
#5281=PLANE('',#70034) ;
#5282=PLANE('',#70035) ;
#5283=PLANE('',#70036) ;
#5284=PLANE('',#70037) ;
#5285=PLANE('',#70038) ;
#5286=PLANE('',#70040) ;
#5287=PLANE('',#70057) ;
#5288=PLANE('',#70074) ;
#5289=PLANE('',#70075) ;
#5290=PLANE('',#70076) ;
#5291=PLANE('',#70077) ;
#5292=PLANE('',#70079) ;
#5293=PLANE('',#70080) ;
#5294=PLANE('',#70081) ;
#5295=PLANE('',#70084) ;
#5296=PLANE('',#70098) ;
#5297=PLANE('',#70101) ;
#5298=PLANE('',#70104) ;
#5299=PLANE('',#70106) ;
#5300=PLANE('',#70108) ;
#5301=PLANE('',#70109) ;
#5302=PLANE('',#70110) ;
#5303=PLANE('',#70111) ;
#5304=PLANE('',#70112) ;
#5305=PLANE('',#70113) ;
#5306=PLANE('',#70114) ;
#5307=PLANE('',#70119) ;
#5308=PLANE('',#70123) ;
#5309=PLANE('',#70124) ;
#5310=PLANE('',#70131) ;
#5311=PLANE('',#70132) ;
#5312=PLANE('',#70133) ;
#5313=PLANE('',#70137) ;
#5314=PLANE('',#70139) ;
#5315=PLANE('',#70143) ;
#5316=PLANE('',#70147) ;
#5317=PLANE('',#70148) ;
#5318=PLANE('',#70149) ;
#5319=PLANE('',#70151) ;
#5320=PLANE('',#70152) ;
#5321=PLANE('',#70156) ;
#5322=PLANE('',#70157) ;
#5323=PLANE('',#70158) ;
#5324=PLANE('',#70159) ;
#5325=PLANE('',#70160) ;
#5326=PLANE('',#70161) ;
#5327=PLANE('',#70162) ;
#5328=PLANE('',#70163) ;
#5329=PLANE('',#70164) ;
#5330=PLANE('',#70167) ;
#5331=PLANE('',#70173) ;
#5332=PLANE('',#70174) ;
#5333=PLANE('',#70175) ;
#5334=PLANE('',#70176) ;
#5335=PLANE('',#70177) ;
#5336=PLANE('',#70181) ;
#5337=PLANE('',#70182) ;
#5338=PLANE('',#70183) ;
#5339=PLANE('',#70184) ;
#5340=PLANE('',#70185) ;
#5341=PLANE('',#70191) ;
#5342=PLANE('',#70641) ;
#5343=PLANE('',#70643) ;
#5344=PLANE('',#70644) ;
#5345=PLANE('',#70645) ;
#5346=PLANE('',#70646) ;
#5347=PLANE('',#70647) ;
#5348=PLANE('',#70648) ;
#5349=PLANE('',#70650) ;
#5350=PLANE('',#70667) ;
#5351=PLANE('',#70684) ;
#5352=PLANE('',#70685) ;
#5353=PLANE('',#70686) ;
#5354=PLANE('',#70687) ;
#5355=PLANE('',#70689) ;
#5356=PLANE('',#70690) ;
#5357=PLANE('',#70691) ;
#5358=PLANE('',#70694) ;
#5359=PLANE('',#70708) ;
#5360=PLANE('',#70711) ;
#5361=PLANE('',#70714) ;
#5362=PLANE('',#70716) ;
#5363=PLANE('',#70718) ;
#5364=PLANE('',#70719) ;
#5365=PLANE('',#70720) ;
#5366=PLANE('',#70721) ;
#5367=PLANE('',#70722) ;
#5368=PLANE('',#70723) ;
#5369=PLANE('',#70724) ;
#5370=PLANE('',#70729) ;
#5371=PLANE('',#70733) ;
#5372=PLANE('',#70734) ;
#5373=PLANE('',#70741) ;
#5374=PLANE('',#70742) ;
#5375=PLANE('',#70743) ;
#5376=PLANE('',#70747) ;
#5377=PLANE('',#70749) ;
#5378=PLANE('',#70753) ;
#5379=PLANE('',#70757) ;
#5380=PLANE('',#70758) ;
#5381=PLANE('',#70759) ;
#5382=PLANE('',#70761) ;
#5383=PLANE('',#70762) ;
#5384=PLANE('',#70766) ;
#5385=PLANE('',#70767) ;
#5386=PLANE('',#70768) ;
#5387=PLANE('',#70769) ;
#5388=PLANE('',#70770) ;
#5389=PLANE('',#70771) ;
#5390=PLANE('',#70772) ;
#5391=PLANE('',#70773) ;
#5392=PLANE('',#70774) ;
#5393=PLANE('',#70777) ;
#5394=PLANE('',#70783) ;
#5395=PLANE('',#70784) ;
#5396=PLANE('',#70785) ;
#5397=PLANE('',#70786) ;
#5398=PLANE('',#70787) ;
#5399=PLANE('',#70791) ;
#5400=PLANE('',#70792) ;
#5401=PLANE('',#70793) ;
#5402=PLANE('',#70794) ;
#5403=PLANE('',#70795) ;
#5404=PLANE('',#70801) ;
#5405=PLANE('',#71251) ;
#5406=PLANE('',#71253) ;
#5407=PLANE('',#71254) ;
#5408=PLANE('',#71255) ;
#5409=PLANE('',#71256) ;
#5410=PLANE('',#71257) ;
#5411=PLANE('',#71258) ;
#5412=PLANE('',#71260) ;
#5413=PLANE('',#71277) ;
#5414=PLANE('',#71294) ;
#5415=PLANE('',#71295) ;
#5416=PLANE('',#71296) ;
#5417=PLANE('',#71297) ;
#5418=PLANE('',#71299) ;
#5419=PLANE('',#71300) ;
#5420=PLANE('',#71301) ;
#5421=PLANE('',#71304) ;
#5422=PLANE('',#71318) ;
#5423=PLANE('',#71321) ;
#5424=PLANE('',#71324) ;
#5425=PLANE('',#71326) ;
#5426=PLANE('',#71328) ;
#5427=PLANE('',#71329) ;
#5428=PLANE('',#71330) ;
#5429=PLANE('',#71331) ;
#5430=PLANE('',#71332) ;
#5431=PLANE('',#71333) ;
#5432=PLANE('',#71334) ;
#5433=PLANE('',#71339) ;
#5434=PLANE('',#71343) ;
#5435=PLANE('',#71344) ;
#5436=PLANE('',#71351) ;
#5437=PLANE('',#71352) ;
#5438=PLANE('',#71353) ;
#5439=PLANE('',#71357) ;
#5440=PLANE('',#71359) ;
#5441=PLANE('',#71363) ;
#5442=PLANE('',#71367) ;
#5443=PLANE('',#71368) ;
#5444=PLANE('',#71369) ;
#5445=PLANE('',#71371) ;
#5446=PLANE('',#71372) ;
#5447=PLANE('',#71376) ;
#5448=PLANE('',#71377) ;
#5449=PLANE('',#71378) ;
#5450=PLANE('',#71379) ;
#5451=PLANE('',#71380) ;
#5452=PLANE('',#71381) ;
#5453=PLANE('',#71382) ;
#5454=PLANE('',#71383) ;
#5455=PLANE('',#71384) ;
#5456=PLANE('',#71387) ;
#5457=PLANE('',#71393) ;
#5458=PLANE('',#71394) ;
#5459=PLANE('',#71395) ;
#5460=PLANE('',#71396) ;
#5461=PLANE('',#71397) ;
#5462=PLANE('',#71401) ;
#5463=PLANE('',#71402) ;
#5464=PLANE('',#71403) ;
#5465=PLANE('',#71404) ;
#5466=PLANE('',#71405) ;
#5467=PLANE('',#71411) ;
#6166=CYLINDRICAL_SURFACE('',#68794,0.1) ;
#6167=CYLINDRICAL_SURFACE('',#68798,0.1) ;
#6168=CYLINDRICAL_SURFACE('',#68806,1.5) ;
#6169=CYLINDRICAL_SURFACE('',#68807,3.) ;
#6170=CYLINDRICAL_SURFACE('',#68905,1.75) ;
#6171=CYLINDRICAL_SURFACE('',#68908,1.75) ;
#6172=CYLINDRICAL_SURFACE('',#68920,1.75) ;
#6173=CYLINDRICAL_SURFACE('',#68924,1.75) ;
#6174=CYLINDRICAL_SURFACE('',#68950,2.) ;
#6175=CYLINDRICAL_SURFACE('',#68958,1.) ;
#6176=CYLINDRICAL_SURFACE('',#68973,0.1) ;
#6177=CYLINDRICAL_SURFACE('',#68978,0.1) ;
#6178=CYLINDRICAL_SURFACE('',#68980,0.1) ;
#6179=CYLINDRICAL_SURFACE('',#68989,0.1) ;
#6180=CYLINDRICAL_SURFACE('',#68991,0.1) ;
#6181=CYLINDRICAL_SURFACE('',#68994,0.1) ;
#6182=CYLINDRICAL_SURFACE('',#68998,0.1) ;
#6183=CYLINDRICAL_SURFACE('',#69000,0.1) ;
#6184=CYLINDRICAL_SURFACE('',#69002,0.1) ;
#6185=CYLINDRICAL_SURFACE('',#69014,0.1) ;
#6186=CYLINDRICAL_SURFACE('',#69019,0.1) ;
#6187=CYLINDRICAL_SURFACE('',#69021,0.1) ;
#6188=CYLINDRICAL_SURFACE('',#69029,0.1) ;
#6189=CYLINDRICAL_SURFACE('',#69031,0.1) ;
#6190=CYLINDRICAL_SURFACE('',#69033,0.1) ;
#6191=CYLINDRICAL_SURFACE('',#69035,0.1) ;
#6192=CYLINDRICAL_SURFACE('',#69041,0.1) ;
#6193=CYLINDRICAL_SURFACE('',#69046,0.1) ;
#6194=CYLINDRICAL_SURFACE('',#69048,0.1) ;
#6195=CYLINDRICAL_SURFACE('',#69050,0.1) ;
#6196=CYLINDRICAL_SURFACE('',#69052,0.1) ;
#6197=CYLINDRICAL_SURFACE('',#69055,0.1) ;
#6198=CYLINDRICAL_SURFACE('',#69061,0.1) ;
#6199=CYLINDRICAL_SURFACE('',#69066,0.1) ;
#6200=CYLINDRICAL_SURFACE('',#69069,0.1) ;
#6201=CYLINDRICAL_SURFACE('',#69072,0.1) ;
#6202=CYLINDRICAL_SURFACE('',#69074,0.1) ;
#6203=CYLINDRICAL_SURFACE('',#69079,0.1) ;
#6204=CYLINDRICAL_SURFACE('',#69086,0.1) ;
#6205=CYLINDRICAL_SURFACE('',#69088,0.1) ;
#6206=CYLINDRICAL_SURFACE('',#69093,0.1) ;
#6207=CYLINDRICAL_SURFACE('',#69095,0.1) ;
#6208=CYLINDRICAL_SURFACE('',#69101,0.1) ;
#6209=CYLINDRICAL_SURFACE('',#69108,0.1) ;
#6210=CYLINDRICAL_SURFACE('',#69110,0.1) ;
#6211=CYLINDRICAL_SURFACE('',#69112,0.1) ;
#6212=CYLINDRICAL_SURFACE('',#69115,0.1) ;
#6213=CYLINDRICAL_SURFACE('',#69116,0.0999999999999998) ;
#6214=CYLINDRICAL_SURFACE('',#69121,0.0999999999999998) ;
#6215=CYLINDRICAL_SURFACE('',#69123,0.0999999999999998) ;
#6216=CYLINDRICAL_SURFACE('',#69127,0.1) ;
#6217=CYLINDRICAL_SURFACE('',#69129,0.1) ;
#6218=CYLINDRICAL_SURFACE('',#69141,0.0999999999999998) ;
#6219=CYLINDRICAL_SURFACE('',#69143,0.1) ;
#6220=CYLINDRICAL_SURFACE('',#69147,0.1) ;
#6221=CYLINDRICAL_SURFACE('',#69150,0.1) ;
#6222=CYLINDRICAL_SURFACE('',#69152,0.0999999999999998) ;
#6223=CYLINDRICAL_SURFACE('',#69162,0.1) ;
#6224=CYLINDRICAL_SURFACE('',#69165,0.1) ;
#6225=CYLINDRICAL_SURFACE('',#69170,0.0999999999999998) ;
#6226=CYLINDRICAL_SURFACE('',#69172,0.0999999999999998) ;
#6227=CYLINDRICAL_SURFACE('',#69183,0.0999999999999998) ;
#6228=CYLINDRICAL_SURFACE('',#69189,0.1) ;
#6229=CYLINDRICAL_SURFACE('',#69192,0.1) ;
#6230=CYLINDRICAL_SURFACE('',#69196,0.1) ;
#6231=CYLINDRICAL_SURFACE('',#69201,0.1) ;
#6232=CYLINDRICAL_SURFACE('',#69206,0.1) ;
#6233=CYLINDRICAL_SURFACE('',#69208,0.1) ;
#6234=CYLINDRICAL_SURFACE('',#69211,0.1) ;
#6235=CYLINDRICAL_SURFACE('',#69213,0.1) ;
#6236=CYLINDRICAL_SURFACE('',#69215,0.1) ;
#6237=CYLINDRICAL_SURFACE('',#69222,0.1) ;
#6238=CYLINDRICAL_SURFACE('',#69224,0.1) ;
#6239=CYLINDRICAL_SURFACE('',#69228,0.1) ;
#6240=CYLINDRICAL_SURFACE('',#69230,0.1) ;
#6241=CYLINDRICAL_SURFACE('',#69234,0.0999999999999998) ;
#6242=CYLINDRICAL_SURFACE('',#69236,0.1) ;
#6243=CYLINDRICAL_SURFACE('',#69238,0.1) ;
#6244=CYLINDRICAL_SURFACE('',#69241,0.1) ;
#6245=CYLINDRICAL_SURFACE('',#69244,0.1) ;
#6246=CYLINDRICAL_SURFACE('',#69249,0.0999999999999998) ;
#6247=CYLINDRICAL_SURFACE('',#69251,0.1) ;
#6248=CYLINDRICAL_SURFACE('',#69255,0.0999999999999994) ;
#6249=CYLINDRICAL_SURFACE('',#69257,0.1) ;
#6250=CYLINDRICAL_SURFACE('',#69260,0.1) ;
#6251=CYLINDRICAL_SURFACE('',#69263,0.0999999999999994) ;
#6252=CYLINDRICAL_SURFACE('',#69269,0.1) ;
#6253=CYLINDRICAL_SURFACE('',#69270,0.0999999999999994) ;
#6254=CYLINDRICAL_SURFACE('',#69272,0.1) ;
#6255=CYLINDRICAL_SURFACE('',#69276,0.0999999999999994) ;
#6256=CYLINDRICAL_SURFACE('',#69278,0.0999999999999994) ;
#6257=CYLINDRICAL_SURFACE('',#69282,0.0999999999999998) ;
#6258=CYLINDRICAL_SURFACE('',#69283,0.1) ;
#6259=CYLINDRICAL_SURFACE('',#69286,0.0999999999999994) ;
#6260=CYLINDRICAL_SURFACE('',#69290,0.0999999999999994) ;
#6261=CYLINDRICAL_SURFACE('',#69292,0.0999999999999994) ;
#6262=CYLINDRICAL_SURFACE('',#69296,0.0999999999999998) ;
#6263=CYLINDRICAL_SURFACE('',#69298,0.1) ;
#6264=CYLINDRICAL_SURFACE('',#69301,0.1) ;
#6265=CYLINDRICAL_SURFACE('',#69302,0.1) ;
#6266=CYLINDRICAL_SURFACE('',#69303,0.1) ;
#6267=CYLINDRICAL_SURFACE('',#69304,0.0999999999999994) ;
#6268=CYLINDRICAL_SURFACE('',#69305,0.0999999999999994) ;
#6269=CYLINDRICAL_SURFACE('',#69310,0.0999999999999994) ;
#6270=CYLINDRICAL_SURFACE('',#69313,0.1) ;
#6271=CYLINDRICAL_SURFACE('',#69317,0.1) ;
#6272=CYLINDRICAL_SURFACE('',#69320,0.1) ;
#6273=CYLINDRICAL_SURFACE('',#69324,0.1) ;
#6274=CYLINDRICAL_SURFACE('',#69327,0.1) ;
#6275=CYLINDRICAL_SURFACE('',#69329,0.0999999999999994) ;
#6276=CYLINDRICAL_SURFACE('',#69332,0.0999999999999994) ;
#6277=CYLINDRICAL_SURFACE('',#69334,0.0999999999999994) ;
#6278=CYLINDRICAL_SURFACE('',#69336,0.1) ;
#6279=CYLINDRICAL_SURFACE('',#69338,0.0999999999999994) ;
#6280=CYLINDRICAL_SURFACE('',#69347,0.1) ;
#6281=CYLINDRICAL_SURFACE('',#69349,0.1) ;
#6282=CYLINDRICAL_SURFACE('',#69355,0.1) ;
#6283=CYLINDRICAL_SURFACE('',#69357,0.1) ;
#6284=CYLINDRICAL_SURFACE('',#69363,0.0999999999999994) ;
#6285=CYLINDRICAL_SURFACE('',#69365,0.0999999999999994) ;
#6286=CYLINDRICAL_SURFACE('',#69371,0.0999999999999994) ;
#6287=CYLINDRICAL_SURFACE('',#69373,0.0999999999999994) ;
#6288=CYLINDRICAL_SURFACE('',#69376,0.0999999999999994) ;
#6289=CYLINDRICAL_SURFACE('',#69382,0.0999999999999994) ;
#6290=CYLINDRICAL_SURFACE('',#69385,0.0999999999999994) ;
#6291=CYLINDRICAL_SURFACE('',#69388,0.0999999999999994) ;
#6292=CYLINDRICAL_SURFACE('',#69404,0.1) ;
#6293=CYLINDRICAL_SURFACE('',#69408,0.1) ;
#6294=CYLINDRICAL_SURFACE('',#69416,1.5) ;
#6295=CYLINDRICAL_SURFACE('',#69417,3.) ;
#6296=CYLINDRICAL_SURFACE('',#69515,1.75) ;
#6297=CYLINDRICAL_SURFACE('',#69518,1.75) ;
#6298=CYLINDRICAL_SURFACE('',#69530,1.75) ;
#6299=CYLINDRICAL_SURFACE('',#69534,1.75) ;
#6300=CYLINDRICAL_SURFACE('',#69560,2.) ;
#6301=CYLINDRICAL_SURFACE('',#69568,1.) ;
#6302=CYLINDRICAL_SURFACE('',#69583,0.1) ;
#6303=CYLINDRICAL_SURFACE('',#69588,0.1) ;
#6304=CYLINDRICAL_SURFACE('',#69590,0.1) ;
#6305=CYLINDRICAL_SURFACE('',#69599,0.1) ;
#6306=CYLINDRICAL_SURFACE('',#69601,0.1) ;
#6307=CYLINDRICAL_SURFACE('',#69604,0.1) ;
#6308=CYLINDRICAL_SURFACE('',#69608,0.1) ;
#6309=CYLINDRICAL_SURFACE('',#69610,0.1) ;
#6310=CYLINDRICAL_SURFACE('',#69612,0.1) ;
#6311=CYLINDRICAL_SURFACE('',#69624,0.1) ;
#6312=CYLINDRICAL_SURFACE('',#69629,0.1) ;
#6313=CYLINDRICAL_SURFACE('',#69631,0.1) ;
#6314=CYLINDRICAL_SURFACE('',#69639,0.1) ;
#6315=CYLINDRICAL_SURFACE('',#69641,0.1) ;
#6316=CYLINDRICAL_SURFACE('',#69643,0.1) ;
#6317=CYLINDRICAL_SURFACE('',#69645,0.1) ;
#6318=CYLINDRICAL_SURFACE('',#69651,0.1) ;
#6319=CYLINDRICAL_SURFACE('',#69656,0.1) ;
#6320=CYLINDRICAL_SURFACE('',#69658,0.1) ;
#6321=CYLINDRICAL_SURFACE('',#69660,0.1) ;
#6322=CYLINDRICAL_SURFACE('',#69662,0.1) ;
#6323=CYLINDRICAL_SURFACE('',#69665,0.1) ;
#6324=CYLINDRICAL_SURFACE('',#69671,0.1) ;
#6325=CYLINDRICAL_SURFACE('',#69676,0.1) ;
#6326=CYLINDRICAL_SURFACE('',#69679,0.1) ;
#6327=CYLINDRICAL_SURFACE('',#69682,0.1) ;
#6328=CYLINDRICAL_SURFACE('',#69684,0.1) ;
#6329=CYLINDRICAL_SURFACE('',#69689,0.1) ;
#6330=CYLINDRICAL_SURFACE('',#69696,0.1) ;
#6331=CYLINDRICAL_SURFACE('',#69698,0.1) ;
#6332=CYLINDRICAL_SURFACE('',#69703,0.1) ;
#6333=CYLINDRICAL_SURFACE('',#69705,0.1) ;
#6334=CYLINDRICAL_SURFACE('',#69711,0.0999999999999998) ;
#6335=CYLINDRICAL_SURFACE('',#69718,0.1) ;
#6336=CYLINDRICAL_SURFACE('',#69720,0.0999999999999998) ;
#6337=CYLINDRICAL_SURFACE('',#69722,0.0999999999999998) ;
#6338=CYLINDRICAL_SURFACE('',#69725,0.0999999999999998) ;
#6339=CYLINDRICAL_SURFACE('',#69726,0.0999999999999998) ;
#6340=CYLINDRICAL_SURFACE('',#69731,0.0999999999999998) ;
#6341=CYLINDRICAL_SURFACE('',#69733,0.0999999999999998) ;
#6342=CYLINDRICAL_SURFACE('',#69737,0.1) ;
#6343=CYLINDRICAL_SURFACE('',#69739,0.1) ;
#6344=CYLINDRICAL_SURFACE('',#69751,0.0999999999999998) ;
#6345=CYLINDRICAL_SURFACE('',#69753,0.1) ;
#6346=CYLINDRICAL_SURFACE('',#69757,0.1) ;
#6347=CYLINDRICAL_SURFACE('',#69760,0.1) ;
#6348=CYLINDRICAL_SURFACE('',#69762,0.0999999999999998) ;
#6349=CYLINDRICAL_SURFACE('',#69772,0.1) ;
#6350=CYLINDRICAL_SURFACE('',#69775,0.1) ;
#6351=CYLINDRICAL_SURFACE('',#69780,0.0999999999999998) ;
#6352=CYLINDRICAL_SURFACE('',#69782,0.0999999999999998) ;
#6353=CYLINDRICAL_SURFACE('',#69793,0.0999999999999998) ;
#6354=CYLINDRICAL_SURFACE('',#69799,0.1) ;
#6355=CYLINDRICAL_SURFACE('',#69802,0.1) ;
#6356=CYLINDRICAL_SURFACE('',#69806,0.1) ;
#6357=CYLINDRICAL_SURFACE('',#69811,0.1) ;
#6358=CYLINDRICAL_SURFACE('',#69816,0.1) ;
#6359=CYLINDRICAL_SURFACE('',#69818,0.1) ;
#6360=CYLINDRICAL_SURFACE('',#69821,0.1) ;
#6361=CYLINDRICAL_SURFACE('',#69823,0.1) ;
#6362=CYLINDRICAL_SURFACE('',#69825,0.1) ;
#6363=CYLINDRICAL_SURFACE('',#69832,0.1) ;
#6364=CYLINDRICAL_SURFACE('',#69834,0.1) ;
#6365=CYLINDRICAL_SURFACE('',#69838,0.1) ;
#6366=CYLINDRICAL_SURFACE('',#69840,0.1) ;
#6367=CYLINDRICAL_SURFACE('',#69844,0.0999999999999998) ;
#6368=CYLINDRICAL_SURFACE('',#69846,0.1) ;
#6369=CYLINDRICAL_SURFACE('',#69848,0.1) ;
#6370=CYLINDRICAL_SURFACE('',#69851,0.1) ;
#6371=CYLINDRICAL_SURFACE('',#69854,0.1) ;
#6372=CYLINDRICAL_SURFACE('',#69859,0.0999999999999998) ;
#6373=CYLINDRICAL_SURFACE('',#69861,0.1) ;
#6374=CYLINDRICAL_SURFACE('',#69865,0.0999999999999994) ;
#6375=CYLINDRICAL_SURFACE('',#69867,0.1) ;
#6376=CYLINDRICAL_SURFACE('',#69870,0.1) ;
#6377=CYLINDRICAL_SURFACE('',#69873,0.0999999999999994) ;
#6378=CYLINDRICAL_SURFACE('',#69879,0.1) ;
#6379=CYLINDRICAL_SURFACE('',#69880,0.0999999999999994) ;
#6380=CYLINDRICAL_SURFACE('',#69882,0.1) ;
#6381=CYLINDRICAL_SURFACE('',#69886,0.0999999999999994) ;
#6382=CYLINDRICAL_SURFACE('',#69888,0.0999999999999994) ;
#6383=CYLINDRICAL_SURFACE('',#69892,0.0999999999999998) ;
#6384=CYLINDRICAL_SURFACE('',#69893,0.1) ;
#6385=CYLINDRICAL_SURFACE('',#69896,0.0999999999999994) ;
#6386=CYLINDRICAL_SURFACE('',#69900,0.0999999999999994) ;
#6387=CYLINDRICAL_SURFACE('',#69902,0.0999999999999994) ;
#6388=CYLINDRICAL_SURFACE('',#69906,0.0999999999999998) ;
#6389=CYLINDRICAL_SURFACE('',#69908,0.1) ;
#6390=CYLINDRICAL_SURFACE('',#69911,0.1) ;
#6391=CYLINDRICAL_SURFACE('',#69912,0.1) ;
#6392=CYLINDRICAL_SURFACE('',#69913,0.1) ;
#6393=CYLINDRICAL_SURFACE('',#69914,0.0999999999999994) ;
#6394=CYLINDRICAL_SURFACE('',#69915,0.0999999999999994) ;
#6395=CYLINDRICAL_SURFACE('',#69920,0.0999999999999994) ;
#6396=CYLINDRICAL_SURFACE('',#69923,0.1) ;
#6397=CYLINDRICAL_SURFACE('',#69927,0.1) ;
#6398=CYLINDRICAL_SURFACE('',#69930,0.1) ;
#6399=CYLINDRICAL_SURFACE('',#69934,0.1) ;
#6400=CYLINDRICAL_SURFACE('',#69937,0.1) ;
#6401=CYLINDRICAL_SURFACE('',#69939,0.0999999999999994) ;
#6402=CYLINDRICAL_SURFACE('',#69942,0.0999999999999994) ;
#6403=CYLINDRICAL_SURFACE('',#69944,0.0999999999999994) ;
#6404=CYLINDRICAL_SURFACE('',#69946,0.1) ;
#6405=CYLINDRICAL_SURFACE('',#69948,0.0999999999999994) ;
#6406=CYLINDRICAL_SURFACE('',#69957,0.1) ;
#6407=CYLINDRICAL_SURFACE('',#69959,0.1) ;
#6408=CYLINDRICAL_SURFACE('',#69965,0.1) ;
#6409=CYLINDRICAL_SURFACE('',#69967,0.1) ;
#6410=CYLINDRICAL_SURFACE('',#69973,0.0999999999999994) ;
#6411=CYLINDRICAL_SURFACE('',#69975,0.0999999999999994) ;
#6412=CYLINDRICAL_SURFACE('',#69981,0.0999999999999994) ;
#6413=CYLINDRICAL_SURFACE('',#69983,0.0999999999999994) ;
#6414=CYLINDRICAL_SURFACE('',#69986,0.0999999999999994) ;
#6415=CYLINDRICAL_SURFACE('',#69992,0.0999999999999994) ;
#6416=CYLINDRICAL_SURFACE('',#69995,0.0999999999999994) ;
#6417=CYLINDRICAL_SURFACE('',#69998,0.0999999999999994) ;
#6418=CYLINDRICAL_SURFACE('',#70014,0.1) ;
#6419=CYLINDRICAL_SURFACE('',#70018,0.1) ;
#6420=CYLINDRICAL_SURFACE('',#70026,1.5) ;
#6421=CYLINDRICAL_SURFACE('',#70027,3.) ;
#6422=CYLINDRICAL_SURFACE('',#70125,1.75) ;
#6423=CYLINDRICAL_SURFACE('',#70128,1.75) ;
#6424=CYLINDRICAL_SURFACE('',#70140,1.75) ;
#6425=CYLINDRICAL_SURFACE('',#70144,1.75) ;
#6426=CYLINDRICAL_SURFACE('',#70170,2.) ;
#6427=CYLINDRICAL_SURFACE('',#70178,1.) ;
#6428=CYLINDRICAL_SURFACE('',#70193,0.1) ;
#6429=CYLINDRICAL_SURFACE('',#70198,0.1) ;
#6430=CYLINDRICAL_SURFACE('',#70200,0.1) ;
#6431=CYLINDRICAL_SURFACE('',#70209,0.1) ;
#6432=CYLINDRICAL_SURFACE('',#70211,0.1) ;
#6433=CYLINDRICAL_SURFACE('',#70214,0.1) ;
#6434=CYLINDRICAL_SURFACE('',#70218,0.1) ;
#6435=CYLINDRICAL_SURFACE('',#70220,0.0999999999999994) ;
#6436=CYLINDRICAL_SURFACE('',#70222,0.1) ;
#6437=CYLINDRICAL_SURFACE('',#70234,0.1) ;
#6438=CYLINDRICAL_SURFACE('',#70239,0.0999999999999994) ;
#6439=CYLINDRICAL_SURFACE('',#70241,0.0999999999999994) ;
#6440=CYLINDRICAL_SURFACE('',#70249,0.1) ;
#6441=CYLINDRICAL_SURFACE('',#70251,0.1) ;
#6442=CYLINDRICAL_SURFACE('',#70253,0.1) ;
#6443=CYLINDRICAL_SURFACE('',#70255,0.1) ;
#6444=CYLINDRICAL_SURFACE('',#70261,0.0999999999999994) ;
#6445=CYLINDRICAL_SURFACE('',#70266,0.0999999999999994) ;
#6446=CYLINDRICAL_SURFACE('',#70268,0.0999999999999994) ;
#6447=CYLINDRICAL_SURFACE('',#70270,0.1) ;
#6448=CYLINDRICAL_SURFACE('',#70272,0.1) ;
#6449=CYLINDRICAL_SURFACE('',#70275,0.1) ;
#6450=CYLINDRICAL_SURFACE('',#70281,0.0999999999999994) ;
#6451=CYLINDRICAL_SURFACE('',#70286,0.0999999999999994) ;
#6452=CYLINDRICAL_SURFACE('',#70289,0.1) ;
#6453=CYLINDRICAL_SURFACE('',#70292,0.0999999999999994) ;
#6454=CYLINDRICAL_SURFACE('',#70294,0.0999999999999994) ;
#6455=CYLINDRICAL_SURFACE('',#70299,0.1) ;
#6456=CYLINDRICAL_SURFACE('',#70306,0.0999999999999994) ;
#6457=CYLINDRICAL_SURFACE('',#70308,0.1) ;
#6458=CYLINDRICAL_SURFACE('',#70313,0.1) ;
#6459=CYLINDRICAL_SURFACE('',#70315,0.1) ;
#6460=CYLINDRICAL_SURFACE('',#70321,0.0999999999999994) ;
#6461=CYLINDRICAL_SURFACE('',#70328,0.1) ;
#6462=CYLINDRICAL_SURFACE('',#70330,0.0999999999999994) ;
#6463=CYLINDRICAL_SURFACE('',#70332,0.0999999999999994) ;
#6464=CYLINDRICAL_SURFACE('',#70335,0.0999999999999994) ;
#6465=CYLINDRICAL_SURFACE('',#70336,0.0999999999999998) ;
#6466=CYLINDRICAL_SURFACE('',#70341,0.0999999999999998) ;
#6467=CYLINDRICAL_SURFACE('',#70343,0.0999999999999998) ;
#6468=CYLINDRICAL_SURFACE('',#70347,0.1) ;
#6469=CYLINDRICAL_SURFACE('',#70349,0.1) ;
#6470=CYLINDRICAL_SURFACE('',#70361,0.0999999999999998) ;
#6471=CYLINDRICAL_SURFACE('',#70363,0.1) ;
#6472=CYLINDRICAL_SURFACE('',#70367,0.1) ;
#6473=CYLINDRICAL_SURFACE('',#70370,0.1) ;
#6474=CYLINDRICAL_SURFACE('',#70372,0.0999999999999998) ;
#6475=CYLINDRICAL_SURFACE('',#70382,0.1) ;
#6476=CYLINDRICAL_SURFACE('',#70385,0.0999999999999994) ;
#6477=CYLINDRICAL_SURFACE('',#70390,0.0999999999999998) ;
#6478=CYLINDRICAL_SURFACE('',#70392,0.0999999999999998) ;
#6479=CYLINDRICAL_SURFACE('',#70403,0.0999999999999998) ;
#6480=CYLINDRICAL_SURFACE('',#70409,0.0999999999999994) ;
#6481=CYLINDRICAL_SURFACE('',#70412,0.0999999999999994) ;
#6482=CYLINDRICAL_SURFACE('',#70416,0.1) ;
#6483=CYLINDRICAL_SURFACE('',#70421,0.0999999999999994) ;
#6484=CYLINDRICAL_SURFACE('',#70426,0.0999999999999994) ;
#6485=CYLINDRICAL_SURFACE('',#70428,0.1) ;
#6486=CYLINDRICAL_SURFACE('',#70431,0.0999999999999994) ;
#6487=CYLINDRICAL_SURFACE('',#70433,0.1) ;
#6488=CYLINDRICAL_SURFACE('',#70435,0.1) ;
#6489=CYLINDRICAL_SURFACE('',#70442,0.1) ;
#6490=CYLINDRICAL_SURFACE('',#70444,0.0999999999999994) ;
#6491=CYLINDRICAL_SURFACE('',#70448,0.1) ;
#6492=CYLINDRICAL_SURFACE('',#70450,0.0999999999999994) ;
#6493=CYLINDRICAL_SURFACE('',#70454,0.0999999999999998) ;
#6494=CYLINDRICAL_SURFACE('',#70456,0.1) ;
#6495=CYLINDRICAL_SURFACE('',#70458,0.1) ;
#6496=CYLINDRICAL_SURFACE('',#70461,0.1) ;
#6497=CYLINDRICAL_SURFACE('',#70464,0.0999999999999994) ;
#6498=CYLINDRICAL_SURFACE('',#70469,0.0999999999999998) ;
#6499=CYLINDRICAL_SURFACE('',#70471,0.1) ;
#6500=CYLINDRICAL_SURFACE('',#70475,0.0999999999999994) ;
#6501=CYLINDRICAL_SURFACE('',#70477,0.1) ;
#6502=CYLINDRICAL_SURFACE('',#70480,0.1) ;
#6503=CYLINDRICAL_SURFACE('',#70483,0.0999999999999994) ;
#6504=CYLINDRICAL_SURFACE('',#70489,0.0999999999999994) ;
#6505=CYLINDRICAL_SURFACE('',#70490,0.0999999999999994) ;
#6506=CYLINDRICAL_SURFACE('',#70492,0.0999999999999995) ;
#6507=CYLINDRICAL_SURFACE('',#70496,0.0999999999999994) ;
#6508=CYLINDRICAL_SURFACE('',#70498,0.0999999999999994) ;
#6509=CYLINDRICAL_SURFACE('',#70502,0.0999999999999998) ;
#6510=CYLINDRICAL_SURFACE('',#70503,0.0999999999999995) ;
#6511=CYLINDRICAL_SURFACE('',#70506,0.0999999999999994) ;
#6512=CYLINDRICAL_SURFACE('',#70510,0.0999999999999994) ;
#6513=CYLINDRICAL_SURFACE('',#70512,0.0999999999999994) ;
#6514=CYLINDRICAL_SURFACE('',#70516,0.0999999999999998) ;
#6515=CYLINDRICAL_SURFACE('',#70518,0.1) ;
#6516=CYLINDRICAL_SURFACE('',#70521,0.1) ;
#6517=CYLINDRICAL_SURFACE('',#70522,0.1) ;
#6518=CYLINDRICAL_SURFACE('',#70523,0.1) ;
#6519=CYLINDRICAL_SURFACE('',#70524,0.0999999999999994) ;
#6520=CYLINDRICAL_SURFACE('',#70525,0.0999999999999994) ;
#6521=CYLINDRICAL_SURFACE('',#70530,0.0999999999999994) ;
#6522=CYLINDRICAL_SURFACE('',#70533,0.0999999999999994) ;
#6523=CYLINDRICAL_SURFACE('',#70537,0.1) ;
#6524=CYLINDRICAL_SURFACE('',#70540,0.1) ;
#6525=CYLINDRICAL_SURFACE('',#70544,0.1) ;
#6526=CYLINDRICAL_SURFACE('',#70547,0.0999999999999994) ;
#6527=CYLINDRICAL_SURFACE('',#70549,0.0999999999999994) ;
#6528=CYLINDRICAL_SURFACE('',#70552,0.0999999999999994) ;
#6529=CYLINDRICAL_SURFACE('',#70554,0.0999999999999994) ;
#6530=CYLINDRICAL_SURFACE('',#70556,0.0999999999999994) ;
#6531=CYLINDRICAL_SURFACE('',#70558,0.0999999999999994) ;
#6532=CYLINDRICAL_SURFACE('',#70567,0.1) ;
#6533=CYLINDRICAL_SURFACE('',#70569,0.0999999999999994) ;
#6534=CYLINDRICAL_SURFACE('',#70575,0.0999999999999994) ;
#6535=CYLINDRICAL_SURFACE('',#70577,0.1) ;
#6536=CYLINDRICAL_SURFACE('',#70583,0.0999999999999994) ;
#6537=CYLINDRICAL_SURFACE('',#70585,0.0999999999999994) ;
#6538=CYLINDRICAL_SURFACE('',#70591,0.0999999999999994) ;
#6539=CYLINDRICAL_SURFACE('',#70593,0.0999999999999994) ;
#6540=CYLINDRICAL_SURFACE('',#70596,0.0999999999999994) ;
#6541=CYLINDRICAL_SURFACE('',#70602,0.0999999999999994) ;
#6542=CYLINDRICAL_SURFACE('',#70605,0.0999999999999994) ;
#6543=CYLINDRICAL_SURFACE('',#70608,0.0999999999999994) ;
#6544=CYLINDRICAL_SURFACE('',#70624,0.1) ;
#6545=CYLINDRICAL_SURFACE('',#70628,0.1) ;
#6546=CYLINDRICAL_SURFACE('',#70636,1.5) ;
#6547=CYLINDRICAL_SURFACE('',#70637,3.) ;
#6548=CYLINDRICAL_SURFACE('',#70735,1.75) ;
#6549=CYLINDRICAL_SURFACE('',#70738,1.75) ;
#6550=CYLINDRICAL_SURFACE('',#70750,1.75) ;
#6551=CYLINDRICAL_SURFACE('',#70754,1.75) ;
#6552=CYLINDRICAL_SURFACE('',#70780,2.) ;
#6553=CYLINDRICAL_SURFACE('',#70788,1.) ;
#6554=CYLINDRICAL_SURFACE('',#70803,0.1) ;
#6555=CYLINDRICAL_SURFACE('',#70808,0.1) ;
#6556=CYLINDRICAL_SURFACE('',#70810,0.1) ;
#6557=CYLINDRICAL_SURFACE('',#70819,0.1) ;
#6558=CYLINDRICAL_SURFACE('',#70821,0.1) ;
#6559=CYLINDRICAL_SURFACE('',#70824,0.1) ;
#6560=CYLINDRICAL_SURFACE('',#70828,0.1) ;
#6561=CYLINDRICAL_SURFACE('',#70830,0.0999999999999994) ;
#6562=CYLINDRICAL_SURFACE('',#70832,0.1) ;
#6563=CYLINDRICAL_SURFACE('',#70844,0.1) ;
#6564=CYLINDRICAL_SURFACE('',#70849,0.0999999999999994) ;
#6565=CYLINDRICAL_SURFACE('',#70851,0.0999999999999994) ;
#6566=CYLINDRICAL_SURFACE('',#70859,0.1) ;
#6567=CYLINDRICAL_SURFACE('',#70861,0.1) ;
#6568=CYLINDRICAL_SURFACE('',#70863,0.1) ;
#6569=CYLINDRICAL_SURFACE('',#70865,0.1) ;
#6570=CYLINDRICAL_SURFACE('',#70871,0.0999999999999994) ;
#6571=CYLINDRICAL_SURFACE('',#70876,0.0999999999999994) ;
#6572=CYLINDRICAL_SURFACE('',#70878,0.0999999999999994) ;
#6573=CYLINDRICAL_SURFACE('',#70880,0.1) ;
#6574=CYLINDRICAL_SURFACE('',#70882,0.1) ;
#6575=CYLINDRICAL_SURFACE('',#70885,0.1) ;
#6576=CYLINDRICAL_SURFACE('',#70891,0.0999999999999994) ;
#6577=CYLINDRICAL_SURFACE('',#70896,0.0999999999999994) ;
#6578=CYLINDRICAL_SURFACE('',#70899,0.1) ;
#6579=CYLINDRICAL_SURFACE('',#70902,0.0999999999999994) ;
#6580=CYLINDRICAL_SURFACE('',#70904,0.0999999999999994) ;
#6581=CYLINDRICAL_SURFACE('',#70909,0.1) ;
#6582=CYLINDRICAL_SURFACE('',#70916,0.0999999999999994) ;
#6583=CYLINDRICAL_SURFACE('',#70918,0.1) ;
#6584=CYLINDRICAL_SURFACE('',#70923,0.1) ;
#6585=CYLINDRICAL_SURFACE('',#70925,0.1) ;
#6586=CYLINDRICAL_SURFACE('',#70931,0.0999999999999994) ;
#6587=CYLINDRICAL_SURFACE('',#70938,0.1) ;
#6588=CYLINDRICAL_SURFACE('',#70940,0.0999999999999994) ;
#6589=CYLINDRICAL_SURFACE('',#70942,0.0999999999999994) ;
#6590=CYLINDRICAL_SURFACE('',#70945,0.0999999999999994) ;
#6591=CYLINDRICAL_SURFACE('',#70946,0.0999999999999998) ;
#6592=CYLINDRICAL_SURFACE('',#70951,0.0999999999999998) ;
#6593=CYLINDRICAL_SURFACE('',#70953,0.0999999999999998) ;
#6594=CYLINDRICAL_SURFACE('',#70957,0.1) ;
#6595=CYLINDRICAL_SURFACE('',#70959,0.1) ;
#6596=CYLINDRICAL_SURFACE('',#70971,0.0999999999999998) ;
#6597=CYLINDRICAL_SURFACE('',#70973,0.1) ;
#6598=CYLINDRICAL_SURFACE('',#70977,0.1) ;
#6599=CYLINDRICAL_SURFACE('',#70980,0.1) ;
#6600=CYLINDRICAL_SURFACE('',#70982,0.0999999999999998) ;
#6601=CYLINDRICAL_SURFACE('',#70992,0.1) ;
#6602=CYLINDRICAL_SURFACE('',#70995,0.0999999999999994) ;
#6603=CYLINDRICAL_SURFACE('',#71000,0.0999999999999998) ;
#6604=CYLINDRICAL_SURFACE('',#71002,0.0999999999999998) ;
#6605=CYLINDRICAL_SURFACE('',#71013,0.0999999999999998) ;
#6606=CYLINDRICAL_SURFACE('',#71019,0.0999999999999994) ;
#6607=CYLINDRICAL_SURFACE('',#71022,0.0999999999999994) ;
#6608=CYLINDRICAL_SURFACE('',#71026,0.1) ;
#6609=CYLINDRICAL_SURFACE('',#71031,0.0999999999999994) ;
#6610=CYLINDRICAL_SURFACE('',#71036,0.0999999999999994) ;
#6611=CYLINDRICAL_SURFACE('',#71038,0.1) ;
#6612=CYLINDRICAL_SURFACE('',#71041,0.0999999999999994) ;
#6613=CYLINDRICAL_SURFACE('',#71043,0.1) ;
#6614=CYLINDRICAL_SURFACE('',#71045,0.1) ;
#6615=CYLINDRICAL_SURFACE('',#71052,0.1) ;
#6616=CYLINDRICAL_SURFACE('',#71054,0.0999999999999994) ;
#6617=CYLINDRICAL_SURFACE('',#71058,0.1) ;
#6618=CYLINDRICAL_SURFACE('',#71060,0.0999999999999994) ;
#6619=CYLINDRICAL_SURFACE('',#71064,0.0999999999999998) ;
#6620=CYLINDRICAL_SURFACE('',#71066,0.1) ;
#6621=CYLINDRICAL_SURFACE('',#71068,0.1) ;
#6622=CYLINDRICAL_SURFACE('',#71071,0.1) ;
#6623=CYLINDRICAL_SURFACE('',#71074,0.0999999999999994) ;
#6624=CYLINDRICAL_SURFACE('',#71079,0.0999999999999998) ;
#6625=CYLINDRICAL_SURFACE('',#71081,0.1) ;
#6626=CYLINDRICAL_SURFACE('',#71085,0.0999999999999994) ;
#6627=CYLINDRICAL_SURFACE('',#71087,0.1) ;
#6628=CYLINDRICAL_SURFACE('',#71090,0.1) ;
#6629=CYLINDRICAL_SURFACE('',#71093,0.0999999999999994) ;
#6630=CYLINDRICAL_SURFACE('',#71099,0.0999999999999994) ;
#6631=CYLINDRICAL_SURFACE('',#71100,0.0999999999999994) ;
#6632=CYLINDRICAL_SURFACE('',#71102,0.0999999999999995) ;
#6633=CYLINDRICAL_SURFACE('',#71106,0.0999999999999994) ;
#6634=CYLINDRICAL_SURFACE('',#71108,0.0999999999999994) ;
#6635=CYLINDRICAL_SURFACE('',#71112,0.0999999999999998) ;
#6636=CYLINDRICAL_SURFACE('',#71113,0.0999999999999995) ;
#6637=CYLINDRICAL_SURFACE('',#71116,0.0999999999999994) ;
#6638=CYLINDRICAL_SURFACE('',#71120,0.0999999999999994) ;
#6639=CYLINDRICAL_SURFACE('',#71122,0.0999999999999994) ;
#6640=CYLINDRICAL_SURFACE('',#71126,0.0999999999999998) ;
#6641=CYLINDRICAL_SURFACE('',#71128,0.1) ;
#6642=CYLINDRICAL_SURFACE('',#71131,0.1) ;
#6643=CYLINDRICAL_SURFACE('',#71132,0.1) ;
#6644=CYLINDRICAL_SURFACE('',#71133,0.1) ;
#6645=CYLINDRICAL_SURFACE('',#71134,0.0999999999999994) ;
#6646=CYLINDRICAL_SURFACE('',#71135,0.0999999999999994) ;
#6647=CYLINDRICAL_SURFACE('',#71140,0.0999999999999994) ;
#6648=CYLINDRICAL_SURFACE('',#71143,0.0999999999999994) ;
#6649=CYLINDRICAL_SURFACE('',#71147,0.1) ;
#6650=CYLINDRICAL_SURFACE('',#71150,0.1) ;
#6651=CYLINDRICAL_SURFACE('',#71154,0.1) ;
#6652=CYLINDRICAL_SURFACE('',#71157,0.0999999999999994) ;
#6653=CYLINDRICAL_SURFACE('',#71159,0.0999999999999994) ;
#6654=CYLINDRICAL_SURFACE('',#71162,0.0999999999999994) ;
#6655=CYLINDRICAL_SURFACE('',#71164,0.0999999999999994) ;
#6656=CYLINDRICAL_SURFACE('',#71166,0.0999999999999994) ;
#6657=CYLINDRICAL_SURFACE('',#71168,0.0999999999999994) ;
#6658=CYLINDRICAL_SURFACE('',#71177,0.1) ;
#6659=CYLINDRICAL_SURFACE('',#71179,0.0999999999999994) ;
#6660=CYLINDRICAL_SURFACE('',#71185,0.0999999999999994) ;
#6661=CYLINDRICAL_SURFACE('',#71187,0.1) ;
#6662=CYLINDRICAL_SURFACE('',#71193,0.0999999999999994) ;
#6663=CYLINDRICAL_SURFACE('',#71195,0.0999999999999994) ;
#6664=CYLINDRICAL_SURFACE('',#71201,0.0999999999999994) ;
#6665=CYLINDRICAL_SURFACE('',#71203,0.0999999999999994) ;
#6666=CYLINDRICAL_SURFACE('',#71206,0.0999999999999994) ;
#6667=CYLINDRICAL_SURFACE('',#71212,0.0999999999999994) ;
#6668=CYLINDRICAL_SURFACE('',#71215,0.0999999999999994) ;
#6669=CYLINDRICAL_SURFACE('',#71218,0.0999999999999994) ;
#6670=CYLINDRICAL_SURFACE('',#71234,0.1) ;
#6671=CYLINDRICAL_SURFACE('',#71238,0.1) ;
#6672=CYLINDRICAL_SURFACE('',#71246,1.5) ;
#6673=CYLINDRICAL_SURFACE('',#71247,3.) ;
#6674=CYLINDRICAL_SURFACE('',#71345,1.75) ;
#6675=CYLINDRICAL_SURFACE('',#71348,1.75) ;
#6676=CYLINDRICAL_SURFACE('',#71360,1.75) ;
#6677=CYLINDRICAL_SURFACE('',#71364,1.75) ;
#6678=CYLINDRICAL_SURFACE('',#71390,2.) ;
#6679=CYLINDRICAL_SURFACE('',#71398,1.) ;
#6680=CYLINDRICAL_SURFACE('',#71413,0.1) ;
#6681=CYLINDRICAL_SURFACE('',#71418,0.1) ;
#6682=CYLINDRICAL_SURFACE('',#71420,0.1) ;
#6683=CYLINDRICAL_SURFACE('',#71429,0.1) ;
#6684=CYLINDRICAL_SURFACE('',#71431,0.1) ;
#6685=CYLINDRICAL_SURFACE('',#71434,0.1) ;
#6686=CYLINDRICAL_SURFACE('',#71438,0.1) ;
#6687=CYLINDRICAL_SURFACE('',#71440,0.0999999999999994) ;
#6688=CYLINDRICAL_SURFACE('',#71442,0.1) ;
#6689=CYLINDRICAL_SURFACE('',#71454,0.1) ;
#6690=CYLINDRICAL_SURFACE('',#71459,0.0999999999999994) ;
#6691=CYLINDRICAL_SURFACE('',#71461,0.0999999999999994) ;
#6692=CYLINDRICAL_SURFACE('',#71469,0.1) ;
#6693=CYLINDRICAL_SURFACE('',#71471,0.1) ;
#6694=CYLINDRICAL_SURFACE('',#71473,0.1) ;
#6695=CYLINDRICAL_SURFACE('',#71475,0.1) ;
#6696=CYLINDRICAL_SURFACE('',#71481,0.0999999999999994) ;
#6697=CYLINDRICAL_SURFACE('',#71486,0.0999999999999994) ;
#6698=CYLINDRICAL_SURFACE('',#71488,0.0999999999999994) ;
#6699=CYLINDRICAL_SURFACE('',#71490,0.1) ;
#6700=CYLINDRICAL_SURFACE('',#71492,0.1) ;
#6701=CYLINDRICAL_SURFACE('',#71495,0.1) ;
#6702=CYLINDRICAL_SURFACE('',#71501,0.0999999999999994) ;
#6703=CYLINDRICAL_SURFACE('',#71506,0.0999999999999994) ;
#6704=CYLINDRICAL_SURFACE('',#71509,0.1) ;
#6705=CYLINDRICAL_SURFACE('',#71512,0.0999999999999994) ;
#6706=CYLINDRICAL_SURFACE('',#71514,0.0999999999999994) ;
#6707=CYLINDRICAL_SURFACE('',#71519,0.1) ;
#6708=CYLINDRICAL_SURFACE('',#71526,0.0999999999999994) ;
#6709=CYLINDRICAL_SURFACE('',#71528,0.1) ;
#6710=CYLINDRICAL_SURFACE('',#71533,0.1) ;
#6711=CYLINDRICAL_SURFACE('',#71535,0.1) ;
#6712=CYLINDRICAL_SURFACE('',#71541,0.0999999999999994) ;
#6713=CYLINDRICAL_SURFACE('',#71548,0.1) ;
#6714=CYLINDRICAL_SURFACE('',#71550,0.0999999999999994) ;
#6715=CYLINDRICAL_SURFACE('',#71552,0.0999999999999994) ;
#6716=CYLINDRICAL_SURFACE('',#71555,0.0999999999999994) ;
#6717=CYLINDRICAL_SURFACE('',#71556,0.0999999999999998) ;
#6718=CYLINDRICAL_SURFACE('',#71561,0.0999999999999998) ;
#6719=CYLINDRICAL_SURFACE('',#71563,0.0999999999999998) ;
#6720=CYLINDRICAL_SURFACE('',#71567,0.1) ;
#6721=CYLINDRICAL_SURFACE('',#71569,0.1) ;
#6722=CYLINDRICAL_SURFACE('',#71581,0.0999999999999998) ;
#6723=CYLINDRICAL_SURFACE('',#71583,0.1) ;
#6724=CYLINDRICAL_SURFACE('',#71587,0.1) ;
#6725=CYLINDRICAL_SURFACE('',#71590,0.1) ;
#6726=CYLINDRICAL_SURFACE('',#71592,0.0999999999999998) ;
#6727=CYLINDRICAL_SURFACE('',#71602,0.1) ;
#6728=CYLINDRICAL_SURFACE('',#71605,0.0999999999999994) ;
#6729=CYLINDRICAL_SURFACE('',#71610,0.0999999999999998) ;
#6730=CYLINDRICAL_SURFACE('',#71612,0.0999999999999998) ;
#6731=CYLINDRICAL_SURFACE('',#71623,0.0999999999999998) ;
#6732=CYLINDRICAL_SURFACE('',#71629,0.0999999999999994) ;
#6733=CYLINDRICAL_SURFACE('',#71632,0.0999999999999994) ;
#6734=CYLINDRICAL_SURFACE('',#71636,0.1) ;
#6735=CYLINDRICAL_SURFACE('',#71641,0.0999999999999994) ;
#6736=CYLINDRICAL_SURFACE('',#71646,0.0999999999999994) ;
#6737=CYLINDRICAL_SURFACE('',#71648,0.1) ;
#6738=CYLINDRICAL_SURFACE('',#71651,0.0999999999999994) ;
#6739=CYLINDRICAL_SURFACE('',#71653,0.1) ;
#6740=CYLINDRICAL_SURFACE('',#71655,0.1) ;
#6741=CYLINDRICAL_SURFACE('',#71662,0.1) ;
#6742=CYLINDRICAL_SURFACE('',#71664,0.0999999999999994) ;
#6743=CYLINDRICAL_SURFACE('',#71668,0.1) ;
#6744=CYLINDRICAL_SURFACE('',#71670,0.0999999999999994) ;
#6745=CYLINDRICAL_SURFACE('',#71674,0.0999999999999998) ;
#6746=CYLINDRICAL_SURFACE('',#71676,0.1) ;
#6747=CYLINDRICAL_SURFACE('',#71678,0.1) ;
#6748=CYLINDRICAL_SURFACE('',#71681,0.1) ;
#6749=CYLINDRICAL_SURFACE('',#71684,0.0999999999999994) ;
#6750=CYLINDRICAL_SURFACE('',#71689,0.0999999999999998) ;
#6751=CYLINDRICAL_SURFACE('',#71691,0.1) ;
#6752=CYLINDRICAL_SURFACE('',#71695,0.0999999999999994) ;
#6753=CYLINDRICAL_SURFACE('',#71697,0.1) ;
#6754=CYLINDRICAL_SURFACE('',#71700,0.1) ;
#6755=CYLINDRICAL_SURFACE('',#71703,0.0999999999999994) ;
#6756=CYLINDRICAL_SURFACE('',#71709,0.0999999999999994) ;
#6757=CYLINDRICAL_SURFACE('',#71710,0.0999999999999994) ;
#6758=CYLINDRICAL_SURFACE('',#71712,0.0999999999999995) ;
#6759=CYLINDRICAL_SURFACE('',#71716,0.0999999999999994) ;
#6760=CYLINDRICAL_SURFACE('',#71718,0.0999999999999994) ;
#6761=CYLINDRICAL_SURFACE('',#71722,0.0999999999999998) ;
#6762=CYLINDRICAL_SURFACE('',#71723,0.0999999999999995) ;
#6763=CYLINDRICAL_SURFACE('',#71726,0.0999999999999994) ;
#6764=CYLINDRICAL_SURFACE('',#71730,0.0999999999999994) ;
#6765=CYLINDRICAL_SURFACE('',#71732,0.0999999999999994) ;
#6766=CYLINDRICAL_SURFACE('',#71736,0.0999999999999998) ;
#6767=CYLINDRICAL_SURFACE('',#71738,0.1) ;
#6768=CYLINDRICAL_SURFACE('',#71741,0.1) ;
#6769=CYLINDRICAL_SURFACE('',#71742,0.1) ;
#6770=CYLINDRICAL_SURFACE('',#71743,0.1) ;
#6771=CYLINDRICAL_SURFACE('',#71744,0.0999999999999994) ;
#6772=CYLINDRICAL_SURFACE('',#71745,0.0999999999999994) ;
#6773=CYLINDRICAL_SURFACE('',#71750,0.0999999999999994) ;
#6774=CYLINDRICAL_SURFACE('',#71753,0.0999999999999994) ;
#6775=CYLINDRICAL_SURFACE('',#71757,0.1) ;
#6776=CYLINDRICAL_SURFACE('',#71760,0.1) ;
#6777=CYLINDRICAL_SURFACE('',#71764,0.1) ;
#6778=CYLINDRICAL_SURFACE('',#71767,0.0999999999999994) ;
#6779=CYLINDRICAL_SURFACE('',#71769,0.0999999999999994) ;
#6780=CYLINDRICAL_SURFACE('',#71772,0.0999999999999994) ;
#6781=CYLINDRICAL_SURFACE('',#71774,0.0999999999999994) ;
#6782=CYLINDRICAL_SURFACE('',#71776,0.0999999999999994) ;
#6783=CYLINDRICAL_SURFACE('',#71778,0.0999999999999994) ;
#6784=CYLINDRICAL_SURFACE('',#71787,0.1) ;
#6785=CYLINDRICAL_SURFACE('',#71789,0.0999999999999994) ;
#6786=CYLINDRICAL_SURFACE('',#71795,0.0999999999999994) ;
#6787=CYLINDRICAL_SURFACE('',#71797,0.1) ;
#6788=CYLINDRICAL_SURFACE('',#71803,0.0999999999999994) ;
#6789=CYLINDRICAL_SURFACE('',#71805,0.0999999999999994) ;
#6790=CYLINDRICAL_SURFACE('',#71811,0.0999999999999994) ;
#6791=CYLINDRICAL_SURFACE('',#71813,0.0999999999999994) ;
#6792=CYLINDRICAL_SURFACE('',#71816,0.0999999999999994) ;
#6793=CYLINDRICAL_SURFACE('',#71822,0.0999999999999994) ;
#6794=CYLINDRICAL_SURFACE('',#71825,0.0999999999999994) ;
#6795=CYLINDRICAL_SURFACE('',#71828,0.0999999999999994) ;
#8351=LINE('',#101276,#12467) ;
#8352=LINE('',#101281,#12468) ;
#8353=LINE('',#101287,#12469) ;
#8354=LINE('',#101290,#12470) ;
#8355=LINE('',#101301,#12471) ;
#8356=LINE('',#101304,#12472) ;
#8357=LINE('',#101323,#12473) ;
#8358=LINE('',#101327,#12474) ;
#8359=LINE('',#101329,#12475) ;
#8360=LINE('',#101338,#12476) ;
#8361=LINE('',#101341,#12477) ;
#8362=LINE('',#101345,#12478) ;
#8363=LINE('',#101347,#12479) ;
#8364=LINE('',#101389,#12480) ;
#8365=LINE('',#101390,#12481) ;
#8366=LINE('',#101394,#12482) ;
#8367=LINE('',#101396,#12483) ;
#8368=LINE('',#101398,#12484) ;
#8369=LINE('',#101399,#12485) ;
#8370=LINE('',#101403,#12486) ;
#8371=LINE('',#101426,#12487) ;
#8372=LINE('',#101428,#12488) ;
#8373=LINE('',#101429,#12489) ;
#8374=LINE('',#101433,#12490) ;
#8375=LINE('',#101435,#12491) ;
#8376=LINE('',#101437,#12492) ;
#8377=LINE('',#101438,#12493) ;
#8378=LINE('',#101442,#12494) ;
#8379=LINE('',#101444,#12495) ;
#8380=LINE('',#101446,#12496) ;
#8381=LINE('',#101447,#12497) ;
#8382=LINE('',#101451,#12498) ;
#8383=LINE('',#101453,#12499) ;
#8384=LINE('',#101455,#12500) ;
#8385=LINE('',#101457,#12501) ;
#8386=LINE('',#101460,#12502) ;
#8387=LINE('',#101464,#12503) ;
#8388=LINE('',#101471,#12504) ;
#8389=LINE('',#101475,#12505) ;
#8390=LINE('',#101479,#12506) ;
#8391=LINE('',#101483,#12507) ;
#8392=LINE('',#101487,#12508) ;
#8393=LINE('',#101491,#12509) ;
#8394=LINE('',#101496,#12510) ;
#8395=LINE('',#101501,#12511) ;
#8396=LINE('',#101503,#12512) ;
#8397=LINE('',#101507,#12513) ;
#8398=LINE('',#101511,#12514) ;
#8399=LINE('',#101516,#12515) ;
#8400=LINE('',#101520,#12516) ;
#8401=LINE('',#101524,#12517) ;
#8402=LINE('',#101528,#12518) ;
#8403=LINE('',#101532,#12519) ;
#8404=LINE('',#101534,#12520) ;
#8405=LINE('',#101539,#12521) ;
#8406=LINE('',#101544,#12522) ;
#8407=LINE('',#101548,#12523) ;
#8408=LINE('',#101552,#12524) ;
#8409=LINE('',#101556,#12525) ;
#8410=LINE('',#101560,#12526) ;
#8411=LINE('',#101564,#12527) ;
#8412=LINE('',#101568,#12528) ;
#8413=LINE('',#101572,#12529) ;
#8414=LINE('',#101575,#12530) ;
#8415=LINE('',#101576,#12531) ;
#8416=LINE('',#101578,#12532) ;
#8417=LINE('',#101579,#12533) ;
#8418=LINE('',#101623,#12534) ;
#8419=LINE('',#101624,#12535) ;
#8420=LINE('',#101626,#12536) ;
#8421=LINE('',#101668,#12537) ;
#8422=LINE('',#101681,#12538) ;
#8423=LINE('',#101683,#12539) ;
#8424=LINE('',#101684,#12540) ;
#8425=LINE('',#101688,#12541) ;
#8426=LINE('',#101689,#12542) ;
#8427=LINE('',#101690,#12543) ;
#8428=LINE('',#101708,#12544) ;
#8429=LINE('',#101709,#12545) ;
#8430=LINE('',#101710,#12546) ;
#8431=LINE('',#101713,#12547) ;
#8432=LINE('',#101750,#12548) ;
#8433=LINE('',#101804,#12549) ;
#8434=LINE('',#101806,#12550) ;
#8435=LINE('',#101808,#12551) ;
#8436=LINE('',#101812,#12552) ;
#8437=LINE('',#101816,#12553) ;
#8438=LINE('',#101817,#12554) ;
#8439=LINE('',#101822,#12555) ;
#8440=LINE('',#101824,#12556) ;
#8441=LINE('',#101832,#12557) ;
#8442=LINE('',#101834,#12558) ;
#8443=LINE('',#101836,#12559) ;
#8444=LINE('',#101843,#12560) ;
#8445=LINE('',#101845,#12561) ;
#8446=LINE('',#101853,#12562) ;
#8447=LINE('',#101857,#12563) ;
#8448=LINE('',#101866,#12564) ;
#8449=LINE('',#101867,#12565) ;
#8450=LINE('',#101868,#12566) ;
#8451=LINE('',#101870,#12567) ;
#8452=LINE('',#101872,#12568) ;
#8453=LINE('',#101875,#12569) ;
#8454=LINE('',#101880,#12570) ;
#8455=LINE('',#101881,#12571) ;
#8456=LINE('',#101883,#12572) ;
#8457=LINE('',#101886,#12573) ;
#8458=LINE('',#101890,#12574) ;
#8459=LINE('',#101892,#12575) ;
#8460=LINE('',#101899,#12576) ;
#8461=LINE('',#101900,#12577) ;
#8462=LINE('',#101904,#12578) ;
#8463=LINE('',#101906,#12579) ;
#8464=LINE('',#101908,#12580) ;
#8465=LINE('',#101910,#12581) ;
#8466=LINE('',#101912,#12582) ;
#8467=LINE('',#101914,#12583) ;
#8468=LINE('',#101916,#12584) ;
#8469=LINE('',#101917,#12585) ;
#8470=LINE('',#101921,#12586) ;
#8471=LINE('',#101923,#12587) ;
#8472=LINE('',#101925,#12588) ;
#8473=LINE('',#101926,#12589) ;
#8474=LINE('',#101930,#12590) ;
#8475=LINE('',#101932,#12591) ;
#8476=LINE('',#101934,#12592) ;
#8477=LINE('',#101935,#12593) ;
#8478=LINE('',#101939,#12594) ;
#8479=LINE('',#101941,#12595) ;
#8480=LINE('',#101943,#12596) ;
#8481=LINE('',#101944,#12597) ;
#8482=LINE('',#101957,#12598) ;
#8483=LINE('',#101959,#12599) ;
#8484=LINE('',#101961,#12600) ;
#8485=LINE('',#101971,#12601) ;
#8486=LINE('',#101975,#12602) ;
#8487=LINE('',#101977,#12603) ;
#8488=LINE('',#101979,#12604) ;
#8489=LINE('',#101981,#12605) ;
#8490=LINE('',#101983,#12606) ;
#8491=LINE('',#101985,#12607) ;
#8492=LINE('',#101987,#12608) ;
#8493=LINE('',#101988,#12609) ;
#8494=LINE('',#101992,#12610) ;
#8495=LINE('',#101996,#12611) ;
#8496=LINE('',#102000,#12612) ;
#8497=LINE('',#102004,#12613) ;
#8498=LINE('',#102010,#12614) ;
#8499=LINE('',#102012,#12615) ;
#8500=LINE('',#102016,#12616) ;
#8501=LINE('',#102020,#12617) ;
#8502=LINE('',#102022,#12618) ;
#8503=LINE('',#102023,#12619) ;
#8504=LINE('',#102027,#12620) ;
#8505=LINE('',#102028,#12621) ;
#8506=LINE('',#102029,#12622) ;
#8507=LINE('',#102035,#12623) ;
#8508=LINE('',#102038,#12624) ;
#8509=LINE('',#102044,#12625) ;
#8510=LINE('',#102047,#12626) ;
#8511=LINE('',#102050,#12627) ;
#8512=LINE('',#102052,#12628) ;
#8513=LINE('',#102053,#12629) ;
#8514=LINE('',#102057,#12630) ;
#8515=LINE('',#102058,#12631) ;
#8516=LINE('',#102059,#12632) ;
#8517=LINE('',#102064,#12633) ;
#8518=LINE('',#102066,#12634) ;
#8519=LINE('',#102071,#12635) ;
#8520=LINE('',#102076,#12636) ;
#8521=LINE('',#102078,#12637) ;
#8522=LINE('',#102079,#12638) ;
#8523=LINE('',#102083,#12639) ;
#8524=LINE('',#102084,#12640) ;
#8525=LINE('',#102085,#12641) ;
#8526=LINE('',#102091,#12642) ;
#8527=LINE('',#102094,#12643) ;
#8528=LINE('',#102098,#12644) ;
#8529=LINE('',#102100,#12645) ;
#8530=LINE('',#102102,#12646) ;
#8531=LINE('',#102103,#12647) ;
#8532=LINE('',#102109,#12648) ;
#8533=LINE('',#102112,#12649) ;
#8534=LINE('',#102115,#12650) ;
#8535=LINE('',#102117,#12651) ;
#8536=LINE('',#102118,#12652) ;
#8537=LINE('',#102122,#12653) ;
#8538=LINE('',#102124,#12654) ;
#8539=LINE('',#102126,#12655) ;
#8540=LINE('',#102127,#12656) ;
#8541=LINE('',#102131,#12657) ;
#8542=LINE('',#102132,#12658) ;
#8543=LINE('',#102134,#12659) ;
#8544=LINE('',#102139,#12660) ;
#8545=LINE('',#102141,#12661) ;
#8546=LINE('',#102143,#12662) ;
#8547=LINE('',#102144,#12663) ;
#8548=LINE('',#102149,#12664) ;
#8549=LINE('',#102151,#12665) ;
#8550=LINE('',#102155,#12666) ;
#8551=LINE('',#102158,#12667) ;
#8552=LINE('',#102162,#12668) ;
#8553=LINE('',#102163,#12669) ;
#8554=LINE('',#102165,#12670) ;
#8555=LINE('',#102166,#12671) ;
#8556=LINE('',#102170,#12672) ;
#8557=LINE('',#102172,#12673) ;
#8558=LINE('',#102174,#12674) ;
#8559=LINE('',#102175,#12675) ;
#8560=LINE('',#102179,#12676) ;
#8561=LINE('',#102181,#12677) ;
#8562=LINE('',#102183,#12678) ;
#8563=LINE('',#102184,#12679) ;
#8564=LINE('',#102188,#12680) ;
#8565=LINE('',#102190,#12681) ;
#8566=LINE('',#102192,#12682) ;
#8567=LINE('',#102193,#12683) ;
#8568=LINE('',#102196,#12684) ;
#8569=LINE('',#102198,#12685) ;
#8570=LINE('',#102199,#12686) ;
#8571=LINE('',#102202,#12687) ;
#8572=LINE('',#102204,#12688) ;
#8573=LINE('',#102205,#12689) ;
#8574=LINE('',#102208,#12690) ;
#8575=LINE('',#102210,#12691) ;
#8576=LINE('',#102211,#12692) ;
#8577=LINE('',#102214,#12693) ;
#8578=LINE('',#102216,#12694) ;
#8579=LINE('',#102217,#12695) ;
#8580=LINE('',#102221,#12696) ;
#8581=LINE('',#102223,#12697) ;
#8582=LINE('',#102225,#12698) ;
#8583=LINE('',#102229,#12699) ;
#8584=LINE('',#102234,#12700) ;
#8585=LINE('',#102236,#12701) ;
#8586=LINE('',#102238,#12702) ;
#8587=LINE('',#102242,#12703) ;
#8588=LINE('',#102247,#12704) ;
#8589=LINE('',#102252,#12705) ;
#8590=LINE('',#102254,#12706) ;
#8591=LINE('',#102255,#12707) ;
#8592=LINE('',#102259,#12708) ;
#8593=LINE('',#102261,#12709) ;
#8594=LINE('',#102263,#12710) ;
#8595=LINE('',#102264,#12711) ;
#8596=LINE('',#102268,#12712) ;
#8597=LINE('',#102270,#12713) ;
#8598=LINE('',#102272,#12714) ;
#8599=LINE('',#102273,#12715) ;
#8600=LINE('',#102277,#12716) ;
#8601=LINE('',#102279,#12717) ;
#8602=LINE('',#102281,#12718) ;
#8603=LINE('',#102282,#12719) ;
#8604=LINE('',#102286,#12720) ;
#8605=LINE('',#102288,#12721) ;
#8606=LINE('',#102290,#12722) ;
#8607=LINE('',#102291,#12723) ;
#8608=LINE('',#102298,#12724) ;
#8609=LINE('',#102300,#12725) ;
#8610=LINE('',#102302,#12726) ;
#8611=LINE('',#102303,#12727) ;
#8612=LINE('',#102307,#12728) ;
#8613=LINE('',#102309,#12729) ;
#8614=LINE('',#102311,#12730) ;
#8615=LINE('',#102312,#12731) ;
#8616=LINE('',#102316,#12732) ;
#8617=LINE('',#102318,#12733) ;
#8618=LINE('',#102320,#12734) ;
#8619=LINE('',#102321,#12735) ;
#8620=LINE('',#102325,#12736) ;
#8621=LINE('',#102327,#12737) ;
#8622=LINE('',#102329,#12738) ;
#8623=LINE('',#102330,#12739) ;
#8624=LINE('',#102333,#12740) ;
#8625=LINE('',#102336,#12741) ;
#8626=LINE('',#102345,#12742) ;
#8627=LINE('',#102348,#12743) ;
#8628=LINE('',#102529,#12744) ;
#8629=LINE('',#102574,#12745) ;
#8630=LINE('',#102582,#12746) ;
#8631=LINE('',#102603,#12747) ;
#8632=LINE('',#102609,#12748) ;
#8633=LINE('',#102622,#12749) ;
#8634=LINE('',#103788,#12750) ;
#8635=LINE('',#103793,#12751) ;
#8636=LINE('',#103799,#12752) ;
#8637=LINE('',#103802,#12753) ;
#8638=LINE('',#103813,#12754) ;
#8639=LINE('',#103816,#12755) ;
#8640=LINE('',#103835,#12756) ;
#8641=LINE('',#103839,#12757) ;
#8642=LINE('',#103841,#12758) ;
#8643=LINE('',#103850,#12759) ;
#8644=LINE('',#103853,#12760) ;
#8645=LINE('',#103857,#12761) ;
#8646=LINE('',#103859,#12762) ;
#8647=LINE('',#103901,#12763) ;
#8648=LINE('',#103902,#12764) ;
#8649=LINE('',#103906,#12765) ;
#8650=LINE('',#103908,#12766) ;
#8651=LINE('',#103910,#12767) ;
#8652=LINE('',#103911,#12768) ;
#8653=LINE('',#103915,#12769) ;
#8654=LINE('',#103938,#12770) ;
#8655=LINE('',#103940,#12771) ;
#8656=LINE('',#103941,#12772) ;
#8657=LINE('',#103945,#12773) ;
#8658=LINE('',#103947,#12774) ;
#8659=LINE('',#103949,#12775) ;
#8660=LINE('',#103950,#12776) ;
#8661=LINE('',#103954,#12777) ;
#8662=LINE('',#103956,#12778) ;
#8663=LINE('',#103958,#12779) ;
#8664=LINE('',#103959,#12780) ;
#8665=LINE('',#103963,#12781) ;
#8666=LINE('',#103965,#12782) ;
#8667=LINE('',#103967,#12783) ;
#8668=LINE('',#103969,#12784) ;
#8669=LINE('',#103972,#12785) ;
#8670=LINE('',#103976,#12786) ;
#8671=LINE('',#103983,#12787) ;
#8672=LINE('',#103987,#12788) ;
#8673=LINE('',#103991,#12789) ;
#8674=LINE('',#103995,#12790) ;
#8675=LINE('',#103999,#12791) ;
#8676=LINE('',#104003,#12792) ;
#8677=LINE('',#104008,#12793) ;
#8678=LINE('',#104013,#12794) ;
#8679=LINE('',#104015,#12795) ;
#8680=LINE('',#104019,#12796) ;
#8681=LINE('',#104023,#12797) ;
#8682=LINE('',#104028,#12798) ;
#8683=LINE('',#104032,#12799) ;
#8684=LINE('',#104036,#12800) ;
#8685=LINE('',#104040,#12801) ;
#8686=LINE('',#104044,#12802) ;
#8687=LINE('',#104046,#12803) ;
#8688=LINE('',#104051,#12804) ;
#8689=LINE('',#104056,#12805) ;
#8690=LINE('',#104060,#12806) ;
#8691=LINE('',#104064,#12807) ;
#8692=LINE('',#104068,#12808) ;
#8693=LINE('',#104072,#12809) ;
#8694=LINE('',#104076,#12810) ;
#8695=LINE('',#104080,#12811) ;
#8696=LINE('',#104084,#12812) ;
#8697=LINE('',#104087,#12813) ;
#8698=LINE('',#104088,#12814) ;
#8699=LINE('',#104090,#12815) ;
#8700=LINE('',#104091,#12816) ;
#8701=LINE('',#104135,#12817) ;
#8702=LINE('',#104136,#12818) ;
#8703=LINE('',#104138,#12819) ;
#8704=LINE('',#104180,#12820) ;
#8705=LINE('',#104193,#12821) ;
#8706=LINE('',#104195,#12822) ;
#8707=LINE('',#104196,#12823) ;
#8708=LINE('',#104200,#12824) ;
#8709=LINE('',#104201,#12825) ;
#8710=LINE('',#104202,#12826) ;
#8711=LINE('',#104220,#12827) ;
#8712=LINE('',#104221,#12828) ;
#8713=LINE('',#104222,#12829) ;
#8714=LINE('',#104225,#12830) ;
#8715=LINE('',#104262,#12831) ;
#8716=LINE('',#104316,#12832) ;
#8717=LINE('',#104318,#12833) ;
#8718=LINE('',#104320,#12834) ;
#8719=LINE('',#104324,#12835) ;
#8720=LINE('',#104328,#12836) ;
#8721=LINE('',#104329,#12837) ;
#8722=LINE('',#104334,#12838) ;
#8723=LINE('',#104336,#12839) ;
#8724=LINE('',#104344,#12840) ;
#8725=LINE('',#104346,#12841) ;
#8726=LINE('',#104348,#12842) ;
#8727=LINE('',#104355,#12843) ;
#8728=LINE('',#104357,#12844) ;
#8729=LINE('',#104365,#12845) ;
#8730=LINE('',#104369,#12846) ;
#8731=LINE('',#104378,#12847) ;
#8732=LINE('',#104379,#12848) ;
#8733=LINE('',#104380,#12849) ;
#8734=LINE('',#104382,#12850) ;
#8735=LINE('',#104384,#12851) ;
#8736=LINE('',#104387,#12852) ;
#8737=LINE('',#104392,#12853) ;
#8738=LINE('',#104393,#12854) ;
#8739=LINE('',#104395,#12855) ;
#8740=LINE('',#104398,#12856) ;
#8741=LINE('',#104402,#12857) ;
#8742=LINE('',#104404,#12858) ;
#8743=LINE('',#104411,#12859) ;
#8744=LINE('',#104412,#12860) ;
#8745=LINE('',#104416,#12861) ;
#8746=LINE('',#104418,#12862) ;
#8747=LINE('',#104420,#12863) ;
#8748=LINE('',#104422,#12864) ;
#8749=LINE('',#104424,#12865) ;
#8750=LINE('',#104426,#12866) ;
#8751=LINE('',#104428,#12867) ;
#8752=LINE('',#104429,#12868) ;
#8753=LINE('',#104433,#12869) ;
#8754=LINE('',#104435,#12870) ;
#8755=LINE('',#104437,#12871) ;
#8756=LINE('',#104438,#12872) ;
#8757=LINE('',#104442,#12873) ;
#8758=LINE('',#104444,#12874) ;
#8759=LINE('',#104446,#12875) ;
#8760=LINE('',#104447,#12876) ;
#8761=LINE('',#104451,#12877) ;
#8762=LINE('',#104453,#12878) ;
#8763=LINE('',#104455,#12879) ;
#8764=LINE('',#104456,#12880) ;
#8765=LINE('',#104469,#12881) ;
#8766=LINE('',#104471,#12882) ;
#8767=LINE('',#104473,#12883) ;
#8768=LINE('',#104483,#12884) ;
#8769=LINE('',#104487,#12885) ;
#8770=LINE('',#104489,#12886) ;
#8771=LINE('',#104491,#12887) ;
#8772=LINE('',#104493,#12888) ;
#8773=LINE('',#104495,#12889) ;
#8774=LINE('',#104497,#12890) ;
#8775=LINE('',#104499,#12891) ;
#8776=LINE('',#104500,#12892) ;
#8777=LINE('',#104504,#12893) ;
#8778=LINE('',#104508,#12894) ;
#8779=LINE('',#104512,#12895) ;
#8780=LINE('',#104516,#12896) ;
#8781=LINE('',#104522,#12897) ;
#8782=LINE('',#104524,#12898) ;
#8783=LINE('',#104528,#12899) ;
#8784=LINE('',#104532,#12900) ;
#8785=LINE('',#104534,#12901) ;
#8786=LINE('',#104535,#12902) ;
#8787=LINE('',#104539,#12903) ;
#8788=LINE('',#104540,#12904) ;
#8789=LINE('',#104541,#12905) ;
#8790=LINE('',#104547,#12906) ;
#8791=LINE('',#104550,#12907) ;
#8792=LINE('',#104556,#12908) ;
#8793=LINE('',#104559,#12909) ;
#8794=LINE('',#104562,#12910) ;
#8795=LINE('',#104564,#12911) ;
#8796=LINE('',#104565,#12912) ;
#8797=LINE('',#104569,#12913) ;
#8798=LINE('',#104570,#12914) ;
#8799=LINE('',#104571,#12915) ;
#8800=LINE('',#104576,#12916) ;
#8801=LINE('',#104578,#12917) ;
#8802=LINE('',#104583,#12918) ;
#8803=LINE('',#104588,#12919) ;
#8804=LINE('',#104590,#12920) ;
#8805=LINE('',#104591,#12921) ;
#8806=LINE('',#104595,#12922) ;
#8807=LINE('',#104596,#12923) ;
#8808=LINE('',#104597,#12924) ;
#8809=LINE('',#104603,#12925) ;
#8810=LINE('',#104606,#12926) ;
#8811=LINE('',#104610,#12927) ;
#8812=LINE('',#104612,#12928) ;
#8813=LINE('',#104614,#12929) ;
#8814=LINE('',#104615,#12930) ;
#8815=LINE('',#104621,#12931) ;
#8816=LINE('',#104624,#12932) ;
#8817=LINE('',#104627,#12933) ;
#8818=LINE('',#104629,#12934) ;
#8819=LINE('',#104630,#12935) ;
#8820=LINE('',#104634,#12936) ;
#8821=LINE('',#104636,#12937) ;
#8822=LINE('',#104638,#12938) ;
#8823=LINE('',#104639,#12939) ;
#8824=LINE('',#104643,#12940) ;
#8825=LINE('',#104644,#12941) ;
#8826=LINE('',#104646,#12942) ;
#8827=LINE('',#104651,#12943) ;
#8828=LINE('',#104653,#12944) ;
#8829=LINE('',#104655,#12945) ;
#8830=LINE('',#104656,#12946) ;
#8831=LINE('',#104661,#12947) ;
#8832=LINE('',#104663,#12948) ;
#8833=LINE('',#104667,#12949) ;
#8834=LINE('',#104670,#12950) ;
#8835=LINE('',#104674,#12951) ;
#8836=LINE('',#104675,#12952) ;
#8837=LINE('',#104677,#12953) ;
#8838=LINE('',#104678,#12954) ;
#8839=LINE('',#104682,#12955) ;
#8840=LINE('',#104684,#12956) ;
#8841=LINE('',#104686,#12957) ;
#8842=LINE('',#104687,#12958) ;
#8843=LINE('',#104691,#12959) ;
#8844=LINE('',#104693,#12960) ;
#8845=LINE('',#104695,#12961) ;
#8846=LINE('',#104696,#12962) ;
#8847=LINE('',#104700,#12963) ;
#8848=LINE('',#104702,#12964) ;
#8849=LINE('',#104704,#12965) ;
#8850=LINE('',#104705,#12966) ;
#8851=LINE('',#104708,#12967) ;
#8852=LINE('',#104710,#12968) ;
#8853=LINE('',#104711,#12969) ;
#8854=LINE('',#104714,#12970) ;
#8855=LINE('',#104716,#12971) ;
#8856=LINE('',#104717,#12972) ;
#8857=LINE('',#104720,#12973) ;
#8858=LINE('',#104722,#12974) ;
#8859=LINE('',#104723,#12975) ;
#8860=LINE('',#104726,#12976) ;
#8861=LINE('',#104728,#12977) ;
#8862=LINE('',#104729,#12978) ;
#8863=LINE('',#104733,#12979) ;
#8864=LINE('',#104735,#12980) ;
#8865=LINE('',#104737,#12981) ;
#8866=LINE('',#104741,#12982) ;
#8867=LINE('',#104746,#12983) ;
#8868=LINE('',#104748,#12984) ;
#8869=LINE('',#104750,#12985) ;
#8870=LINE('',#104754,#12986) ;
#8871=LINE('',#104759,#12987) ;
#8872=LINE('',#104764,#12988) ;
#8873=LINE('',#104766,#12989) ;
#8874=LINE('',#104767,#12990) ;
#8875=LINE('',#104771,#12991) ;
#8876=LINE('',#104773,#12992) ;
#8877=LINE('',#104775,#12993) ;
#8878=LINE('',#104776,#12994) ;
#8879=LINE('',#104780,#12995) ;
#8880=LINE('',#104782,#12996) ;
#8881=LINE('',#104784,#12997) ;
#8882=LINE('',#104785,#12998) ;
#8883=LINE('',#104789,#12999) ;
#8884=LINE('',#104791,#13000) ;
#8885=LINE('',#104793,#13001) ;
#8886=LINE('',#104794,#13002) ;
#8887=LINE('',#104798,#13003) ;
#8888=LINE('',#104800,#13004) ;
#8889=LINE('',#104802,#13005) ;
#8890=LINE('',#104803,#13006) ;
#8891=LINE('',#104810,#13007) ;
#8892=LINE('',#104812,#13008) ;
#8893=LINE('',#104814,#13009) ;
#8894=LINE('',#104815,#13010) ;
#8895=LINE('',#104819,#13011) ;
#8896=LINE('',#104821,#13012) ;
#8897=LINE('',#104823,#13013) ;
#8898=LINE('',#104824,#13014) ;
#8899=LINE('',#104828,#13015) ;
#8900=LINE('',#104830,#13016) ;
#8901=LINE('',#104832,#13017) ;
#8902=LINE('',#104833,#13018) ;
#8903=LINE('',#104837,#13019) ;
#8904=LINE('',#104839,#13020) ;
#8905=LINE('',#104841,#13021) ;
#8906=LINE('',#104842,#13022) ;
#8907=LINE('',#104845,#13023) ;
#8908=LINE('',#104848,#13024) ;
#8909=LINE('',#104857,#13025) ;
#8910=LINE('',#104860,#13026) ;
#8911=LINE('',#105041,#13027) ;
#8912=LINE('',#105086,#13028) ;
#8913=LINE('',#105094,#13029) ;
#8914=LINE('',#105115,#13030) ;
#8915=LINE('',#105121,#13031) ;
#8916=LINE('',#105134,#13032) ;
#8917=LINE('',#106300,#13033) ;
#8918=LINE('',#106305,#13034) ;
#8919=LINE('',#106311,#13035) ;
#8920=LINE('',#106314,#13036) ;
#8921=LINE('',#106325,#13037) ;
#8922=LINE('',#106328,#13038) ;
#8923=LINE('',#106347,#13039) ;
#8924=LINE('',#106351,#13040) ;
#8925=LINE('',#106353,#13041) ;
#8926=LINE('',#106362,#13042) ;
#8927=LINE('',#106365,#13043) ;
#8928=LINE('',#106369,#13044) ;
#8929=LINE('',#106371,#13045) ;
#8930=LINE('',#106413,#13046) ;
#8931=LINE('',#106414,#13047) ;
#8932=LINE('',#106418,#13048) ;
#8933=LINE('',#106420,#13049) ;
#8934=LINE('',#106422,#13050) ;
#8935=LINE('',#106423,#13051) ;
#8936=LINE('',#106427,#13052) ;
#8937=LINE('',#106450,#13053) ;
#8938=LINE('',#106452,#13054) ;
#8939=LINE('',#106453,#13055) ;
#8940=LINE('',#106457,#13056) ;
#8941=LINE('',#106459,#13057) ;
#8942=LINE('',#106461,#13058) ;
#8943=LINE('',#106462,#13059) ;
#8944=LINE('',#106466,#13060) ;
#8945=LINE('',#106468,#13061) ;
#8946=LINE('',#106470,#13062) ;
#8947=LINE('',#106471,#13063) ;
#8948=LINE('',#106475,#13064) ;
#8949=LINE('',#106477,#13065) ;
#8950=LINE('',#106479,#13066) ;
#8951=LINE('',#106481,#13067) ;
#8952=LINE('',#106484,#13068) ;
#8953=LINE('',#106488,#13069) ;
#8954=LINE('',#106495,#13070) ;
#8955=LINE('',#106499,#13071) ;
#8956=LINE('',#106503,#13072) ;
#8957=LINE('',#106507,#13073) ;
#8958=LINE('',#106511,#13074) ;
#8959=LINE('',#106515,#13075) ;
#8960=LINE('',#106520,#13076) ;
#8961=LINE('',#106525,#13077) ;
#8962=LINE('',#106527,#13078) ;
#8963=LINE('',#106531,#13079) ;
#8964=LINE('',#106535,#13080) ;
#8965=LINE('',#106540,#13081) ;
#8966=LINE('',#106544,#13082) ;
#8967=LINE('',#106548,#13083) ;
#8968=LINE('',#106552,#13084) ;
#8969=LINE('',#106556,#13085) ;
#8970=LINE('',#106558,#13086) ;
#8971=LINE('',#106563,#13087) ;
#8972=LINE('',#106568,#13088) ;
#8973=LINE('',#106572,#13089) ;
#8974=LINE('',#106576,#13090) ;
#8975=LINE('',#106580,#13091) ;
#8976=LINE('',#106584,#13092) ;
#8977=LINE('',#106588,#13093) ;
#8978=LINE('',#106592,#13094) ;
#8979=LINE('',#106596,#13095) ;
#8980=LINE('',#106599,#13096) ;
#8981=LINE('',#106600,#13097) ;
#8982=LINE('',#106602,#13098) ;
#8983=LINE('',#106603,#13099) ;
#8984=LINE('',#106647,#13100) ;
#8985=LINE('',#106648,#13101) ;
#8986=LINE('',#106650,#13102) ;
#8987=LINE('',#106692,#13103) ;
#8988=LINE('',#106705,#13104) ;
#8989=LINE('',#106707,#13105) ;
#8990=LINE('',#106708,#13106) ;
#8991=LINE('',#106712,#13107) ;
#8992=LINE('',#106713,#13108) ;
#8993=LINE('',#106714,#13109) ;
#8994=LINE('',#106732,#13110) ;
#8995=LINE('',#106733,#13111) ;
#8996=LINE('',#106734,#13112) ;
#8997=LINE('',#106737,#13113) ;
#8998=LINE('',#106774,#13114) ;
#8999=LINE('',#106828,#13115) ;
#9000=LINE('',#106830,#13116) ;
#9001=LINE('',#106832,#13117) ;
#9002=LINE('',#106836,#13118) ;
#9003=LINE('',#106840,#13119) ;
#9004=LINE('',#106841,#13120) ;
#9005=LINE('',#106846,#13121) ;
#9006=LINE('',#106848,#13122) ;
#9007=LINE('',#106856,#13123) ;
#9008=LINE('',#106858,#13124) ;
#9009=LINE('',#106860,#13125) ;
#9010=LINE('',#106867,#13126) ;
#9011=LINE('',#106869,#13127) ;
#9012=LINE('',#106877,#13128) ;
#9013=LINE('',#106881,#13129) ;
#9014=LINE('',#106890,#13130) ;
#9015=LINE('',#106891,#13131) ;
#9016=LINE('',#106892,#13132) ;
#9017=LINE('',#106894,#13133) ;
#9018=LINE('',#106896,#13134) ;
#9019=LINE('',#106899,#13135) ;
#9020=LINE('',#106904,#13136) ;
#9021=LINE('',#106905,#13137) ;
#9022=LINE('',#106907,#13138) ;
#9023=LINE('',#106910,#13139) ;
#9024=LINE('',#106914,#13140) ;
#9025=LINE('',#106916,#13141) ;
#9026=LINE('',#106923,#13142) ;
#9027=LINE('',#106924,#13143) ;
#9028=LINE('',#106928,#13144) ;
#9029=LINE('',#106930,#13145) ;
#9030=LINE('',#106932,#13146) ;
#9031=LINE('',#106934,#13147) ;
#9032=LINE('',#106936,#13148) ;
#9033=LINE('',#106938,#13149) ;
#9034=LINE('',#106940,#13150) ;
#9035=LINE('',#106941,#13151) ;
#9036=LINE('',#106945,#13152) ;
#9037=LINE('',#106947,#13153) ;
#9038=LINE('',#106949,#13154) ;
#9039=LINE('',#106950,#13155) ;
#9040=LINE('',#106954,#13156) ;
#9041=LINE('',#106956,#13157) ;
#9042=LINE('',#106958,#13158) ;
#9043=LINE('',#106959,#13159) ;
#9044=LINE('',#106963,#13160) ;
#9045=LINE('',#106965,#13161) ;
#9046=LINE('',#106967,#13162) ;
#9047=LINE('',#106968,#13163) ;
#9048=LINE('',#106981,#13164) ;
#9049=LINE('',#106983,#13165) ;
#9050=LINE('',#106985,#13166) ;
#9051=LINE('',#106995,#13167) ;
#9052=LINE('',#106999,#13168) ;
#9053=LINE('',#107001,#13169) ;
#9054=LINE('',#107003,#13170) ;
#9055=LINE('',#107005,#13171) ;
#9056=LINE('',#107007,#13172) ;
#9057=LINE('',#107009,#13173) ;
#9058=LINE('',#107011,#13174) ;
#9059=LINE('',#107012,#13175) ;
#9060=LINE('',#107016,#13176) ;
#9061=LINE('',#107020,#13177) ;
#9062=LINE('',#107024,#13178) ;
#9063=LINE('',#107028,#13179) ;
#9064=LINE('',#107034,#13180) ;
#9065=LINE('',#107036,#13181) ;
#9066=LINE('',#107040,#13182) ;
#9067=LINE('',#107044,#13183) ;
#9068=LINE('',#107046,#13184) ;
#9069=LINE('',#107047,#13185) ;
#9070=LINE('',#107051,#13186) ;
#9071=LINE('',#107052,#13187) ;
#9072=LINE('',#107053,#13188) ;
#9073=LINE('',#107059,#13189) ;
#9074=LINE('',#107062,#13190) ;
#9075=LINE('',#107068,#13191) ;
#9076=LINE('',#107071,#13192) ;
#9077=LINE('',#107074,#13193) ;
#9078=LINE('',#107076,#13194) ;
#9079=LINE('',#107077,#13195) ;
#9080=LINE('',#107081,#13196) ;
#9081=LINE('',#107082,#13197) ;
#9082=LINE('',#107083,#13198) ;
#9083=LINE('',#107088,#13199) ;
#9084=LINE('',#107090,#13200) ;
#9085=LINE('',#107095,#13201) ;
#9086=LINE('',#107100,#13202) ;
#9087=LINE('',#107102,#13203) ;
#9088=LINE('',#107103,#13204) ;
#9089=LINE('',#107107,#13205) ;
#9090=LINE('',#107108,#13206) ;
#9091=LINE('',#107109,#13207) ;
#9092=LINE('',#107115,#13208) ;
#9093=LINE('',#107118,#13209) ;
#9094=LINE('',#107122,#13210) ;
#9095=LINE('',#107124,#13211) ;
#9096=LINE('',#107126,#13212) ;
#9097=LINE('',#107127,#13213) ;
#9098=LINE('',#107133,#13214) ;
#9099=LINE('',#107136,#13215) ;
#9100=LINE('',#107139,#13216) ;
#9101=LINE('',#107141,#13217) ;
#9102=LINE('',#107142,#13218) ;
#9103=LINE('',#107146,#13219) ;
#9104=LINE('',#107148,#13220) ;
#9105=LINE('',#107150,#13221) ;
#9106=LINE('',#107151,#13222) ;
#9107=LINE('',#107155,#13223) ;
#9108=LINE('',#107156,#13224) ;
#9109=LINE('',#107158,#13225) ;
#9110=LINE('',#107163,#13226) ;
#9111=LINE('',#107165,#13227) ;
#9112=LINE('',#107167,#13228) ;
#9113=LINE('',#107168,#13229) ;
#9114=LINE('',#107173,#13230) ;
#9115=LINE('',#107175,#13231) ;
#9116=LINE('',#107179,#13232) ;
#9117=LINE('',#107182,#13233) ;
#9118=LINE('',#107186,#13234) ;
#9119=LINE('',#107187,#13235) ;
#9120=LINE('',#107189,#13236) ;
#9121=LINE('',#107190,#13237) ;
#9122=LINE('',#107194,#13238) ;
#9123=LINE('',#107196,#13239) ;
#9124=LINE('',#107198,#13240) ;
#9125=LINE('',#107199,#13241) ;
#9126=LINE('',#107203,#13242) ;
#9127=LINE('',#107205,#13243) ;
#9128=LINE('',#107207,#13244) ;
#9129=LINE('',#107208,#13245) ;
#9130=LINE('',#107212,#13246) ;
#9131=LINE('',#107214,#13247) ;
#9132=LINE('',#107216,#13248) ;
#9133=LINE('',#107217,#13249) ;
#9134=LINE('',#107220,#13250) ;
#9135=LINE('',#107222,#13251) ;
#9136=LINE('',#107223,#13252) ;
#9137=LINE('',#107226,#13253) ;
#9138=LINE('',#107228,#13254) ;
#9139=LINE('',#107229,#13255) ;
#9140=LINE('',#107232,#13256) ;
#9141=LINE('',#107234,#13257) ;
#9142=LINE('',#107235,#13258) ;
#9143=LINE('',#107238,#13259) ;
#9144=LINE('',#107240,#13260) ;
#9145=LINE('',#107241,#13261) ;
#9146=LINE('',#107245,#13262) ;
#9147=LINE('',#107247,#13263) ;
#9148=LINE('',#107249,#13264) ;
#9149=LINE('',#107253,#13265) ;
#9150=LINE('',#107258,#13266) ;
#9151=LINE('',#107260,#13267) ;
#9152=LINE('',#107262,#13268) ;
#9153=LINE('',#107266,#13269) ;
#9154=LINE('',#107271,#13270) ;
#9155=LINE('',#107276,#13271) ;
#9156=LINE('',#107278,#13272) ;
#9157=LINE('',#107279,#13273) ;
#9158=LINE('',#107283,#13274) ;
#9159=LINE('',#107285,#13275) ;
#9160=LINE('',#107287,#13276) ;
#9161=LINE('',#107288,#13277) ;
#9162=LINE('',#107292,#13278) ;
#9163=LINE('',#107294,#13279) ;
#9164=LINE('',#107296,#13280) ;
#9165=LINE('',#107297,#13281) ;
#9166=LINE('',#107301,#13282) ;
#9167=LINE('',#107303,#13283) ;
#9168=LINE('',#107305,#13284) ;
#9169=LINE('',#107306,#13285) ;
#9170=LINE('',#107310,#13286) ;
#9171=LINE('',#107312,#13287) ;
#9172=LINE('',#107314,#13288) ;
#9173=LINE('',#107315,#13289) ;
#9174=LINE('',#107322,#13290) ;
#9175=LINE('',#107324,#13291) ;
#9176=LINE('',#107326,#13292) ;
#9177=LINE('',#107327,#13293) ;
#9178=LINE('',#107331,#13294) ;
#9179=LINE('',#107333,#13295) ;
#9180=LINE('',#107335,#13296) ;
#9181=LINE('',#107336,#13297) ;
#9182=LINE('',#107340,#13298) ;
#9183=LINE('',#107342,#13299) ;
#9184=LINE('',#107344,#13300) ;
#9185=LINE('',#107345,#13301) ;
#9186=LINE('',#107349,#13302) ;
#9187=LINE('',#107351,#13303) ;
#9188=LINE('',#107353,#13304) ;
#9189=LINE('',#107354,#13305) ;
#9190=LINE('',#107357,#13306) ;
#9191=LINE('',#107360,#13307) ;
#9192=LINE('',#107369,#13308) ;
#9193=LINE('',#107372,#13309) ;
#9194=LINE('',#107553,#13310) ;
#9195=LINE('',#107598,#13311) ;
#9196=LINE('',#107606,#13312) ;
#9197=LINE('',#107627,#13313) ;
#9198=LINE('',#107633,#13314) ;
#9199=LINE('',#107646,#13315) ;
#9200=LINE('',#108812,#13316) ;
#9201=LINE('',#108817,#13317) ;
#9202=LINE('',#108823,#13318) ;
#9203=LINE('',#108826,#13319) ;
#9204=LINE('',#108837,#13320) ;
#9205=LINE('',#108840,#13321) ;
#9206=LINE('',#108859,#13322) ;
#9207=LINE('',#108863,#13323) ;
#9208=LINE('',#108865,#13324) ;
#9209=LINE('',#108874,#13325) ;
#9210=LINE('',#108877,#13326) ;
#9211=LINE('',#108881,#13327) ;
#9212=LINE('',#108883,#13328) ;
#9213=LINE('',#108925,#13329) ;
#9214=LINE('',#108926,#13330) ;
#9215=LINE('',#108930,#13331) ;
#9216=LINE('',#108932,#13332) ;
#9217=LINE('',#108934,#13333) ;
#9218=LINE('',#108935,#13334) ;
#9219=LINE('',#108939,#13335) ;
#9220=LINE('',#108962,#13336) ;
#9221=LINE('',#108964,#13337) ;
#9222=LINE('',#108965,#13338) ;
#9223=LINE('',#108969,#13339) ;
#9224=LINE('',#108971,#13340) ;
#9225=LINE('',#108973,#13341) ;
#9226=LINE('',#108974,#13342) ;
#9227=LINE('',#108978,#13343) ;
#9228=LINE('',#108980,#13344) ;
#9229=LINE('',#108982,#13345) ;
#9230=LINE('',#108983,#13346) ;
#9231=LINE('',#108987,#13347) ;
#9232=LINE('',#108989,#13348) ;
#9233=LINE('',#108991,#13349) ;
#9234=LINE('',#108993,#13350) ;
#9235=LINE('',#108996,#13351) ;
#9236=LINE('',#109000,#13352) ;
#9237=LINE('',#109007,#13353) ;
#9238=LINE('',#109011,#13354) ;
#9239=LINE('',#109015,#13355) ;
#9240=LINE('',#109019,#13356) ;
#9241=LINE('',#109023,#13357) ;
#9242=LINE('',#109027,#13358) ;
#9243=LINE('',#109032,#13359) ;
#9244=LINE('',#109037,#13360) ;
#9245=LINE('',#109039,#13361) ;
#9246=LINE('',#109043,#13362) ;
#9247=LINE('',#109047,#13363) ;
#9248=LINE('',#109052,#13364) ;
#9249=LINE('',#109056,#13365) ;
#9250=LINE('',#109060,#13366) ;
#9251=LINE('',#109064,#13367) ;
#9252=LINE('',#109068,#13368) ;
#9253=LINE('',#109070,#13369) ;
#9254=LINE('',#109075,#13370) ;
#9255=LINE('',#109080,#13371) ;
#9256=LINE('',#109084,#13372) ;
#9257=LINE('',#109088,#13373) ;
#9258=LINE('',#109092,#13374) ;
#9259=LINE('',#109096,#13375) ;
#9260=LINE('',#109100,#13376) ;
#9261=LINE('',#109104,#13377) ;
#9262=LINE('',#109108,#13378) ;
#9263=LINE('',#109111,#13379) ;
#9264=LINE('',#109112,#13380) ;
#9265=LINE('',#109114,#13381) ;
#9266=LINE('',#109115,#13382) ;
#9267=LINE('',#109159,#13383) ;
#9268=LINE('',#109160,#13384) ;
#9269=LINE('',#109162,#13385) ;
#9270=LINE('',#109204,#13386) ;
#9271=LINE('',#109217,#13387) ;
#9272=LINE('',#109219,#13388) ;
#9273=LINE('',#109220,#13389) ;
#9274=LINE('',#109224,#13390) ;
#9275=LINE('',#109225,#13391) ;
#9276=LINE('',#109226,#13392) ;
#9277=LINE('',#109244,#13393) ;
#9278=LINE('',#109245,#13394) ;
#9279=LINE('',#109246,#13395) ;
#9280=LINE('',#109249,#13396) ;
#9281=LINE('',#109286,#13397) ;
#9282=LINE('',#109340,#13398) ;
#9283=LINE('',#109342,#13399) ;
#9284=LINE('',#109344,#13400) ;
#9285=LINE('',#109348,#13401) ;
#9286=LINE('',#109352,#13402) ;
#9287=LINE('',#109353,#13403) ;
#9288=LINE('',#109358,#13404) ;
#9289=LINE('',#109360,#13405) ;
#9290=LINE('',#109368,#13406) ;
#9291=LINE('',#109370,#13407) ;
#9292=LINE('',#109372,#13408) ;
#9293=LINE('',#109379,#13409) ;
#9294=LINE('',#109381,#13410) ;
#9295=LINE('',#109389,#13411) ;
#9296=LINE('',#109393,#13412) ;
#9297=LINE('',#109402,#13413) ;
#9298=LINE('',#109403,#13414) ;
#9299=LINE('',#109404,#13415) ;
#9300=LINE('',#109406,#13416) ;
#9301=LINE('',#109408,#13417) ;
#9302=LINE('',#109411,#13418) ;
#9303=LINE('',#109416,#13419) ;
#9304=LINE('',#109417,#13420) ;
#9305=LINE('',#109419,#13421) ;
#9306=LINE('',#109422,#13422) ;
#9307=LINE('',#109426,#13423) ;
#9308=LINE('',#109428,#13424) ;
#9309=LINE('',#109435,#13425) ;
#9310=LINE('',#109436,#13426) ;
#9311=LINE('',#109440,#13427) ;
#9312=LINE('',#109442,#13428) ;
#9313=LINE('',#109444,#13429) ;
#9314=LINE('',#109446,#13430) ;
#9315=LINE('',#109448,#13431) ;
#9316=LINE('',#109450,#13432) ;
#9317=LINE('',#109452,#13433) ;
#9318=LINE('',#109453,#13434) ;
#9319=LINE('',#109457,#13435) ;
#9320=LINE('',#109459,#13436) ;
#9321=LINE('',#109461,#13437) ;
#9322=LINE('',#109462,#13438) ;
#9323=LINE('',#109466,#13439) ;
#9324=LINE('',#109468,#13440) ;
#9325=LINE('',#109470,#13441) ;
#9326=LINE('',#109471,#13442) ;
#9327=LINE('',#109475,#13443) ;
#9328=LINE('',#109477,#13444) ;
#9329=LINE('',#109479,#13445) ;
#9330=LINE('',#109480,#13446) ;
#9331=LINE('',#109493,#13447) ;
#9332=LINE('',#109495,#13448) ;
#9333=LINE('',#109497,#13449) ;
#9334=LINE('',#109507,#13450) ;
#9335=LINE('',#109511,#13451) ;
#9336=LINE('',#109513,#13452) ;
#9337=LINE('',#109515,#13453) ;
#9338=LINE('',#109517,#13454) ;
#9339=LINE('',#109519,#13455) ;
#9340=LINE('',#109521,#13456) ;
#9341=LINE('',#109523,#13457) ;
#9342=LINE('',#109524,#13458) ;
#9343=LINE('',#109528,#13459) ;
#9344=LINE('',#109532,#13460) ;
#9345=LINE('',#109536,#13461) ;
#9346=LINE('',#109540,#13462) ;
#9347=LINE('',#109546,#13463) ;
#9348=LINE('',#109548,#13464) ;
#9349=LINE('',#109552,#13465) ;
#9350=LINE('',#109556,#13466) ;
#9351=LINE('',#109558,#13467) ;
#9352=LINE('',#109559,#13468) ;
#9353=LINE('',#109563,#13469) ;
#9354=LINE('',#109564,#13470) ;
#9355=LINE('',#109565,#13471) ;
#9356=LINE('',#109571,#13472) ;
#9357=LINE('',#109574,#13473) ;
#9358=LINE('',#109580,#13474) ;
#9359=LINE('',#109583,#13475) ;
#9360=LINE('',#109586,#13476) ;
#9361=LINE('',#109588,#13477) ;
#9362=LINE('',#109589,#13478) ;
#9363=LINE('',#109593,#13479) ;
#9364=LINE('',#109594,#13480) ;
#9365=LINE('',#109595,#13481) ;
#9366=LINE('',#109600,#13482) ;
#9367=LINE('',#109602,#13483) ;
#9368=LINE('',#109607,#13484) ;
#9369=LINE('',#109612,#13485) ;
#9370=LINE('',#109614,#13486) ;
#9371=LINE('',#109615,#13487) ;
#9372=LINE('',#109619,#13488) ;
#9373=LINE('',#109620,#13489) ;
#9374=LINE('',#109621,#13490) ;
#9375=LINE('',#109627,#13491) ;
#9376=LINE('',#109630,#13492) ;
#9377=LINE('',#109634,#13493) ;
#9378=LINE('',#109636,#13494) ;
#9379=LINE('',#109638,#13495) ;
#9380=LINE('',#109639,#13496) ;
#9381=LINE('',#109645,#13497) ;
#9382=LINE('',#109648,#13498) ;
#9383=LINE('',#109651,#13499) ;
#9384=LINE('',#109653,#13500) ;
#9385=LINE('',#109654,#13501) ;
#9386=LINE('',#109658,#13502) ;
#9387=LINE('',#109660,#13503) ;
#9388=LINE('',#109662,#13504) ;
#9389=LINE('',#109663,#13505) ;
#9390=LINE('',#109667,#13506) ;
#9391=LINE('',#109668,#13507) ;
#9392=LINE('',#109670,#13508) ;
#9393=LINE('',#109675,#13509) ;
#9394=LINE('',#109677,#13510) ;
#9395=LINE('',#109679,#13511) ;
#9396=LINE('',#109680,#13512) ;
#9397=LINE('',#109685,#13513) ;
#9398=LINE('',#109687,#13514) ;
#9399=LINE('',#109691,#13515) ;
#9400=LINE('',#109694,#13516) ;
#9401=LINE('',#109698,#13517) ;
#9402=LINE('',#109699,#13518) ;
#9403=LINE('',#109701,#13519) ;
#9404=LINE('',#109702,#13520) ;
#9405=LINE('',#109706,#13521) ;
#9406=LINE('',#109708,#13522) ;
#9407=LINE('',#109710,#13523) ;
#9408=LINE('',#109711,#13524) ;
#9409=LINE('',#109715,#13525) ;
#9410=LINE('',#109717,#13526) ;
#9411=LINE('',#109719,#13527) ;
#9412=LINE('',#109720,#13528) ;
#9413=LINE('',#109724,#13529) ;
#9414=LINE('',#109726,#13530) ;
#9415=LINE('',#109728,#13531) ;
#9416=LINE('',#109729,#13532) ;
#9417=LINE('',#109732,#13533) ;
#9418=LINE('',#109734,#13534) ;
#9419=LINE('',#109735,#13535) ;
#9420=LINE('',#109738,#13536) ;
#9421=LINE('',#109740,#13537) ;
#9422=LINE('',#109741,#13538) ;
#9423=LINE('',#109744,#13539) ;
#9424=LINE('',#109746,#13540) ;
#9425=LINE('',#109747,#13541) ;
#9426=LINE('',#109750,#13542) ;
#9427=LINE('',#109752,#13543) ;
#9428=LINE('',#109753,#13544) ;
#9429=LINE('',#109757,#13545) ;
#9430=LINE('',#109759,#13546) ;
#9431=LINE('',#109761,#13547) ;
#9432=LINE('',#109765,#13548) ;
#9433=LINE('',#109770,#13549) ;
#9434=LINE('',#109772,#13550) ;
#9435=LINE('',#109774,#13551) ;
#9436=LINE('',#109778,#13552) ;
#9437=LINE('',#109783,#13553) ;
#9438=LINE('',#109788,#13554) ;
#9439=LINE('',#109790,#13555) ;
#9440=LINE('',#109791,#13556) ;
#9441=LINE('',#109795,#13557) ;
#9442=LINE('',#109797,#13558) ;
#9443=LINE('',#109799,#13559) ;
#9444=LINE('',#109800,#13560) ;
#9445=LINE('',#109804,#13561) ;
#9446=LINE('',#109806,#13562) ;
#9447=LINE('',#109808,#13563) ;
#9448=LINE('',#109809,#13564) ;
#9449=LINE('',#109813,#13565) ;
#9450=LINE('',#109815,#13566) ;
#9451=LINE('',#109817,#13567) ;
#9452=LINE('',#109818,#13568) ;
#9453=LINE('',#109822,#13569) ;
#9454=LINE('',#109824,#13570) ;
#9455=LINE('',#109826,#13571) ;
#9456=LINE('',#109827,#13572) ;
#9457=LINE('',#109834,#13573) ;
#9458=LINE('',#109836,#13574) ;
#9459=LINE('',#109838,#13575) ;
#9460=LINE('',#109839,#13576) ;
#9461=LINE('',#109843,#13577) ;
#9462=LINE('',#109845,#13578) ;
#9463=LINE('',#109847,#13579) ;
#9464=LINE('',#109848,#13580) ;
#9465=LINE('',#109852,#13581) ;
#9466=LINE('',#109854,#13582) ;
#9467=LINE('',#109856,#13583) ;
#9468=LINE('',#109857,#13584) ;
#9469=LINE('',#109861,#13585) ;
#9470=LINE('',#109863,#13586) ;
#9471=LINE('',#109865,#13587) ;
#9472=LINE('',#109866,#13588) ;
#9473=LINE('',#109869,#13589) ;
#9474=LINE('',#109872,#13590) ;
#9475=LINE('',#109881,#13591) ;
#9476=LINE('',#109884,#13592) ;
#9477=LINE('',#110065,#13593) ;
#9478=LINE('',#110110,#13594) ;
#9479=LINE('',#110118,#13595) ;
#9480=LINE('',#110139,#13596) ;
#9481=LINE('',#110145,#13597) ;
#9482=LINE('',#110158,#13598) ;
#9483=LINE('',#111324,#13599) ;
#9484=LINE('',#111329,#13600) ;
#9485=LINE('',#111335,#13601) ;
#9486=LINE('',#111338,#13602) ;
#9487=LINE('',#111349,#13603) ;
#9488=LINE('',#111352,#13604) ;
#9489=LINE('',#111371,#13605) ;
#9490=LINE('',#111375,#13606) ;
#9491=LINE('',#111377,#13607) ;
#9492=LINE('',#111386,#13608) ;
#9493=LINE('',#111389,#13609) ;
#9494=LINE('',#111393,#13610) ;
#9495=LINE('',#111395,#13611) ;
#9496=LINE('',#111437,#13612) ;
#9497=LINE('',#111438,#13613) ;
#9498=LINE('',#111442,#13614) ;
#9499=LINE('',#111444,#13615) ;
#9500=LINE('',#111446,#13616) ;
#9501=LINE('',#111447,#13617) ;
#9502=LINE('',#111451,#13618) ;
#9503=LINE('',#111474,#13619) ;
#9504=LINE('',#111476,#13620) ;
#9505=LINE('',#111477,#13621) ;
#9506=LINE('',#111481,#13622) ;
#9507=LINE('',#111483,#13623) ;
#9508=LINE('',#111485,#13624) ;
#9509=LINE('',#111486,#13625) ;
#9510=LINE('',#111490,#13626) ;
#9511=LINE('',#111492,#13627) ;
#9512=LINE('',#111494,#13628) ;
#9513=LINE('',#111495,#13629) ;
#9514=LINE('',#111499,#13630) ;
#9515=LINE('',#111501,#13631) ;
#9516=LINE('',#111503,#13632) ;
#9517=LINE('',#111505,#13633) ;
#9518=LINE('',#111508,#13634) ;
#9519=LINE('',#111512,#13635) ;
#9520=LINE('',#111519,#13636) ;
#9521=LINE('',#111523,#13637) ;
#9522=LINE('',#111527,#13638) ;
#9523=LINE('',#111531,#13639) ;
#9524=LINE('',#111535,#13640) ;
#9525=LINE('',#111539,#13641) ;
#9526=LINE('',#111544,#13642) ;
#9527=LINE('',#111549,#13643) ;
#9528=LINE('',#111551,#13644) ;
#9529=LINE('',#111555,#13645) ;
#9530=LINE('',#111559,#13646) ;
#9531=LINE('',#111564,#13647) ;
#9532=LINE('',#111568,#13648) ;
#9533=LINE('',#111572,#13649) ;
#9534=LINE('',#111576,#13650) ;
#9535=LINE('',#111580,#13651) ;
#9536=LINE('',#111582,#13652) ;
#9537=LINE('',#111587,#13653) ;
#9538=LINE('',#111592,#13654) ;
#9539=LINE('',#111596,#13655) ;
#9540=LINE('',#111600,#13656) ;
#9541=LINE('',#111604,#13657) ;
#9542=LINE('',#111608,#13658) ;
#9543=LINE('',#111612,#13659) ;
#9544=LINE('',#111616,#13660) ;
#9545=LINE('',#111620,#13661) ;
#9546=LINE('',#111623,#13662) ;
#9547=LINE('',#111624,#13663) ;
#9548=LINE('',#111626,#13664) ;
#9549=LINE('',#111627,#13665) ;
#9550=LINE('',#111671,#13666) ;
#9551=LINE('',#111672,#13667) ;
#9552=LINE('',#111674,#13668) ;
#9553=LINE('',#111716,#13669) ;
#9554=LINE('',#111729,#13670) ;
#9555=LINE('',#111731,#13671) ;
#9556=LINE('',#111732,#13672) ;
#9557=LINE('',#111736,#13673) ;
#9558=LINE('',#111737,#13674) ;
#9559=LINE('',#111738,#13675) ;
#9560=LINE('',#111756,#13676) ;
#9561=LINE('',#111757,#13677) ;
#9562=LINE('',#111758,#13678) ;
#9563=LINE('',#111761,#13679) ;
#9564=LINE('',#111798,#13680) ;
#9565=LINE('',#111852,#13681) ;
#9566=LINE('',#111854,#13682) ;
#9567=LINE('',#111856,#13683) ;
#9568=LINE('',#111860,#13684) ;
#9569=LINE('',#111864,#13685) ;
#9570=LINE('',#111865,#13686) ;
#9571=LINE('',#111870,#13687) ;
#9572=LINE('',#111872,#13688) ;
#9573=LINE('',#111880,#13689) ;
#9574=LINE('',#111882,#13690) ;
#9575=LINE('',#111884,#13691) ;
#9576=LINE('',#111891,#13692) ;
#9577=LINE('',#111893,#13693) ;
#9578=LINE('',#111901,#13694) ;
#9579=LINE('',#111905,#13695) ;
#9580=LINE('',#111914,#13696) ;
#9581=LINE('',#111915,#13697) ;
#9582=LINE('',#111916,#13698) ;
#9583=LINE('',#111918,#13699) ;
#9584=LINE('',#111920,#13700) ;
#9585=LINE('',#111923,#13701) ;
#9586=LINE('',#111928,#13702) ;
#9587=LINE('',#111929,#13703) ;
#9588=LINE('',#111931,#13704) ;
#9589=LINE('',#111934,#13705) ;
#9590=LINE('',#111938,#13706) ;
#9591=LINE('',#111940,#13707) ;
#9592=LINE('',#111947,#13708) ;
#9593=LINE('',#111948,#13709) ;
#9594=LINE('',#111952,#13710) ;
#9595=LINE('',#111954,#13711) ;
#9596=LINE('',#111956,#13712) ;
#9597=LINE('',#111958,#13713) ;
#9598=LINE('',#111960,#13714) ;
#9599=LINE('',#111962,#13715) ;
#9600=LINE('',#111964,#13716) ;
#9601=LINE('',#111965,#13717) ;
#9602=LINE('',#111969,#13718) ;
#9603=LINE('',#111971,#13719) ;
#9604=LINE('',#111973,#13720) ;
#9605=LINE('',#111974,#13721) ;
#9606=LINE('',#111978,#13722) ;
#9607=LINE('',#111980,#13723) ;
#9608=LINE('',#111982,#13724) ;
#9609=LINE('',#111983,#13725) ;
#9610=LINE('',#111987,#13726) ;
#9611=LINE('',#111989,#13727) ;
#9612=LINE('',#111991,#13728) ;
#9613=LINE('',#111992,#13729) ;
#9614=LINE('',#112005,#13730) ;
#9615=LINE('',#112007,#13731) ;
#9616=LINE('',#112009,#13732) ;
#9617=LINE('',#112019,#13733) ;
#9618=LINE('',#112023,#13734) ;
#9619=LINE('',#112025,#13735) ;
#9620=LINE('',#112027,#13736) ;
#9621=LINE('',#112029,#13737) ;
#9622=LINE('',#112031,#13738) ;
#9623=LINE('',#112033,#13739) ;
#9624=LINE('',#112035,#13740) ;
#9625=LINE('',#112036,#13741) ;
#9626=LINE('',#112040,#13742) ;
#9627=LINE('',#112044,#13743) ;
#9628=LINE('',#112048,#13744) ;
#9629=LINE('',#112052,#13745) ;
#9630=LINE('',#112058,#13746) ;
#9631=LINE('',#112060,#13747) ;
#9632=LINE('',#112064,#13748) ;
#9633=LINE('',#112068,#13749) ;
#9634=LINE('',#112070,#13750) ;
#9635=LINE('',#112071,#13751) ;
#9636=LINE('',#112075,#13752) ;
#9637=LINE('',#112076,#13753) ;
#9638=LINE('',#112077,#13754) ;
#9639=LINE('',#112083,#13755) ;
#9640=LINE('',#112086,#13756) ;
#9641=LINE('',#112092,#13757) ;
#9642=LINE('',#112095,#13758) ;
#9643=LINE('',#112098,#13759) ;
#9644=LINE('',#112100,#13760) ;
#9645=LINE('',#112101,#13761) ;
#9646=LINE('',#112105,#13762) ;
#9647=LINE('',#112106,#13763) ;
#9648=LINE('',#112107,#13764) ;
#9649=LINE('',#112112,#13765) ;
#9650=LINE('',#112114,#13766) ;
#9651=LINE('',#112119,#13767) ;
#9652=LINE('',#112124,#13768) ;
#9653=LINE('',#112126,#13769) ;
#9654=LINE('',#112127,#13770) ;
#9655=LINE('',#112131,#13771) ;
#9656=LINE('',#112132,#13772) ;
#9657=LINE('',#112133,#13773) ;
#9658=LINE('',#112139,#13774) ;
#9659=LINE('',#112142,#13775) ;
#9660=LINE('',#112146,#13776) ;
#9661=LINE('',#112148,#13777) ;
#9662=LINE('',#112150,#13778) ;
#9663=LINE('',#112151,#13779) ;
#9664=LINE('',#112157,#13780) ;
#9665=LINE('',#112160,#13781) ;
#9666=LINE('',#112163,#13782) ;
#9667=LINE('',#112165,#13783) ;
#9668=LINE('',#112166,#13784) ;
#9669=LINE('',#112170,#13785) ;
#9670=LINE('',#112172,#13786) ;
#9671=LINE('',#112174,#13787) ;
#9672=LINE('',#112175,#13788) ;
#9673=LINE('',#112179,#13789) ;
#9674=LINE('',#112180,#13790) ;
#9675=LINE('',#112182,#13791) ;
#9676=LINE('',#112187,#13792) ;
#9677=LINE('',#112189,#13793) ;
#9678=LINE('',#112191,#13794) ;
#9679=LINE('',#112192,#13795) ;
#9680=LINE('',#112197,#13796) ;
#9681=LINE('',#112199,#13797) ;
#9682=LINE('',#112203,#13798) ;
#9683=LINE('',#112206,#13799) ;
#9684=LINE('',#112210,#13800) ;
#9685=LINE('',#112211,#13801) ;
#9686=LINE('',#112213,#13802) ;
#9687=LINE('',#112214,#13803) ;
#9688=LINE('',#112218,#13804) ;
#9689=LINE('',#112220,#13805) ;
#9690=LINE('',#112222,#13806) ;
#9691=LINE('',#112223,#13807) ;
#9692=LINE('',#112227,#13808) ;
#9693=LINE('',#112229,#13809) ;
#9694=LINE('',#112231,#13810) ;
#9695=LINE('',#112232,#13811) ;
#9696=LINE('',#112236,#13812) ;
#9697=LINE('',#112238,#13813) ;
#9698=LINE('',#112240,#13814) ;
#9699=LINE('',#112241,#13815) ;
#9700=LINE('',#112244,#13816) ;
#9701=LINE('',#112246,#13817) ;
#9702=LINE('',#112247,#13818) ;
#9703=LINE('',#112250,#13819) ;
#9704=LINE('',#112252,#13820) ;
#9705=LINE('',#112253,#13821) ;
#9706=LINE('',#112256,#13822) ;
#9707=LINE('',#112258,#13823) ;
#9708=LINE('',#112259,#13824) ;
#9709=LINE('',#112262,#13825) ;
#9710=LINE('',#112264,#13826) ;
#9711=LINE('',#112265,#13827) ;
#9712=LINE('',#112269,#13828) ;
#9713=LINE('',#112271,#13829) ;
#9714=LINE('',#112273,#13830) ;
#9715=LINE('',#112277,#13831) ;
#9716=LINE('',#112282,#13832) ;
#9717=LINE('',#112284,#13833) ;
#9718=LINE('',#112286,#13834) ;
#9719=LINE('',#112290,#13835) ;
#9720=LINE('',#112295,#13836) ;
#9721=LINE('',#112300,#13837) ;
#9722=LINE('',#112302,#13838) ;
#9723=LINE('',#112303,#13839) ;
#9724=LINE('',#112307,#13840) ;
#9725=LINE('',#112309,#13841) ;
#9726=LINE('',#112311,#13842) ;
#9727=LINE('',#112312,#13843) ;
#9728=LINE('',#112316,#13844) ;
#9729=LINE('',#112318,#13845) ;
#9730=LINE('',#112320,#13846) ;
#9731=LINE('',#112321,#13847) ;
#9732=LINE('',#112325,#13848) ;
#9733=LINE('',#112327,#13849) ;
#9734=LINE('',#112329,#13850) ;
#9735=LINE('',#112330,#13851) ;
#9736=LINE('',#112334,#13852) ;
#9737=LINE('',#112336,#13853) ;
#9738=LINE('',#112338,#13854) ;
#9739=LINE('',#112339,#13855) ;
#9740=LINE('',#112346,#13856) ;
#9741=LINE('',#112348,#13857) ;
#9742=LINE('',#112350,#13858) ;
#9743=LINE('',#112351,#13859) ;
#9744=LINE('',#112355,#13860) ;
#9745=LINE('',#112357,#13861) ;
#9746=LINE('',#112359,#13862) ;
#9747=LINE('',#112360,#13863) ;
#9748=LINE('',#112364,#13864) ;
#9749=LINE('',#112366,#13865) ;
#9750=LINE('',#112368,#13866) ;
#9751=LINE('',#112369,#13867) ;
#9752=LINE('',#112373,#13868) ;
#9753=LINE('',#112375,#13869) ;
#9754=LINE('',#112377,#13870) ;
#9755=LINE('',#112378,#13871) ;
#9756=LINE('',#112381,#13872) ;
#9757=LINE('',#112384,#13873) ;
#9758=LINE('',#112393,#13874) ;
#9759=LINE('',#112396,#13875) ;
#9760=LINE('',#112577,#13876) ;
#9761=LINE('',#112622,#13877) ;
#9762=LINE('',#112630,#13878) ;
#9763=LINE('',#112651,#13879) ;
#9764=LINE('',#112657,#13880) ;
#9765=LINE('',#112670,#13881) ;
#12467=VECTOR('',#79373,1000.) ;
#12468=VECTOR('',#79378,1000.) ;
#12469=VECTOR('',#79383,1000.) ;
#12470=VECTOR('',#79386,1000.) ;
#12471=VECTOR('',#79399,1.5) ;
#12472=VECTOR('',#79402,1000.) ;
#12473=VECTOR('',#79409,1000.) ;
#12474=VECTOR('',#79412,1000.) ;
#12475=VECTOR('',#79413,1000.) ;
#12476=VECTOR('',#79414,1000.) ;
#12477=VECTOR('',#79417,1000.) ;
#12478=VECTOR('',#79420,1000.) ;
#12479=VECTOR('',#79421,1000.) ;
#12480=VECTOR('',#79422,999.999999999999) ;
#12481=VECTOR('',#79423,1000.) ;
#12482=VECTOR('',#79426,1000.) ;
#12483=VECTOR('',#79427,1000.) ;
#12484=VECTOR('',#79428,1000.) ;
#12485=VECTOR('',#79429,1000.) ;
#12486=VECTOR('',#79432,1000.) ;
#12487=VECTOR('',#79433,1000.) ;
#12488=VECTOR('',#79434,1000.) ;
#12489=VECTOR('',#79435,1000.) ;
#12490=VECTOR('',#79438,1000.) ;
#12491=VECTOR('',#79439,1000.) ;
#12492=VECTOR('',#79440,1000.) ;
#12493=VECTOR('',#79441,1000.) ;
#12494=VECTOR('',#79444,1000.) ;
#12495=VECTOR('',#79445,1000.) ;
#12496=VECTOR('',#79446,1000.) ;
#12497=VECTOR('',#79447,1000.) ;
#12498=VECTOR('',#79450,1000.) ;
#12499=VECTOR('',#79451,1000.) ;
#12500=VECTOR('',#79452,1000.) ;
#12501=VECTOR('',#79453,1000.) ;
#12502=VECTOR('',#79456,1000.) ;
#12503=VECTOR('',#79459,1000.) ;
#12504=VECTOR('',#79468,1000.) ;
#12505=VECTOR('',#79471,1000.) ;
#12506=VECTOR('',#79474,1000.) ;
#12507=VECTOR('',#79477,1000.) ;
#12508=VECTOR('',#79480,1000.) ;
#12509=VECTOR('',#79483,1000.) ;
#12510=VECTOR('',#79488,1000.) ;
#12511=VECTOR('',#79493,1000.) ;
#12512=VECTOR('',#79494,1000.) ;
#12513=VECTOR('',#79497,1000.) ;
#12514=VECTOR('',#79500,1000.) ;
#12515=VECTOR('',#79505,1000.) ;
#12516=VECTOR('',#79508,1000.) ;
#12517=VECTOR('',#79511,1000.) ;
#12518=VECTOR('',#79514,1000.) ;
#12519=VECTOR('',#79517,1000.) ;
#12520=VECTOR('',#79518,1000.) ;
#12521=VECTOR('',#79523,1000.) ;
#12522=VECTOR('',#79528,1000.) ;
#12523=VECTOR('',#79531,1000.) ;
#12524=VECTOR('',#79534,1000.) ;
#12525=VECTOR('',#79537,1000.) ;
#12526=VECTOR('',#79540,1000.) ;
#12527=VECTOR('',#79543,1000.) ;
#12528=VECTOR('',#79546,1000.) ;
#12529=VECTOR('',#79549,1000.) ;
#12530=VECTOR('',#79554,1000.) ;
#12531=VECTOR('',#79555,1000.) ;
#12532=VECTOR('',#79558,1000.) ;
#12533=VECTOR('',#79559,1000.) ;
#12534=VECTOR('',#79562,1000.) ;
#12535=VECTOR('',#79563,1000.) ;
#12536=VECTOR('',#79564,1000.) ;
#12537=VECTOR('',#79565,1000.) ;
#12538=VECTOR('',#79570,1000.) ;
#12539=VECTOR('',#79571,1000.) ;
#12540=VECTOR('',#79572,999.999999999999) ;
#12541=VECTOR('',#79575,1000.) ;
#12542=VECTOR('',#79576,1000.) ;
#12543=VECTOR('',#79577,1000.) ;
#12544=VECTOR('',#79580,1000.) ;
#12545=VECTOR('',#79581,1000.) ;
#12546=VECTOR('',#79582,1000.) ;
#12547=VECTOR('',#79585,1000.) ;
#12548=VECTOR('',#79586,1000.) ;
#12549=VECTOR('',#79587,1000.) ;
#12550=VECTOR('',#79588,1000.) ;
#12551=VECTOR('',#79589,1000.) ;
#12552=VECTOR('',#79592,1000.) ;
#12553=VECTOR('',#79595,1000.) ;
#12554=VECTOR('',#79596,1000.) ;
#12555=VECTOR('',#79601,1000.) ;
#12556=VECTOR('',#79602,1000.) ;
#12557=VECTOR('',#79609,1000.) ;
#12558=VECTOR('',#79610,1000.) ;
#12559=VECTOR('',#79611,1000.) ;
#12560=VECTOR('',#79618,1000.) ;
#12561=VECTOR('',#79619,1000.) ;
#12562=VECTOR('',#79626,1000.) ;
#12563=VECTOR('',#79629,1000.) ;
#12564=VECTOR('',#79638,1000.) ;
#12565=VECTOR('',#79639,1000.) ;
#12566=VECTOR('',#79640,1000.) ;
#12567=VECTOR('',#79641,1000.) ;
#12568=VECTOR('',#79642,1000.) ;
#12569=VECTOR('',#79645,1000.) ;
#12570=VECTOR('',#79650,1000.) ;
#12571=VECTOR('',#79651,1000.) ;
#12572=VECTOR('',#79652,1000.) ;
#12573=VECTOR('',#79655,1000.) ;
#12574=VECTOR('',#79658,1000.) ;
#12575=VECTOR('',#79659,1000.) ;
#12576=VECTOR('',#79666,1000.) ;
#12577=VECTOR('',#79667,1000.) ;
#12578=VECTOR('',#79670,1000.) ;
#12579=VECTOR('',#79671,1000.) ;
#12580=VECTOR('',#79672,1000.) ;
#12581=VECTOR('',#79673,1000.) ;
#12582=VECTOR('',#79674,1000.) ;
#12583=VECTOR('',#79675,1000.) ;
#12584=VECTOR('',#79676,1000.) ;
#12585=VECTOR('',#79677,1000.) ;
#12586=VECTOR('',#79680,1000.) ;
#12587=VECTOR('',#79681,1000.) ;
#12588=VECTOR('',#79682,1000.) ;
#12589=VECTOR('',#79683,1000.) ;
#12590=VECTOR('',#79686,1000.) ;
#12591=VECTOR('',#79687,1000.) ;
#12592=VECTOR('',#79688,1000.) ;
#12593=VECTOR('',#79689,1000.) ;
#12594=VECTOR('',#79692,1000.) ;
#12595=VECTOR('',#79693,1000.) ;
#12596=VECTOR('',#79694,1000.) ;
#12597=VECTOR('',#79695,1000.) ;
#12598=VECTOR('',#79698,1000.) ;
#12599=VECTOR('',#79699,1000.) ;
#12600=VECTOR('',#79700,1000.) ;
#12601=VECTOR('',#79701,1000.) ;
#12602=VECTOR('',#79704,1000.) ;
#12603=VECTOR('',#79705,1000.) ;
#12604=VECTOR('',#79706,1000.) ;
#12605=VECTOR('',#79707,1000.) ;
#12606=VECTOR('',#79708,1000.) ;
#12607=VECTOR('',#79709,1000.) ;
#12608=VECTOR('',#79710,1000.) ;
#12609=VECTOR('',#79711,1000.) ;
#12610=VECTOR('',#79714,1000.) ;
#12611=VECTOR('',#79717,1000.) ;
#12612=VECTOR('',#79720,1000.) ;
#12613=VECTOR('',#79723,1000.) ;
#12614=VECTOR('',#79730,1000.) ;
#12615=VECTOR('',#79731,1000.) ;
#12616=VECTOR('',#79734,1000.) ;
#12617=VECTOR('',#79739,1000.) ;
#12618=VECTOR('',#79740,1000.) ;
#12619=VECTOR('',#79741,1000.) ;
#12620=VECTOR('',#79744,1000.) ;
#12621=VECTOR('',#79745,1000.) ;
#12622=VECTOR('',#79746,1000.) ;
#12623=VECTOR('',#79751,1000.) ;
#12624=VECTOR('',#79754,1000.) ;
#12625=VECTOR('',#79759,1000.) ;
#12626=VECTOR('',#79762,1000.) ;
#12627=VECTOR('',#79765,1000.) ;
#12628=VECTOR('',#79766,1000.) ;
#12629=VECTOR('',#79767,1000.) ;
#12630=VECTOR('',#79770,1000.) ;
#12631=VECTOR('',#79771,1000.) ;
#12632=VECTOR('',#79772,1000.) ;
#12633=VECTOR('',#79777,1000.) ;
#12634=VECTOR('',#79778,1000.) ;
#12635=VECTOR('',#79783,1000.) ;
#12636=VECTOR('',#79788,1000.) ;
#12637=VECTOR('',#79789,1000.) ;
#12638=VECTOR('',#79790,1000.) ;
#12639=VECTOR('',#79793,1000.) ;
#12640=VECTOR('',#79794,1000.) ;
#12641=VECTOR('',#79795,1000.) ;
#12642=VECTOR('',#79800,1000.) ;
#12643=VECTOR('',#79803,1000.) ;
#12644=VECTOR('',#79806,1000.) ;
#12645=VECTOR('',#79807,1000.) ;
#12646=VECTOR('',#79808,1000.) ;
#12647=VECTOR('',#79809,1000.) ;
#12648=VECTOR('',#79814,1000.) ;
#12649=VECTOR('',#79817,1000.) ;
#12650=VECTOR('',#79820,1000.) ;
#12651=VECTOR('',#79821,1000.) ;
#12652=VECTOR('',#79822,1000.) ;
#12653=VECTOR('',#79825,1000.) ;
#12654=VECTOR('',#79826,1000.) ;
#12655=VECTOR('',#79827,1000.) ;
#12656=VECTOR('',#79828,1000.) ;
#12657=VECTOR('',#79831,1000.) ;
#12658=VECTOR('',#79832,1000.) ;
#12659=VECTOR('',#79833,1000.) ;
#12660=VECTOR('',#79838,1000.) ;
#12661=VECTOR('',#79839,1000.) ;
#12662=VECTOR('',#79840,1000.) ;
#12663=VECTOR('',#79841,1000.) ;
#12664=VECTOR('',#79846,1000.) ;
#12665=VECTOR('',#79847,1000.) ;
#12666=VECTOR('',#79850,1000.) ;
#12667=VECTOR('',#79853,1000.) ;
#12668=VECTOR('',#79856,1000.) ;
#12669=VECTOR('',#79857,1000.) ;
#12670=VECTOR('',#79858,1000.) ;
#12671=VECTOR('',#79859,1000.) ;
#12672=VECTOR('',#79862,1000.) ;
#12673=VECTOR('',#79863,1000.) ;
#12674=VECTOR('',#79864,1000.) ;
#12675=VECTOR('',#79865,1000.) ;
#12676=VECTOR('',#79868,1000.) ;
#12677=VECTOR('',#79869,1000.) ;
#12678=VECTOR('',#79870,1000.) ;
#12679=VECTOR('',#79871,1000.) ;
#12680=VECTOR('',#79874,1000.) ;
#12681=VECTOR('',#79875,1000.) ;
#12682=VECTOR('',#79876,1000.) ;
#12683=VECTOR('',#79877,1000.) ;
#12684=VECTOR('',#79880,1000.) ;
#12685=VECTOR('',#79881,1000.) ;
#12686=VECTOR('',#79882,1000.) ;
#12687=VECTOR('',#79885,1000.) ;
#12688=VECTOR('',#79886,1000.) ;
#12689=VECTOR('',#79887,1000.) ;
#12690=VECTOR('',#79890,1000.) ;
#12691=VECTOR('',#79891,1000.) ;
#12692=VECTOR('',#79892,1000.) ;
#12693=VECTOR('',#79895,1000.) ;
#12694=VECTOR('',#79896,1000.) ;
#12695=VECTOR('',#79897,1000.) ;
#12696=VECTOR('',#79900,1000.) ;
#12697=VECTOR('',#79901,1000.) ;
#12698=VECTOR('',#79902,1000.) ;
#12699=VECTOR('',#79905,1000.) ;
#12700=VECTOR('',#79910,1000.) ;
#12701=VECTOR('',#79911,1000.) ;
#12702=VECTOR('',#79912,1000.) ;
#12703=VECTOR('',#79915,1000.) ;
#12704=VECTOR('',#79920,1000.) ;
#12705=VECTOR('',#79927,1000.) ;
#12706=VECTOR('',#79928,1000.) ;
#12707=VECTOR('',#79929,1000.) ;
#12708=VECTOR('',#79932,1000.) ;
#12709=VECTOR('',#79933,1000.) ;
#12710=VECTOR('',#79934,1000.) ;
#12711=VECTOR('',#79935,1000.) ;
#12712=VECTOR('',#79938,1000.) ;
#12713=VECTOR('',#79939,1000.) ;
#12714=VECTOR('',#79940,1000.) ;
#12715=VECTOR('',#79941,1000.) ;
#12716=VECTOR('',#79944,1000.) ;
#12717=VECTOR('',#79945,1000.) ;
#12718=VECTOR('',#79946,1000.) ;
#12719=VECTOR('',#79947,1000.) ;
#12720=VECTOR('',#79950,1000.) ;
#12721=VECTOR('',#79951,1000.) ;
#12722=VECTOR('',#79952,1000.) ;
#12723=VECTOR('',#79953,1000.) ;
#12724=VECTOR('',#79962,1000.) ;
#12725=VECTOR('',#79963,1000.) ;
#12726=VECTOR('',#79964,1000.) ;
#12727=VECTOR('',#79965,1000.) ;
#12728=VECTOR('',#79968,1000.) ;
#12729=VECTOR('',#79969,1000.) ;
#12730=VECTOR('',#79970,1000.) ;
#12731=VECTOR('',#79971,1000.) ;
#12732=VECTOR('',#79974,1000.) ;
#12733=VECTOR('',#79975,1000.) ;
#12734=VECTOR('',#79976,1000.) ;
#12735=VECTOR('',#79977,1000.) ;
#12736=VECTOR('',#79980,1000.) ;
#12737=VECTOR('',#79981,1000.) ;
#12738=VECTOR('',#79982,1000.) ;
#12739=VECTOR('',#79983,1000.) ;
#12740=VECTOR('',#79986,1000.) ;
#12741=VECTOR('',#79989,1000.) ;
#12742=VECTOR('',#80000,1000.) ;
#12743=VECTOR('',#80003,1000.) ;
#12744=VECTOR('',#80182,1000.) ;
#12745=VECTOR('',#80207,1000.) ;
#12746=VECTOR('',#80220,1000.) ;
#12747=VECTOR('',#80255,1000.) ;
#12748=VECTOR('',#80266,1000.) ;
#12749=VECTOR('',#80289,1000.) ;
#12750=VECTOR('',#80876,1000.) ;
#12751=VECTOR('',#80881,1000.) ;
#12752=VECTOR('',#80886,1000.) ;
#12753=VECTOR('',#80889,1000.) ;
#12754=VECTOR('',#80902,1.5) ;
#12755=VECTOR('',#80905,1000.) ;
#12756=VECTOR('',#80912,1000.) ;
#12757=VECTOR('',#80915,1000.) ;
#12758=VECTOR('',#80916,1000.) ;
#12759=VECTOR('',#80917,1000.) ;
#12760=VECTOR('',#80920,1000.) ;
#12761=VECTOR('',#80923,1000.) ;
#12762=VECTOR('',#80924,1000.) ;
#12763=VECTOR('',#80925,1000.) ;
#12764=VECTOR('',#80926,1000.) ;
#12765=VECTOR('',#80929,1000.) ;
#12766=VECTOR('',#80930,1000.) ;
#12767=VECTOR('',#80931,1000.) ;
#12768=VECTOR('',#80932,1000.) ;
#12769=VECTOR('',#80935,1000.) ;
#12770=VECTOR('',#80936,1000.) ;
#12771=VECTOR('',#80937,1000.) ;
#12772=VECTOR('',#80938,1000.) ;
#12773=VECTOR('',#80941,1000.) ;
#12774=VECTOR('',#80942,1000.) ;
#12775=VECTOR('',#80943,1000.) ;
#12776=VECTOR('',#80944,1000.) ;
#12777=VECTOR('',#80947,1000.) ;
#12778=VECTOR('',#80948,1000.) ;
#12779=VECTOR('',#80949,1000.) ;
#12780=VECTOR('',#80950,1000.) ;
#12781=VECTOR('',#80953,1000.) ;
#12782=VECTOR('',#80954,1000.) ;
#12783=VECTOR('',#80955,1000.) ;
#12784=VECTOR('',#80956,1000.) ;
#12785=VECTOR('',#80959,1000.) ;
#12786=VECTOR('',#80962,1000.) ;
#12787=VECTOR('',#80971,1000.) ;
#12788=VECTOR('',#80974,1000.) ;
#12789=VECTOR('',#80977,1000.) ;
#12790=VECTOR('',#80980,1000.) ;
#12791=VECTOR('',#80983,1000.) ;
#12792=VECTOR('',#80986,1000.) ;
#12793=VECTOR('',#80991,1000.) ;
#12794=VECTOR('',#80996,1000.) ;
#12795=VECTOR('',#80997,1000.) ;
#12796=VECTOR('',#81000,1000.) ;
#12797=VECTOR('',#81003,1000.) ;
#12798=VECTOR('',#81008,1000.) ;
#12799=VECTOR('',#81011,1000.) ;
#12800=VECTOR('',#81014,1000.) ;
#12801=VECTOR('',#81017,1000.) ;
#12802=VECTOR('',#81020,1000.) ;
#12803=VECTOR('',#81021,1000.) ;
#12804=VECTOR('',#81026,1000.) ;
#12805=VECTOR('',#81031,1000.) ;
#12806=VECTOR('',#81034,1000.) ;
#12807=VECTOR('',#81037,1000.) ;
#12808=VECTOR('',#81040,1000.) ;
#12809=VECTOR('',#81043,1000.) ;
#12810=VECTOR('',#81046,1000.) ;
#12811=VECTOR('',#81049,1000.) ;
#12812=VECTOR('',#81052,1000.) ;
#12813=VECTOR('',#81057,1000.) ;
#12814=VECTOR('',#81058,1000.) ;
#12815=VECTOR('',#81061,1000.) ;
#12816=VECTOR('',#81062,1000.) ;
#12817=VECTOR('',#81065,1000.) ;
#12818=VECTOR('',#81066,1000.) ;
#12819=VECTOR('',#81067,1000.) ;
#12820=VECTOR('',#81068,1000.) ;
#12821=VECTOR('',#81073,1000.) ;
#12822=VECTOR('',#81074,1000.) ;
#12823=VECTOR('',#81075,1000.) ;
#12824=VECTOR('',#81078,1000.) ;
#12825=VECTOR('',#81079,1000.) ;
#12826=VECTOR('',#81080,1000.) ;
#12827=VECTOR('',#81083,1000.) ;
#12828=VECTOR('',#81084,1000.) ;
#12829=VECTOR('',#81085,1000.) ;
#12830=VECTOR('',#81088,1000.) ;
#12831=VECTOR('',#81089,1000.) ;
#12832=VECTOR('',#81090,1000.) ;
#12833=VECTOR('',#81091,1000.) ;
#12834=VECTOR('',#81092,1000.) ;
#12835=VECTOR('',#81095,1000.) ;
#12836=VECTOR('',#81098,1000.) ;
#12837=VECTOR('',#81099,1000.) ;
#12838=VECTOR('',#81104,1000.) ;
#12839=VECTOR('',#81105,1000.) ;
#12840=VECTOR('',#81112,1000.) ;
#12841=VECTOR('',#81113,1000.) ;
#12842=VECTOR('',#81114,1000.) ;
#12843=VECTOR('',#81121,1000.) ;
#12844=VECTOR('',#81122,1000.) ;
#12845=VECTOR('',#81129,1000.) ;
#12846=VECTOR('',#81132,1000.) ;
#12847=VECTOR('',#81141,1000.) ;
#12848=VECTOR('',#81142,1000.) ;
#12849=VECTOR('',#81143,1000.) ;
#12850=VECTOR('',#81144,1000.) ;
#12851=VECTOR('',#81145,1000.) ;
#12852=VECTOR('',#81148,1000.) ;
#12853=VECTOR('',#81153,1000.) ;
#12854=VECTOR('',#81154,1000.) ;
#12855=VECTOR('',#81155,1000.) ;
#12856=VECTOR('',#81158,1000.) ;
#12857=VECTOR('',#81161,1000.) ;
#12858=VECTOR('',#81162,1000.) ;
#12859=VECTOR('',#81169,1000.) ;
#12860=VECTOR('',#81170,1000.) ;
#12861=VECTOR('',#81173,1000.) ;
#12862=VECTOR('',#81174,1000.) ;
#12863=VECTOR('',#81175,1000.) ;
#12864=VECTOR('',#81176,1000.) ;
#12865=VECTOR('',#81177,1000.) ;
#12866=VECTOR('',#81178,1000.) ;
#12867=VECTOR('',#81179,1000.) ;
#12868=VECTOR('',#81180,1000.) ;
#12869=VECTOR('',#81183,1000.) ;
#12870=VECTOR('',#81184,1000.) ;
#12871=VECTOR('',#81185,1000.) ;
#12872=VECTOR('',#81186,1000.) ;
#12873=VECTOR('',#81189,1000.) ;
#12874=VECTOR('',#81190,1000.) ;
#12875=VECTOR('',#81191,1000.) ;
#12876=VECTOR('',#81192,1000.) ;
#12877=VECTOR('',#81195,1000.) ;
#12878=VECTOR('',#81196,1000.) ;
#12879=VECTOR('',#81197,1000.) ;
#12880=VECTOR('',#81198,1000.) ;
#12881=VECTOR('',#81201,1000.) ;
#12882=VECTOR('',#81202,1000.) ;
#12883=VECTOR('',#81203,1000.) ;
#12884=VECTOR('',#81204,1000.) ;
#12885=VECTOR('',#81207,1000.) ;
#12886=VECTOR('',#81208,1000.) ;
#12887=VECTOR('',#81209,1000.) ;
#12888=VECTOR('',#81210,1000.) ;
#12889=VECTOR('',#81211,1000.) ;
#12890=VECTOR('',#81212,1000.) ;
#12891=VECTOR('',#81213,1000.) ;
#12892=VECTOR('',#81214,1000.) ;
#12893=VECTOR('',#81217,1000.) ;
#12894=VECTOR('',#81220,1000.) ;
#12895=VECTOR('',#81223,1000.) ;
#12896=VECTOR('',#81226,1000.) ;
#12897=VECTOR('',#81233,1000.) ;
#12898=VECTOR('',#81234,1000.) ;
#12899=VECTOR('',#81237,1000.) ;
#12900=VECTOR('',#81242,1000.) ;
#12901=VECTOR('',#81243,1000.) ;
#12902=VECTOR('',#81244,1000.) ;
#12903=VECTOR('',#81247,1000.) ;
#12904=VECTOR('',#81248,1000.) ;
#12905=VECTOR('',#81249,1000.) ;
#12906=VECTOR('',#81254,1000.) ;
#12907=VECTOR('',#81257,1000.) ;
#12908=VECTOR('',#81262,1000.) ;
#12909=VECTOR('',#81265,1000.) ;
#12910=VECTOR('',#81268,1000.) ;
#12911=VECTOR('',#81269,1000.) ;
#12912=VECTOR('',#81270,1000.) ;
#12913=VECTOR('',#81273,1000.) ;
#12914=VECTOR('',#81274,1000.) ;
#12915=VECTOR('',#81275,1000.) ;
#12916=VECTOR('',#81280,1000.) ;
#12917=VECTOR('',#81281,1000.) ;
#12918=VECTOR('',#81286,1000.) ;
#12919=VECTOR('',#81291,1000.) ;
#12920=VECTOR('',#81292,1000.) ;
#12921=VECTOR('',#81293,1000.) ;
#12922=VECTOR('',#81296,1000.) ;
#12923=VECTOR('',#81297,1000.) ;
#12924=VECTOR('',#81298,1000.) ;
#12925=VECTOR('',#81303,1000.) ;
#12926=VECTOR('',#81306,1000.) ;
#12927=VECTOR('',#81309,1000.) ;
#12928=VECTOR('',#81310,1000.) ;
#12929=VECTOR('',#81311,1000.) ;
#12930=VECTOR('',#81312,1000.) ;
#12931=VECTOR('',#81317,1000.) ;
#12932=VECTOR('',#81320,1000.) ;
#12933=VECTOR('',#81323,1000.) ;
#12934=VECTOR('',#81324,1000.) ;
#12935=VECTOR('',#81325,1000.) ;
#12936=VECTOR('',#81328,1000.) ;
#12937=VECTOR('',#81329,1000.) ;
#12938=VECTOR('',#81330,1000.) ;
#12939=VECTOR('',#81331,1000.) ;
#12940=VECTOR('',#81334,1000.) ;
#12941=VECTOR('',#81335,1000.) ;
#12942=VECTOR('',#81336,1000.) ;
#12943=VECTOR('',#81341,1000.) ;
#12944=VECTOR('',#81342,1000.) ;
#12945=VECTOR('',#81343,1000.) ;
#12946=VECTOR('',#81344,1000.) ;
#12947=VECTOR('',#81349,1000.) ;
#12948=VECTOR('',#81350,1000.) ;
#12949=VECTOR('',#81353,1000.) ;
#12950=VECTOR('',#81356,1000.) ;
#12951=VECTOR('',#81359,1000.) ;
#12952=VECTOR('',#81360,1000.) ;
#12953=VECTOR('',#81361,1000.) ;
#12954=VECTOR('',#81362,1000.) ;
#12955=VECTOR('',#81365,1000.) ;
#12956=VECTOR('',#81366,1000.) ;
#12957=VECTOR('',#81367,1000.) ;
#12958=VECTOR('',#81368,1000.) ;
#12959=VECTOR('',#81371,1000.) ;
#12960=VECTOR('',#81372,1000.) ;
#12961=VECTOR('',#81373,1000.) ;
#12962=VECTOR('',#81374,1000.) ;
#12963=VECTOR('',#81377,1000.) ;
#12964=VECTOR('',#81378,1000.) ;
#12965=VECTOR('',#81379,1000.) ;
#12966=VECTOR('',#81380,1000.) ;
#12967=VECTOR('',#81383,1000.) ;
#12968=VECTOR('',#81384,1000.) ;
#12969=VECTOR('',#81385,1000.) ;
#12970=VECTOR('',#81388,1000.) ;
#12971=VECTOR('',#81389,1000.) ;
#12972=VECTOR('',#81390,1000.) ;
#12973=VECTOR('',#81393,1000.) ;
#12974=VECTOR('',#81394,1000.) ;
#12975=VECTOR('',#81395,1000.) ;
#12976=VECTOR('',#81398,1000.) ;
#12977=VECTOR('',#81399,1000.) ;
#12978=VECTOR('',#81400,1000.) ;
#12979=VECTOR('',#81403,1000.) ;
#12980=VECTOR('',#81404,1000.) ;
#12981=VECTOR('',#81405,1000.) ;
#12982=VECTOR('',#81408,1000.) ;
#12983=VECTOR('',#81413,1000.) ;
#12984=VECTOR('',#81414,1000.) ;
#12985=VECTOR('',#81415,1000.) ;
#12986=VECTOR('',#81418,1000.) ;
#12987=VECTOR('',#81423,1000.) ;
#12988=VECTOR('',#81430,1000.) ;
#12989=VECTOR('',#81431,1000.) ;
#12990=VECTOR('',#81432,1000.) ;
#12991=VECTOR('',#81435,1000.) ;
#12992=VECTOR('',#81436,1000.) ;
#12993=VECTOR('',#81437,1000.) ;
#12994=VECTOR('',#81438,1000.) ;
#12995=VECTOR('',#81441,1000.) ;
#12996=VECTOR('',#81442,1000.) ;
#12997=VECTOR('',#81443,1000.) ;
#12998=VECTOR('',#81444,1000.) ;
#12999=VECTOR('',#81447,1000.) ;
#13000=VECTOR('',#81448,1000.) ;
#13001=VECTOR('',#81449,1000.) ;
#13002=VECTOR('',#81450,1000.) ;
#13003=VECTOR('',#81453,1000.) ;
#13004=VECTOR('',#81454,1000.) ;
#13005=VECTOR('',#81455,1000.) ;
#13006=VECTOR('',#81456,1000.) ;
#13007=VECTOR('',#81465,1000.) ;
#13008=VECTOR('',#81466,1000.) ;
#13009=VECTOR('',#81467,1000.) ;
#13010=VECTOR('',#81468,1000.) ;
#13011=VECTOR('',#81471,1000.) ;
#13012=VECTOR('',#81472,1000.) ;
#13013=VECTOR('',#81473,1000.) ;
#13014=VECTOR('',#81474,1000.) ;
#13015=VECTOR('',#81477,1000.) ;
#13016=VECTOR('',#81478,1000.) ;
#13017=VECTOR('',#81479,1000.) ;
#13018=VECTOR('',#81480,1000.) ;
#13019=VECTOR('',#81483,1000.) ;
#13020=VECTOR('',#81484,1000.) ;
#13021=VECTOR('',#81485,1000.) ;
#13022=VECTOR('',#81486,1000.) ;
#13023=VECTOR('',#81489,1000.) ;
#13024=VECTOR('',#81492,1000.) ;
#13025=VECTOR('',#81503,1000.) ;
#13026=VECTOR('',#81506,1000.) ;
#13027=VECTOR('',#81685,1000.) ;
#13028=VECTOR('',#81710,1000.) ;
#13029=VECTOR('',#81723,1000.) ;
#13030=VECTOR('',#81758,1000.) ;
#13031=VECTOR('',#81769,1000.) ;
#13032=VECTOR('',#81792,1000.) ;
#13033=VECTOR('',#82379,1000.) ;
#13034=VECTOR('',#82384,1000.) ;
#13035=VECTOR('',#82389,1000.) ;
#13036=VECTOR('',#82392,1000.) ;
#13037=VECTOR('',#82405,1.5) ;
#13038=VECTOR('',#82408,1000.) ;
#13039=VECTOR('',#82415,1000.) ;
#13040=VECTOR('',#82418,1000.) ;
#13041=VECTOR('',#82419,1000.) ;
#13042=VECTOR('',#82420,1000.) ;
#13043=VECTOR('',#82423,1000.) ;
#13044=VECTOR('',#82426,1000.) ;
#13045=VECTOR('',#82427,1000.) ;
#13046=VECTOR('',#82428,1000.) ;
#13047=VECTOR('',#82429,1000.) ;
#13048=VECTOR('',#82432,1000.) ;
#13049=VECTOR('',#82433,1000.) ;
#13050=VECTOR('',#82434,1000.) ;
#13051=VECTOR('',#82435,1000.) ;
#13052=VECTOR('',#82438,1000.) ;
#13053=VECTOR('',#82439,1000.) ;
#13054=VECTOR('',#82440,1000.) ;
#13055=VECTOR('',#82441,1000.) ;
#13056=VECTOR('',#82444,1000.) ;
#13057=VECTOR('',#82445,1000.) ;
#13058=VECTOR('',#82446,1000.) ;
#13059=VECTOR('',#82447,1000.) ;
#13060=VECTOR('',#82450,1000.) ;
#13061=VECTOR('',#82451,1000.) ;
#13062=VECTOR('',#82452,1000.) ;
#13063=VECTOR('',#82453,1000.) ;
#13064=VECTOR('',#82456,1000.) ;
#13065=VECTOR('',#82457,1000.) ;
#13066=VECTOR('',#82458,1000.) ;
#13067=VECTOR('',#82459,1000.) ;
#13068=VECTOR('',#82462,1000.) ;
#13069=VECTOR('',#82465,1000.) ;
#13070=VECTOR('',#82474,1000.) ;
#13071=VECTOR('',#82477,1000.) ;
#13072=VECTOR('',#82480,1000.) ;
#13073=VECTOR('',#82483,1000.) ;
#13074=VECTOR('',#82486,1000.) ;
#13075=VECTOR('',#82489,1000.) ;
#13076=VECTOR('',#82494,1000.) ;
#13077=VECTOR('',#82499,1000.) ;
#13078=VECTOR('',#82500,1000.) ;
#13079=VECTOR('',#82503,1000.) ;
#13080=VECTOR('',#82506,1000.) ;
#13081=VECTOR('',#82511,1000.) ;
#13082=VECTOR('',#82514,1000.) ;
#13083=VECTOR('',#82517,1000.) ;
#13084=VECTOR('',#82520,1000.) ;
#13085=VECTOR('',#82523,1000.) ;
#13086=VECTOR('',#82524,1000.) ;
#13087=VECTOR('',#82529,1000.) ;
#13088=VECTOR('',#82534,1000.) ;
#13089=VECTOR('',#82537,1000.) ;
#13090=VECTOR('',#82540,1000.) ;
#13091=VECTOR('',#82543,1000.) ;
#13092=VECTOR('',#82546,1000.) ;
#13093=VECTOR('',#82549,1000.) ;
#13094=VECTOR('',#82552,1000.) ;
#13095=VECTOR('',#82555,1000.) ;
#13096=VECTOR('',#82560,1000.) ;
#13097=VECTOR('',#82561,1000.) ;
#13098=VECTOR('',#82564,1000.) ;
#13099=VECTOR('',#82565,1000.) ;
#13100=VECTOR('',#82568,1000.) ;
#13101=VECTOR('',#82569,1000.) ;
#13102=VECTOR('',#82570,1000.) ;
#13103=VECTOR('',#82571,1000.) ;
#13104=VECTOR('',#82576,1000.) ;
#13105=VECTOR('',#82577,1000.) ;
#13106=VECTOR('',#82578,1000.) ;
#13107=VECTOR('',#82581,1000.) ;
#13108=VECTOR('',#82582,1000.) ;
#13109=VECTOR('',#82583,1000.) ;
#13110=VECTOR('',#82586,1000.) ;
#13111=VECTOR('',#82587,1000.) ;
#13112=VECTOR('',#82588,1000.) ;
#13113=VECTOR('',#82591,1000.) ;
#13114=VECTOR('',#82592,1000.) ;
#13115=VECTOR('',#82593,1000.) ;
#13116=VECTOR('',#82594,1000.) ;
#13117=VECTOR('',#82595,1000.) ;
#13118=VECTOR('',#82598,1000.) ;
#13119=VECTOR('',#82601,1000.) ;
#13120=VECTOR('',#82602,1000.) ;
#13121=VECTOR('',#82607,1000.) ;
#13122=VECTOR('',#82608,1000.) ;
#13123=VECTOR('',#82615,1000.) ;
#13124=VECTOR('',#82616,1000.) ;
#13125=VECTOR('',#82617,1000.) ;
#13126=VECTOR('',#82624,1000.) ;
#13127=VECTOR('',#82625,1000.) ;
#13128=VECTOR('',#82632,1000.) ;
#13129=VECTOR('',#82635,1000.) ;
#13130=VECTOR('',#82644,1000.) ;
#13131=VECTOR('',#82645,1000.) ;
#13132=VECTOR('',#82646,1000.) ;
#13133=VECTOR('',#82647,1000.) ;
#13134=VECTOR('',#82648,1000.) ;
#13135=VECTOR('',#82651,1000.) ;
#13136=VECTOR('',#82656,1000.) ;
#13137=VECTOR('',#82657,1000.) ;
#13138=VECTOR('',#82658,1000.) ;
#13139=VECTOR('',#82661,1000.) ;
#13140=VECTOR('',#82664,1000.) ;
#13141=VECTOR('',#82665,1000.) ;
#13142=VECTOR('',#82672,1000.) ;
#13143=VECTOR('',#82673,1000.) ;
#13144=VECTOR('',#82676,1000.) ;
#13145=VECTOR('',#82677,1000.) ;
#13146=VECTOR('',#82678,1000.) ;
#13147=VECTOR('',#82679,1000.) ;
#13148=VECTOR('',#82680,1000.) ;
#13149=VECTOR('',#82681,1000.) ;
#13150=VECTOR('',#82682,1000.) ;
#13151=VECTOR('',#82683,1000.) ;
#13152=VECTOR('',#82686,1000.) ;
#13153=VECTOR('',#82687,1000.) ;
#13154=VECTOR('',#82688,1000.) ;
#13155=VECTOR('',#82689,1000.) ;
#13156=VECTOR('',#82692,1000.) ;
#13157=VECTOR('',#82693,1000.) ;
#13158=VECTOR('',#82694,1000.) ;
#13159=VECTOR('',#82695,1000.) ;
#13160=VECTOR('',#82698,1000.) ;
#13161=VECTOR('',#82699,1000.) ;
#13162=VECTOR('',#82700,1000.) ;
#13163=VECTOR('',#82701,1000.) ;
#13164=VECTOR('',#82704,1000.) ;
#13165=VECTOR('',#82705,1000.) ;
#13166=VECTOR('',#82706,1000.) ;
#13167=VECTOR('',#82707,1000.) ;
#13168=VECTOR('',#82710,1000.) ;
#13169=VECTOR('',#82711,1000.) ;
#13170=VECTOR('',#82712,1000.) ;
#13171=VECTOR('',#82713,1000.) ;
#13172=VECTOR('',#82714,1000.) ;
#13173=VECTOR('',#82715,1000.) ;
#13174=VECTOR('',#82716,1000.) ;
#13175=VECTOR('',#82717,1000.) ;
#13176=VECTOR('',#82720,1000.) ;
#13177=VECTOR('',#82723,1000.) ;
#13178=VECTOR('',#82726,1000.) ;
#13179=VECTOR('',#82729,1000.) ;
#13180=VECTOR('',#82736,1000.) ;
#13181=VECTOR('',#82737,1000.) ;
#13182=VECTOR('',#82740,1000.) ;
#13183=VECTOR('',#82745,1000.) ;
#13184=VECTOR('',#82746,1000.) ;
#13185=VECTOR('',#82747,1000.) ;
#13186=VECTOR('',#82750,1000.) ;
#13187=VECTOR('',#82751,1000.) ;
#13188=VECTOR('',#82752,1000.) ;
#13189=VECTOR('',#82757,1000.) ;
#13190=VECTOR('',#82760,1000.) ;
#13191=VECTOR('',#82765,1000.) ;
#13192=VECTOR('',#82768,1000.) ;
#13193=VECTOR('',#82771,1000.) ;
#13194=VECTOR('',#82772,1000.) ;
#13195=VECTOR('',#82773,1000.) ;
#13196=VECTOR('',#82776,1000.) ;
#13197=VECTOR('',#82777,1000.) ;
#13198=VECTOR('',#82778,1000.) ;
#13199=VECTOR('',#82783,1000.) ;
#13200=VECTOR('',#82784,1000.) ;
#13201=VECTOR('',#82789,1000.) ;
#13202=VECTOR('',#82794,1000.) ;
#13203=VECTOR('',#82795,1000.) ;
#13204=VECTOR('',#82796,1000.) ;
#13205=VECTOR('',#82799,1000.) ;
#13206=VECTOR('',#82800,1000.) ;
#13207=VECTOR('',#82801,1000.) ;
#13208=VECTOR('',#82806,1000.) ;
#13209=VECTOR('',#82809,1000.) ;
#13210=VECTOR('',#82812,1000.) ;
#13211=VECTOR('',#82813,1000.) ;
#13212=VECTOR('',#82814,1000.) ;
#13213=VECTOR('',#82815,1000.) ;
#13214=VECTOR('',#82820,1000.) ;
#13215=VECTOR('',#82823,1000.) ;
#13216=VECTOR('',#82826,1000.) ;
#13217=VECTOR('',#82827,1000.) ;
#13218=VECTOR('',#82828,1000.) ;
#13219=VECTOR('',#82831,1000.) ;
#13220=VECTOR('',#82832,1000.) ;
#13221=VECTOR('',#82833,1000.) ;
#13222=VECTOR('',#82834,1000.) ;
#13223=VECTOR('',#82837,1000.) ;
#13224=VECTOR('',#82838,1000.) ;
#13225=VECTOR('',#82839,1000.) ;
#13226=VECTOR('',#82844,1000.) ;
#13227=VECTOR('',#82845,1000.) ;
#13228=VECTOR('',#82846,1000.) ;
#13229=VECTOR('',#82847,1000.) ;
#13230=VECTOR('',#82852,1000.) ;
#13231=VECTOR('',#82853,1000.) ;
#13232=VECTOR('',#82856,1000.) ;
#13233=VECTOR('',#82859,1000.) ;
#13234=VECTOR('',#82862,1000.) ;
#13235=VECTOR('',#82863,1000.) ;
#13236=VECTOR('',#82864,1000.) ;
#13237=VECTOR('',#82865,1000.) ;
#13238=VECTOR('',#82868,1000.) ;
#13239=VECTOR('',#82869,1000.) ;
#13240=VECTOR('',#82870,1000.) ;
#13241=VECTOR('',#82871,1000.) ;
#13242=VECTOR('',#82874,1000.) ;
#13243=VECTOR('',#82875,1000.) ;
#13244=VECTOR('',#82876,1000.) ;
#13245=VECTOR('',#82877,1000.) ;
#13246=VECTOR('',#82880,1000.) ;
#13247=VECTOR('',#82881,1000.) ;
#13248=VECTOR('',#82882,1000.) ;
#13249=VECTOR('',#82883,1000.) ;
#13250=VECTOR('',#82886,1000.) ;
#13251=VECTOR('',#82887,1000.) ;
#13252=VECTOR('',#82888,1000.) ;
#13253=VECTOR('',#82891,1000.) ;
#13254=VECTOR('',#82892,1000.) ;
#13255=VECTOR('',#82893,1000.) ;
#13256=VECTOR('',#82896,1000.) ;
#13257=VECTOR('',#82897,1000.) ;
#13258=VECTOR('',#82898,1000.) ;
#13259=VECTOR('',#82901,1000.) ;
#13260=VECTOR('',#82902,1000.) ;
#13261=VECTOR('',#82903,1000.) ;
#13262=VECTOR('',#82906,1000.) ;
#13263=VECTOR('',#82907,1000.) ;
#13264=VECTOR('',#82908,1000.) ;
#13265=VECTOR('',#82911,1000.) ;
#13266=VECTOR('',#82916,1000.) ;
#13267=VECTOR('',#82917,1000.) ;
#13268=VECTOR('',#82918,1000.) ;
#13269=VECTOR('',#82921,1000.) ;
#13270=VECTOR('',#82926,1000.) ;
#13271=VECTOR('',#82933,1000.) ;
#13272=VECTOR('',#82934,1000.) ;
#13273=VECTOR('',#82935,1000.) ;
#13274=VECTOR('',#82938,1000.) ;
#13275=VECTOR('',#82939,1000.) ;
#13276=VECTOR('',#82940,1000.) ;
#13277=VECTOR('',#82941,1000.) ;
#13278=VECTOR('',#82944,1000.) ;
#13279=VECTOR('',#82945,1000.) ;
#13280=VECTOR('',#82946,1000.) ;
#13281=VECTOR('',#82947,1000.) ;
#13282=VECTOR('',#82950,1000.) ;
#13283=VECTOR('',#82951,1000.) ;
#13284=VECTOR('',#82952,1000.) ;
#13285=VECTOR('',#82953,1000.) ;
#13286=VECTOR('',#82956,1000.) ;
#13287=VECTOR('',#82957,1000.) ;
#13288=VECTOR('',#82958,1000.) ;
#13289=VECTOR('',#82959,1000.) ;
#13290=VECTOR('',#82968,1000.) ;
#13291=VECTOR('',#82969,1000.) ;
#13292=VECTOR('',#82970,1000.) ;
#13293=VECTOR('',#82971,1000.) ;
#13294=VECTOR('',#82974,1000.) ;
#13295=VECTOR('',#82975,1000.) ;
#13296=VECTOR('',#82976,1000.) ;
#13297=VECTOR('',#82977,1000.) ;
#13298=VECTOR('',#82980,1000.) ;
#13299=VECTOR('',#82981,1000.) ;
#13300=VECTOR('',#82982,1000.) ;
#13301=VECTOR('',#82983,1000.) ;
#13302=VECTOR('',#82986,1000.) ;
#13303=VECTOR('',#82987,1000.) ;
#13304=VECTOR('',#82988,1000.) ;
#13305=VECTOR('',#82989,1000.) ;
#13306=VECTOR('',#82992,1000.) ;
#13307=VECTOR('',#82995,1000.) ;
#13308=VECTOR('',#83006,1000.) ;
#13309=VECTOR('',#83009,1000.) ;
#13310=VECTOR('',#83188,1000.) ;
#13311=VECTOR('',#83213,1000.) ;
#13312=VECTOR('',#83226,1000.) ;
#13313=VECTOR('',#83261,1000.) ;
#13314=VECTOR('',#83272,1000.) ;
#13315=VECTOR('',#83295,1000.) ;
#13316=VECTOR('',#83882,1000.) ;
#13317=VECTOR('',#83887,1000.) ;
#13318=VECTOR('',#83892,1000.) ;
#13319=VECTOR('',#83895,1000.) ;
#13320=VECTOR('',#83908,1.5) ;
#13321=VECTOR('',#83911,1000.) ;
#13322=VECTOR('',#83918,1000.) ;
#13323=VECTOR('',#83921,1000.) ;
#13324=VECTOR('',#83922,1000.) ;
#13325=VECTOR('',#83923,1000.) ;
#13326=VECTOR('',#83926,1000.) ;
#13327=VECTOR('',#83929,1000.) ;
#13328=VECTOR('',#83930,1000.) ;
#13329=VECTOR('',#83931,999.999999999999) ;
#13330=VECTOR('',#83932,1000.) ;
#13331=VECTOR('',#83935,1000.) ;
#13332=VECTOR('',#83936,1000.) ;
#13333=VECTOR('',#83937,1000.) ;
#13334=VECTOR('',#83938,1000.) ;
#13335=VECTOR('',#83941,1000.) ;
#13336=VECTOR('',#83942,1000.) ;
#13337=VECTOR('',#83943,1000.) ;
#13338=VECTOR('',#83944,1000.) ;
#13339=VECTOR('',#83947,1000.) ;
#13340=VECTOR('',#83948,1000.) ;
#13341=VECTOR('',#83949,1000.) ;
#13342=VECTOR('',#83950,1000.) ;
#13343=VECTOR('',#83953,1000.) ;
#13344=VECTOR('',#83954,1000.) ;
#13345=VECTOR('',#83955,1000.) ;
#13346=VECTOR('',#83956,1000.) ;
#13347=VECTOR('',#83959,1000.) ;
#13348=VECTOR('',#83960,1000.) ;
#13349=VECTOR('',#83961,1000.) ;
#13350=VECTOR('',#83962,1000.) ;
#13351=VECTOR('',#83965,1000.) ;
#13352=VECTOR('',#83968,1000.) ;
#13353=VECTOR('',#83977,1000.) ;
#13354=VECTOR('',#83980,1000.) ;
#13355=VECTOR('',#83983,1000.) ;
#13356=VECTOR('',#83986,1000.) ;
#13357=VECTOR('',#83989,1000.) ;
#13358=VECTOR('',#83992,1000.) ;
#13359=VECTOR('',#83997,1000.) ;
#13360=VECTOR('',#84002,1000.) ;
#13361=VECTOR('',#84003,1000.) ;
#13362=VECTOR('',#84006,1000.) ;
#13363=VECTOR('',#84009,1000.) ;
#13364=VECTOR('',#84014,1000.) ;
#13365=VECTOR('',#84017,1000.) ;
#13366=VECTOR('',#84020,1000.) ;
#13367=VECTOR('',#84023,1000.) ;
#13368=VECTOR('',#84026,1000.) ;
#13369=VECTOR('',#84027,1000.) ;
#13370=VECTOR('',#84032,1000.) ;
#13371=VECTOR('',#84037,1000.) ;
#13372=VECTOR('',#84040,1000.) ;
#13373=VECTOR('',#84043,1000.) ;
#13374=VECTOR('',#84046,1000.) ;
#13375=VECTOR('',#84049,1000.) ;
#13376=VECTOR('',#84052,1000.) ;
#13377=VECTOR('',#84055,1000.) ;
#13378=VECTOR('',#84058,1000.) ;
#13379=VECTOR('',#84063,1000.) ;
#13380=VECTOR('',#84064,1000.) ;
#13381=VECTOR('',#84067,1000.) ;
#13382=VECTOR('',#84068,1000.) ;
#13383=VECTOR('',#84071,1000.) ;
#13384=VECTOR('',#84072,1000.) ;
#13385=VECTOR('',#84073,1000.) ;
#13386=VECTOR('',#84074,1000.) ;
#13387=VECTOR('',#84079,1000.) ;
#13388=VECTOR('',#84080,1000.) ;
#13389=VECTOR('',#84081,999.999999999999) ;
#13390=VECTOR('',#84084,1000.) ;
#13391=VECTOR('',#84085,1000.) ;
#13392=VECTOR('',#84086,1000.) ;
#13393=VECTOR('',#84089,1000.) ;
#13394=VECTOR('',#84090,1000.) ;
#13395=VECTOR('',#84091,1000.) ;
#13396=VECTOR('',#84094,1000.) ;
#13397=VECTOR('',#84095,1000.) ;
#13398=VECTOR('',#84096,1000.) ;
#13399=VECTOR('',#84097,1000.) ;
#13400=VECTOR('',#84098,1000.) ;
#13401=VECTOR('',#84101,1000.) ;
#13402=VECTOR('',#84104,1000.) ;
#13403=VECTOR('',#84105,1000.) ;
#13404=VECTOR('',#84110,1000.) ;
#13405=VECTOR('',#84111,1000.) ;
#13406=VECTOR('',#84118,1000.) ;
#13407=VECTOR('',#84119,1000.) ;
#13408=VECTOR('',#84120,1000.) ;
#13409=VECTOR('',#84127,1000.) ;
#13410=VECTOR('',#84128,1000.) ;
#13411=VECTOR('',#84135,1000.) ;
#13412=VECTOR('',#84138,1000.) ;
#13413=VECTOR('',#84147,1000.) ;
#13414=VECTOR('',#84148,1000.) ;
#13415=VECTOR('',#84149,1000.) ;
#13416=VECTOR('',#84150,1000.) ;
#13417=VECTOR('',#84151,1000.) ;
#13418=VECTOR('',#84154,1000.) ;
#13419=VECTOR('',#84159,1000.) ;
#13420=VECTOR('',#84160,1000.) ;
#13421=VECTOR('',#84161,1000.) ;
#13422=VECTOR('',#84164,1000.) ;
#13423=VECTOR('',#84167,1000.) ;
#13424=VECTOR('',#84168,1000.) ;
#13425=VECTOR('',#84175,1000.) ;
#13426=VECTOR('',#84176,1000.) ;
#13427=VECTOR('',#84179,1000.) ;
#13428=VECTOR('',#84180,1000.) ;
#13429=VECTOR('',#84181,1000.) ;
#13430=VECTOR('',#84182,1000.) ;
#13431=VECTOR('',#84183,1000.) ;
#13432=VECTOR('',#84184,1000.) ;
#13433=VECTOR('',#84185,1000.) ;
#13434=VECTOR('',#84186,1000.) ;
#13435=VECTOR('',#84189,1000.) ;
#13436=VECTOR('',#84190,1000.) ;
#13437=VECTOR('',#84191,1000.) ;
#13438=VECTOR('',#84192,1000.) ;
#13439=VECTOR('',#84195,1000.) ;
#13440=VECTOR('',#84196,1000.) ;
#13441=VECTOR('',#84197,1000.) ;
#13442=VECTOR('',#84198,1000.) ;
#13443=VECTOR('',#84201,1000.) ;
#13444=VECTOR('',#84202,1000.) ;
#13445=VECTOR('',#84203,1000.) ;
#13446=VECTOR('',#84204,1000.) ;
#13447=VECTOR('',#84207,1000.) ;
#13448=VECTOR('',#84208,1000.) ;
#13449=VECTOR('',#84209,1000.) ;
#13450=VECTOR('',#84210,1000.) ;
#13451=VECTOR('',#84213,1000.) ;
#13452=VECTOR('',#84214,1000.) ;
#13453=VECTOR('',#84215,1000.) ;
#13454=VECTOR('',#84216,1000.) ;
#13455=VECTOR('',#84217,1000.) ;
#13456=VECTOR('',#84218,1000.) ;
#13457=VECTOR('',#84219,1000.) ;
#13458=VECTOR('',#84220,1000.) ;
#13459=VECTOR('',#84223,1000.) ;
#13460=VECTOR('',#84226,1000.) ;
#13461=VECTOR('',#84229,1000.) ;
#13462=VECTOR('',#84232,1000.) ;
#13463=VECTOR('',#84239,1000.) ;
#13464=VECTOR('',#84240,1000.) ;
#13465=VECTOR('',#84243,1000.) ;
#13466=VECTOR('',#84248,1000.) ;
#13467=VECTOR('',#84249,1000.) ;
#13468=VECTOR('',#84250,1000.) ;
#13469=VECTOR('',#84253,1000.) ;
#13470=VECTOR('',#84254,1000.) ;
#13471=VECTOR('',#84255,1000.) ;
#13472=VECTOR('',#84260,1000.) ;
#13473=VECTOR('',#84263,1000.) ;
#13474=VECTOR('',#84268,1000.) ;
#13475=VECTOR('',#84271,1000.) ;
#13476=VECTOR('',#84274,1000.) ;
#13477=VECTOR('',#84275,1000.) ;
#13478=VECTOR('',#84276,1000.) ;
#13479=VECTOR('',#84279,1000.) ;
#13480=VECTOR('',#84280,1000.) ;
#13481=VECTOR('',#84281,1000.) ;
#13482=VECTOR('',#84286,1000.) ;
#13483=VECTOR('',#84287,1000.) ;
#13484=VECTOR('',#84292,1000.) ;
#13485=VECTOR('',#84297,1000.) ;
#13486=VECTOR('',#84298,1000.) ;
#13487=VECTOR('',#84299,1000.) ;
#13488=VECTOR('',#84302,1000.) ;
#13489=VECTOR('',#84303,1000.) ;
#13490=VECTOR('',#84304,1000.) ;
#13491=VECTOR('',#84309,1000.) ;
#13492=VECTOR('',#84312,1000.) ;
#13493=VECTOR('',#84315,1000.) ;
#13494=VECTOR('',#84316,1000.) ;
#13495=VECTOR('',#84317,1000.) ;
#13496=VECTOR('',#84318,1000.) ;
#13497=VECTOR('',#84323,1000.) ;
#13498=VECTOR('',#84326,1000.) ;
#13499=VECTOR('',#84329,1000.) ;
#13500=VECTOR('',#84330,1000.) ;
#13501=VECTOR('',#84331,1000.) ;
#13502=VECTOR('',#84334,1000.) ;
#13503=VECTOR('',#84335,1000.) ;
#13504=VECTOR('',#84336,1000.) ;
#13505=VECTOR('',#84337,1000.) ;
#13506=VECTOR('',#84340,1000.) ;
#13507=VECTOR('',#84341,1000.) ;
#13508=VECTOR('',#84342,1000.) ;
#13509=VECTOR('',#84347,1000.) ;
#13510=VECTOR('',#84348,1000.) ;
#13511=VECTOR('',#84349,1000.) ;
#13512=VECTOR('',#84350,1000.) ;
#13513=VECTOR('',#84355,1000.) ;
#13514=VECTOR('',#84356,1000.) ;
#13515=VECTOR('',#84359,1000.) ;
#13516=VECTOR('',#84362,1000.) ;
#13517=VECTOR('',#84365,1000.) ;
#13518=VECTOR('',#84366,1000.) ;
#13519=VECTOR('',#84367,1000.) ;
#13520=VECTOR('',#84368,1000.) ;
#13521=VECTOR('',#84371,1000.) ;
#13522=VECTOR('',#84372,1000.) ;
#13523=VECTOR('',#84373,1000.) ;
#13524=VECTOR('',#84374,1000.) ;
#13525=VECTOR('',#84377,1000.) ;
#13526=VECTOR('',#84378,1000.) ;
#13527=VECTOR('',#84379,1000.) ;
#13528=VECTOR('',#84380,1000.) ;
#13529=VECTOR('',#84383,1000.) ;
#13530=VECTOR('',#84384,1000.) ;
#13531=VECTOR('',#84385,1000.) ;
#13532=VECTOR('',#84386,1000.) ;
#13533=VECTOR('',#84389,1000.) ;
#13534=VECTOR('',#84390,1000.) ;
#13535=VECTOR('',#84391,1000.) ;
#13536=VECTOR('',#84394,1000.) ;
#13537=VECTOR('',#84395,1000.) ;
#13538=VECTOR('',#84396,1000.) ;
#13539=VECTOR('',#84399,1000.) ;
#13540=VECTOR('',#84400,1000.) ;
#13541=VECTOR('',#84401,1000.) ;
#13542=VECTOR('',#84404,1000.) ;
#13543=VECTOR('',#84405,1000.) ;
#13544=VECTOR('',#84406,1000.) ;
#13545=VECTOR('',#84409,1000.) ;
#13546=VECTOR('',#84410,1000.) ;
#13547=VECTOR('',#84411,1000.) ;
#13548=VECTOR('',#84414,1000.) ;
#13549=VECTOR('',#84419,1000.) ;
#13550=VECTOR('',#84420,1000.) ;
#13551=VECTOR('',#84421,1000.) ;
#13552=VECTOR('',#84424,1000.) ;
#13553=VECTOR('',#84429,1000.) ;
#13554=VECTOR('',#84436,1000.) ;
#13555=VECTOR('',#84437,1000.) ;
#13556=VECTOR('',#84438,1000.) ;
#13557=VECTOR('',#84441,1000.) ;
#13558=VECTOR('',#84442,1000.) ;
#13559=VECTOR('',#84443,1000.) ;
#13560=VECTOR('',#84444,1000.) ;
#13561=VECTOR('',#84447,1000.) ;
#13562=VECTOR('',#84448,1000.) ;
#13563=VECTOR('',#84449,1000.) ;
#13564=VECTOR('',#84450,1000.) ;
#13565=VECTOR('',#84453,1000.) ;
#13566=VECTOR('',#84454,1000.) ;
#13567=VECTOR('',#84455,1000.) ;
#13568=VECTOR('',#84456,1000.) ;
#13569=VECTOR('',#84459,1000.) ;
#13570=VECTOR('',#84460,1000.) ;
#13571=VECTOR('',#84461,1000.) ;
#13572=VECTOR('',#84462,1000.) ;
#13573=VECTOR('',#84471,1000.) ;
#13574=VECTOR('',#84472,1000.) ;
#13575=VECTOR('',#84473,1000.) ;
#13576=VECTOR('',#84474,1000.) ;
#13577=VECTOR('',#84477,1000.) ;
#13578=VECTOR('',#84478,1000.) ;
#13579=VECTOR('',#84479,1000.) ;
#13580=VECTOR('',#84480,1000.) ;
#13581=VECTOR('',#84483,1000.) ;
#13582=VECTOR('',#84484,1000.) ;
#13583=VECTOR('',#84485,1000.) ;
#13584=VECTOR('',#84486,1000.) ;
#13585=VECTOR('',#84489,1000.) ;
#13586=VECTOR('',#84490,1000.) ;
#13587=VECTOR('',#84491,1000.) ;
#13588=VECTOR('',#84492,1000.) ;
#13589=VECTOR('',#84495,1000.) ;
#13590=VECTOR('',#84498,1000.) ;
#13591=VECTOR('',#84509,1000.) ;
#13592=VECTOR('',#84512,1000.) ;
#13593=VECTOR('',#84691,1000.) ;
#13594=VECTOR('',#84716,1000.) ;
#13595=VECTOR('',#84729,1000.) ;
#13596=VECTOR('',#84764,1000.) ;
#13597=VECTOR('',#84775,1000.) ;
#13598=VECTOR('',#84798,1000.) ;
#13599=VECTOR('',#85385,1000.) ;
#13600=VECTOR('',#85390,1000.) ;
#13601=VECTOR('',#85395,1000.) ;
#13602=VECTOR('',#85398,1000.) ;
#13603=VECTOR('',#85411,1.5) ;
#13604=VECTOR('',#85414,1000.) ;
#13605=VECTOR('',#85421,1000.) ;
#13606=VECTOR('',#85424,1000.) ;
#13607=VECTOR('',#85425,1000.) ;
#13608=VECTOR('',#85426,1000.) ;
#13609=VECTOR('',#85429,1000.) ;
#13610=VECTOR('',#85432,1000.) ;
#13611=VECTOR('',#85433,1000.) ;
#13612=VECTOR('',#85434,1000.) ;
#13613=VECTOR('',#85435,1000.) ;
#13614=VECTOR('',#85438,1000.) ;
#13615=VECTOR('',#85439,1000.) ;
#13616=VECTOR('',#85440,1000.) ;
#13617=VECTOR('',#85441,1000.) ;
#13618=VECTOR('',#85444,1000.) ;
#13619=VECTOR('',#85445,1000.) ;
#13620=VECTOR('',#85446,1000.) ;
#13621=VECTOR('',#85447,1000.) ;
#13622=VECTOR('',#85450,1000.) ;
#13623=VECTOR('',#85451,1000.) ;
#13624=VECTOR('',#85452,1000.) ;
#13625=VECTOR('',#85453,1000.) ;
#13626=VECTOR('',#85456,1000.) ;
#13627=VECTOR('',#85457,1000.) ;
#13628=VECTOR('',#85458,1000.) ;
#13629=VECTOR('',#85459,1000.) ;
#13630=VECTOR('',#85462,1000.) ;
#13631=VECTOR('',#85463,1000.) ;
#13632=VECTOR('',#85464,1000.) ;
#13633=VECTOR('',#85465,1000.) ;
#13634=VECTOR('',#85468,1000.) ;
#13635=VECTOR('',#85471,1000.) ;
#13636=VECTOR('',#85480,1000.) ;
#13637=VECTOR('',#85483,1000.) ;
#13638=VECTOR('',#85486,1000.) ;
#13639=VECTOR('',#85489,1000.) ;
#13640=VECTOR('',#85492,1000.) ;
#13641=VECTOR('',#85495,1000.) ;
#13642=VECTOR('',#85500,1000.) ;
#13643=VECTOR('',#85505,1000.) ;
#13644=VECTOR('',#85506,1000.) ;
#13645=VECTOR('',#85509,1000.) ;
#13646=VECTOR('',#85512,1000.) ;
#13647=VECTOR('',#85517,1000.) ;
#13648=VECTOR('',#85520,1000.) ;
#13649=VECTOR('',#85523,1000.) ;
#13650=VECTOR('',#85526,1000.) ;
#13651=VECTOR('',#85529,1000.) ;
#13652=VECTOR('',#85530,1000.) ;
#13653=VECTOR('',#85535,1000.) ;
#13654=VECTOR('',#85540,1000.) ;
#13655=VECTOR('',#85543,1000.) ;
#13656=VECTOR('',#85546,1000.) ;
#13657=VECTOR('',#85549,1000.) ;
#13658=VECTOR('',#85552,1000.) ;
#13659=VECTOR('',#85555,1000.) ;
#13660=VECTOR('',#85558,1000.) ;
#13661=VECTOR('',#85561,1000.) ;
#13662=VECTOR('',#85566,1000.) ;
#13663=VECTOR('',#85567,1000.) ;
#13664=VECTOR('',#85570,1000.) ;
#13665=VECTOR('',#85571,1000.) ;
#13666=VECTOR('',#85574,1000.) ;
#13667=VECTOR('',#85575,1000.) ;
#13668=VECTOR('',#85576,1000.) ;
#13669=VECTOR('',#85577,1000.) ;
#13670=VECTOR('',#85582,1000.) ;
#13671=VECTOR('',#85583,1000.) ;
#13672=VECTOR('',#85584,999.999999999999) ;
#13673=VECTOR('',#85587,1000.) ;
#13674=VECTOR('',#85588,1000.) ;
#13675=VECTOR('',#85589,1000.) ;
#13676=VECTOR('',#85592,1000.) ;
#13677=VECTOR('',#85593,1000.) ;
#13678=VECTOR('',#85594,1000.) ;
#13679=VECTOR('',#85597,1000.) ;
#13680=VECTOR('',#85598,1000.) ;
#13681=VECTOR('',#85599,1000.) ;
#13682=VECTOR('',#85600,1000.) ;
#13683=VECTOR('',#85601,1000.) ;
#13684=VECTOR('',#85604,1000.) ;
#13685=VECTOR('',#85607,1000.) ;
#13686=VECTOR('',#85608,1000.) ;
#13687=VECTOR('',#85613,1000.) ;
#13688=VECTOR('',#85614,1000.) ;
#13689=VECTOR('',#85621,1000.) ;
#13690=VECTOR('',#85622,1000.) ;
#13691=VECTOR('',#85623,1000.) ;
#13692=VECTOR('',#85630,1000.) ;
#13693=VECTOR('',#85631,1000.) ;
#13694=VECTOR('',#85638,1000.) ;
#13695=VECTOR('',#85641,1000.) ;
#13696=VECTOR('',#85650,1000.) ;
#13697=VECTOR('',#85651,1000.) ;
#13698=VECTOR('',#85652,1000.) ;
#13699=VECTOR('',#85653,1000.) ;
#13700=VECTOR('',#85654,1000.) ;
#13701=VECTOR('',#85657,1000.) ;
#13702=VECTOR('',#85662,1000.) ;
#13703=VECTOR('',#85663,1000.) ;
#13704=VECTOR('',#85664,1000.) ;
#13705=VECTOR('',#85667,1000.) ;
#13706=VECTOR('',#85670,1000.) ;
#13707=VECTOR('',#85671,1000.) ;
#13708=VECTOR('',#85678,1000.) ;
#13709=VECTOR('',#85679,1000.) ;
#13710=VECTOR('',#85682,1000.) ;
#13711=VECTOR('',#85683,1000.) ;
#13712=VECTOR('',#85684,1000.) ;
#13713=VECTOR('',#85685,1000.) ;
#13714=VECTOR('',#85686,1000.) ;
#13715=VECTOR('',#85687,1000.) ;
#13716=VECTOR('',#85688,1000.) ;
#13717=VECTOR('',#85689,1000.) ;
#13718=VECTOR('',#85692,1000.) ;
#13719=VECTOR('',#85693,1000.) ;
#13720=VECTOR('',#85694,1000.) ;
#13721=VECTOR('',#85695,1000.) ;
#13722=VECTOR('',#85698,1000.) ;
#13723=VECTOR('',#85699,1000.) ;
#13724=VECTOR('',#85700,1000.) ;
#13725=VECTOR('',#85701,1000.) ;
#13726=VECTOR('',#85704,1000.) ;
#13727=VECTOR('',#85705,1000.) ;
#13728=VECTOR('',#85706,1000.) ;
#13729=VECTOR('',#85707,1000.) ;
#13730=VECTOR('',#85710,1000.) ;
#13731=VECTOR('',#85711,1000.) ;
#13732=VECTOR('',#85712,1000.) ;
#13733=VECTOR('',#85713,1000.) ;
#13734=VECTOR('',#85716,1000.) ;
#13735=VECTOR('',#85717,1000.) ;
#13736=VECTOR('',#85718,1000.) ;
#13737=VECTOR('',#85719,1000.) ;
#13738=VECTOR('',#85720,1000.) ;
#13739=VECTOR('',#85721,1000.) ;
#13740=VECTOR('',#85722,1000.) ;
#13741=VECTOR('',#85723,1000.) ;
#13742=VECTOR('',#85726,1000.) ;
#13743=VECTOR('',#85729,1000.) ;
#13744=VECTOR('',#85732,1000.) ;
#13745=VECTOR('',#85735,1000.) ;
#13746=VECTOR('',#85742,1000.) ;
#13747=VECTOR('',#85743,1000.) ;
#13748=VECTOR('',#85746,1000.) ;
#13749=VECTOR('',#85751,1000.) ;
#13750=VECTOR('',#85752,1000.) ;
#13751=VECTOR('',#85753,1000.) ;
#13752=VECTOR('',#85756,1000.) ;
#13753=VECTOR('',#85757,1000.) ;
#13754=VECTOR('',#85758,1000.) ;
#13755=VECTOR('',#85763,1000.) ;
#13756=VECTOR('',#85766,1000.) ;
#13757=VECTOR('',#85771,1000.) ;
#13758=VECTOR('',#85774,1000.) ;
#13759=VECTOR('',#85777,1000.) ;
#13760=VECTOR('',#85778,1000.) ;
#13761=VECTOR('',#85779,1000.) ;
#13762=VECTOR('',#85782,1000.) ;
#13763=VECTOR('',#85783,1000.) ;
#13764=VECTOR('',#85784,1000.) ;
#13765=VECTOR('',#85789,1000.) ;
#13766=VECTOR('',#85790,1000.) ;
#13767=VECTOR('',#85795,1000.) ;
#13768=VECTOR('',#85800,1000.) ;
#13769=VECTOR('',#85801,1000.) ;
#13770=VECTOR('',#85802,1000.) ;
#13771=VECTOR('',#85805,1000.) ;
#13772=VECTOR('',#85806,1000.) ;
#13773=VECTOR('',#85807,1000.) ;
#13774=VECTOR('',#85812,1000.) ;
#13775=VECTOR('',#85815,1000.) ;
#13776=VECTOR('',#85818,1000.) ;
#13777=VECTOR('',#85819,1000.) ;
#13778=VECTOR('',#85820,1000.) ;
#13779=VECTOR('',#85821,1000.) ;
#13780=VECTOR('',#85826,1000.) ;
#13781=VECTOR('',#85829,1000.) ;
#13782=VECTOR('',#85832,1000.) ;
#13783=VECTOR('',#85833,1000.) ;
#13784=VECTOR('',#85834,1000.) ;
#13785=VECTOR('',#85837,1000.) ;
#13786=VECTOR('',#85838,1000.) ;
#13787=VECTOR('',#85839,1000.) ;
#13788=VECTOR('',#85840,1000.) ;
#13789=VECTOR('',#85843,1000.) ;
#13790=VECTOR('',#85844,1000.) ;
#13791=VECTOR('',#85845,1000.) ;
#13792=VECTOR('',#85850,1000.) ;
#13793=VECTOR('',#85851,1000.) ;
#13794=VECTOR('',#85852,1000.) ;
#13795=VECTOR('',#85853,1000.) ;
#13796=VECTOR('',#85858,1000.) ;
#13797=VECTOR('',#85859,1000.) ;
#13798=VECTOR('',#85862,1000.) ;
#13799=VECTOR('',#85865,1000.) ;
#13800=VECTOR('',#85868,1000.) ;
#13801=VECTOR('',#85869,1000.) ;
#13802=VECTOR('',#85870,1000.) ;
#13803=VECTOR('',#85871,1000.) ;
#13804=VECTOR('',#85874,1000.) ;
#13805=VECTOR('',#85875,1000.) ;
#13806=VECTOR('',#85876,1000.) ;
#13807=VECTOR('',#85877,1000.) ;
#13808=VECTOR('',#85880,1000.) ;
#13809=VECTOR('',#85881,1000.) ;
#13810=VECTOR('',#85882,1000.) ;
#13811=VECTOR('',#85883,1000.) ;
#13812=VECTOR('',#85886,1000.) ;
#13813=VECTOR('',#85887,1000.) ;
#13814=VECTOR('',#85888,1000.) ;
#13815=VECTOR('',#85889,1000.) ;
#13816=VECTOR('',#85892,1000.) ;
#13817=VECTOR('',#85893,1000.) ;
#13818=VECTOR('',#85894,1000.) ;
#13819=VECTOR('',#85897,1000.) ;
#13820=VECTOR('',#85898,1000.) ;
#13821=VECTOR('',#85899,1000.) ;
#13822=VECTOR('',#85902,1000.) ;
#13823=VECTOR('',#85903,1000.) ;
#13824=VECTOR('',#85904,1000.) ;
#13825=VECTOR('',#85907,1000.) ;
#13826=VECTOR('',#85908,1000.) ;
#13827=VECTOR('',#85909,1000.) ;
#13828=VECTOR('',#85912,1000.) ;
#13829=VECTOR('',#85913,1000.) ;
#13830=VECTOR('',#85914,1000.) ;
#13831=VECTOR('',#85917,1000.) ;
#13832=VECTOR('',#85922,1000.) ;
#13833=VECTOR('',#85923,1000.) ;
#13834=VECTOR('',#85924,1000.) ;
#13835=VECTOR('',#85927,1000.) ;
#13836=VECTOR('',#85932,1000.) ;
#13837=VECTOR('',#85939,1000.) ;
#13838=VECTOR('',#85940,1000.) ;
#13839=VECTOR('',#85941,1000.) ;
#13840=VECTOR('',#85944,1000.) ;
#13841=VECTOR('',#85945,1000.) ;
#13842=VECTOR('',#85946,1000.) ;
#13843=VECTOR('',#85947,1000.) ;
#13844=VECTOR('',#85950,1000.) ;
#13845=VECTOR('',#85951,1000.) ;
#13846=VECTOR('',#85952,1000.) ;
#13847=VECTOR('',#85953,1000.) ;
#13848=VECTOR('',#85956,1000.) ;
#13849=VECTOR('',#85957,1000.) ;
#13850=VECTOR('',#85958,1000.) ;
#13851=VECTOR('',#85959,1000.) ;
#13852=VECTOR('',#85962,1000.) ;
#13853=VECTOR('',#85963,1000.) ;
#13854=VECTOR('',#85964,1000.) ;
#13855=VECTOR('',#85965,1000.) ;
#13856=VECTOR('',#85974,1000.) ;
#13857=VECTOR('',#85975,1000.) ;
#13858=VECTOR('',#85976,1000.) ;
#13859=VECTOR('',#85977,1000.) ;
#13860=VECTOR('',#85980,1000.) ;
#13861=VECTOR('',#85981,1000.) ;
#13862=VECTOR('',#85982,1000.) ;
#13863=VECTOR('',#85983,1000.) ;
#13864=VECTOR('',#85986,1000.) ;
#13865=VECTOR('',#85987,1000.) ;
#13866=VECTOR('',#85988,1000.) ;
#13867=VECTOR('',#85989,1000.) ;
#13868=VECTOR('',#85992,1000.) ;
#13869=VECTOR('',#85993,1000.) ;
#13870=VECTOR('',#85994,1000.) ;
#13871=VECTOR('',#85995,1000.) ;
#13872=VECTOR('',#85998,1000.) ;
#13873=VECTOR('',#86001,1000.) ;
#13874=VECTOR('',#86012,1000.) ;
#13875=VECTOR('',#86015,1000.) ;
#13876=VECTOR('',#86194,1000.) ;
#13877=VECTOR('',#86219,1000.) ;
#13878=VECTOR('',#86232,1000.) ;
#13879=VECTOR('',#86267,1000.) ;
#13880=VECTOR('',#86278,1000.) ;
#13881=VECTOR('',#86301,1000.) ;
#16130=CONICAL_SURFACE('',#68967,3.,0.165148677414624) ;
#16131=CONICAL_SURFACE('',#69577,3.,0.165148677414624) ;
#16132=CONICAL_SURFACE('',#70187,3.,0.165148677414624) ;
#16133=CONICAL_SURFACE('',#70797,3.,0.165148677414624) ;
#16134=CONICAL_SURFACE('',#71407,3.,0.165148677414624) ;
#16610=FACE_OUTER_BOUND('',#20882,.T.) ;
#16611=FACE_OUTER_BOUND('',#20883,.T.) ;
#16612=FACE_OUTER_BOUND('',#20884,.T.) ;
#16613=FACE_OUTER_BOUND('',#20885,.T.) ;
#16614=FACE_OUTER_BOUND('',#20886,.T.) ;
#16615=FACE_OUTER_BOUND('',#20887,.T.) ;
#16616=FACE_OUTER_BOUND('',#20888,.T.) ;
#16617=FACE_OUTER_BOUND('',#20889,.T.) ;
#16618=FACE_OUTER_BOUND('',#20890,.T.) ;
#16619=FACE_OUTER_BOUND('',#20891,.T.) ;
#16620=FACE_OUTER_BOUND('',#20892,.T.) ;
#16621=FACE_OUTER_BOUND('',#20893,.T.) ;
#16622=FACE_OUTER_BOUND('',#20894,.T.) ;
#16623=FACE_OUTER_BOUND('',#20895,.T.) ;
#16624=FACE_OUTER_BOUND('',#20896,.T.) ;
#16625=FACE_OUTER_BOUND('',#20897,.T.) ;
#16626=FACE_OUTER_BOUND('',#20898,.T.) ;
#16627=FACE_OUTER_BOUND('',#20899,.T.) ;
#16628=FACE_OUTER_BOUND('',#20900,.T.) ;
#16629=FACE_OUTER_BOUND('',#20901,.T.) ;
#16630=FACE_OUTER_BOUND('',#20902,.T.) ;
#16631=FACE_OUTER_BOUND('',#20903,.T.) ;
#16632=FACE_OUTER_BOUND('',#20904,.T.) ;
#16633=FACE_OUTER_BOUND('',#20905,.T.) ;
#16634=FACE_OUTER_BOUND('',#20906,.T.) ;
#16635=FACE_OUTER_BOUND('',#20907,.T.) ;
#16636=FACE_OUTER_BOUND('',#20909,.T.) ;
#16637=FACE_OUTER_BOUND('',#20910,.T.) ;
#16638=FACE_OUTER_BOUND('',#20911,.T.) ;
#16639=FACE_OUTER_BOUND('',#20912,.T.) ;
#16640=FACE_OUTER_BOUND('',#20913,.T.) ;
#16641=FACE_OUTER_BOUND('',#20914,.T.) ;
#16642=FACE_OUTER_BOUND('',#20915,.T.) ;
#16643=FACE_OUTER_BOUND('',#20916,.T.) ;
#16644=FACE_OUTER_BOUND('',#20917,.T.) ;
#16645=FACE_OUTER_BOUND('',#20918,.T.) ;
#16646=FACE_OUTER_BOUND('',#20919,.T.) ;
#16647=FACE_OUTER_BOUND('',#20921,.T.) ;
#16648=FACE_OUTER_BOUND('',#20922,.T.) ;
#16649=FACE_OUTER_BOUND('',#20923,.T.) ;
#16650=FACE_OUTER_BOUND('',#20924,.T.) ;
#16651=FACE_OUTER_BOUND('',#20925,.T.) ;
#16652=FACE_OUTER_BOUND('',#20926,.T.) ;
#16653=FACE_OUTER_BOUND('',#20927,.T.) ;
#16654=FACE_OUTER_BOUND('',#20928,.T.) ;
#16655=FACE_OUTER_BOUND('',#20929,.T.) ;
#16656=FACE_OUTER_BOUND('',#20930,.T.) ;
#16657=FACE_OUTER_BOUND('',#20931,.T.) ;
#16658=FACE_OUTER_BOUND('',#20932,.T.) ;
#16659=FACE_OUTER_BOUND('',#20933,.T.) ;
#16660=FACE_OUTER_BOUND('',#20934,.T.) ;
#16661=FACE_OUTER_BOUND('',#20935,.T.) ;
#16662=FACE_OUTER_BOUND('',#20936,.T.) ;
#16663=FACE_OUTER_BOUND('',#20937,.T.) ;
#16664=FACE_OUTER_BOUND('',#20938,.T.) ;
#16665=FACE_OUTER_BOUND('',#20939,.T.) ;
#16666=FACE_OUTER_BOUND('',#20940,.T.) ;
#16667=FACE_OUTER_BOUND('',#20941,.T.) ;
#16668=FACE_OUTER_BOUND('',#20942,.T.) ;
#16669=FACE_OUTER_BOUND('',#20943,.T.) ;
#16670=FACE_OUTER_BOUND('',#20944,.T.) ;
#16671=FACE_OUTER_BOUND('',#20945,.T.) ;
#16672=FACE_OUTER_BOUND('',#20946,.T.) ;
#16673=FACE_OUTER_BOUND('',#20947,.T.) ;
#16674=FACE_OUTER_BOUND('',#20948,.T.) ;
#16675=FACE_OUTER_BOUND('',#20949,.T.) ;
#16676=FACE_OUTER_BOUND('',#20950,.T.) ;
#16677=FACE_OUTER_BOUND('',#20951,.T.) ;
#16678=FACE_OUTER_BOUND('',#20952,.T.) ;
#16679=FACE_OUTER_BOUND('',#20953,.T.) ;
#16680=FACE_OUTER_BOUND('',#20954,.T.) ;
#16681=FACE_OUTER_BOUND('',#20955,.T.) ;
#16682=FACE_OUTER_BOUND('',#20956,.T.) ;
#16683=FACE_OUTER_BOUND('',#20957,.T.) ;
#16684=FACE_OUTER_BOUND('',#20958,.T.) ;
#16685=FACE_OUTER_BOUND('',#20959,.T.) ;
#16686=FACE_OUTER_BOUND('',#20960,.T.) ;
#16687=FACE_OUTER_BOUND('',#20961,.T.) ;
#16688=FACE_OUTER_BOUND('',#20962,.T.) ;
#16689=FACE_OUTER_BOUND('',#20963,.T.) ;
#16690=FACE_OUTER_BOUND('',#20964,.T.) ;
#16691=FACE_OUTER_BOUND('',#20965,.T.) ;
#16692=FACE_OUTER_BOUND('',#20966,.T.) ;
#16693=FACE_OUTER_BOUND('',#20967,.T.) ;
#16694=FACE_OUTER_BOUND('',#20968,.T.) ;
#16695=FACE_OUTER_BOUND('',#20969,.T.) ;
#16696=FACE_OUTER_BOUND('',#20970,.T.) ;
#16697=FACE_OUTER_BOUND('',#20971,.T.) ;
#16698=FACE_OUTER_BOUND('',#20972,.T.) ;
#16699=FACE_OUTER_BOUND('',#20973,.T.) ;
#16700=FACE_OUTER_BOUND('',#20974,.T.) ;
#16701=FACE_OUTER_BOUND('',#20975,.T.) ;
#16702=FACE_OUTER_BOUND('',#20976,.T.) ;
#16703=FACE_OUTER_BOUND('',#20977,.T.) ;
#16704=FACE_OUTER_BOUND('',#20978,.T.) ;
#16705=FACE_OUTER_BOUND('',#20979,.T.) ;
#16706=FACE_OUTER_BOUND('',#20980,.T.) ;
#16707=FACE_OUTER_BOUND('',#20981,.T.) ;
#16708=FACE_OUTER_BOUND('',#20982,.T.) ;
#16709=FACE_OUTER_BOUND('',#20983,.T.) ;
#16710=FACE_OUTER_BOUND('',#20984,.T.) ;
#16711=FACE_OUTER_BOUND('',#20985,.T.) ;
#16712=FACE_OUTER_BOUND('',#20986,.T.) ;
#16713=FACE_OUTER_BOUND('',#20987,.T.) ;
#16714=FACE_OUTER_BOUND('',#20988,.T.) ;
#16715=FACE_OUTER_BOUND('',#20989,.T.) ;
#16716=FACE_OUTER_BOUND('',#20990,.T.) ;
#16717=FACE_OUTER_BOUND('',#20991,.T.) ;
#16718=FACE_OUTER_BOUND('',#20992,.T.) ;
#16719=FACE_OUTER_BOUND('',#20993,.T.) ;
#16720=FACE_OUTER_BOUND('',#20994,.T.) ;
#16721=FACE_OUTER_BOUND('',#20995,.T.) ;
#16722=FACE_OUTER_BOUND('',#20996,.T.) ;
#16723=FACE_OUTER_BOUND('',#20997,.T.) ;
#16724=FACE_OUTER_BOUND('',#20998,.T.) ;
#16725=FACE_OUTER_BOUND('',#20999,.T.) ;
#16726=FACE_OUTER_BOUND('',#21000,.T.) ;
#16727=FACE_OUTER_BOUND('',#21001,.T.) ;
#16728=FACE_OUTER_BOUND('',#21002,.T.) ;
#16729=FACE_OUTER_BOUND('',#21003,.T.) ;
#16730=FACE_OUTER_BOUND('',#21004,.T.) ;
#16731=FACE_OUTER_BOUND('',#21005,.T.) ;
#16732=FACE_OUTER_BOUND('',#21006,.T.) ;
#16733=FACE_OUTER_BOUND('',#21007,.T.) ;
#16734=FACE_OUTER_BOUND('',#21008,.T.) ;
#16735=FACE_OUTER_BOUND('',#21009,.T.) ;
#16736=FACE_OUTER_BOUND('',#21010,.T.) ;
#16737=FACE_OUTER_BOUND('',#21011,.T.) ;
#16738=FACE_OUTER_BOUND('',#21012,.T.) ;
#16739=FACE_OUTER_BOUND('',#21013,.T.) ;
#16740=FACE_OUTER_BOUND('',#21014,.T.) ;
#16741=FACE_OUTER_BOUND('',#21015,.T.) ;
#16742=FACE_OUTER_BOUND('',#21016,.T.) ;
#16743=FACE_OUTER_BOUND('',#21017,.T.) ;
#16744=FACE_OUTER_BOUND('',#21018,.T.) ;
#16745=FACE_OUTER_BOUND('',#21019,.T.) ;
#16746=FACE_OUTER_BOUND('',#21020,.T.) ;
#16747=FACE_OUTER_BOUND('',#21021,.T.) ;
#16748=FACE_OUTER_BOUND('',#21022,.T.) ;
#16749=FACE_OUTER_BOUND('',#21023,.T.) ;
#16750=FACE_OUTER_BOUND('',#21024,.T.) ;
#16751=FACE_OUTER_BOUND('',#21025,.T.) ;
#16752=FACE_OUTER_BOUND('',#21026,.T.) ;
#16753=FACE_OUTER_BOUND('',#21027,.T.) ;
#16754=FACE_OUTER_BOUND('',#21028,.T.) ;
#16755=FACE_OUTER_BOUND('',#21029,.T.) ;
#16756=FACE_OUTER_BOUND('',#21030,.T.) ;
#16757=FACE_OUTER_BOUND('',#21031,.T.) ;
#16758=FACE_OUTER_BOUND('',#21032,.T.) ;
#16759=FACE_OUTER_BOUND('',#21033,.T.) ;
#16760=FACE_OUTER_BOUND('',#21034,.T.) ;
#16761=FACE_OUTER_BOUND('',#21035,.T.) ;
#16762=FACE_OUTER_BOUND('',#21036,.T.) ;
#16763=FACE_OUTER_BOUND('',#21037,.T.) ;
#16764=FACE_OUTER_BOUND('',#21038,.T.) ;
#16765=FACE_OUTER_BOUND('',#21039,.T.) ;
#16766=FACE_OUTER_BOUND('',#21040,.T.) ;
#16767=FACE_OUTER_BOUND('',#21041,.T.) ;
#16768=FACE_OUTER_BOUND('',#21042,.T.) ;
#16769=FACE_OUTER_BOUND('',#21043,.T.) ;
#16770=FACE_OUTER_BOUND('',#21044,.T.) ;
#16771=FACE_OUTER_BOUND('',#21045,.T.) ;
#16772=FACE_OUTER_BOUND('',#21046,.T.) ;
#16773=FACE_OUTER_BOUND('',#21047,.T.) ;
#16774=FACE_OUTER_BOUND('',#21048,.T.) ;
#16775=FACE_OUTER_BOUND('',#21049,.T.) ;
#16776=FACE_OUTER_BOUND('',#21050,.T.) ;
#16777=FACE_OUTER_BOUND('',#21051,.T.) ;
#16778=FACE_OUTER_BOUND('',#21052,.T.) ;
#16779=FACE_OUTER_BOUND('',#21053,.T.) ;
#16780=FACE_OUTER_BOUND('',#21054,.T.) ;
#16781=FACE_OUTER_BOUND('',#21055,.T.) ;
#16782=FACE_OUTER_BOUND('',#21056,.T.) ;
#16783=FACE_OUTER_BOUND('',#21057,.T.) ;
#16784=FACE_OUTER_BOUND('',#21058,.T.) ;
#16785=FACE_OUTER_BOUND('',#21059,.T.) ;
#16786=FACE_OUTER_BOUND('',#21060,.T.) ;
#16787=FACE_OUTER_BOUND('',#21061,.T.) ;
#16788=FACE_OUTER_BOUND('',#21062,.T.) ;
#16789=FACE_OUTER_BOUND('',#21063,.T.) ;
#16790=FACE_OUTER_BOUND('',#21064,.T.) ;
#16791=FACE_OUTER_BOUND('',#21065,.T.) ;
#16792=FACE_OUTER_BOUND('',#21066,.T.) ;
#16793=FACE_OUTER_BOUND('',#21067,.T.) ;
#16794=FACE_OUTER_BOUND('',#21068,.T.) ;
#16795=FACE_OUTER_BOUND('',#21069,.T.) ;
#16796=FACE_OUTER_BOUND('',#21070,.T.) ;
#16797=FACE_OUTER_BOUND('',#21071,.T.) ;
#16798=FACE_OUTER_BOUND('',#21072,.T.) ;
#16799=FACE_OUTER_BOUND('',#21073,.T.) ;
#16800=FACE_OUTER_BOUND('',#21074,.T.) ;
#16801=FACE_OUTER_BOUND('',#21075,.T.) ;
#16802=FACE_OUTER_BOUND('',#21076,.T.) ;
#16803=FACE_OUTER_BOUND('',#21077,.T.) ;
#16804=FACE_OUTER_BOUND('',#21078,.T.) ;
#16805=FACE_OUTER_BOUND('',#21079,.T.) ;
#16806=FACE_OUTER_BOUND('',#21080,.T.) ;
#16807=FACE_OUTER_BOUND('',#21081,.T.) ;
#16808=FACE_OUTER_BOUND('',#21082,.T.) ;
#16809=FACE_OUTER_BOUND('',#21083,.T.) ;
#16810=FACE_OUTER_BOUND('',#21084,.T.) ;
#16811=FACE_OUTER_BOUND('',#21085,.T.) ;
#16812=FACE_OUTER_BOUND('',#21086,.T.) ;
#16813=FACE_OUTER_BOUND('',#21087,.T.) ;
#16814=FACE_OUTER_BOUND('',#21088,.T.) ;
#16815=FACE_OUTER_BOUND('',#21089,.T.) ;
#16816=FACE_OUTER_BOUND('',#21090,.T.) ;
#16817=FACE_OUTER_BOUND('',#21091,.T.) ;
#16818=FACE_OUTER_BOUND('',#21092,.T.) ;
#16819=FACE_OUTER_BOUND('',#21093,.T.) ;
#16820=FACE_OUTER_BOUND('',#21094,.T.) ;
#16821=FACE_OUTER_BOUND('',#21095,.T.) ;
#16822=FACE_OUTER_BOUND('',#21096,.T.) ;
#16823=FACE_OUTER_BOUND('',#21097,.T.) ;
#16824=FACE_OUTER_BOUND('',#21098,.T.) ;
#16825=FACE_OUTER_BOUND('',#21099,.T.) ;
#16826=FACE_OUTER_BOUND('',#21100,.T.) ;
#16827=FACE_OUTER_BOUND('',#21101,.T.) ;
#16828=FACE_OUTER_BOUND('',#21102,.T.) ;
#16829=FACE_OUTER_BOUND('',#21103,.T.) ;
#16830=FACE_OUTER_BOUND('',#21104,.T.) ;
#16831=FACE_OUTER_BOUND('',#21105,.T.) ;
#16832=FACE_OUTER_BOUND('',#21106,.T.) ;
#16833=FACE_OUTER_BOUND('',#21107,.T.) ;
#16834=FACE_OUTER_BOUND('',#21108,.T.) ;
#16835=FACE_OUTER_BOUND('',#21109,.T.) ;
#16836=FACE_OUTER_BOUND('',#21110,.T.) ;
#16837=FACE_OUTER_BOUND('',#21111,.T.) ;
#16838=FACE_OUTER_BOUND('',#21112,.T.) ;
#16839=FACE_OUTER_BOUND('',#21113,.T.) ;
#16840=FACE_OUTER_BOUND('',#21114,.T.) ;
#16841=FACE_OUTER_BOUND('',#21115,.T.) ;
#16842=FACE_OUTER_BOUND('',#21116,.T.) ;
#16843=FACE_OUTER_BOUND('',#21117,.T.) ;
#16844=FACE_OUTER_BOUND('',#21118,.T.) ;
#16845=FACE_OUTER_BOUND('',#21119,.T.) ;
#16846=FACE_OUTER_BOUND('',#21120,.T.) ;
#16847=FACE_OUTER_BOUND('',#21121,.T.) ;
#16848=FACE_OUTER_BOUND('',#21122,.T.) ;
#16849=FACE_OUTER_BOUND('',#21123,.T.) ;
#16850=FACE_OUTER_BOUND('',#21124,.T.) ;
#16851=FACE_OUTER_BOUND('',#21125,.T.) ;
#16852=FACE_OUTER_BOUND('',#21126,.T.) ;
#16853=FACE_OUTER_BOUND('',#21127,.T.) ;
#16854=FACE_OUTER_BOUND('',#21128,.T.) ;
#16855=FACE_OUTER_BOUND('',#21129,.T.) ;
#16856=FACE_OUTER_BOUND('',#21130,.T.) ;
#16857=FACE_OUTER_BOUND('',#21131,.T.) ;
#16858=FACE_OUTER_BOUND('',#21132,.T.) ;
#16859=FACE_OUTER_BOUND('',#21133,.T.) ;
#16860=FACE_OUTER_BOUND('',#21134,.T.) ;
#16861=FACE_OUTER_BOUND('',#21135,.T.) ;
#16862=FACE_OUTER_BOUND('',#21136,.T.) ;
#16863=FACE_OUTER_BOUND('',#21137,.T.) ;
#16864=FACE_OUTER_BOUND('',#21138,.T.) ;
#16865=FACE_OUTER_BOUND('',#21139,.T.) ;
#16866=FACE_OUTER_BOUND('',#21140,.T.) ;
#16867=FACE_OUTER_BOUND('',#21141,.T.) ;
#16868=FACE_OUTER_BOUND('',#21142,.T.) ;
#16869=FACE_OUTER_BOUND('',#21143,.T.) ;
#16870=FACE_OUTER_BOUND('',#21144,.T.) ;
#16871=FACE_OUTER_BOUND('',#21145,.T.) ;
#16872=FACE_OUTER_BOUND('',#21146,.T.) ;
#16873=FACE_OUTER_BOUND('',#21147,.T.) ;
#16874=FACE_OUTER_BOUND('',#21148,.T.) ;
#16875=FACE_OUTER_BOUND('',#21149,.T.) ;
#16876=FACE_OUTER_BOUND('',#21150,.T.) ;
#16877=FACE_OUTER_BOUND('',#21151,.T.) ;
#16878=FACE_OUTER_BOUND('',#21152,.T.) ;
#16879=FACE_OUTER_BOUND('',#21153,.T.) ;
#16880=FACE_OUTER_BOUND('',#21154,.T.) ;
#16881=FACE_OUTER_BOUND('',#21155,.T.) ;
#16882=FACE_OUTER_BOUND('',#21156,.T.) ;
#16883=FACE_OUTER_BOUND('',#21157,.T.) ;
#16884=FACE_OUTER_BOUND('',#21158,.T.) ;
#16885=FACE_OUTER_BOUND('',#21159,.T.) ;
#16886=FACE_OUTER_BOUND('',#21160,.T.) ;
#16887=FACE_OUTER_BOUND('',#21161,.T.) ;
#16888=FACE_OUTER_BOUND('',#21162,.T.) ;
#16889=FACE_OUTER_BOUND('',#21163,.T.) ;
#16890=FACE_OUTER_BOUND('',#21164,.T.) ;
#16891=FACE_OUTER_BOUND('',#21165,.T.) ;
#16892=FACE_OUTER_BOUND('',#21166,.T.) ;
#16893=FACE_OUTER_BOUND('',#21167,.T.) ;
#16894=FACE_OUTER_BOUND('',#21168,.T.) ;
#16895=FACE_OUTER_BOUND('',#21169,.T.) ;
#16896=FACE_OUTER_BOUND('',#21170,.T.) ;
#16897=FACE_OUTER_BOUND('',#21171,.T.) ;
#16898=FACE_OUTER_BOUND('',#21172,.T.) ;
#16899=FACE_OUTER_BOUND('',#21173,.T.) ;
#16900=FACE_OUTER_BOUND('',#21174,.T.) ;
#16901=FACE_OUTER_BOUND('',#21175,.T.) ;
#16902=FACE_OUTER_BOUND('',#21176,.T.) ;
#16903=FACE_OUTER_BOUND('',#21177,.T.) ;
#16904=FACE_OUTER_BOUND('',#21178,.T.) ;
#16905=FACE_OUTER_BOUND('',#21179,.T.) ;
#16906=FACE_OUTER_BOUND('',#21180,.T.) ;
#16907=FACE_OUTER_BOUND('',#21181,.T.) ;
#16908=FACE_OUTER_BOUND('',#21182,.T.) ;
#16909=FACE_OUTER_BOUND('',#21183,.T.) ;
#16910=FACE_OUTER_BOUND('',#21184,.T.) ;
#16911=FACE_OUTER_BOUND('',#21185,.T.) ;
#16912=FACE_OUTER_BOUND('',#21186,.T.) ;
#16913=FACE_OUTER_BOUND('',#21187,.T.) ;
#16914=FACE_OUTER_BOUND('',#21188,.T.) ;
#16915=FACE_OUTER_BOUND('',#21189,.T.) ;
#16916=FACE_OUTER_BOUND('',#21190,.T.) ;
#16917=FACE_OUTER_BOUND('',#21191,.T.) ;
#16918=FACE_OUTER_BOUND('',#21192,.T.) ;
#16919=FACE_OUTER_BOUND('',#21193,.T.) ;
#16920=FACE_OUTER_BOUND('',#21194,.T.) ;
#16921=FACE_OUTER_BOUND('',#21195,.T.) ;
#16922=FACE_OUTER_BOUND('',#21196,.T.) ;
#16923=FACE_OUTER_BOUND('',#21197,.T.) ;
#16924=FACE_OUTER_BOUND('',#21198,.T.) ;
#16925=FACE_OUTER_BOUND('',#21200,.T.) ;
#16926=FACE_OUTER_BOUND('',#21201,.T.) ;
#16927=FACE_OUTER_BOUND('',#21202,.T.) ;
#16928=FACE_OUTER_BOUND('',#21203,.T.) ;
#16929=FACE_OUTER_BOUND('',#21204,.T.) ;
#16930=FACE_OUTER_BOUND('',#21205,.T.) ;
#16931=FACE_OUTER_BOUND('',#21206,.T.) ;
#16932=FACE_OUTER_BOUND('',#21207,.T.) ;
#16933=FACE_OUTER_BOUND('',#21208,.T.) ;
#16934=FACE_OUTER_BOUND('',#21209,.T.) ;
#16935=FACE_OUTER_BOUND('',#21210,.T.) ;
#16936=FACE_OUTER_BOUND('',#21212,.T.) ;
#16937=FACE_OUTER_BOUND('',#21213,.T.) ;
#16938=FACE_OUTER_BOUND('',#21214,.T.) ;
#16939=FACE_OUTER_BOUND('',#21215,.T.) ;
#16940=FACE_OUTER_BOUND('',#21216,.T.) ;
#16941=FACE_OUTER_BOUND('',#21217,.T.) ;
#16942=FACE_OUTER_BOUND('',#21218,.T.) ;
#16943=FACE_OUTER_BOUND('',#21219,.T.) ;
#16944=FACE_OUTER_BOUND('',#21220,.T.) ;
#16945=FACE_OUTER_BOUND('',#21221,.T.) ;
#16946=FACE_OUTER_BOUND('',#21222,.T.) ;
#16947=FACE_OUTER_BOUND('',#21223,.T.) ;
#16948=FACE_OUTER_BOUND('',#21224,.T.) ;
#16949=FACE_OUTER_BOUND('',#21225,.T.) ;
#16950=FACE_OUTER_BOUND('',#21226,.T.) ;
#16951=FACE_OUTER_BOUND('',#21227,.T.) ;
#16952=FACE_OUTER_BOUND('',#21228,.T.) ;
#16953=FACE_OUTER_BOUND('',#21229,.T.) ;
#16954=FACE_OUTER_BOUND('',#21230,.T.) ;
#16955=FACE_OUTER_BOUND('',#21231,.T.) ;
#16956=FACE_OUTER_BOUND('',#21232,.T.) ;
#16957=FACE_OUTER_BOUND('',#21233,.T.) ;
#16958=FACE_OUTER_BOUND('',#21234,.T.) ;
#16959=FACE_OUTER_BOUND('',#21235,.T.) ;
#16960=FACE_OUTER_BOUND('',#21236,.T.) ;
#16961=FACE_OUTER_BOUND('',#21237,.T.) ;
#16962=FACE_OUTER_BOUND('',#21238,.T.) ;
#16963=FACE_OUTER_BOUND('',#21239,.T.) ;
#16964=FACE_OUTER_BOUND('',#21240,.T.) ;
#16965=FACE_OUTER_BOUND('',#21241,.T.) ;
#16966=FACE_OUTER_BOUND('',#21242,.T.) ;
#16967=FACE_OUTER_BOUND('',#21243,.T.) ;
#16968=FACE_OUTER_BOUND('',#21244,.T.) ;
#16969=FACE_OUTER_BOUND('',#21245,.T.) ;
#16970=FACE_OUTER_BOUND('',#21246,.T.) ;
#16971=FACE_OUTER_BOUND('',#21247,.T.) ;
#16972=FACE_OUTER_BOUND('',#21248,.T.) ;
#16973=FACE_OUTER_BOUND('',#21249,.T.) ;
#16974=FACE_OUTER_BOUND('',#21250,.T.) ;
#16975=FACE_OUTER_BOUND('',#21251,.T.) ;
#16976=FACE_OUTER_BOUND('',#21252,.T.) ;
#16977=FACE_OUTER_BOUND('',#21253,.T.) ;
#16978=FACE_OUTER_BOUND('',#21254,.T.) ;
#16979=FACE_OUTER_BOUND('',#21255,.T.) ;
#16980=FACE_OUTER_BOUND('',#21256,.T.) ;
#16981=FACE_OUTER_BOUND('',#21257,.T.) ;
#16982=FACE_OUTER_BOUND('',#21258,.T.) ;
#16983=FACE_OUTER_BOUND('',#21259,.T.) ;
#16984=FACE_OUTER_BOUND('',#21260,.T.) ;
#16985=FACE_OUTER_BOUND('',#21261,.T.) ;
#16986=FACE_OUTER_BOUND('',#21262,.T.) ;
#16987=FACE_OUTER_BOUND('',#21263,.T.) ;
#16988=FACE_OUTER_BOUND('',#21264,.T.) ;
#16989=FACE_OUTER_BOUND('',#21265,.T.) ;
#16990=FACE_OUTER_BOUND('',#21266,.T.) ;
#16991=FACE_OUTER_BOUND('',#21267,.T.) ;
#16992=FACE_OUTER_BOUND('',#21268,.T.) ;
#16993=FACE_OUTER_BOUND('',#21269,.T.) ;
#16994=FACE_OUTER_BOUND('',#21270,.T.) ;
#16995=FACE_OUTER_BOUND('',#21271,.T.) ;
#16996=FACE_OUTER_BOUND('',#21272,.T.) ;
#16997=FACE_OUTER_BOUND('',#21273,.T.) ;
#16998=FACE_OUTER_BOUND('',#21274,.T.) ;
#16999=FACE_OUTER_BOUND('',#21275,.T.) ;
#17000=FACE_OUTER_BOUND('',#21276,.T.) ;
#17001=FACE_OUTER_BOUND('',#21277,.T.) ;
#17002=FACE_OUTER_BOUND('',#21278,.T.) ;
#17003=FACE_OUTER_BOUND('',#21279,.T.) ;
#17004=FACE_OUTER_BOUND('',#21280,.T.) ;
#17005=FACE_OUTER_BOUND('',#21281,.T.) ;
#17006=FACE_OUTER_BOUND('',#21282,.T.) ;
#17007=FACE_OUTER_BOUND('',#21283,.T.) ;
#17008=FACE_OUTER_BOUND('',#21284,.T.) ;
#17009=FACE_OUTER_BOUND('',#21285,.T.) ;
#17010=FACE_OUTER_BOUND('',#21286,.T.) ;
#17011=FACE_OUTER_BOUND('',#21287,.T.) ;
#17012=FACE_OUTER_BOUND('',#21288,.T.) ;
#17013=FACE_OUTER_BOUND('',#21289,.T.) ;
#17014=FACE_OUTER_BOUND('',#21290,.T.) ;
#17015=FACE_OUTER_BOUND('',#21291,.T.) ;
#17016=FACE_OUTER_BOUND('',#21292,.T.) ;
#17017=FACE_OUTER_BOUND('',#21293,.T.) ;
#17018=FACE_OUTER_BOUND('',#21294,.T.) ;
#17019=FACE_OUTER_BOUND('',#21295,.T.) ;
#17020=FACE_OUTER_BOUND('',#21296,.T.) ;
#17021=FACE_OUTER_BOUND('',#21297,.T.) ;
#17022=FACE_OUTER_BOUND('',#21298,.T.) ;
#17023=FACE_OUTER_BOUND('',#21299,.T.) ;
#17024=FACE_OUTER_BOUND('',#21300,.T.) ;
#17025=FACE_OUTER_BOUND('',#21301,.T.) ;
#17026=FACE_OUTER_BOUND('',#21302,.T.) ;
#17027=FACE_OUTER_BOUND('',#21303,.T.) ;
#17028=FACE_OUTER_BOUND('',#21304,.T.) ;
#17029=FACE_OUTER_BOUND('',#21305,.T.) ;
#17030=FACE_OUTER_BOUND('',#21306,.T.) ;
#17031=FACE_OUTER_BOUND('',#21307,.T.) ;
#17032=FACE_OUTER_BOUND('',#21308,.T.) ;
#17033=FACE_OUTER_BOUND('',#21309,.T.) ;
#17034=FACE_OUTER_BOUND('',#21310,.T.) ;
#17035=FACE_OUTER_BOUND('',#21311,.T.) ;
#17036=FACE_OUTER_BOUND('',#21312,.T.) ;
#17037=FACE_OUTER_BOUND('',#21313,.T.) ;
#17038=FACE_OUTER_BOUND('',#21314,.T.) ;
#17039=FACE_OUTER_BOUND('',#21315,.T.) ;
#17040=FACE_OUTER_BOUND('',#21316,.T.) ;
#17041=FACE_OUTER_BOUND('',#21317,.T.) ;
#17042=FACE_OUTER_BOUND('',#21318,.T.) ;
#17043=FACE_OUTER_BOUND('',#21319,.T.) ;
#17044=FACE_OUTER_BOUND('',#21320,.T.) ;
#17045=FACE_OUTER_BOUND('',#21321,.T.) ;
#17046=FACE_OUTER_BOUND('',#21322,.T.) ;
#17047=FACE_OUTER_BOUND('',#21323,.T.) ;
#17048=FACE_OUTER_BOUND('',#21324,.T.) ;
#17049=FACE_OUTER_BOUND('',#21325,.T.) ;
#17050=FACE_OUTER_BOUND('',#21326,.T.) ;
#17051=FACE_OUTER_BOUND('',#21327,.T.) ;
#17052=FACE_OUTER_BOUND('',#21328,.T.) ;
#17053=FACE_OUTER_BOUND('',#21329,.T.) ;
#17054=FACE_OUTER_BOUND('',#21330,.T.) ;
#17055=FACE_OUTER_BOUND('',#21331,.T.) ;
#17056=FACE_OUTER_BOUND('',#21332,.T.) ;
#17057=FACE_OUTER_BOUND('',#21333,.T.) ;
#17058=FACE_OUTER_BOUND('',#21334,.T.) ;
#17059=FACE_OUTER_BOUND('',#21335,.T.) ;
#17060=FACE_OUTER_BOUND('',#21336,.T.) ;
#17061=FACE_OUTER_BOUND('',#21337,.T.) ;
#17062=FACE_OUTER_BOUND('',#21338,.T.) ;
#17063=FACE_OUTER_BOUND('',#21339,.T.) ;
#17064=FACE_OUTER_BOUND('',#21340,.T.) ;
#17065=FACE_OUTER_BOUND('',#21341,.T.) ;
#17066=FACE_OUTER_BOUND('',#21342,.T.) ;
#17067=FACE_OUTER_BOUND('',#21343,.T.) ;
#17068=FACE_OUTER_BOUND('',#21344,.T.) ;
#17069=FACE_OUTER_BOUND('',#21345,.T.) ;
#17070=FACE_OUTER_BOUND('',#21346,.T.) ;
#17071=FACE_OUTER_BOUND('',#21347,.T.) ;
#17072=FACE_OUTER_BOUND('',#21348,.T.) ;
#17073=FACE_OUTER_BOUND('',#21349,.T.) ;
#17074=FACE_OUTER_BOUND('',#21350,.T.) ;
#17075=FACE_OUTER_BOUND('',#21351,.T.) ;
#17076=FACE_OUTER_BOUND('',#21352,.T.) ;
#17077=FACE_OUTER_BOUND('',#21353,.T.) ;
#17078=FACE_OUTER_BOUND('',#21354,.T.) ;
#17079=FACE_OUTER_BOUND('',#21355,.T.) ;
#17080=FACE_OUTER_BOUND('',#21356,.T.) ;
#17081=FACE_OUTER_BOUND('',#21357,.T.) ;
#17082=FACE_OUTER_BOUND('',#21358,.T.) ;
#17083=FACE_OUTER_BOUND('',#21359,.T.) ;
#17084=FACE_OUTER_BOUND('',#21360,.T.) ;
#17085=FACE_OUTER_BOUND('',#21361,.T.) ;
#17086=FACE_OUTER_BOUND('',#21362,.T.) ;
#17087=FACE_OUTER_BOUND('',#21363,.T.) ;
#17088=FACE_OUTER_BOUND('',#21364,.T.) ;
#17089=FACE_OUTER_BOUND('',#21365,.T.) ;
#17090=FACE_OUTER_BOUND('',#21366,.T.) ;
#17091=FACE_OUTER_BOUND('',#21367,.T.) ;
#17092=FACE_OUTER_BOUND('',#21368,.T.) ;
#17093=FACE_OUTER_BOUND('',#21369,.T.) ;
#17094=FACE_OUTER_BOUND('',#21370,.T.) ;
#17095=FACE_OUTER_BOUND('',#21371,.T.) ;
#17096=FACE_OUTER_BOUND('',#21372,.T.) ;
#17097=FACE_OUTER_BOUND('',#21373,.T.) ;
#17098=FACE_OUTER_BOUND('',#21374,.T.) ;
#17099=FACE_OUTER_BOUND('',#21375,.T.) ;
#17100=FACE_OUTER_BOUND('',#21376,.T.) ;
#17101=FACE_OUTER_BOUND('',#21377,.T.) ;
#17102=FACE_OUTER_BOUND('',#21378,.T.) ;
#17103=FACE_OUTER_BOUND('',#21379,.T.) ;
#17104=FACE_OUTER_BOUND('',#21380,.T.) ;
#17105=FACE_OUTER_BOUND('',#21381,.T.) ;
#17106=FACE_OUTER_BOUND('',#21382,.T.) ;
#17107=FACE_OUTER_BOUND('',#21383,.T.) ;
#17108=FACE_OUTER_BOUND('',#21384,.T.) ;
#17109=FACE_OUTER_BOUND('',#21385,.T.) ;
#17110=FACE_OUTER_BOUND('',#21386,.T.) ;
#17111=FACE_OUTER_BOUND('',#21387,.T.) ;
#17112=FACE_OUTER_BOUND('',#21388,.T.) ;
#17113=FACE_OUTER_BOUND('',#21389,.T.) ;
#17114=FACE_OUTER_BOUND('',#21390,.T.) ;
#17115=FACE_OUTER_BOUND('',#21391,.T.) ;
#17116=FACE_OUTER_BOUND('',#21392,.T.) ;
#17117=FACE_OUTER_BOUND('',#21393,.T.) ;
#17118=FACE_OUTER_BOUND('',#21394,.T.) ;
#17119=FACE_OUTER_BOUND('',#21395,.T.) ;
#17120=FACE_OUTER_BOUND('',#21396,.T.) ;
#17121=FACE_OUTER_BOUND('',#21397,.T.) ;
#17122=FACE_OUTER_BOUND('',#21398,.T.) ;
#17123=FACE_OUTER_BOUND('',#21399,.T.) ;
#17124=FACE_OUTER_BOUND('',#21400,.T.) ;
#17125=FACE_OUTER_BOUND('',#21401,.T.) ;
#17126=FACE_OUTER_BOUND('',#21402,.T.) ;
#17127=FACE_OUTER_BOUND('',#21403,.T.) ;
#17128=FACE_OUTER_BOUND('',#21404,.T.) ;
#17129=FACE_OUTER_BOUND('',#21405,.T.) ;
#17130=FACE_OUTER_BOUND('',#21406,.T.) ;
#17131=FACE_OUTER_BOUND('',#21407,.T.) ;
#17132=FACE_OUTER_BOUND('',#21408,.T.) ;
#17133=FACE_OUTER_BOUND('',#21409,.T.) ;
#17134=FACE_OUTER_BOUND('',#21410,.T.) ;
#17135=FACE_OUTER_BOUND('',#21411,.T.) ;
#17136=FACE_OUTER_BOUND('',#21412,.T.) ;
#17137=FACE_OUTER_BOUND('',#21413,.T.) ;
#17138=FACE_OUTER_BOUND('',#21414,.T.) ;
#17139=FACE_OUTER_BOUND('',#21415,.T.) ;
#17140=FACE_OUTER_BOUND('',#21416,.T.) ;
#17141=FACE_OUTER_BOUND('',#21417,.T.) ;
#17142=FACE_OUTER_BOUND('',#21418,.T.) ;
#17143=FACE_OUTER_BOUND('',#21419,.T.) ;
#17144=FACE_OUTER_BOUND('',#21420,.T.) ;
#17145=FACE_OUTER_BOUND('',#21421,.T.) ;
#17146=FACE_OUTER_BOUND('',#21422,.T.) ;
#17147=FACE_OUTER_BOUND('',#21423,.T.) ;
#17148=FACE_OUTER_BOUND('',#21424,.T.) ;
#17149=FACE_OUTER_BOUND('',#21425,.T.) ;
#17150=FACE_OUTER_BOUND('',#21426,.T.) ;
#17151=FACE_OUTER_BOUND('',#21427,.T.) ;
#17152=FACE_OUTER_BOUND('',#21428,.T.) ;
#17153=FACE_OUTER_BOUND('',#21429,.T.) ;
#17154=FACE_OUTER_BOUND('',#21430,.T.) ;
#17155=FACE_OUTER_BOUND('',#21431,.T.) ;
#17156=FACE_OUTER_BOUND('',#21432,.T.) ;
#17157=FACE_OUTER_BOUND('',#21433,.T.) ;
#17158=FACE_OUTER_BOUND('',#21434,.T.) ;
#17159=FACE_OUTER_BOUND('',#21435,.T.) ;
#17160=FACE_OUTER_BOUND('',#21436,.T.) ;
#17161=FACE_OUTER_BOUND('',#21437,.T.) ;
#17162=FACE_OUTER_BOUND('',#21438,.T.) ;
#17163=FACE_OUTER_BOUND('',#21439,.T.) ;
#17164=FACE_OUTER_BOUND('',#21440,.T.) ;
#17165=FACE_OUTER_BOUND('',#21441,.T.) ;
#17166=FACE_OUTER_BOUND('',#21442,.T.) ;
#17167=FACE_OUTER_BOUND('',#21443,.T.) ;
#17168=FACE_OUTER_BOUND('',#21444,.T.) ;
#17169=FACE_OUTER_BOUND('',#21445,.T.) ;
#17170=FACE_OUTER_BOUND('',#21446,.T.) ;
#17171=FACE_OUTER_BOUND('',#21447,.T.) ;
#17172=FACE_OUTER_BOUND('',#21448,.T.) ;
#17173=FACE_OUTER_BOUND('',#21449,.T.) ;
#17174=FACE_OUTER_BOUND('',#21450,.T.) ;
#17175=FACE_OUTER_BOUND('',#21451,.T.) ;
#17176=FACE_OUTER_BOUND('',#21452,.T.) ;
#17177=FACE_OUTER_BOUND('',#21453,.T.) ;
#17178=FACE_OUTER_BOUND('',#21454,.T.) ;
#17179=FACE_OUTER_BOUND('',#21455,.T.) ;
#17180=FACE_OUTER_BOUND('',#21456,.T.) ;
#17181=FACE_OUTER_BOUND('',#21457,.T.) ;
#17182=FACE_OUTER_BOUND('',#21458,.T.) ;
#17183=FACE_OUTER_BOUND('',#21459,.T.) ;
#17184=FACE_OUTER_BOUND('',#21460,.T.) ;
#17185=FACE_OUTER_BOUND('',#21461,.T.) ;
#17186=FACE_OUTER_BOUND('',#21462,.T.) ;
#17187=FACE_OUTER_BOUND('',#21463,.T.) ;
#17188=FACE_OUTER_BOUND('',#21464,.T.) ;
#17189=FACE_OUTER_BOUND('',#21465,.T.) ;
#17190=FACE_OUTER_BOUND('',#21466,.T.) ;
#17191=FACE_OUTER_BOUND('',#21467,.T.) ;
#17192=FACE_OUTER_BOUND('',#21468,.T.) ;
#17193=FACE_OUTER_BOUND('',#21469,.T.) ;
#17194=FACE_OUTER_BOUND('',#21470,.T.) ;
#17195=FACE_OUTER_BOUND('',#21471,.T.) ;
#17196=FACE_OUTER_BOUND('',#21472,.T.) ;
#17197=FACE_OUTER_BOUND('',#21473,.T.) ;
#17198=FACE_OUTER_BOUND('',#21474,.T.) ;
#17199=FACE_OUTER_BOUND('',#21475,.T.) ;
#17200=FACE_OUTER_BOUND('',#21476,.T.) ;
#17201=FACE_OUTER_BOUND('',#21477,.T.) ;
#17202=FACE_OUTER_BOUND('',#21478,.T.) ;
#17203=FACE_OUTER_BOUND('',#21479,.T.) ;
#17204=FACE_OUTER_BOUND('',#21480,.T.) ;
#17205=FACE_OUTER_BOUND('',#21481,.T.) ;
#17206=FACE_OUTER_BOUND('',#21482,.T.) ;
#17207=FACE_OUTER_BOUND('',#21483,.T.) ;
#17208=FACE_OUTER_BOUND('',#21484,.T.) ;
#17209=FACE_OUTER_BOUND('',#21485,.T.) ;
#17210=FACE_OUTER_BOUND('',#21486,.T.) ;
#17211=FACE_OUTER_BOUND('',#21487,.T.) ;
#17212=FACE_OUTER_BOUND('',#21488,.T.) ;
#17213=FACE_OUTER_BOUND('',#21489,.T.) ;
#17214=FACE_OUTER_BOUND('',#21491,.T.) ;
#17215=FACE_OUTER_BOUND('',#21492,.T.) ;
#17216=FACE_OUTER_BOUND('',#21493,.T.) ;
#17217=FACE_OUTER_BOUND('',#21494,.T.) ;
#17218=FACE_OUTER_BOUND('',#21495,.T.) ;
#17219=FACE_OUTER_BOUND('',#21496,.T.) ;
#17220=FACE_OUTER_BOUND('',#21497,.T.) ;
#17221=FACE_OUTER_BOUND('',#21498,.T.) ;
#17222=FACE_OUTER_BOUND('',#21499,.T.) ;
#17223=FACE_OUTER_BOUND('',#21500,.T.) ;
#17224=FACE_OUTER_BOUND('',#21501,.T.) ;
#17225=FACE_OUTER_BOUND('',#21503,.T.) ;
#17226=FACE_OUTER_BOUND('',#21504,.T.) ;
#17227=FACE_OUTER_BOUND('',#21505,.T.) ;
#17228=FACE_OUTER_BOUND('',#21506,.T.) ;
#17229=FACE_OUTER_BOUND('',#21507,.T.) ;
#17230=FACE_OUTER_BOUND('',#21508,.T.) ;
#17231=FACE_OUTER_BOUND('',#21509,.T.) ;
#17232=FACE_OUTER_BOUND('',#21510,.T.) ;
#17233=FACE_OUTER_BOUND('',#21511,.T.) ;
#17234=FACE_OUTER_BOUND('',#21512,.T.) ;
#17235=FACE_OUTER_BOUND('',#21513,.T.) ;
#17236=FACE_OUTER_BOUND('',#21514,.T.) ;
#17237=FACE_OUTER_BOUND('',#21515,.T.) ;
#17238=FACE_OUTER_BOUND('',#21516,.T.) ;
#17239=FACE_OUTER_BOUND('',#21517,.T.) ;
#17240=FACE_OUTER_BOUND('',#21518,.T.) ;
#17241=FACE_OUTER_BOUND('',#21519,.T.) ;
#17242=FACE_OUTER_BOUND('',#21520,.T.) ;
#17243=FACE_OUTER_BOUND('',#21521,.T.) ;
#17244=FACE_OUTER_BOUND('',#21522,.T.) ;
#17245=FACE_OUTER_BOUND('',#21523,.T.) ;
#17246=FACE_OUTER_BOUND('',#21524,.T.) ;
#17247=FACE_OUTER_BOUND('',#21525,.T.) ;
#17248=FACE_OUTER_BOUND('',#21526,.T.) ;
#17249=FACE_OUTER_BOUND('',#21527,.T.) ;
#17250=FACE_OUTER_BOUND('',#21528,.T.) ;
#17251=FACE_OUTER_BOUND('',#21529,.T.) ;
#17252=FACE_OUTER_BOUND('',#21530,.T.) ;
#17253=FACE_OUTER_BOUND('',#21531,.T.) ;
#17254=FACE_OUTER_BOUND('',#21532,.T.) ;
#17255=FACE_OUTER_BOUND('',#21533,.T.) ;
#17256=FACE_OUTER_BOUND('',#21534,.T.) ;
#17257=FACE_OUTER_BOUND('',#21535,.T.) ;
#17258=FACE_OUTER_BOUND('',#21536,.T.) ;
#17259=FACE_OUTER_BOUND('',#21537,.T.) ;
#17260=FACE_OUTER_BOUND('',#21538,.T.) ;
#17261=FACE_OUTER_BOUND('',#21539,.T.) ;
#17262=FACE_OUTER_BOUND('',#21540,.T.) ;
#17263=FACE_OUTER_BOUND('',#21541,.T.) ;
#17264=FACE_OUTER_BOUND('',#21542,.T.) ;
#17265=FACE_OUTER_BOUND('',#21543,.T.) ;
#17266=FACE_OUTER_BOUND('',#21544,.T.) ;
#17267=FACE_OUTER_BOUND('',#21545,.T.) ;
#17268=FACE_OUTER_BOUND('',#21546,.T.) ;
#17269=FACE_OUTER_BOUND('',#21547,.T.) ;
#17270=FACE_OUTER_BOUND('',#21548,.T.) ;
#17271=FACE_OUTER_BOUND('',#21549,.T.) ;
#17272=FACE_OUTER_BOUND('',#21550,.T.) ;
#17273=FACE_OUTER_BOUND('',#21551,.T.) ;
#17274=FACE_OUTER_BOUND('',#21552,.T.) ;
#17275=FACE_OUTER_BOUND('',#21553,.T.) ;
#17276=FACE_OUTER_BOUND('',#21554,.T.) ;
#17277=FACE_OUTER_BOUND('',#21555,.T.) ;
#17278=FACE_OUTER_BOUND('',#21556,.T.) ;
#17279=FACE_OUTER_BOUND('',#21557,.T.) ;
#17280=FACE_OUTER_BOUND('',#21558,.T.) ;
#17281=FACE_OUTER_BOUND('',#21559,.T.) ;
#17282=FACE_OUTER_BOUND('',#21560,.T.) ;
#17283=FACE_OUTER_BOUND('',#21561,.T.) ;
#17284=FACE_OUTER_BOUND('',#21562,.T.) ;
#17285=FACE_OUTER_BOUND('',#21563,.T.) ;
#17286=FACE_OUTER_BOUND('',#21564,.T.) ;
#17287=FACE_OUTER_BOUND('',#21565,.T.) ;
#17288=FACE_OUTER_BOUND('',#21566,.T.) ;
#17289=FACE_OUTER_BOUND('',#21567,.T.) ;
#17290=FACE_OUTER_BOUND('',#21568,.T.) ;
#17291=FACE_OUTER_BOUND('',#21569,.T.) ;
#17292=FACE_OUTER_BOUND('',#21570,.T.) ;
#17293=FACE_OUTER_BOUND('',#21571,.T.) ;
#17294=FACE_OUTER_BOUND('',#21572,.T.) ;
#17295=FACE_OUTER_BOUND('',#21573,.T.) ;
#17296=FACE_OUTER_BOUND('',#21574,.T.) ;
#17297=FACE_OUTER_BOUND('',#21575,.T.) ;
#17298=FACE_OUTER_BOUND('',#21576,.T.) ;
#17299=FACE_OUTER_BOUND('',#21577,.T.) ;
#17300=FACE_OUTER_BOUND('',#21578,.T.) ;
#17301=FACE_OUTER_BOUND('',#21579,.T.) ;
#17302=FACE_OUTER_BOUND('',#21580,.T.) ;
#17303=FACE_OUTER_BOUND('',#21581,.T.) ;
#17304=FACE_OUTER_BOUND('',#21582,.T.) ;
#17305=FACE_OUTER_BOUND('',#21583,.T.) ;
#17306=FACE_OUTER_BOUND('',#21584,.T.) ;
#17307=FACE_OUTER_BOUND('',#21585,.T.) ;
#17308=FACE_OUTER_BOUND('',#21586,.T.) ;
#17309=FACE_OUTER_BOUND('',#21587,.T.) ;
#17310=FACE_OUTER_BOUND('',#21588,.T.) ;
#17311=FACE_OUTER_BOUND('',#21589,.T.) ;
#17312=FACE_OUTER_BOUND('',#21590,.T.) ;
#17313=FACE_OUTER_BOUND('',#21591,.T.) ;
#17314=FACE_OUTER_BOUND('',#21592,.T.) ;
#17315=FACE_OUTER_BOUND('',#21593,.T.) ;
#17316=FACE_OUTER_BOUND('',#21594,.T.) ;
#17317=FACE_OUTER_BOUND('',#21595,.T.) ;
#17318=FACE_OUTER_BOUND('',#21596,.T.) ;
#17319=FACE_OUTER_BOUND('',#21597,.T.) ;
#17320=FACE_OUTER_BOUND('',#21598,.T.) ;
#17321=FACE_OUTER_BOUND('',#21599,.T.) ;
#17322=FACE_OUTER_BOUND('',#21600,.T.) ;
#17323=FACE_OUTER_BOUND('',#21601,.T.) ;
#17324=FACE_OUTER_BOUND('',#21602,.T.) ;
#17325=FACE_OUTER_BOUND('',#21603,.T.) ;
#17326=FACE_OUTER_BOUND('',#21604,.T.) ;
#17327=FACE_OUTER_BOUND('',#21605,.T.) ;
#17328=FACE_OUTER_BOUND('',#21606,.T.) ;
#17329=FACE_OUTER_BOUND('',#21607,.T.) ;
#17330=FACE_OUTER_BOUND('',#21608,.T.) ;
#17331=FACE_OUTER_BOUND('',#21609,.T.) ;
#17332=FACE_OUTER_BOUND('',#21610,.T.) ;
#17333=FACE_OUTER_BOUND('',#21611,.T.) ;
#17334=FACE_OUTER_BOUND('',#21612,.T.) ;
#17335=FACE_OUTER_BOUND('',#21613,.T.) ;
#17336=FACE_OUTER_BOUND('',#21614,.T.) ;
#17337=FACE_OUTER_BOUND('',#21615,.T.) ;
#17338=FACE_OUTER_BOUND('',#21616,.T.) ;
#17339=FACE_OUTER_BOUND('',#21617,.T.) ;
#17340=FACE_OUTER_BOUND('',#21618,.T.) ;
#17341=FACE_OUTER_BOUND('',#21619,.T.) ;
#17342=FACE_OUTER_BOUND('',#21620,.T.) ;
#17343=FACE_OUTER_BOUND('',#21621,.T.) ;
#17344=FACE_OUTER_BOUND('',#21622,.T.) ;
#17345=FACE_OUTER_BOUND('',#21623,.T.) ;
#17346=FACE_OUTER_BOUND('',#21624,.T.) ;
#17347=FACE_OUTER_BOUND('',#21625,.T.) ;
#17348=FACE_OUTER_BOUND('',#21626,.T.) ;
#17349=FACE_OUTER_BOUND('',#21627,.T.) ;
#17350=FACE_OUTER_BOUND('',#21628,.T.) ;
#17351=FACE_OUTER_BOUND('',#21629,.T.) ;
#17352=FACE_OUTER_BOUND('',#21630,.T.) ;
#17353=FACE_OUTER_BOUND('',#21631,.T.) ;
#17354=FACE_OUTER_BOUND('',#21632,.T.) ;
#17355=FACE_OUTER_BOUND('',#21633,.T.) ;
#17356=FACE_OUTER_BOUND('',#21634,.T.) ;
#17357=FACE_OUTER_BOUND('',#21635,.T.) ;
#17358=FACE_OUTER_BOUND('',#21636,.T.) ;
#17359=FACE_OUTER_BOUND('',#21637,.T.) ;
#17360=FACE_OUTER_BOUND('',#21638,.T.) ;
#17361=FACE_OUTER_BOUND('',#21639,.T.) ;
#17362=FACE_OUTER_BOUND('',#21640,.T.) ;
#17363=FACE_OUTER_BOUND('',#21641,.T.) ;
#17364=FACE_OUTER_BOUND('',#21642,.T.) ;
#17365=FACE_OUTER_BOUND('',#21643,.T.) ;
#17366=FACE_OUTER_BOUND('',#21644,.T.) ;
#17367=FACE_OUTER_BOUND('',#21645,.T.) ;
#17368=FACE_OUTER_BOUND('',#21646,.T.) ;
#17369=FACE_OUTER_BOUND('',#21647,.T.) ;
#17370=FACE_OUTER_BOUND('',#21648,.T.) ;
#17371=FACE_OUTER_BOUND('',#21649,.T.) ;
#17372=FACE_OUTER_BOUND('',#21650,.T.) ;
#17373=FACE_OUTER_BOUND('',#21651,.T.) ;
#17374=FACE_OUTER_BOUND('',#21652,.T.) ;
#17375=FACE_OUTER_BOUND('',#21653,.T.) ;
#17376=FACE_OUTER_BOUND('',#21654,.T.) ;
#17377=FACE_OUTER_BOUND('',#21655,.T.) ;
#17378=FACE_OUTER_BOUND('',#21656,.T.) ;
#17379=FACE_OUTER_BOUND('',#21657,.T.) ;
#17380=FACE_OUTER_BOUND('',#21658,.T.) ;
#17381=FACE_OUTER_BOUND('',#21659,.T.) ;
#17382=FACE_OUTER_BOUND('',#21660,.T.) ;
#17383=FACE_OUTER_BOUND('',#21661,.T.) ;
#17384=FACE_OUTER_BOUND('',#21662,.T.) ;
#17385=FACE_OUTER_BOUND('',#21663,.T.) ;
#17386=FACE_OUTER_BOUND('',#21664,.T.) ;
#17387=FACE_OUTER_BOUND('',#21665,.T.) ;
#17388=FACE_OUTER_BOUND('',#21666,.T.) ;
#17389=FACE_OUTER_BOUND('',#21667,.T.) ;
#17390=FACE_OUTER_BOUND('',#21668,.T.) ;
#17391=FACE_OUTER_BOUND('',#21669,.T.) ;
#17392=FACE_OUTER_BOUND('',#21670,.T.) ;
#17393=FACE_OUTER_BOUND('',#21671,.T.) ;
#17394=FACE_OUTER_BOUND('',#21672,.T.) ;
#17395=FACE_OUTER_BOUND('',#21673,.T.) ;
#17396=FACE_OUTER_BOUND('',#21674,.T.) ;
#17397=FACE_OUTER_BOUND('',#21675,.T.) ;
#17398=FACE_OUTER_BOUND('',#21676,.T.) ;
#17399=FACE_OUTER_BOUND('',#21677,.T.) ;
#17400=FACE_OUTER_BOUND('',#21678,.T.) ;
#17401=FACE_OUTER_BOUND('',#21679,.T.) ;
#17402=FACE_OUTER_BOUND('',#21680,.T.) ;
#17403=FACE_OUTER_BOUND('',#21681,.T.) ;
#17404=FACE_OUTER_BOUND('',#21682,.T.) ;
#17405=FACE_OUTER_BOUND('',#21683,.T.) ;
#17406=FACE_OUTER_BOUND('',#21684,.T.) ;
#17407=FACE_OUTER_BOUND('',#21685,.T.) ;
#17408=FACE_OUTER_BOUND('',#21686,.T.) ;
#17409=FACE_OUTER_BOUND('',#21687,.T.) ;
#17410=FACE_OUTER_BOUND('',#21688,.T.) ;
#17411=FACE_OUTER_BOUND('',#21689,.T.) ;
#17412=FACE_OUTER_BOUND('',#21690,.T.) ;
#17413=FACE_OUTER_BOUND('',#21691,.T.) ;
#17414=FACE_OUTER_BOUND('',#21692,.T.) ;
#17415=FACE_OUTER_BOUND('',#21693,.T.) ;
#17416=FACE_OUTER_BOUND('',#21694,.T.) ;
#17417=FACE_OUTER_BOUND('',#21695,.T.) ;
#17418=FACE_OUTER_BOUND('',#21696,.T.) ;
#17419=FACE_OUTER_BOUND('',#21697,.T.) ;
#17420=FACE_OUTER_BOUND('',#21698,.T.) ;
#17421=FACE_OUTER_BOUND('',#21699,.T.) ;
#17422=FACE_OUTER_BOUND('',#21700,.T.) ;
#17423=FACE_OUTER_BOUND('',#21701,.T.) ;
#17424=FACE_OUTER_BOUND('',#21702,.T.) ;
#17425=FACE_OUTER_BOUND('',#21703,.T.) ;
#17426=FACE_OUTER_BOUND('',#21704,.T.) ;
#17427=FACE_OUTER_BOUND('',#21705,.T.) ;
#17428=FACE_OUTER_BOUND('',#21706,.T.) ;
#17429=FACE_OUTER_BOUND('',#21707,.T.) ;
#17430=FACE_OUTER_BOUND('',#21708,.T.) ;
#17431=FACE_OUTER_BOUND('',#21709,.T.) ;
#17432=FACE_OUTER_BOUND('',#21710,.T.) ;
#17433=FACE_OUTER_BOUND('',#21711,.T.) ;
#17434=FACE_OUTER_BOUND('',#21712,.T.) ;
#17435=FACE_OUTER_BOUND('',#21713,.T.) ;
#17436=FACE_OUTER_BOUND('',#21714,.T.) ;
#17437=FACE_OUTER_BOUND('',#21715,.T.) ;
#17438=FACE_OUTER_BOUND('',#21716,.T.) ;
#17439=FACE_OUTER_BOUND('',#21717,.T.) ;
#17440=FACE_OUTER_BOUND('',#21718,.T.) ;
#17441=FACE_OUTER_BOUND('',#21719,.T.) ;
#17442=FACE_OUTER_BOUND('',#21720,.T.) ;
#17443=FACE_OUTER_BOUND('',#21721,.T.) ;
#17444=FACE_OUTER_BOUND('',#21722,.T.) ;
#17445=FACE_OUTER_BOUND('',#21723,.T.) ;
#17446=FACE_OUTER_BOUND('',#21724,.T.) ;
#17447=FACE_OUTER_BOUND('',#21725,.T.) ;
#17448=FACE_OUTER_BOUND('',#21726,.T.) ;
#17449=FACE_OUTER_BOUND('',#21727,.T.) ;
#17450=FACE_OUTER_BOUND('',#21728,.T.) ;
#17451=FACE_OUTER_BOUND('',#21729,.T.) ;
#17452=FACE_OUTER_BOUND('',#21730,.T.) ;
#17453=FACE_OUTER_BOUND('',#21731,.T.) ;
#17454=FACE_OUTER_BOUND('',#21732,.T.) ;
#17455=FACE_OUTER_BOUND('',#21733,.T.) ;
#17456=FACE_OUTER_BOUND('',#21734,.T.) ;
#17457=FACE_OUTER_BOUND('',#21735,.T.) ;
#17458=FACE_OUTER_BOUND('',#21736,.T.) ;
#17459=FACE_OUTER_BOUND('',#21737,.T.) ;
#17460=FACE_OUTER_BOUND('',#21738,.T.) ;
#17461=FACE_OUTER_BOUND('',#21739,.T.) ;
#17462=FACE_OUTER_BOUND('',#21740,.T.) ;
#17463=FACE_OUTER_BOUND('',#21741,.T.) ;
#17464=FACE_OUTER_BOUND('',#21742,.T.) ;
#17465=FACE_OUTER_BOUND('',#21743,.T.) ;
#17466=FACE_OUTER_BOUND('',#21744,.T.) ;
#17467=FACE_OUTER_BOUND('',#21745,.T.) ;
#17468=FACE_OUTER_BOUND('',#21746,.T.) ;
#17469=FACE_OUTER_BOUND('',#21747,.T.) ;
#17470=FACE_OUTER_BOUND('',#21748,.T.) ;
#17471=FACE_OUTER_BOUND('',#21749,.T.) ;
#17472=FACE_OUTER_BOUND('',#21750,.T.) ;
#17473=FACE_OUTER_BOUND('',#21751,.T.) ;
#17474=FACE_OUTER_BOUND('',#21752,.T.) ;
#17475=FACE_OUTER_BOUND('',#21753,.T.) ;
#17476=FACE_OUTER_BOUND('',#21754,.T.) ;
#17477=FACE_OUTER_BOUND('',#21755,.T.) ;
#17478=FACE_OUTER_BOUND('',#21756,.T.) ;
#17479=FACE_OUTER_BOUND('',#21757,.T.) ;
#17480=FACE_OUTER_BOUND('',#21758,.T.) ;
#17481=FACE_OUTER_BOUND('',#21759,.T.) ;
#17482=FACE_OUTER_BOUND('',#21760,.T.) ;
#17483=FACE_OUTER_BOUND('',#21761,.T.) ;
#17484=FACE_OUTER_BOUND('',#21762,.T.) ;
#17485=FACE_OUTER_BOUND('',#21763,.T.) ;
#17486=FACE_OUTER_BOUND('',#21764,.T.) ;
#17487=FACE_OUTER_BOUND('',#21765,.T.) ;
#17488=FACE_OUTER_BOUND('',#21766,.T.) ;
#17489=FACE_OUTER_BOUND('',#21767,.T.) ;
#17490=FACE_OUTER_BOUND('',#21768,.T.) ;
#17491=FACE_OUTER_BOUND('',#21769,.T.) ;
#17492=FACE_OUTER_BOUND('',#21770,.T.) ;
#17493=FACE_OUTER_BOUND('',#21771,.T.) ;
#17494=FACE_OUTER_BOUND('',#21772,.T.) ;
#17495=FACE_OUTER_BOUND('',#21773,.T.) ;
#17496=FACE_OUTER_BOUND('',#21774,.T.) ;
#17497=FACE_OUTER_BOUND('',#21775,.T.) ;
#17498=FACE_OUTER_BOUND('',#21776,.T.) ;
#17499=FACE_OUTER_BOUND('',#21777,.T.) ;
#17500=FACE_OUTER_BOUND('',#21778,.T.) ;
#17501=FACE_OUTER_BOUND('',#21779,.T.) ;
#17502=FACE_OUTER_BOUND('',#21780,.T.) ;
#17503=FACE_OUTER_BOUND('',#21782,.T.) ;
#17504=FACE_OUTER_BOUND('',#21783,.T.) ;
#17505=FACE_OUTER_BOUND('',#21784,.T.) ;
#17506=FACE_OUTER_BOUND('',#21785,.T.) ;
#17507=FACE_OUTER_BOUND('',#21786,.T.) ;
#17508=FACE_OUTER_BOUND('',#21787,.T.) ;
#17509=FACE_OUTER_BOUND('',#21788,.T.) ;
#17510=FACE_OUTER_BOUND('',#21789,.T.) ;
#17511=FACE_OUTER_BOUND('',#21790,.T.) ;
#17512=FACE_OUTER_BOUND('',#21791,.T.) ;
#17513=FACE_OUTER_BOUND('',#21792,.T.) ;
#17514=FACE_OUTER_BOUND('',#21794,.T.) ;
#17515=FACE_OUTER_BOUND('',#21795,.T.) ;
#17516=FACE_OUTER_BOUND('',#21796,.T.) ;
#17517=FACE_OUTER_BOUND('',#21797,.T.) ;
#17518=FACE_OUTER_BOUND('',#21798,.T.) ;
#17519=FACE_OUTER_BOUND('',#21799,.T.) ;
#17520=FACE_OUTER_BOUND('',#21800,.T.) ;
#17521=FACE_OUTER_BOUND('',#21801,.T.) ;
#17522=FACE_OUTER_BOUND('',#21802,.T.) ;
#17523=FACE_OUTER_BOUND('',#21803,.T.) ;
#17524=FACE_OUTER_BOUND('',#21804,.T.) ;
#17525=FACE_OUTER_BOUND('',#21805,.T.) ;
#17526=FACE_OUTER_BOUND('',#21806,.T.) ;
#17527=FACE_OUTER_BOUND('',#21807,.T.) ;
#17528=FACE_OUTER_BOUND('',#21808,.T.) ;
#17529=FACE_OUTER_BOUND('',#21809,.T.) ;
#17530=FACE_OUTER_BOUND('',#21810,.T.) ;
#17531=FACE_OUTER_BOUND('',#21811,.T.) ;
#17532=FACE_OUTER_BOUND('',#21812,.T.) ;
#17533=FACE_OUTER_BOUND('',#21813,.T.) ;
#17534=FACE_OUTER_BOUND('',#21814,.T.) ;
#17535=FACE_OUTER_BOUND('',#21815,.T.) ;
#17536=FACE_OUTER_BOUND('',#21816,.T.) ;
#17537=FACE_OUTER_BOUND('',#21817,.T.) ;
#17538=FACE_OUTER_BOUND('',#21818,.T.) ;
#17539=FACE_OUTER_BOUND('',#21819,.T.) ;
#17540=FACE_OUTER_BOUND('',#21820,.T.) ;
#17541=FACE_OUTER_BOUND('',#21821,.T.) ;
#17542=FACE_OUTER_BOUND('',#21822,.T.) ;
#17543=FACE_OUTER_BOUND('',#21823,.T.) ;
#17544=FACE_OUTER_BOUND('',#21824,.T.) ;
#17545=FACE_OUTER_BOUND('',#21825,.T.) ;
#17546=FACE_OUTER_BOUND('',#21826,.T.) ;
#17547=FACE_OUTER_BOUND('',#21827,.T.) ;
#17548=FACE_OUTER_BOUND('',#21828,.T.) ;
#17549=FACE_OUTER_BOUND('',#21829,.T.) ;
#17550=FACE_OUTER_BOUND('',#21830,.T.) ;
#17551=FACE_OUTER_BOUND('',#21831,.T.) ;
#17552=FACE_OUTER_BOUND('',#21832,.T.) ;
#17553=FACE_OUTER_BOUND('',#21833,.T.) ;
#17554=FACE_OUTER_BOUND('',#21834,.T.) ;
#17555=FACE_OUTER_BOUND('',#21835,.T.) ;
#17556=FACE_OUTER_BOUND('',#21836,.T.) ;
#17557=FACE_OUTER_BOUND('',#21837,.T.) ;
#17558=FACE_OUTER_BOUND('',#21838,.T.) ;
#17559=FACE_OUTER_BOUND('',#21839,.T.) ;
#17560=FACE_OUTER_BOUND('',#21840,.T.) ;
#17561=FACE_OUTER_BOUND('',#21841,.T.) ;
#17562=FACE_OUTER_BOUND('',#21842,.T.) ;
#17563=FACE_OUTER_BOUND('',#21843,.T.) ;
#17564=FACE_OUTER_BOUND('',#21844,.T.) ;
#17565=FACE_OUTER_BOUND('',#21845,.T.) ;
#17566=FACE_OUTER_BOUND('',#21846,.T.) ;
#17567=FACE_OUTER_BOUND('',#21847,.T.) ;
#17568=FACE_OUTER_BOUND('',#21848,.T.) ;
#17569=FACE_OUTER_BOUND('',#21849,.T.) ;
#17570=FACE_OUTER_BOUND('',#21850,.T.) ;
#17571=FACE_OUTER_BOUND('',#21851,.T.) ;
#17572=FACE_OUTER_BOUND('',#21852,.T.) ;
#17573=FACE_OUTER_BOUND('',#21853,.T.) ;
#17574=FACE_OUTER_BOUND('',#21854,.T.) ;
#17575=FACE_OUTER_BOUND('',#21855,.T.) ;
#17576=FACE_OUTER_BOUND('',#21856,.T.) ;
#17577=FACE_OUTER_BOUND('',#21857,.T.) ;
#17578=FACE_OUTER_BOUND('',#21858,.T.) ;
#17579=FACE_OUTER_BOUND('',#21859,.T.) ;
#17580=FACE_OUTER_BOUND('',#21860,.T.) ;
#17581=FACE_OUTER_BOUND('',#21861,.T.) ;
#17582=FACE_OUTER_BOUND('',#21862,.T.) ;
#17583=FACE_OUTER_BOUND('',#21863,.T.) ;
#17584=FACE_OUTER_BOUND('',#21864,.T.) ;
#17585=FACE_OUTER_BOUND('',#21865,.T.) ;
#17586=FACE_OUTER_BOUND('',#21866,.T.) ;
#17587=FACE_OUTER_BOUND('',#21867,.T.) ;
#17588=FACE_OUTER_BOUND('',#21868,.T.) ;
#17589=FACE_OUTER_BOUND('',#21869,.T.) ;
#17590=FACE_OUTER_BOUND('',#21870,.T.) ;
#17591=FACE_OUTER_BOUND('',#21871,.T.) ;
#17592=FACE_OUTER_BOUND('',#21872,.T.) ;
#17593=FACE_OUTER_BOUND('',#21873,.T.) ;
#17594=FACE_OUTER_BOUND('',#21874,.T.) ;
#17595=FACE_OUTER_BOUND('',#21875,.T.) ;
#17596=FACE_OUTER_BOUND('',#21876,.T.) ;
#17597=FACE_OUTER_BOUND('',#21877,.T.) ;
#17598=FACE_OUTER_BOUND('',#21878,.T.) ;
#17599=FACE_OUTER_BOUND('',#21879,.T.) ;
#17600=FACE_OUTER_BOUND('',#21880,.T.) ;
#17601=FACE_OUTER_BOUND('',#21881,.T.) ;
#17602=FACE_OUTER_BOUND('',#21882,.T.) ;
#17603=FACE_OUTER_BOUND('',#21883,.T.) ;
#17604=FACE_OUTER_BOUND('',#21884,.T.) ;
#17605=FACE_OUTER_BOUND('',#21885,.T.) ;
#17606=FACE_OUTER_BOUND('',#21886,.T.) ;
#17607=FACE_OUTER_BOUND('',#21887,.T.) ;
#17608=FACE_OUTER_BOUND('',#21888,.T.) ;
#17609=FACE_OUTER_BOUND('',#21889,.T.) ;
#17610=FACE_OUTER_BOUND('',#21890,.T.) ;
#17611=FACE_OUTER_BOUND('',#21891,.T.) ;
#17612=FACE_OUTER_BOUND('',#21892,.T.) ;
#17613=FACE_OUTER_BOUND('',#21893,.T.) ;
#17614=FACE_OUTER_BOUND('',#21894,.T.) ;
#17615=FACE_OUTER_BOUND('',#21895,.T.) ;
#17616=FACE_OUTER_BOUND('',#21896,.T.) ;
#17617=FACE_OUTER_BOUND('',#21897,.T.) ;
#17618=FACE_OUTER_BOUND('',#21898,.T.) ;
#17619=FACE_OUTER_BOUND('',#21899,.T.) ;
#17620=FACE_OUTER_BOUND('',#21900,.T.) ;
#17621=FACE_OUTER_BOUND('',#21901,.T.) ;
#17622=FACE_OUTER_BOUND('',#21902,.T.) ;
#17623=FACE_OUTER_BOUND('',#21903,.T.) ;
#17624=FACE_OUTER_BOUND('',#21904,.T.) ;
#17625=FACE_OUTER_BOUND('',#21905,.T.) ;
#17626=FACE_OUTER_BOUND('',#21906,.T.) ;
#17627=FACE_OUTER_BOUND('',#21907,.T.) ;
#17628=FACE_OUTER_BOUND('',#21908,.T.) ;
#17629=FACE_OUTER_BOUND('',#21909,.T.) ;
#17630=FACE_OUTER_BOUND('',#21910,.T.) ;
#17631=FACE_OUTER_BOUND('',#21911,.T.) ;
#17632=FACE_OUTER_BOUND('',#21912,.T.) ;
#17633=FACE_OUTER_BOUND('',#21913,.T.) ;
#17634=FACE_OUTER_BOUND('',#21914,.T.) ;
#17635=FACE_OUTER_BOUND('',#21915,.T.) ;
#17636=FACE_OUTER_BOUND('',#21916,.T.) ;
#17637=FACE_OUTER_BOUND('',#21917,.T.) ;
#17638=FACE_OUTER_BOUND('',#21918,.T.) ;
#17639=FACE_OUTER_BOUND('',#21919,.T.) ;
#17640=FACE_OUTER_BOUND('',#21920,.T.) ;
#17641=FACE_OUTER_BOUND('',#21921,.T.) ;
#17642=FACE_OUTER_BOUND('',#21922,.T.) ;
#17643=FACE_OUTER_BOUND('',#21923,.T.) ;
#17644=FACE_OUTER_BOUND('',#21924,.T.) ;
#17645=FACE_OUTER_BOUND('',#21925,.T.) ;
#17646=FACE_OUTER_BOUND('',#21926,.T.) ;
#17647=FACE_OUTER_BOUND('',#21927,.T.) ;
#17648=FACE_OUTER_BOUND('',#21928,.T.) ;
#17649=FACE_OUTER_BOUND('',#21929,.T.) ;
#17650=FACE_OUTER_BOUND('',#21930,.T.) ;
#17651=FACE_OUTER_BOUND('',#21931,.T.) ;
#17652=FACE_OUTER_BOUND('',#21932,.T.) ;
#17653=FACE_OUTER_BOUND('',#21933,.T.) ;
#17654=FACE_OUTER_BOUND('',#21934,.T.) ;
#17655=FACE_OUTER_BOUND('',#21935,.T.) ;
#17656=FACE_OUTER_BOUND('',#21936,.T.) ;
#17657=FACE_OUTER_BOUND('',#21937,.T.) ;
#17658=FACE_OUTER_BOUND('',#21938,.T.) ;
#17659=FACE_OUTER_BOUND('',#21939,.T.) ;
#17660=FACE_OUTER_BOUND('',#21940,.T.) ;
#17661=FACE_OUTER_BOUND('',#21941,.T.) ;
#17662=FACE_OUTER_BOUND('',#21942,.T.) ;
#17663=FACE_OUTER_BOUND('',#21943,.T.) ;
#17664=FACE_OUTER_BOUND('',#21944,.T.) ;
#17665=FACE_OUTER_BOUND('',#21945,.T.) ;
#17666=FACE_OUTER_BOUND('',#21946,.T.) ;
#17667=FACE_OUTER_BOUND('',#21947,.T.) ;
#17668=FACE_OUTER_BOUND('',#21948,.T.) ;
#17669=FACE_OUTER_BOUND('',#21949,.T.) ;
#17670=FACE_OUTER_BOUND('',#21950,.T.) ;
#17671=FACE_OUTER_BOUND('',#21951,.T.) ;
#17672=FACE_OUTER_BOUND('',#21952,.T.) ;
#17673=FACE_OUTER_BOUND('',#21953,.T.) ;
#17674=FACE_OUTER_BOUND('',#21954,.T.) ;
#17675=FACE_OUTER_BOUND('',#21955,.T.) ;
#17676=FACE_OUTER_BOUND('',#21956,.T.) ;
#17677=FACE_OUTER_BOUND('',#21957,.T.) ;
#17678=FACE_OUTER_BOUND('',#21958,.T.) ;
#17679=FACE_OUTER_BOUND('',#21959,.T.) ;
#17680=FACE_OUTER_BOUND('',#21960,.T.) ;
#17681=FACE_OUTER_BOUND('',#21961,.T.) ;
#17682=FACE_OUTER_BOUND('',#21962,.T.) ;
#17683=FACE_OUTER_BOUND('',#21963,.T.) ;
#17684=FACE_OUTER_BOUND('',#21964,.T.) ;
#17685=FACE_OUTER_BOUND('',#21965,.T.) ;
#17686=FACE_OUTER_BOUND('',#21966,.T.) ;
#17687=FACE_OUTER_BOUND('',#21967,.T.) ;
#17688=FACE_OUTER_BOUND('',#21968,.T.) ;
#17689=FACE_OUTER_BOUND('',#21969,.T.) ;
#17690=FACE_OUTER_BOUND('',#21970,.T.) ;
#17691=FACE_OUTER_BOUND('',#21971,.T.) ;
#17692=FACE_OUTER_BOUND('',#21972,.T.) ;
#17693=FACE_OUTER_BOUND('',#21973,.T.) ;
#17694=FACE_OUTER_BOUND('',#21974,.T.) ;
#17695=FACE_OUTER_BOUND('',#21975,.T.) ;
#17696=FACE_OUTER_BOUND('',#21976,.T.) ;
#17697=FACE_OUTER_BOUND('',#21977,.T.) ;
#17698=FACE_OUTER_BOUND('',#21978,.T.) ;
#17699=FACE_OUTER_BOUND('',#21979,.T.) ;
#17700=FACE_OUTER_BOUND('',#21980,.T.) ;
#17701=FACE_OUTER_BOUND('',#21981,.T.) ;
#17702=FACE_OUTER_BOUND('',#21982,.T.) ;
#17703=FACE_OUTER_BOUND('',#21983,.T.) ;
#17704=FACE_OUTER_BOUND('',#21984,.T.) ;
#17705=FACE_OUTER_BOUND('',#21985,.T.) ;
#17706=FACE_OUTER_BOUND('',#21986,.T.) ;
#17707=FACE_OUTER_BOUND('',#21987,.T.) ;
#17708=FACE_OUTER_BOUND('',#21988,.T.) ;
#17709=FACE_OUTER_BOUND('',#21989,.T.) ;
#17710=FACE_OUTER_BOUND('',#21990,.T.) ;
#17711=FACE_OUTER_BOUND('',#21991,.T.) ;
#17712=FACE_OUTER_BOUND('',#21992,.T.) ;
#17713=FACE_OUTER_BOUND('',#21993,.T.) ;
#17714=FACE_OUTER_BOUND('',#21994,.T.) ;
#17715=FACE_OUTER_BOUND('',#21995,.T.) ;
#17716=FACE_OUTER_BOUND('',#21996,.T.) ;
#17717=FACE_OUTER_BOUND('',#21997,.T.) ;
#17718=FACE_OUTER_BOUND('',#21998,.T.) ;
#17719=FACE_OUTER_BOUND('',#21999,.T.) ;
#17720=FACE_OUTER_BOUND('',#22000,.T.) ;
#17721=FACE_OUTER_BOUND('',#22001,.T.) ;
#17722=FACE_OUTER_BOUND('',#22002,.T.) ;
#17723=FACE_OUTER_BOUND('',#22003,.T.) ;
#17724=FACE_OUTER_BOUND('',#22004,.T.) ;
#17725=FACE_OUTER_BOUND('',#22005,.T.) ;
#17726=FACE_OUTER_BOUND('',#22006,.T.) ;
#17727=FACE_OUTER_BOUND('',#22007,.T.) ;
#17728=FACE_OUTER_BOUND('',#22008,.T.) ;
#17729=FACE_OUTER_BOUND('',#22009,.T.) ;
#17730=FACE_OUTER_BOUND('',#22010,.T.) ;
#17731=FACE_OUTER_BOUND('',#22011,.T.) ;
#17732=FACE_OUTER_BOUND('',#22012,.T.) ;
#17733=FACE_OUTER_BOUND('',#22013,.T.) ;
#17734=FACE_OUTER_BOUND('',#22014,.T.) ;
#17735=FACE_OUTER_BOUND('',#22015,.T.) ;
#17736=FACE_OUTER_BOUND('',#22016,.T.) ;
#17737=FACE_OUTER_BOUND('',#22017,.T.) ;
#17738=FACE_OUTER_BOUND('',#22018,.T.) ;
#17739=FACE_OUTER_BOUND('',#22019,.T.) ;
#17740=FACE_OUTER_BOUND('',#22020,.T.) ;
#17741=FACE_OUTER_BOUND('',#22021,.T.) ;
#17742=FACE_OUTER_BOUND('',#22022,.T.) ;
#17743=FACE_OUTER_BOUND('',#22023,.T.) ;
#17744=FACE_OUTER_BOUND('',#22024,.T.) ;
#17745=FACE_OUTER_BOUND('',#22025,.T.) ;
#17746=FACE_OUTER_BOUND('',#22026,.T.) ;
#17747=FACE_OUTER_BOUND('',#22027,.T.) ;
#17748=FACE_OUTER_BOUND('',#22028,.T.) ;
#17749=FACE_OUTER_BOUND('',#22029,.T.) ;
#17750=FACE_OUTER_BOUND('',#22030,.T.) ;
#17751=FACE_OUTER_BOUND('',#22031,.T.) ;
#17752=FACE_OUTER_BOUND('',#22032,.T.) ;
#17753=FACE_OUTER_BOUND('',#22033,.T.) ;
#17754=FACE_OUTER_BOUND('',#22034,.T.) ;
#17755=FACE_OUTER_BOUND('',#22035,.T.) ;
#17756=FACE_OUTER_BOUND('',#22036,.T.) ;
#17757=FACE_OUTER_BOUND('',#22037,.T.) ;
#17758=FACE_OUTER_BOUND('',#22038,.T.) ;
#17759=FACE_OUTER_BOUND('',#22039,.T.) ;
#17760=FACE_OUTER_BOUND('',#22040,.T.) ;
#17761=FACE_OUTER_BOUND('',#22041,.T.) ;
#17762=FACE_OUTER_BOUND('',#22042,.T.) ;
#17763=FACE_OUTER_BOUND('',#22043,.T.) ;
#17764=FACE_OUTER_BOUND('',#22044,.T.) ;
#17765=FACE_OUTER_BOUND('',#22045,.T.) ;
#17766=FACE_OUTER_BOUND('',#22046,.T.) ;
#17767=FACE_OUTER_BOUND('',#22047,.T.) ;
#17768=FACE_OUTER_BOUND('',#22048,.T.) ;
#17769=FACE_OUTER_BOUND('',#22049,.T.) ;
#17770=FACE_OUTER_BOUND('',#22050,.T.) ;
#17771=FACE_OUTER_BOUND('',#22051,.T.) ;
#17772=FACE_OUTER_BOUND('',#22052,.T.) ;
#17773=FACE_OUTER_BOUND('',#22053,.T.) ;
#17774=FACE_OUTER_BOUND('',#22054,.T.) ;
#17775=FACE_OUTER_BOUND('',#22055,.T.) ;
#17776=FACE_OUTER_BOUND('',#22056,.T.) ;
#17777=FACE_OUTER_BOUND('',#22057,.T.) ;
#17778=FACE_OUTER_BOUND('',#22058,.T.) ;
#17779=FACE_OUTER_BOUND('',#22059,.T.) ;
#17780=FACE_OUTER_BOUND('',#22060,.T.) ;
#17781=FACE_OUTER_BOUND('',#22061,.T.) ;
#17782=FACE_OUTER_BOUND('',#22062,.T.) ;
#17783=FACE_OUTER_BOUND('',#22063,.T.) ;
#17784=FACE_OUTER_BOUND('',#22064,.T.) ;
#17785=FACE_OUTER_BOUND('',#22065,.T.) ;
#17786=FACE_OUTER_BOUND('',#22066,.T.) ;
#17787=FACE_OUTER_BOUND('',#22067,.T.) ;
#17788=FACE_OUTER_BOUND('',#22068,.T.) ;
#17789=FACE_OUTER_BOUND('',#22069,.T.) ;
#17790=FACE_OUTER_BOUND('',#22070,.T.) ;
#17791=FACE_OUTER_BOUND('',#22071,.T.) ;
#17792=FACE_OUTER_BOUND('',#22073,.T.) ;
#17793=FACE_OUTER_BOUND('',#22074,.T.) ;
#17794=FACE_OUTER_BOUND('',#22075,.T.) ;
#17795=FACE_OUTER_BOUND('',#22076,.T.) ;
#17796=FACE_OUTER_BOUND('',#22077,.T.) ;
#17797=FACE_OUTER_BOUND('',#22078,.T.) ;
#17798=FACE_OUTER_BOUND('',#22079,.T.) ;
#17799=FACE_OUTER_BOUND('',#22080,.T.) ;
#17800=FACE_OUTER_BOUND('',#22081,.T.) ;
#17801=FACE_OUTER_BOUND('',#22082,.T.) ;
#17802=FACE_OUTER_BOUND('',#22083,.T.) ;
#17803=FACE_OUTER_BOUND('',#22085,.T.) ;
#17804=FACE_OUTER_BOUND('',#22086,.T.) ;
#17805=FACE_OUTER_BOUND('',#22087,.T.) ;
#17806=FACE_OUTER_BOUND('',#22088,.T.) ;
#17807=FACE_OUTER_BOUND('',#22089,.T.) ;
#17808=FACE_OUTER_BOUND('',#22090,.T.) ;
#17809=FACE_OUTER_BOUND('',#22091,.T.) ;
#17810=FACE_OUTER_BOUND('',#22092,.T.) ;
#17811=FACE_OUTER_BOUND('',#22093,.T.) ;
#17812=FACE_OUTER_BOUND('',#22094,.T.) ;
#17813=FACE_OUTER_BOUND('',#22095,.T.) ;
#17814=FACE_OUTER_BOUND('',#22096,.T.) ;
#17815=FACE_OUTER_BOUND('',#22097,.T.) ;
#17816=FACE_OUTER_BOUND('',#22098,.T.) ;
#17817=FACE_OUTER_BOUND('',#22099,.T.) ;
#17818=FACE_OUTER_BOUND('',#22100,.T.) ;
#17819=FACE_OUTER_BOUND('',#22101,.T.) ;
#17820=FACE_OUTER_BOUND('',#22102,.T.) ;
#17821=FACE_OUTER_BOUND('',#22103,.T.) ;
#17822=FACE_OUTER_BOUND('',#22104,.T.) ;
#17823=FACE_OUTER_BOUND('',#22105,.T.) ;
#17824=FACE_OUTER_BOUND('',#22106,.T.) ;
#17825=FACE_OUTER_BOUND('',#22107,.T.) ;
#17826=FACE_OUTER_BOUND('',#22108,.T.) ;
#17827=FACE_OUTER_BOUND('',#22109,.T.) ;
#17828=FACE_OUTER_BOUND('',#22110,.T.) ;
#17829=FACE_OUTER_BOUND('',#22111,.T.) ;
#17830=FACE_OUTER_BOUND('',#22112,.T.) ;
#17831=FACE_OUTER_BOUND('',#22113,.T.) ;
#17832=FACE_OUTER_BOUND('',#22114,.T.) ;
#17833=FACE_OUTER_BOUND('',#22115,.T.) ;
#17834=FACE_OUTER_BOUND('',#22116,.T.) ;
#17835=FACE_OUTER_BOUND('',#22117,.T.) ;
#17836=FACE_OUTER_BOUND('',#22118,.T.) ;
#17837=FACE_OUTER_BOUND('',#22119,.T.) ;
#17838=FACE_OUTER_BOUND('',#22120,.T.) ;
#17839=FACE_OUTER_BOUND('',#22121,.T.) ;
#17840=FACE_OUTER_BOUND('',#22122,.T.) ;
#17841=FACE_OUTER_BOUND('',#22123,.T.) ;
#17842=FACE_OUTER_BOUND('',#22124,.T.) ;
#17843=FACE_OUTER_BOUND('',#22125,.T.) ;
#17844=FACE_OUTER_BOUND('',#22126,.T.) ;
#17845=FACE_OUTER_BOUND('',#22127,.T.) ;
#17846=FACE_OUTER_BOUND('',#22128,.T.) ;
#17847=FACE_OUTER_BOUND('',#22129,.T.) ;
#17848=FACE_OUTER_BOUND('',#22130,.T.) ;
#17849=FACE_OUTER_BOUND('',#22131,.T.) ;
#17850=FACE_OUTER_BOUND('',#22132,.T.) ;
#17851=FACE_OUTER_BOUND('',#22133,.T.) ;
#17852=FACE_OUTER_BOUND('',#22134,.T.) ;
#17853=FACE_OUTER_BOUND('',#22135,.T.) ;
#17854=FACE_OUTER_BOUND('',#22136,.T.) ;
#17855=FACE_OUTER_BOUND('',#22137,.T.) ;
#17856=FACE_OUTER_BOUND('',#22138,.T.) ;
#17857=FACE_OUTER_BOUND('',#22139,.T.) ;
#17858=FACE_OUTER_BOUND('',#22140,.T.) ;
#17859=FACE_OUTER_BOUND('',#22141,.T.) ;
#17860=FACE_OUTER_BOUND('',#22142,.T.) ;
#17861=FACE_OUTER_BOUND('',#22143,.T.) ;
#17862=FACE_OUTER_BOUND('',#22144,.T.) ;
#17863=FACE_OUTER_BOUND('',#22145,.T.) ;
#17864=FACE_OUTER_BOUND('',#22146,.T.) ;
#17865=FACE_OUTER_BOUND('',#22147,.T.) ;
#17866=FACE_OUTER_BOUND('',#22148,.T.) ;
#17867=FACE_OUTER_BOUND('',#22149,.T.) ;
#17868=FACE_OUTER_BOUND('',#22150,.T.) ;
#17869=FACE_OUTER_BOUND('',#22151,.T.) ;
#17870=FACE_OUTER_BOUND('',#22152,.T.) ;
#17871=FACE_OUTER_BOUND('',#22153,.T.) ;
#17872=FACE_OUTER_BOUND('',#22154,.T.) ;
#17873=FACE_OUTER_BOUND('',#22155,.T.) ;
#17874=FACE_OUTER_BOUND('',#22156,.T.) ;
#17875=FACE_OUTER_BOUND('',#22157,.T.) ;
#17876=FACE_OUTER_BOUND('',#22158,.T.) ;
#17877=FACE_OUTER_BOUND('',#22159,.T.) ;
#17878=FACE_OUTER_BOUND('',#22160,.T.) ;
#17879=FACE_OUTER_BOUND('',#22161,.T.) ;
#17880=FACE_OUTER_BOUND('',#22162,.T.) ;
#17881=FACE_OUTER_BOUND('',#22163,.T.) ;
#17882=FACE_OUTER_BOUND('',#22164,.T.) ;
#17883=FACE_OUTER_BOUND('',#22165,.T.) ;
#17884=FACE_OUTER_BOUND('',#22166,.T.) ;
#17885=FACE_OUTER_BOUND('',#22167,.T.) ;
#17886=FACE_OUTER_BOUND('',#22168,.T.) ;
#17887=FACE_OUTER_BOUND('',#22169,.T.) ;
#17888=FACE_OUTER_BOUND('',#22170,.T.) ;
#17889=FACE_OUTER_BOUND('',#22171,.T.) ;
#17890=FACE_OUTER_BOUND('',#22172,.T.) ;
#17891=FACE_OUTER_BOUND('',#22173,.T.) ;
#17892=FACE_OUTER_BOUND('',#22174,.T.) ;
#17893=FACE_OUTER_BOUND('',#22175,.T.) ;
#17894=FACE_OUTER_BOUND('',#22176,.T.) ;
#17895=FACE_OUTER_BOUND('',#22177,.T.) ;
#17896=FACE_OUTER_BOUND('',#22178,.T.) ;
#17897=FACE_OUTER_BOUND('',#22179,.T.) ;
#17898=FACE_OUTER_BOUND('',#22180,.T.) ;
#17899=FACE_OUTER_BOUND('',#22181,.T.) ;
#17900=FACE_OUTER_BOUND('',#22182,.T.) ;
#17901=FACE_OUTER_BOUND('',#22183,.T.) ;
#17902=FACE_OUTER_BOUND('',#22184,.T.) ;
#17903=FACE_OUTER_BOUND('',#22185,.T.) ;
#17904=FACE_OUTER_BOUND('',#22186,.T.) ;
#17905=FACE_OUTER_BOUND('',#22187,.T.) ;
#17906=FACE_OUTER_BOUND('',#22188,.T.) ;
#17907=FACE_OUTER_BOUND('',#22189,.T.) ;
#17908=FACE_OUTER_BOUND('',#22190,.T.) ;
#17909=FACE_OUTER_BOUND('',#22191,.T.) ;
#17910=FACE_OUTER_BOUND('',#22192,.T.) ;
#17911=FACE_OUTER_BOUND('',#22193,.T.) ;
#17912=FACE_OUTER_BOUND('',#22194,.T.) ;
#17913=FACE_OUTER_BOUND('',#22195,.T.) ;
#17914=FACE_OUTER_BOUND('',#22196,.T.) ;
#17915=FACE_OUTER_BOUND('',#22197,.T.) ;
#17916=FACE_OUTER_BOUND('',#22198,.T.) ;
#17917=FACE_OUTER_BOUND('',#22199,.T.) ;
#17918=FACE_OUTER_BOUND('',#22200,.T.) ;
#17919=FACE_OUTER_BOUND('',#22201,.T.) ;
#17920=FACE_OUTER_BOUND('',#22202,.T.) ;
#17921=FACE_OUTER_BOUND('',#22203,.T.) ;
#17922=FACE_OUTER_BOUND('',#22204,.T.) ;
#17923=FACE_OUTER_BOUND('',#22205,.T.) ;
#17924=FACE_OUTER_BOUND('',#22206,.T.) ;
#17925=FACE_OUTER_BOUND('',#22207,.T.) ;
#17926=FACE_OUTER_BOUND('',#22208,.T.) ;
#17927=FACE_OUTER_BOUND('',#22209,.T.) ;
#17928=FACE_OUTER_BOUND('',#22210,.T.) ;
#17929=FACE_OUTER_BOUND('',#22211,.T.) ;
#17930=FACE_OUTER_BOUND('',#22212,.T.) ;
#17931=FACE_OUTER_BOUND('',#22213,.T.) ;
#17932=FACE_OUTER_BOUND('',#22214,.T.) ;
#17933=FACE_OUTER_BOUND('',#22215,.T.) ;
#17934=FACE_OUTER_BOUND('',#22216,.T.) ;
#17935=FACE_OUTER_BOUND('',#22217,.T.) ;
#17936=FACE_OUTER_BOUND('',#22218,.T.) ;
#17937=FACE_OUTER_BOUND('',#22219,.T.) ;
#17938=FACE_OUTER_BOUND('',#22220,.T.) ;
#17939=FACE_OUTER_BOUND('',#22221,.T.) ;
#17940=FACE_OUTER_BOUND('',#22222,.T.) ;
#17941=FACE_OUTER_BOUND('',#22223,.T.) ;
#17942=FACE_OUTER_BOUND('',#22224,.T.) ;
#17943=FACE_OUTER_BOUND('',#22225,.T.) ;
#17944=FACE_OUTER_BOUND('',#22226,.T.) ;
#17945=FACE_OUTER_BOUND('',#22227,.T.) ;
#17946=FACE_OUTER_BOUND('',#22228,.T.) ;
#17947=FACE_OUTER_BOUND('',#22229,.T.) ;
#17948=FACE_OUTER_BOUND('',#22230,.T.) ;
#17949=FACE_OUTER_BOUND('',#22231,.T.) ;
#17950=FACE_OUTER_BOUND('',#22232,.T.) ;
#17951=FACE_OUTER_BOUND('',#22233,.T.) ;
#17952=FACE_OUTER_BOUND('',#22234,.T.) ;
#17953=FACE_OUTER_BOUND('',#22235,.T.) ;
#17954=FACE_OUTER_BOUND('',#22236,.T.) ;
#17955=FACE_OUTER_BOUND('',#22237,.T.) ;
#17956=FACE_OUTER_BOUND('',#22238,.T.) ;
#17957=FACE_OUTER_BOUND('',#22239,.T.) ;
#17958=FACE_OUTER_BOUND('',#22240,.T.) ;
#17959=FACE_OUTER_BOUND('',#22241,.T.) ;
#17960=FACE_OUTER_BOUND('',#22242,.T.) ;
#17961=FACE_OUTER_BOUND('',#22243,.T.) ;
#17962=FACE_OUTER_BOUND('',#22244,.T.) ;
#17963=FACE_OUTER_BOUND('',#22245,.T.) ;
#17964=FACE_OUTER_BOUND('',#22246,.T.) ;
#17965=FACE_OUTER_BOUND('',#22247,.T.) ;
#17966=FACE_OUTER_BOUND('',#22248,.T.) ;
#17967=FACE_OUTER_BOUND('',#22249,.T.) ;
#17968=FACE_OUTER_BOUND('',#22250,.T.) ;
#17969=FACE_OUTER_BOUND('',#22251,.T.) ;
#17970=FACE_OUTER_BOUND('',#22252,.T.) ;
#17971=FACE_OUTER_BOUND('',#22253,.T.) ;
#17972=FACE_OUTER_BOUND('',#22254,.T.) ;
#17973=FACE_OUTER_BOUND('',#22255,.T.) ;
#17974=FACE_OUTER_BOUND('',#22256,.T.) ;
#17975=FACE_OUTER_BOUND('',#22257,.T.) ;
#17976=FACE_OUTER_BOUND('',#22258,.T.) ;
#17977=FACE_OUTER_BOUND('',#22259,.T.) ;
#17978=FACE_OUTER_BOUND('',#22260,.T.) ;
#17979=FACE_OUTER_BOUND('',#22261,.T.) ;
#17980=FACE_OUTER_BOUND('',#22262,.T.) ;
#17981=FACE_OUTER_BOUND('',#22263,.T.) ;
#17982=FACE_OUTER_BOUND('',#22264,.T.) ;
#17983=FACE_OUTER_BOUND('',#22265,.T.) ;
#17984=FACE_OUTER_BOUND('',#22266,.T.) ;
#17985=FACE_OUTER_BOUND('',#22267,.T.) ;
#17986=FACE_OUTER_BOUND('',#22268,.T.) ;
#17987=FACE_OUTER_BOUND('',#22269,.T.) ;
#17988=FACE_OUTER_BOUND('',#22270,.T.) ;
#17989=FACE_OUTER_BOUND('',#22271,.T.) ;
#17990=FACE_OUTER_BOUND('',#22272,.T.) ;
#17991=FACE_OUTER_BOUND('',#22273,.T.) ;
#17992=FACE_OUTER_BOUND('',#22274,.T.) ;
#17993=FACE_OUTER_BOUND('',#22275,.T.) ;
#17994=FACE_OUTER_BOUND('',#22276,.T.) ;
#17995=FACE_OUTER_BOUND('',#22277,.T.) ;
#17996=FACE_OUTER_BOUND('',#22278,.T.) ;
#17997=FACE_OUTER_BOUND('',#22279,.T.) ;
#17998=FACE_OUTER_BOUND('',#22280,.T.) ;
#17999=FACE_OUTER_BOUND('',#22281,.T.) ;
#18000=FACE_OUTER_BOUND('',#22282,.T.) ;
#18001=FACE_OUTER_BOUND('',#22283,.T.) ;
#18002=FACE_OUTER_BOUND('',#22284,.T.) ;
#18003=FACE_OUTER_BOUND('',#22285,.T.) ;
#18004=FACE_OUTER_BOUND('',#22286,.T.) ;
#18005=FACE_OUTER_BOUND('',#22287,.T.) ;
#18006=FACE_OUTER_BOUND('',#22288,.T.) ;
#18007=FACE_OUTER_BOUND('',#22289,.T.) ;
#18008=FACE_OUTER_BOUND('',#22290,.T.) ;
#18009=FACE_OUTER_BOUND('',#22291,.T.) ;
#18010=FACE_OUTER_BOUND('',#22292,.T.) ;
#18011=FACE_OUTER_BOUND('',#22293,.T.) ;
#18012=FACE_OUTER_BOUND('',#22294,.T.) ;
#18013=FACE_OUTER_BOUND('',#22295,.T.) ;
#18014=FACE_OUTER_BOUND('',#22296,.T.) ;
#18015=FACE_OUTER_BOUND('',#22297,.T.) ;
#18016=FACE_OUTER_BOUND('',#22298,.T.) ;
#18017=FACE_OUTER_BOUND('',#22299,.T.) ;
#18018=FACE_OUTER_BOUND('',#22300,.T.) ;
#18019=FACE_OUTER_BOUND('',#22301,.T.) ;
#18020=FACE_OUTER_BOUND('',#22302,.T.) ;
#18021=FACE_OUTER_BOUND('',#22303,.T.) ;
#18022=FACE_OUTER_BOUND('',#22304,.T.) ;
#18023=FACE_OUTER_BOUND('',#22305,.T.) ;
#18024=FACE_OUTER_BOUND('',#22306,.T.) ;
#18025=FACE_OUTER_BOUND('',#22307,.T.) ;
#18026=FACE_OUTER_BOUND('',#22308,.T.) ;
#18027=FACE_OUTER_BOUND('',#22309,.T.) ;
#18028=FACE_OUTER_BOUND('',#22310,.T.) ;
#18029=FACE_OUTER_BOUND('',#22311,.T.) ;
#18030=FACE_OUTER_BOUND('',#22312,.T.) ;
#18031=FACE_OUTER_BOUND('',#22313,.T.) ;
#18032=FACE_OUTER_BOUND('',#22314,.T.) ;
#18033=FACE_OUTER_BOUND('',#22315,.T.) ;
#18034=FACE_OUTER_BOUND('',#22316,.T.) ;
#18035=FACE_OUTER_BOUND('',#22317,.T.) ;
#18036=FACE_OUTER_BOUND('',#22318,.T.) ;
#18037=FACE_OUTER_BOUND('',#22319,.T.) ;
#18038=FACE_OUTER_BOUND('',#22320,.T.) ;
#18039=FACE_OUTER_BOUND('',#22321,.T.) ;
#18040=FACE_OUTER_BOUND('',#22322,.T.) ;
#18041=FACE_OUTER_BOUND('',#22323,.T.) ;
#18042=FACE_OUTER_BOUND('',#22324,.T.) ;
#18043=FACE_OUTER_BOUND('',#22325,.T.) ;
#18044=FACE_OUTER_BOUND('',#22326,.T.) ;
#18045=FACE_OUTER_BOUND('',#22327,.T.) ;
#18046=FACE_OUTER_BOUND('',#22328,.T.) ;
#18047=FACE_OUTER_BOUND('',#22329,.T.) ;
#18048=FACE_OUTER_BOUND('',#22330,.T.) ;
#18049=FACE_OUTER_BOUND('',#22331,.T.) ;
#18050=FACE_OUTER_BOUND('',#22332,.T.) ;
#18051=FACE_OUTER_BOUND('',#22333,.T.) ;
#18052=FACE_OUTER_BOUND('',#22334,.T.) ;
#18053=FACE_OUTER_BOUND('',#22335,.T.) ;
#18054=FACE_OUTER_BOUND('',#22336,.T.) ;
#20882=EDGE_LOOP('',(#46100,#46101,#46102,#46103,#46104)) ;
#20883=EDGE_LOOP('',(#46105,#46106,#46107,#46108,#46109)) ;
#20884=EDGE_LOOP('',(#46110,#46111,#46112,#46113)) ;
#20885=EDGE_LOOP('',(#46114,#46115,#46116,#46117)) ;
#20886=EDGE_LOOP('',(#46118,#46119,#46120,#46121,#46122)) ;
#20887=EDGE_LOOP('',(#46123,#46124,#46125,#46126)) ;
#20888=EDGE_LOOP('',(#46127,#46128,#46129,#46130)) ;
#20889=EDGE_LOOP('',(#46131,#46132,#46133,#46134)) ;
#20890=EDGE_LOOP('',(#46135,#46136,#46137,#46138,#46139,#46140,#46141,#46142,
#46143,#46144)) ;
#20891=EDGE_LOOP('',(#46145,#46146,#46147,#46148,#46149,#46150)) ;
#20892=EDGE_LOOP('',(#46151,#46152,#46153,#46154,#46155,#46156)) ;
#20893=EDGE_LOOP('',(#46157,#46158,#46159,#46160)) ;
#20894=EDGE_LOOP('',(#46161,#46162,#46163,#46164,#46165,#46166)) ;
#20895=EDGE_LOOP('',(#46167,#46168,#46169,#46170)) ;
#20896=EDGE_LOOP('',(#46171,#46172,#46173,#46174)) ;
#20897=EDGE_LOOP('',(#46175,#46176,#46177,#46178,#46179,#46180)) ;
#20898=EDGE_LOOP('',(#46181,#46182,#46183,#46184,#46185,#46186,#46187,#46188,
#46189,#46190,#46191,#46192,#46193,#46194,#46195,#46196,#46197,#46198,#46199,
#46200,#46201,#46202,#46203,#46204,#46205,#46206,#46207,#46208,#46209,#46210,
#46211,#46212,#46213)) ;
#20899=EDGE_LOOP('',(#46214,#46215,#46216,#46217,#46218,#46219,#46220,#46221,
#46222,#46223,#46224,#46225,#46226,#46227,#46228,#46229,#46230,#46231,#46232,
#46233,#46234,#46235,#46236,#46237,#46238,#46239,#46240,#46241,#46242,#46243,
#46244,#46245,#46246)) ;
#20900=EDGE_LOOP('',(#46247,#46248,#46249,#46250)) ;
#20901=EDGE_LOOP('',(#46251,#46252,#46253,#46254)) ;
#20902=EDGE_LOOP('',(#46255,#46256,#46257,#46258,#46259,#46260,#46261,#46262)) ;
#20903=EDGE_LOOP('',(#46263,#46264,#46265,#46266,#46267,#46268)) ;
#20904=EDGE_LOOP('',(#46269,#46270,#46271,#46272)) ;
#20905=EDGE_LOOP('',(#46273,#46274,#46275,#46276,#46277,#46278)) ;
#20906=EDGE_LOOP('',(#46279,#46280,#46281,#46282,#46283,#46284,#46285,#46286,
#46287,#46288,#46289,#46290,#46291,#46292)) ;
#20907=EDGE_LOOP('',(#46293,#46294,#46295,#46296,#46297,#46298,#46299,#46300,
#46301,#46302,#46303,#46304,#46305,#46306,#46307,#46308,#46309,#46310,#46311,
#46312,#46313,#46314,#46315,#46316)) ;
#20908=EDGE_LOOP('',(#46317)) ;
#20909=EDGE_LOOP('',(#46318,#46319,#46320,#46321,#46322,#46323,#46324,#46325,
#46326,#46327)) ;
#20910=EDGE_LOOP('',(#46328,#46329,#46330,#46331,#46332,#46333,#46334,#46335,
#46336,#46337)) ;
#20911=EDGE_LOOP('',(#46338,#46339,#46340)) ;
#20912=EDGE_LOOP('',(#46341,#46342,#46343)) ;
#20913=EDGE_LOOP('',(#46344,#46345,#46346,#46347,#46348,#46349,#46350,#46351)) ;
#20914=EDGE_LOOP('',(#46352,#46353,#46354,#46355)) ;
#20915=EDGE_LOOP('',(#46356,#46357,#46358,#46359)) ;
#20916=EDGE_LOOP('',(#46360,#46361,#46362,#46363)) ;
#20917=EDGE_LOOP('',(#46364,#46365,#46366,#46367,#46368,#46369)) ;
#20918=EDGE_LOOP('',(#46370,#46371,#46372,#46373,#46374,#46375,#46376,#46377)) ;
#20919=EDGE_LOOP('',(#46378)) ;
#20920=EDGE_LOOP('',(#46379,#46380,#46381,#46382,#46383,#46384,#46385,#46386)) ;
#20921=EDGE_LOOP('',(#46387,#46388,#46389,#46390,#46391,#46392,#46393)) ;
#20922=EDGE_LOOP('',(#46394,#46395,#46396,#46397)) ;
#20923=EDGE_LOOP('',(#46398,#46399,#46400,#46401)) ;
#20924=EDGE_LOOP('',(#46402,#46403,#46404,#46405)) ;
#20925=EDGE_LOOP('',(#46406,#46407,#46408,#46409)) ;
#20926=EDGE_LOOP('',(#46410,#46411,#46412,#46413)) ;
#20927=EDGE_LOOP('',(#46414,#46415,#46416,#46417)) ;
#20928=EDGE_LOOP('',(#46418,#46419,#46420,#46421,#46422,#46423,#46424)) ;
#20929=EDGE_LOOP('',(#46425,#46426,#46427,#46428,#46429)) ;
#20930=EDGE_LOOP('',(#46430,#46431,#46432,#46433)) ;
#20931=EDGE_LOOP('',(#46434,#46435,#46436,#46437)) ;
#20932=EDGE_LOOP('',(#46438,#46439,#46440,#46441)) ;
#20933=EDGE_LOOP('',(#46442,#46443,#46444,#46445)) ;
#20934=EDGE_LOOP('',(#46446,#46447,#46448,#46449)) ;
#20935=EDGE_LOOP('',(#46450,#46451,#46452,#46453)) ;
#20936=EDGE_LOOP('',(#46454,#46455,#46456,#46457,#46458)) ;
#20937=EDGE_LOOP('',(#46459,#46460,#46461,#46462)) ;
#20938=EDGE_LOOP('',(#46463,#46464,#46465,#46466,#46467,#46468,#46469,#46470)) ;
#20939=EDGE_LOOP('',(#46471,#46472,#46473,#46474)) ;
#20940=EDGE_LOOP('',(#46475,#46476,#46477,#46478)) ;
#20941=EDGE_LOOP('',(#46479,#46480,#46481,#46482)) ;
#20942=EDGE_LOOP('',(#46483,#46484,#46485,#46486)) ;
#20943=EDGE_LOOP('',(#46487,#46488,#46489,#46490)) ;
#20944=EDGE_LOOP('',(#46491,#46492,#46493,#46494)) ;
#20945=EDGE_LOOP('',(#46495,#46496,#46497,#46498)) ;
#20946=EDGE_LOOP('',(#46499,#46500,#46501,#46502)) ;
#20947=EDGE_LOOP('',(#46503,#46504,#46505,#46506,#46507,#46508)) ;
#20948=EDGE_LOOP('',(#46509,#46510,#46511,#46512,#46513,#46514)) ;
#20949=EDGE_LOOP('',(#46515,#46516,#46517,#46518)) ;
#20950=EDGE_LOOP('',(#46519,#46520,#46521,#46522)) ;
#20951=EDGE_LOOP('',(#46523,#46524,#46525,#46526)) ;
#20952=EDGE_LOOP('',(#46527,#46528,#46529,#46530)) ;
#20953=EDGE_LOOP('',(#46531,#46532,#46533,#46534)) ;
#20954=EDGE_LOOP('',(#46535,#46536,#46537,#46538)) ;
#20955=EDGE_LOOP('',(#46539,#46540,#46541,#46542)) ;
#20956=EDGE_LOOP('',(#46543,#46544,#46545,#46546)) ;
#20957=EDGE_LOOP('',(#46547,#46548,#46549,#46550)) ;
#20958=EDGE_LOOP('',(#46551,#46552,#46553,#46554)) ;
#20959=EDGE_LOOP('',(#46555,#46556,#46557,#46558)) ;
#20960=EDGE_LOOP('',(#46559,#46560,#46561,#46562)) ;
#20961=EDGE_LOOP('',(#46563,#46564,#46565,#46566)) ;
#20962=EDGE_LOOP('',(#46567,#46568,#46569,#46570)) ;
#20963=EDGE_LOOP('',(#46571,#46572,#46573,#46574)) ;
#20964=EDGE_LOOP('',(#46575,#46576,#46577)) ;
#20965=EDGE_LOOP('',(#46578,#46579,#46580,#46581)) ;
#20966=EDGE_LOOP('',(#46582,#46583,#46584,#46585)) ;
#20967=EDGE_LOOP('',(#46586,#46587,#46588,#46589)) ;
#20968=EDGE_LOOP('',(#46590,#46591,#46592,#46593)) ;
#20969=EDGE_LOOP('',(#46594,#46595,#46596)) ;
#20970=EDGE_LOOP('',(#46597,#46598,#46599,#46600)) ;
#20971=EDGE_LOOP('',(#46601,#46602,#46603,#46604)) ;
#20972=EDGE_LOOP('',(#46605,#46606,#46607,#46608)) ;
#20973=EDGE_LOOP('',(#46609,#46610,#46611,#46612)) ;
#20974=EDGE_LOOP('',(#46613,#46614,#46615,#46616)) ;
#20975=EDGE_LOOP('',(#46617,#46618,#46619,#46620)) ;
#20976=EDGE_LOOP('',(#46621,#46622,#46623,#46624)) ;
#20977=EDGE_LOOP('',(#46625,#46626,#46627)) ;
#20978=EDGE_LOOP('',(#46628,#46629,#46630,#46631)) ;
#20979=EDGE_LOOP('',(#46632,#46633,#46634,#46635)) ;
#20980=EDGE_LOOP('',(#46636,#46637,#46638)) ;
#20981=EDGE_LOOP('',(#46639,#46640,#46641,#46642)) ;
#20982=EDGE_LOOP('',(#46643,#46644,#46645,#46646)) ;
#20983=EDGE_LOOP('',(#46647,#46648,#46649,#46650)) ;
#20984=EDGE_LOOP('',(#46651,#46652,#46653,#46654)) ;
#20985=EDGE_LOOP('',(#46655,#46656,#46657,#46658)) ;
#20986=EDGE_LOOP('',(#46659,#46660,#46661)) ;
#20987=EDGE_LOOP('',(#46662,#46663,#46664,#46665)) ;
#20988=EDGE_LOOP('',(#46666,#46667,#46668,#46669)) ;
#20989=EDGE_LOOP('',(#46670,#46671,#46672,#46673)) ;
#20990=EDGE_LOOP('',(#46674,#46675,#46676,#46677)) ;
#20991=EDGE_LOOP('',(#46678,#46679,#46680,#46681)) ;
#20992=EDGE_LOOP('',(#46682,#46683,#46684,#46685)) ;
#20993=EDGE_LOOP('',(#46686,#46687,#46688)) ;
#20994=EDGE_LOOP('',(#46689,#46690,#46691,#46692)) ;
#20995=EDGE_LOOP('',(#46693,#46694,#46695,#46696)) ;
#20996=EDGE_LOOP('',(#46697,#46698,#46699)) ;
#20997=EDGE_LOOP('',(#46700,#46701,#46702,#46703,#46704)) ;
#20998=EDGE_LOOP('',(#46705,#46706,#46707,#46708,#46709)) ;
#20999=EDGE_LOOP('',(#46710,#46711,#46712,#46713)) ;
#21000=EDGE_LOOP('',(#46714,#46715,#46716,#46717,#46718,#46719)) ;
#21001=EDGE_LOOP('',(#46720,#46721,#46722,#46723,#46724,#46725)) ;
#21002=EDGE_LOOP('',(#46726,#46727,#46728,#46729)) ;
#21003=EDGE_LOOP('',(#46730,#46731,#46732,#46733)) ;
#21004=EDGE_LOOP('',(#46734,#46735,#46736)) ;
#21005=EDGE_LOOP('',(#46737,#46738,#46739,#46740,#46741)) ;
#21006=EDGE_LOOP('',(#46742,#46743,#46744,#46745,#46746)) ;
#21007=EDGE_LOOP('',(#46747,#46748,#46749,#46750)) ;
#21008=EDGE_LOOP('',(#46751,#46752,#46753,#46754,#46755)) ;
#21009=EDGE_LOOP('',(#46756,#46757,#46758,#46759)) ;
#21010=EDGE_LOOP('',(#46760,#46761,#46762,#46763)) ;
#21011=EDGE_LOOP('',(#46764,#46765,#46766)) ;
#21012=EDGE_LOOP('',(#46767,#46768,#46769)) ;
#21013=EDGE_LOOP('',(#46770,#46771,#46772,#46773,#46774)) ;
#21014=EDGE_LOOP('',(#46775,#46776,#46777,#46778)) ;
#21015=EDGE_LOOP('',(#46779,#46780,#46781)) ;
#21016=EDGE_LOOP('',(#46782,#46783,#46784,#46785)) ;
#21017=EDGE_LOOP('',(#46786,#46787,#46788,#46789)) ;
#21018=EDGE_LOOP('',(#46790,#46791,#46792,#46793)) ;
#21019=EDGE_LOOP('',(#46794,#46795,#46796,#46797)) ;
#21020=EDGE_LOOP('',(#46798,#46799,#46800,#46801)) ;
#21021=EDGE_LOOP('',(#46802,#46803,#46804,#46805)) ;
#21022=EDGE_LOOP('',(#46806,#46807,#46808)) ;
#21023=EDGE_LOOP('',(#46809,#46810,#46811,#46812)) ;
#21024=EDGE_LOOP('',(#46813,#46814,#46815,#46816,#46817)) ;
#21025=EDGE_LOOP('',(#46818,#46819,#46820,#46821)) ;
#21026=EDGE_LOOP('',(#46822,#46823,#46824,#46825)) ;
#21027=EDGE_LOOP('',(#46826,#46827,#46828,#46829,#46830)) ;
#21028=EDGE_LOOP('',(#46831,#46832,#46833,#46834)) ;
#21029=EDGE_LOOP('',(#46835,#46836,#46837)) ;
#21030=EDGE_LOOP('',(#46838,#46839,#46840,#46841)) ;
#21031=EDGE_LOOP('',(#46842,#46843,#46844,#46845)) ;
#21032=EDGE_LOOP('',(#46846,#46847,#46848,#46849)) ;
#21033=EDGE_LOOP('',(#46850,#46851,#46852,#46853)) ;
#21034=EDGE_LOOP('',(#46854,#46855,#46856,#46857)) ;
#21035=EDGE_LOOP('',(#46858,#46859,#46860,#46861)) ;
#21036=EDGE_LOOP('',(#46862,#46863,#46864)) ;
#21037=EDGE_LOOP('',(#46865,#46866,#46867,#46868)) ;
#21038=EDGE_LOOP('',(#46869,#46870,#46871,#46872)) ;
#21039=EDGE_LOOP('',(#46873,#46874,#46875,#46876)) ;
#21040=EDGE_LOOP('',(#46877,#46878,#46879,#46880)) ;
#21041=EDGE_LOOP('',(#46881,#46882,#46883,#46884)) ;
#21042=EDGE_LOOP('',(#46885,#46886,#46887,#46888)) ;
#21043=EDGE_LOOP('',(#46889,#46890,#46891,#46892)) ;
#21044=EDGE_LOOP('',(#46893,#46894,#46895,#46896)) ;
#21045=EDGE_LOOP('',(#46897,#46898,#46899,#46900)) ;
#21046=EDGE_LOOP('',(#46901,#46902,#46903)) ;
#21047=EDGE_LOOP('',(#46904,#46905,#46906,#46907)) ;
#21048=EDGE_LOOP('',(#46908,#46909,#46910)) ;
#21049=EDGE_LOOP('',(#46911,#46912,#46913,#46914)) ;
#21050=EDGE_LOOP('',(#46915,#46916,#46917,#46918)) ;
#21051=EDGE_LOOP('',(#46919,#46920,#46921,#46922)) ;
#21052=EDGE_LOOP('',(#46923,#46924,#46925,#46926)) ;
#21053=EDGE_LOOP('',(#46927,#46928,#46929,#46930)) ;
#21054=EDGE_LOOP('',(#46931,#46932,#46933,#46934)) ;
#21055=EDGE_LOOP('',(#46935,#46936,#46937,#46938)) ;
#21056=EDGE_LOOP('',(#46939,#46940,#46941,#46942,#46943,#46944)) ;
#21057=EDGE_LOOP('',(#46945,#46946,#46947)) ;
#21058=EDGE_LOOP('',(#46948,#46949,#46950,#46951)) ;
#21059=EDGE_LOOP('',(#46952,#46953,#46954,#46955)) ;
#21060=EDGE_LOOP('',(#46956,#46957,#46958,#46959)) ;
#21061=EDGE_LOOP('',(#46960,#46961,#46962,#46963)) ;
#21062=EDGE_LOOP('',(#46964,#46965,#46966,#46967)) ;
#21063=EDGE_LOOP('',(#46968,#46969,#46970,#46971)) ;
#21064=EDGE_LOOP('',(#46972,#46973,#46974,#46975)) ;
#21065=EDGE_LOOP('',(#46976,#46977,#46978,#46979,#46980)) ;
#21066=EDGE_LOOP('',(#46981,#46982,#46983,#46984)) ;
#21067=EDGE_LOOP('',(#46985,#46986,#46987,#46988,#46989)) ;
#21068=EDGE_LOOP('',(#46990,#46991,#46992,#46993)) ;
#21069=EDGE_LOOP('',(#46994,#46995,#46996,#46997,#46998)) ;
#21070=EDGE_LOOP('',(#46999,#47000,#47001,#47002)) ;
#21071=EDGE_LOOP('',(#47003,#47004,#47005)) ;
#21072=EDGE_LOOP('',(#47006,#47007,#47008,#47009)) ;
#21073=EDGE_LOOP('',(#47010,#47011,#47012,#47013)) ;
#21074=EDGE_LOOP('',(#47014,#47015,#47016,#47017)) ;
#21075=EDGE_LOOP('',(#47018,#47019,#47020,#47021)) ;
#21076=EDGE_LOOP('',(#47022,#47023,#47024,#47025)) ;
#21077=EDGE_LOOP('',(#47026,#47027,#47028)) ;
#21078=EDGE_LOOP('',(#47029,#47030,#47031)) ;
#21079=EDGE_LOOP('',(#47032,#47033,#47034,#47035)) ;
#21080=EDGE_LOOP('',(#47036,#47037,#47038,#47039)) ;
#21081=EDGE_LOOP('',(#47040,#47041,#47042)) ;
#21082=EDGE_LOOP('',(#47043,#47044,#47045,#47046)) ;
#21083=EDGE_LOOP('',(#47047,#47048,#47049,#47050)) ;
#21084=EDGE_LOOP('',(#47051,#47052,#47053,#47054,#47055)) ;
#21085=EDGE_LOOP('',(#47056,#47057,#47058,#47059)) ;
#21086=EDGE_LOOP('',(#47060,#47061,#47062,#47063)) ;
#21087=EDGE_LOOP('',(#47064,#47065,#47066,#47067)) ;
#21088=EDGE_LOOP('',(#47068,#47069,#47070,#47071)) ;
#21089=EDGE_LOOP('',(#47072,#47073,#47074,#47075)) ;
#21090=EDGE_LOOP('',(#47076,#47077,#47078)) ;
#21091=EDGE_LOOP('',(#47079,#47080,#47081,#47082)) ;
#21092=EDGE_LOOP('',(#47083,#47084,#47085,#47086)) ;
#21093=EDGE_LOOP('',(#47087,#47088,#47089)) ;
#21094=EDGE_LOOP('',(#47090,#47091,#47092,#47093)) ;
#21095=EDGE_LOOP('',(#47094,#47095,#47096,#47097)) ;
#21096=EDGE_LOOP('',(#47098,#47099,#47100,#47101)) ;
#21097=EDGE_LOOP('',(#47102,#47103,#47104,#47105)) ;
#21098=EDGE_LOOP('',(#47106,#47107,#47108)) ;
#21099=EDGE_LOOP('',(#47109,#47110,#47111)) ;
#21100=EDGE_LOOP('',(#47112,#47113,#47114,#47115)) ;
#21101=EDGE_LOOP('',(#47116,#47117,#47118,#47119)) ;
#21102=EDGE_LOOP('',(#47120,#47121,#47122,#47123)) ;
#21103=EDGE_LOOP('',(#47124,#47125,#47126)) ;
#21104=EDGE_LOOP('',(#47127,#47128,#47129,#47130)) ;
#21105=EDGE_LOOP('',(#47131,#47132,#47133,#47134)) ;
#21106=EDGE_LOOP('',(#47135,#47136,#47137)) ;
#21107=EDGE_LOOP('',(#47138,#47139,#47140,#47141)) ;
#21108=EDGE_LOOP('',(#47142,#47143,#47144,#47145,#47146)) ;
#21109=EDGE_LOOP('',(#47147,#47148,#47149,#47150)) ;
#21110=EDGE_LOOP('',(#47151,#47152,#47153)) ;
#21111=EDGE_LOOP('',(#47154,#47155,#47156,#47157)) ;
#21112=EDGE_LOOP('',(#47158,#47159,#47160,#47161)) ;
#21113=EDGE_LOOP('',(#47162,#47163,#47164)) ;
#21114=EDGE_LOOP('',(#47165,#47166,#47167,#47168,#47169)) ;
#21115=EDGE_LOOP('',(#47170,#47171,#47172,#47173)) ;
#21116=EDGE_LOOP('',(#47174,#47175,#47176,#47177)) ;
#21117=EDGE_LOOP('',(#47178,#47179,#47180,#47181)) ;
#21118=EDGE_LOOP('',(#47182,#47183,#47184,#47185)) ;
#21119=EDGE_LOOP('',(#47186,#47187,#47188,#47189)) ;
#21120=EDGE_LOOP('',(#47190,#47191,#47192,#47193)) ;
#21121=EDGE_LOOP('',(#47194,#47195,#47196,#47197)) ;
#21122=EDGE_LOOP('',(#47198,#47199,#47200,#47201)) ;
#21123=EDGE_LOOP('',(#47202,#47203,#47204,#47205,#47206)) ;
#21124=EDGE_LOOP('',(#47207,#47208,#47209,#47210,#47211,#47212,#47213,#47214)) ;
#21125=EDGE_LOOP('',(#47215,#47216,#47217)) ;
#21126=EDGE_LOOP('',(#47218,#47219,#47220,#47221)) ;
#21127=EDGE_LOOP('',(#47222,#47223,#47224,#47225,#47226)) ;
#21128=EDGE_LOOP('',(#47227,#47228,#47229,#47230,#47231)) ;
#21129=EDGE_LOOP('',(#47232,#47233,#47234,#47235)) ;
#21130=EDGE_LOOP('',(#47236,#47237,#47238)) ;
#21131=EDGE_LOOP('',(#47239,#47240,#47241,#47242,#47243,#47244,#47245,#47246)) ;
#21132=EDGE_LOOP('',(#47247,#47248,#47249,#47250,#47251)) ;
#21133=EDGE_LOOP('',(#47252,#47253,#47254,#47255,#47256)) ;
#21134=EDGE_LOOP('',(#47257,#47258,#47259,#47260)) ;
#21135=EDGE_LOOP('',(#47261,#47262,#47263,#47264,#47265,#47266,#47267,#47268)) ;
#21136=EDGE_LOOP('',(#47269,#47270,#47271,#47272)) ;
#21137=EDGE_LOOP('',(#47273,#47274,#47275,#47276,#47277,#47278,#47279,#47280)) ;
#21138=EDGE_LOOP('',(#47281,#47282,#47283,#47284)) ;
#21139=EDGE_LOOP('',(#47285,#47286,#47287,#47288)) ;
#21140=EDGE_LOOP('',(#47289,#47290,#47291,#47292)) ;
#21141=EDGE_LOOP('',(#47293,#47294,#47295,#47296)) ;
#21142=EDGE_LOOP('',(#47297,#47298,#47299,#47300,#47301,#47302,#47303,#47304,
#47305)) ;
#21143=EDGE_LOOP('',(#47306,#47307,#47308,#47309,#47310,#47311,#47312)) ;
#21144=EDGE_LOOP('',(#47313,#47314,#47315,#47316)) ;
#21145=EDGE_LOOP('',(#47317,#47318,#47319,#47320)) ;
#21146=EDGE_LOOP('',(#47321,#47322,#47323,#47324)) ;
#21147=EDGE_LOOP('',(#47325,#47326,#47327)) ;
#21148=EDGE_LOOP('',(#47328,#47329,#47330,#47331)) ;
#21149=EDGE_LOOP('',(#47332,#47333,#47334,#47335)) ;
#21150=EDGE_LOOP('',(#47336,#47337,#47338,#47339)) ;
#21151=EDGE_LOOP('',(#47340,#47341,#47342,#47343)) ;
#21152=EDGE_LOOP('',(#47344,#47345,#47346,#47347)) ;
#21153=EDGE_LOOP('',(#47348,#47349,#47350,#47351)) ;
#21154=EDGE_LOOP('',(#47352,#47353,#47354,#47355)) ;
#21155=EDGE_LOOP('',(#47356,#47357,#47358,#47359)) ;
#21156=EDGE_LOOP('',(#47360,#47361,#47362,#47363)) ;
#21157=EDGE_LOOP('',(#47364,#47365,#47366,#47367)) ;
#21158=EDGE_LOOP('',(#47368,#47369,#47370,#47371)) ;
#21159=EDGE_LOOP('',(#47372,#47373,#47374,#47375)) ;
#21160=EDGE_LOOP('',(#47376,#47377,#47378,#47379)) ;
#21161=EDGE_LOOP('',(#47380,#47381,#47382,#47383)) ;
#21162=EDGE_LOOP('',(#47384,#47385,#47386,#47387)) ;
#21163=EDGE_LOOP('',(#47388,#47389,#47390,#47391)) ;
#21164=EDGE_LOOP('',(#47392,#47393,#47394,#47395)) ;
#21165=EDGE_LOOP('',(#47396,#47397,#47398,#47399)) ;
#21166=EDGE_LOOP('',(#47400,#47401,#47402,#47403)) ;
#21167=EDGE_LOOP('',(#47404,#47405,#47406)) ;
#21168=EDGE_LOOP('',(#47407,#47408,#47409,#47410)) ;
#21169=EDGE_LOOP('',(#47411,#47412,#47413,#47414,#47415,#47416)) ;
#21170=EDGE_LOOP('',(#47417,#47418,#47419,#47420)) ;
#21171=EDGE_LOOP('',(#47421,#47422,#47423,#47424,#47425)) ;
#21172=EDGE_LOOP('',(#47426,#47427,#47428,#47429)) ;
#21173=EDGE_LOOP('',(#47430,#47431,#47432,#47433,#47434)) ;
#21174=EDGE_LOOP('',(#47435,#47436,#47437,#47438,#47439)) ;
#21175=EDGE_LOOP('',(#47440,#47441,#47442,#47443)) ;
#21176=EDGE_LOOP('',(#47444,#47445,#47446,#47447)) ;
#21177=EDGE_LOOP('',(#47448,#47449,#47450,#47451,#47452)) ;
#21178=EDGE_LOOP('',(#47453,#47454,#47455,#47456)) ;
#21179=EDGE_LOOP('',(#47457,#47458,#47459,#47460)) ;
#21180=EDGE_LOOP('',(#47461,#47462,#47463,#47464)) ;
#21181=EDGE_LOOP('',(#47465,#47466,#47467,#47468,#47469,#47470,#47471,#47472,
#47473,#47474)) ;
#21182=EDGE_LOOP('',(#47475,#47476,#47477,#47478,#47479,#47480)) ;
#21183=EDGE_LOOP('',(#47481,#47482,#47483,#47484,#47485,#47486)) ;
#21184=EDGE_LOOP('',(#47487,#47488,#47489,#47490)) ;
#21185=EDGE_LOOP('',(#47491,#47492,#47493,#47494,#47495,#47496)) ;
#21186=EDGE_LOOP('',(#47497,#47498,#47499,#47500)) ;
#21187=EDGE_LOOP('',(#47501,#47502,#47503,#47504)) ;
#21188=EDGE_LOOP('',(#47505,#47506,#47507,#47508,#47509,#47510)) ;
#21189=EDGE_LOOP('',(#47511,#47512,#47513,#47514,#47515,#47516,#47517,#47518,
#47519,#47520,#47521,#47522,#47523,#47524,#47525,#47526,#47527,#47528,#47529,
#47530,#47531,#47532,#47533,#47534,#47535,#47536,#47537,#47538,#47539,#47540,
#47541,#47542,#47543)) ;
#21190=EDGE_LOOP('',(#47544,#47545,#47546,#47547,#47548,#47549,#47550,#47551,
#47552,#47553,#47554,#47555,#47556,#47557,#47558,#47559,#47560,#47561,#47562,
#47563,#47564,#47565,#47566,#47567,#47568,#47569,#47570,#47571,#47572,#47573,
#47574,#47575,#47576)) ;
#21191=EDGE_LOOP('',(#47577,#47578,#47579,#47580)) ;
#21192=EDGE_LOOP('',(#47581,#47582,#47583,#47584)) ;
#21193=EDGE_LOOP('',(#47585,#47586,#47587,#47588,#47589,#47590,#47591,#47592)) ;
#21194=EDGE_LOOP('',(#47593,#47594,#47595,#47596,#47597,#47598)) ;
#21195=EDGE_LOOP('',(#47599,#47600,#47601,#47602)) ;
#21196=EDGE_LOOP('',(#47603,#47604,#47605,#47606,#47607,#47608)) ;
#21197=EDGE_LOOP('',(#47609,#47610,#47611,#47612,#47613,#47614,#47615,#47616,
#47617,#47618,#47619,#47620,#47621,#47622)) ;
#21198=EDGE_LOOP('',(#47623,#47624,#47625,#47626,#47627,#47628,#47629,#47630,
#47631,#47632,#47633,#47634,#47635,#47636,#47637,#47638,#47639,#47640,#47641,
#47642,#47643,#47644,#47645,#47646)) ;
#21199=EDGE_LOOP('',(#47647)) ;
#21200=EDGE_LOOP('',(#47648,#47649,#47650,#47651,#47652,#47653,#47654,#47655,
#47656,#47657)) ;
#21201=EDGE_LOOP('',(#47658,#47659,#47660,#47661,#47662,#47663,#47664,#47665,
#47666,#47667)) ;
#21202=EDGE_LOOP('',(#47668,#47669,#47670)) ;
#21203=EDGE_LOOP('',(#47671,#47672,#47673)) ;
#21204=EDGE_LOOP('',(#47674,#47675,#47676,#47677,#47678,#47679,#47680,#47681)) ;
#21205=EDGE_LOOP('',(#47682,#47683,#47684,#47685)) ;
#21206=EDGE_LOOP('',(#47686,#47687,#47688,#47689)) ;
#21207=EDGE_LOOP('',(#47690,#47691,#47692,#47693)) ;
#21208=EDGE_LOOP('',(#47694,#47695,#47696,#47697,#47698,#47699)) ;
#21209=EDGE_LOOP('',(#47700,#47701,#47702,#47703,#47704,#47705,#47706,#47707)) ;
#21210=EDGE_LOOP('',(#47708)) ;
#21211=EDGE_LOOP('',(#47709,#47710,#47711,#47712,#47713,#47714,#47715,#47716)) ;
#21212=EDGE_LOOP('',(#47717,#47718,#47719,#47720,#47721,#47722,#47723)) ;
#21213=EDGE_LOOP('',(#47724,#47725,#47726,#47727)) ;
#21214=EDGE_LOOP('',(#47728,#47729,#47730,#47731)) ;
#21215=EDGE_LOOP('',(#47732,#47733,#47734,#47735)) ;
#21216=EDGE_LOOP('',(#47736,#47737,#47738,#47739)) ;
#21217=EDGE_LOOP('',(#47740,#47741,#47742,#47743)) ;
#21218=EDGE_LOOP('',(#47744,#47745,#47746,#47747)) ;
#21219=EDGE_LOOP('',(#47748,#47749,#47750,#47751,#47752,#47753,#47754)) ;
#21220=EDGE_LOOP('',(#47755,#47756,#47757,#47758,#47759)) ;
#21221=EDGE_LOOP('',(#47760,#47761,#47762,#47763)) ;
#21222=EDGE_LOOP('',(#47764,#47765,#47766,#47767)) ;
#21223=EDGE_LOOP('',(#47768,#47769,#47770,#47771)) ;
#21224=EDGE_LOOP('',(#47772,#47773,#47774,#47775)) ;
#21225=EDGE_LOOP('',(#47776,#47777,#47778,#47779)) ;
#21226=EDGE_LOOP('',(#47780,#47781,#47782,#47783)) ;
#21227=EDGE_LOOP('',(#47784,#47785,#47786,#47787,#47788)) ;
#21228=EDGE_LOOP('',(#47789,#47790,#47791,#47792)) ;
#21229=EDGE_LOOP('',(#47793,#47794,#47795,#47796,#47797,#47798,#47799,#47800)) ;
#21230=EDGE_LOOP('',(#47801,#47802,#47803,#47804)) ;
#21231=EDGE_LOOP('',(#47805,#47806,#47807,#47808)) ;
#21232=EDGE_LOOP('',(#47809,#47810,#47811,#47812)) ;
#21233=EDGE_LOOP('',(#47813,#47814,#47815,#47816)) ;
#21234=EDGE_LOOP('',(#47817,#47818,#47819,#47820)) ;
#21235=EDGE_LOOP('',(#47821,#47822,#47823,#47824)) ;
#21236=EDGE_LOOP('',(#47825,#47826,#47827,#47828)) ;
#21237=EDGE_LOOP('',(#47829,#47830,#47831,#47832)) ;
#21238=EDGE_LOOP('',(#47833,#47834,#47835,#47836,#47837,#47838)) ;
#21239=EDGE_LOOP('',(#47839,#47840,#47841,#47842,#47843,#47844)) ;
#21240=EDGE_LOOP('',(#47845,#47846,#47847,#47848)) ;
#21241=EDGE_LOOP('',(#47849,#47850,#47851,#47852)) ;
#21242=EDGE_LOOP('',(#47853,#47854,#47855,#47856)) ;
#21243=EDGE_LOOP('',(#47857,#47858,#47859,#47860)) ;
#21244=EDGE_LOOP('',(#47861,#47862,#47863,#47864)) ;
#21245=EDGE_LOOP('',(#47865,#47866,#47867,#47868)) ;
#21246=EDGE_LOOP('',(#47869,#47870,#47871,#47872)) ;
#21247=EDGE_LOOP('',(#47873,#47874,#47875,#47876)) ;
#21248=EDGE_LOOP('',(#47877,#47878,#47879,#47880)) ;
#21249=EDGE_LOOP('',(#47881,#47882,#47883,#47884)) ;
#21250=EDGE_LOOP('',(#47885,#47886,#47887,#47888)) ;
#21251=EDGE_LOOP('',(#47889,#47890,#47891,#47892)) ;
#21252=EDGE_LOOP('',(#47893,#47894,#47895,#47896)) ;
#21253=EDGE_LOOP('',(#47897,#47898,#47899,#47900)) ;
#21254=EDGE_LOOP('',(#47901,#47902,#47903,#47904)) ;
#21255=EDGE_LOOP('',(#47905,#47906,#47907)) ;
#21256=EDGE_LOOP('',(#47908,#47909,#47910,#47911)) ;
#21257=EDGE_LOOP('',(#47912,#47913,#47914,#47915)) ;
#21258=EDGE_LOOP('',(#47916,#47917,#47918,#47919)) ;
#21259=EDGE_LOOP('',(#47920,#47921,#47922,#47923)) ;
#21260=EDGE_LOOP('',(#47924,#47925,#47926)) ;
#21261=EDGE_LOOP('',(#47927,#47928,#47929,#47930)) ;
#21262=EDGE_LOOP('',(#47931,#47932,#47933,#47934)) ;
#21263=EDGE_LOOP('',(#47935,#47936,#47937,#47938)) ;
#21264=EDGE_LOOP('',(#47939,#47940,#47941,#47942)) ;
#21265=EDGE_LOOP('',(#47943,#47944,#47945,#47946)) ;
#21266=EDGE_LOOP('',(#47947,#47948,#47949,#47950)) ;
#21267=EDGE_LOOP('',(#47951,#47952,#47953,#47954)) ;
#21268=EDGE_LOOP('',(#47955,#47956,#47957)) ;
#21269=EDGE_LOOP('',(#47958,#47959,#47960,#47961)) ;
#21270=EDGE_LOOP('',(#47962,#47963,#47964,#47965)) ;
#21271=EDGE_LOOP('',(#47966,#47967,#47968)) ;
#21272=EDGE_LOOP('',(#47969,#47970,#47971,#47972)) ;
#21273=EDGE_LOOP('',(#47973,#47974,#47975,#47976)) ;
#21274=EDGE_LOOP('',(#47977,#47978,#47979,#47980)) ;
#21275=EDGE_LOOP('',(#47981,#47982,#47983,#47984)) ;
#21276=EDGE_LOOP('',(#47985,#47986,#47987,#47988)) ;
#21277=EDGE_LOOP('',(#47989,#47990,#47991)) ;
#21278=EDGE_LOOP('',(#47992,#47993,#47994,#47995)) ;
#21279=EDGE_LOOP('',(#47996,#47997,#47998,#47999)) ;
#21280=EDGE_LOOP('',(#48000,#48001,#48002,#48003)) ;
#21281=EDGE_LOOP('',(#48004,#48005,#48006,#48007)) ;
#21282=EDGE_LOOP('',(#48008,#48009,#48010,#48011)) ;
#21283=EDGE_LOOP('',(#48012,#48013,#48014,#48015)) ;
#21284=EDGE_LOOP('',(#48016,#48017,#48018)) ;
#21285=EDGE_LOOP('',(#48019,#48020,#48021,#48022)) ;
#21286=EDGE_LOOP('',(#48023,#48024,#48025,#48026)) ;
#21287=EDGE_LOOP('',(#48027,#48028,#48029)) ;
#21288=EDGE_LOOP('',(#48030,#48031,#48032,#48033,#48034)) ;
#21289=EDGE_LOOP('',(#48035,#48036,#48037,#48038,#48039)) ;
#21290=EDGE_LOOP('',(#48040,#48041,#48042,#48043)) ;
#21291=EDGE_LOOP('',(#48044,#48045,#48046,#48047,#48048,#48049)) ;
#21292=EDGE_LOOP('',(#48050,#48051,#48052,#48053,#48054,#48055)) ;
#21293=EDGE_LOOP('',(#48056,#48057,#48058,#48059)) ;
#21294=EDGE_LOOP('',(#48060,#48061,#48062,#48063)) ;
#21295=EDGE_LOOP('',(#48064,#48065,#48066)) ;
#21296=EDGE_LOOP('',(#48067,#48068,#48069,#48070,#48071)) ;
#21297=EDGE_LOOP('',(#48072,#48073,#48074,#48075,#48076)) ;
#21298=EDGE_LOOP('',(#48077,#48078,#48079,#48080)) ;
#21299=EDGE_LOOP('',(#48081,#48082,#48083,#48084,#48085)) ;
#21300=EDGE_LOOP('',(#48086,#48087,#48088,#48089)) ;
#21301=EDGE_LOOP('',(#48090,#48091,#48092,#48093)) ;
#21302=EDGE_LOOP('',(#48094,#48095,#48096)) ;
#21303=EDGE_LOOP('',(#48097,#48098,#48099)) ;
#21304=EDGE_LOOP('',(#48100,#48101,#48102,#48103,#48104)) ;
#21305=EDGE_LOOP('',(#48105,#48106,#48107,#48108)) ;
#21306=EDGE_LOOP('',(#48109,#48110,#48111)) ;
#21307=EDGE_LOOP('',(#48112,#48113,#48114,#48115)) ;
#21308=EDGE_LOOP('',(#48116,#48117,#48118,#48119)) ;
#21309=EDGE_LOOP('',(#48120,#48121,#48122,#48123)) ;
#21310=EDGE_LOOP('',(#48124,#48125,#48126,#48127)) ;
#21311=EDGE_LOOP('',(#48128,#48129,#48130,#48131)) ;
#21312=EDGE_LOOP('',(#48132,#48133,#48134,#48135)) ;
#21313=EDGE_LOOP('',(#48136,#48137,#48138)) ;
#21314=EDGE_LOOP('',(#48139,#48140,#48141,#48142)) ;
#21315=EDGE_LOOP('',(#48143,#48144,#48145,#48146,#48147)) ;
#21316=EDGE_LOOP('',(#48148,#48149,#48150,#48151)) ;
#21317=EDGE_LOOP('',(#48152,#48153,#48154,#48155)) ;
#21318=EDGE_LOOP('',(#48156,#48157,#48158,#48159,#48160)) ;
#21319=EDGE_LOOP('',(#48161,#48162,#48163,#48164)) ;
#21320=EDGE_LOOP('',(#48165,#48166,#48167)) ;
#21321=EDGE_LOOP('',(#48168,#48169,#48170,#48171)) ;
#21322=EDGE_LOOP('',(#48172,#48173,#48174,#48175)) ;
#21323=EDGE_LOOP('',(#48176,#48177,#48178,#48179)) ;
#21324=EDGE_LOOP('',(#48180,#48181,#48182,#48183)) ;
#21325=EDGE_LOOP('',(#48184,#48185,#48186,#48187)) ;
#21326=EDGE_LOOP('',(#48188,#48189,#48190,#48191)) ;
#21327=EDGE_LOOP('',(#48192,#48193,#48194)) ;
#21328=EDGE_LOOP('',(#48195,#48196,#48197,#48198)) ;
#21329=EDGE_LOOP('',(#48199,#48200,#48201,#48202)) ;
#21330=EDGE_LOOP('',(#48203,#48204,#48205,#48206)) ;
#21331=EDGE_LOOP('',(#48207,#48208,#48209,#48210)) ;
#21332=EDGE_LOOP('',(#48211,#48212,#48213,#48214)) ;
#21333=EDGE_LOOP('',(#48215,#48216,#48217,#48218)) ;
#21334=EDGE_LOOP('',(#48219,#48220,#48221,#48222)) ;
#21335=EDGE_LOOP('',(#48223,#48224,#48225,#48226)) ;
#21336=EDGE_LOOP('',(#48227,#48228,#48229,#48230)) ;
#21337=EDGE_LOOP('',(#48231,#48232,#48233)) ;
#21338=EDGE_LOOP('',(#48234,#48235,#48236,#48237)) ;
#21339=EDGE_LOOP('',(#48238,#48239,#48240)) ;
#21340=EDGE_LOOP('',(#48241,#48242,#48243,#48244)) ;
#21341=EDGE_LOOP('',(#48245,#48246,#48247,#48248)) ;
#21342=EDGE_LOOP('',(#48249,#48250,#48251,#48252)) ;
#21343=EDGE_LOOP('',(#48253,#48254,#48255,#48256)) ;
#21344=EDGE_LOOP('',(#48257,#48258,#48259,#48260)) ;
#21345=EDGE_LOOP('',(#48261,#48262,#48263,#48264)) ;
#21346=EDGE_LOOP('',(#48265,#48266,#48267,#48268)) ;
#21347=EDGE_LOOP('',(#48269,#48270,#48271,#48272,#48273,#48274)) ;
#21348=EDGE_LOOP('',(#48275,#48276,#48277)) ;
#21349=EDGE_LOOP('',(#48278,#48279,#48280,#48281)) ;
#21350=EDGE_LOOP('',(#48282,#48283,#48284,#48285)) ;
#21351=EDGE_LOOP('',(#48286,#48287,#48288,#48289)) ;
#21352=EDGE_LOOP('',(#48290,#48291,#48292,#48293)) ;
#21353=EDGE_LOOP('',(#48294,#48295,#48296,#48297)) ;
#21354=EDGE_LOOP('',(#48298,#48299,#48300,#48301)) ;
#21355=EDGE_LOOP('',(#48302,#48303,#48304,#48305)) ;
#21356=EDGE_LOOP('',(#48306,#48307,#48308,#48309,#48310)) ;
#21357=EDGE_LOOP('',(#48311,#48312,#48313,#48314)) ;
#21358=EDGE_LOOP('',(#48315,#48316,#48317,#48318,#48319)) ;
#21359=EDGE_LOOP('',(#48320,#48321,#48322,#48323)) ;
#21360=EDGE_LOOP('',(#48324,#48325,#48326,#48327,#48328)) ;
#21361=EDGE_LOOP('',(#48329,#48330,#48331,#48332)) ;
#21362=EDGE_LOOP('',(#48333,#48334,#48335)) ;
#21363=EDGE_LOOP('',(#48336,#48337,#48338,#48339)) ;
#21364=EDGE_LOOP('',(#48340,#48341,#48342,#48343)) ;
#21365=EDGE_LOOP('',(#48344,#48345,#48346,#48347)) ;
#21366=EDGE_LOOP('',(#48348,#48349,#48350,#48351)) ;
#21367=EDGE_LOOP('',(#48352,#48353,#48354,#48355)) ;
#21368=EDGE_LOOP('',(#48356,#48357,#48358)) ;
#21369=EDGE_LOOP('',(#48359,#48360,#48361)) ;
#21370=EDGE_LOOP('',(#48362,#48363,#48364,#48365)) ;
#21371=EDGE_LOOP('',(#48366,#48367,#48368,#48369)) ;
#21372=EDGE_LOOP('',(#48370,#48371,#48372)) ;
#21373=EDGE_LOOP('',(#48373,#48374,#48375,#48376)) ;
#21374=EDGE_LOOP('',(#48377,#48378,#48379,#48380)) ;
#21375=EDGE_LOOP('',(#48381,#48382,#48383,#48384,#48385)) ;
#21376=EDGE_LOOP('',(#48386,#48387,#48388,#48389)) ;
#21377=EDGE_LOOP('',(#48390,#48391,#48392,#48393)) ;
#21378=EDGE_LOOP('',(#48394,#48395,#48396,#48397)) ;
#21379=EDGE_LOOP('',(#48398,#48399,#48400,#48401)) ;
#21380=EDGE_LOOP('',(#48402,#48403,#48404,#48405)) ;
#21381=EDGE_LOOP('',(#48406,#48407,#48408)) ;
#21382=EDGE_LOOP('',(#48409,#48410,#48411,#48412)) ;
#21383=EDGE_LOOP('',(#48413,#48414,#48415,#48416)) ;
#21384=EDGE_LOOP('',(#48417,#48418,#48419)) ;
#21385=EDGE_LOOP('',(#48420,#48421,#48422,#48423)) ;
#21386=EDGE_LOOP('',(#48424,#48425,#48426,#48427)) ;
#21387=EDGE_LOOP('',(#48428,#48429,#48430,#48431)) ;
#21388=EDGE_LOOP('',(#48432,#48433,#48434,#48435)) ;
#21389=EDGE_LOOP('',(#48436,#48437,#48438)) ;
#21390=EDGE_LOOP('',(#48439,#48440,#48441)) ;
#21391=EDGE_LOOP('',(#48442,#48443,#48444,#48445)) ;
#21392=EDGE_LOOP('',(#48446,#48447,#48448,#48449)) ;
#21393=EDGE_LOOP('',(#48450,#48451,#48452,#48453)) ;
#21394=EDGE_LOOP('',(#48454,#48455,#48456)) ;
#21395=EDGE_LOOP('',(#48457,#48458,#48459,#48460)) ;
#21396=EDGE_LOOP('',(#48461,#48462,#48463,#48464)) ;
#21397=EDGE_LOOP('',(#48465,#48466,#48467)) ;
#21398=EDGE_LOOP('',(#48468,#48469,#48470,#48471)) ;
#21399=EDGE_LOOP('',(#48472,#48473,#48474,#48475,#48476)) ;
#21400=EDGE_LOOP('',(#48477,#48478,#48479,#48480)) ;
#21401=EDGE_LOOP('',(#48481,#48482,#48483)) ;
#21402=EDGE_LOOP('',(#48484,#48485,#48486,#48487)) ;
#21403=EDGE_LOOP('',(#48488,#48489,#48490,#48491)) ;
#21404=EDGE_LOOP('',(#48492,#48493,#48494)) ;
#21405=EDGE_LOOP('',(#48495,#48496,#48497,#48498,#48499)) ;
#21406=EDGE_LOOP('',(#48500,#48501,#48502,#48503)) ;
#21407=EDGE_LOOP('',(#48504,#48505,#48506,#48507)) ;
#21408=EDGE_LOOP('',(#48508,#48509,#48510,#48511)) ;
#21409=EDGE_LOOP('',(#48512,#48513,#48514,#48515)) ;
#21410=EDGE_LOOP('',(#48516,#48517,#48518,#48519)) ;
#21411=EDGE_LOOP('',(#48520,#48521,#48522,#48523)) ;
#21412=EDGE_LOOP('',(#48524,#48525,#48526,#48527)) ;
#21413=EDGE_LOOP('',(#48528,#48529,#48530,#48531)) ;
#21414=EDGE_LOOP('',(#48532,#48533,#48534,#48535,#48536)) ;
#21415=EDGE_LOOP('',(#48537,#48538,#48539,#48540,#48541,#48542,#48543,#48544)) ;
#21416=EDGE_LOOP('',(#48545,#48546,#48547)) ;
#21417=EDGE_LOOP('',(#48548,#48549,#48550,#48551)) ;
#21418=EDGE_LOOP('',(#48552,#48553,#48554,#48555,#48556)) ;
#21419=EDGE_LOOP('',(#48557,#48558,#48559,#48560,#48561)) ;
#21420=EDGE_LOOP('',(#48562,#48563,#48564,#48565)) ;
#21421=EDGE_LOOP('',(#48566,#48567,#48568)) ;
#21422=EDGE_LOOP('',(#48569,#48570,#48571,#48572,#48573,#48574,#48575,#48576)) ;
#21423=EDGE_LOOP('',(#48577,#48578,#48579,#48580,#48581)) ;
#21424=EDGE_LOOP('',(#48582,#48583,#48584,#48585,#48586)) ;
#21425=EDGE_LOOP('',(#48587,#48588,#48589,#48590)) ;
#21426=EDGE_LOOP('',(#48591,#48592,#48593,#48594,#48595,#48596,#48597,#48598)) ;
#21427=EDGE_LOOP('',(#48599,#48600,#48601,#48602)) ;
#21428=EDGE_LOOP('',(#48603,#48604,#48605,#48606,#48607,#48608,#48609,#48610)) ;
#21429=EDGE_LOOP('',(#48611,#48612,#48613,#48614)) ;
#21430=EDGE_LOOP('',(#48615,#48616,#48617,#48618)) ;
#21431=EDGE_LOOP('',(#48619,#48620,#48621,#48622)) ;
#21432=EDGE_LOOP('',(#48623,#48624,#48625,#48626)) ;
#21433=EDGE_LOOP('',(#48627,#48628,#48629,#48630,#48631,#48632,#48633,#48634,
#48635)) ;
#21434=EDGE_LOOP('',(#48636,#48637,#48638,#48639,#48640,#48641,#48642)) ;
#21435=EDGE_LOOP('',(#48643,#48644,#48645,#48646)) ;
#21436=EDGE_LOOP('',(#48647,#48648,#48649,#48650)) ;
#21437=EDGE_LOOP('',(#48651,#48652,#48653,#48654)) ;
#21438=EDGE_LOOP('',(#48655,#48656,#48657)) ;
#21439=EDGE_LOOP('',(#48658,#48659,#48660,#48661)) ;
#21440=EDGE_LOOP('',(#48662,#48663,#48664,#48665)) ;
#21441=EDGE_LOOP('',(#48666,#48667,#48668,#48669)) ;
#21442=EDGE_LOOP('',(#48670,#48671,#48672,#48673)) ;
#21443=EDGE_LOOP('',(#48674,#48675,#48676,#48677)) ;
#21444=EDGE_LOOP('',(#48678,#48679,#48680,#48681)) ;
#21445=EDGE_LOOP('',(#48682,#48683,#48684,#48685)) ;
#21446=EDGE_LOOP('',(#48686,#48687,#48688,#48689)) ;
#21447=EDGE_LOOP('',(#48690,#48691,#48692,#48693)) ;
#21448=EDGE_LOOP('',(#48694,#48695,#48696,#48697)) ;
#21449=EDGE_LOOP('',(#48698,#48699,#48700,#48701)) ;
#21450=EDGE_LOOP('',(#48702,#48703,#48704,#48705)) ;
#21451=EDGE_LOOP('',(#48706,#48707,#48708,#48709)) ;
#21452=EDGE_LOOP('',(#48710,#48711,#48712,#48713)) ;
#21453=EDGE_LOOP('',(#48714,#48715,#48716,#48717)) ;
#21454=EDGE_LOOP('',(#48718,#48719,#48720,#48721)) ;
#21455=EDGE_LOOP('',(#48722,#48723,#48724,#48725)) ;
#21456=EDGE_LOOP('',(#48726,#48727,#48728,#48729)) ;
#21457=EDGE_LOOP('',(#48730,#48731,#48732,#48733)) ;
#21458=EDGE_LOOP('',(#48734,#48735,#48736)) ;
#21459=EDGE_LOOP('',(#48737,#48738,#48739,#48740)) ;
#21460=EDGE_LOOP('',(#48741,#48742,#48743,#48744,#48745,#48746)) ;
#21461=EDGE_LOOP('',(#48747,#48748,#48749,#48750)) ;
#21462=EDGE_LOOP('',(#48751,#48752,#48753,#48754,#48755)) ;
#21463=EDGE_LOOP('',(#48756,#48757,#48758,#48759)) ;
#21464=EDGE_LOOP('',(#48760,#48761,#48762,#48763,#48764)) ;
#21465=EDGE_LOOP('',(#48765,#48766,#48767,#48768,#48769)) ;
#21466=EDGE_LOOP('',(#48770,#48771,#48772,#48773)) ;
#21467=EDGE_LOOP('',(#48774,#48775,#48776,#48777)) ;
#21468=EDGE_LOOP('',(#48778,#48779,#48780,#48781,#48782)) ;
#21469=EDGE_LOOP('',(#48783,#48784,#48785,#48786)) ;
#21470=EDGE_LOOP('',(#48787,#48788,#48789,#48790)) ;
#21471=EDGE_LOOP('',(#48791,#48792,#48793,#48794)) ;
#21472=EDGE_LOOP('',(#48795,#48796,#48797,#48798,#48799,#48800,#48801,#48802,
#48803,#48804)) ;
#21473=EDGE_LOOP('',(#48805,#48806,#48807,#48808,#48809,#48810)) ;
#21474=EDGE_LOOP('',(#48811,#48812,#48813,#48814,#48815,#48816)) ;
#21475=EDGE_LOOP('',(#48817,#48818,#48819,#48820)) ;
#21476=EDGE_LOOP('',(#48821,#48822,#48823,#48824,#48825,#48826)) ;
#21477=EDGE_LOOP('',(#48827,#48828,#48829,#48830)) ;
#21478=EDGE_LOOP('',(#48831,#48832,#48833,#48834)) ;
#21479=EDGE_LOOP('',(#48835,#48836,#48837,#48838,#48839,#48840)) ;
#21480=EDGE_LOOP('',(#48841,#48842,#48843,#48844,#48845,#48846,#48847,#48848,
#48849,#48850,#48851,#48852,#48853,#48854,#48855,#48856,#48857,#48858,#48859,
#48860,#48861,#48862,#48863,#48864,#48865,#48866,#48867,#48868,#48869,#48870,
#48871,#48872,#48873)) ;
#21481=EDGE_LOOP('',(#48874,#48875,#48876,#48877,#48878,#48879,#48880,#48881,
#48882,#48883,#48884,#48885,#48886,#48887,#48888,#48889,#48890,#48891,#48892,
#48893,#48894,#48895,#48896,#48897,#48898,#48899,#48900,#48901,#48902,#48903,
#48904,#48905,#48906)) ;
#21482=EDGE_LOOP('',(#48907,#48908,#48909,#48910)) ;
#21483=EDGE_LOOP('',(#48911,#48912,#48913,#48914)) ;
#21484=EDGE_LOOP('',(#48915,#48916,#48917,#48918,#48919,#48920,#48921,#48922)) ;
#21485=EDGE_LOOP('',(#48923,#48924,#48925,#48926,#48927,#48928)) ;
#21486=EDGE_LOOP('',(#48929,#48930,#48931,#48932)) ;
#21487=EDGE_LOOP('',(#48933,#48934,#48935,#48936,#48937,#48938)) ;
#21488=EDGE_LOOP('',(#48939,#48940,#48941,#48942,#48943,#48944,#48945,#48946,
#48947,#48948,#48949,#48950,#48951,#48952)) ;
#21489=EDGE_LOOP('',(#48953,#48954,#48955,#48956,#48957,#48958,#48959,#48960,
#48961,#48962,#48963,#48964,#48965,#48966,#48967,#48968,#48969,#48970,#48971,
#48972,#48973,#48974,#48975,#48976)) ;
#21490=EDGE_LOOP('',(#48977)) ;
#21491=EDGE_LOOP('',(#48978,#48979,#48980,#48981,#48982,#48983,#48984,#48985,
#48986,#48987)) ;
#21492=EDGE_LOOP('',(#48988,#48989,#48990,#48991,#48992,#48993,#48994,#48995,
#48996,#48997)) ;
#21493=EDGE_LOOP('',(#48998,#48999,#49000)) ;
#21494=EDGE_LOOP('',(#49001,#49002,#49003)) ;
#21495=EDGE_LOOP('',(#49004,#49005,#49006,#49007,#49008,#49009,#49010,#49011)) ;
#21496=EDGE_LOOP('',(#49012,#49013,#49014,#49015)) ;
#21497=EDGE_LOOP('',(#49016,#49017,#49018,#49019)) ;
#21498=EDGE_LOOP('',(#49020,#49021,#49022,#49023)) ;
#21499=EDGE_LOOP('',(#49024,#49025,#49026,#49027,#49028,#49029)) ;
#21500=EDGE_LOOP('',(#49030,#49031,#49032,#49033,#49034,#49035,#49036,#49037)) ;
#21501=EDGE_LOOP('',(#49038)) ;
#21502=EDGE_LOOP('',(#49039,#49040,#49041,#49042,#49043,#49044,#49045,#49046)) ;
#21503=EDGE_LOOP('',(#49047,#49048,#49049,#49050,#49051,#49052,#49053)) ;
#21504=EDGE_LOOP('',(#49054,#49055,#49056,#49057)) ;
#21505=EDGE_LOOP('',(#49058,#49059,#49060,#49061)) ;
#21506=EDGE_LOOP('',(#49062,#49063,#49064,#49065)) ;
#21507=EDGE_LOOP('',(#49066,#49067,#49068,#49069)) ;
#21508=EDGE_LOOP('',(#49070,#49071,#49072,#49073)) ;
#21509=EDGE_LOOP('',(#49074,#49075,#49076,#49077)) ;
#21510=EDGE_LOOP('',(#49078,#49079,#49080,#49081,#49082,#49083,#49084)) ;
#21511=EDGE_LOOP('',(#49085,#49086,#49087,#49088,#49089)) ;
#21512=EDGE_LOOP('',(#49090,#49091,#49092,#49093)) ;
#21513=EDGE_LOOP('',(#49094,#49095,#49096,#49097)) ;
#21514=EDGE_LOOP('',(#49098,#49099,#49100,#49101)) ;
#21515=EDGE_LOOP('',(#49102,#49103,#49104,#49105)) ;
#21516=EDGE_LOOP('',(#49106,#49107,#49108,#49109)) ;
#21517=EDGE_LOOP('',(#49110,#49111,#49112,#49113)) ;
#21518=EDGE_LOOP('',(#49114,#49115,#49116,#49117,#49118)) ;
#21519=EDGE_LOOP('',(#49119,#49120,#49121,#49122)) ;
#21520=EDGE_LOOP('',(#49123,#49124,#49125,#49126,#49127,#49128,#49129,#49130)) ;
#21521=EDGE_LOOP('',(#49131,#49132,#49133,#49134)) ;
#21522=EDGE_LOOP('',(#49135,#49136,#49137,#49138)) ;
#21523=EDGE_LOOP('',(#49139,#49140,#49141,#49142)) ;
#21524=EDGE_LOOP('',(#49143,#49144,#49145,#49146)) ;
#21525=EDGE_LOOP('',(#49147,#49148,#49149,#49150)) ;
#21526=EDGE_LOOP('',(#49151,#49152,#49153,#49154)) ;
#21527=EDGE_LOOP('',(#49155,#49156,#49157,#49158)) ;
#21528=EDGE_LOOP('',(#49159,#49160,#49161,#49162)) ;
#21529=EDGE_LOOP('',(#49163,#49164,#49165,#49166,#49167,#49168)) ;
#21530=EDGE_LOOP('',(#49169,#49170,#49171,#49172,#49173,#49174)) ;
#21531=EDGE_LOOP('',(#49175,#49176,#49177,#49178)) ;
#21532=EDGE_LOOP('',(#49179,#49180,#49181,#49182)) ;
#21533=EDGE_LOOP('',(#49183,#49184,#49185,#49186)) ;
#21534=EDGE_LOOP('',(#49187,#49188,#49189,#49190)) ;
#21535=EDGE_LOOP('',(#49191,#49192,#49193,#49194)) ;
#21536=EDGE_LOOP('',(#49195,#49196,#49197,#49198)) ;
#21537=EDGE_LOOP('',(#49199,#49200,#49201,#49202)) ;
#21538=EDGE_LOOP('',(#49203,#49204,#49205,#49206)) ;
#21539=EDGE_LOOP('',(#49207,#49208,#49209,#49210)) ;
#21540=EDGE_LOOP('',(#49211,#49212,#49213,#49214)) ;
#21541=EDGE_LOOP('',(#49215,#49216,#49217,#49218)) ;
#21542=EDGE_LOOP('',(#49219,#49220,#49221,#49222)) ;
#21543=EDGE_LOOP('',(#49223,#49224,#49225,#49226)) ;
#21544=EDGE_LOOP('',(#49227,#49228,#49229,#49230)) ;
#21545=EDGE_LOOP('',(#49231,#49232,#49233,#49234)) ;
#21546=EDGE_LOOP('',(#49235,#49236,#49237)) ;
#21547=EDGE_LOOP('',(#49238,#49239,#49240,#49241)) ;
#21548=EDGE_LOOP('',(#49242,#49243,#49244,#49245)) ;
#21549=EDGE_LOOP('',(#49246,#49247,#49248,#49249)) ;
#21550=EDGE_LOOP('',(#49250,#49251,#49252,#49253)) ;
#21551=EDGE_LOOP('',(#49254,#49255,#49256)) ;
#21552=EDGE_LOOP('',(#49257,#49258,#49259,#49260)) ;
#21553=EDGE_LOOP('',(#49261,#49262,#49263,#49264)) ;
#21554=EDGE_LOOP('',(#49265,#49266,#49267,#49268)) ;
#21555=EDGE_LOOP('',(#49269,#49270,#49271,#49272)) ;
#21556=EDGE_LOOP('',(#49273,#49274,#49275,#49276)) ;
#21557=EDGE_LOOP('',(#49277,#49278,#49279,#49280)) ;
#21558=EDGE_LOOP('',(#49281,#49282,#49283,#49284)) ;
#21559=EDGE_LOOP('',(#49285,#49286,#49287)) ;
#21560=EDGE_LOOP('',(#49288,#49289,#49290,#49291)) ;
#21561=EDGE_LOOP('',(#49292,#49293,#49294,#49295)) ;
#21562=EDGE_LOOP('',(#49296,#49297,#49298)) ;
#21563=EDGE_LOOP('',(#49299,#49300,#49301,#49302)) ;
#21564=EDGE_LOOP('',(#49303,#49304,#49305,#49306)) ;
#21565=EDGE_LOOP('',(#49307,#49308,#49309,#49310)) ;
#21566=EDGE_LOOP('',(#49311,#49312,#49313,#49314)) ;
#21567=EDGE_LOOP('',(#49315,#49316,#49317,#49318)) ;
#21568=EDGE_LOOP('',(#49319,#49320,#49321)) ;
#21569=EDGE_LOOP('',(#49322,#49323,#49324,#49325)) ;
#21570=EDGE_LOOP('',(#49326,#49327,#49328,#49329)) ;
#21571=EDGE_LOOP('',(#49330,#49331,#49332,#49333)) ;
#21572=EDGE_LOOP('',(#49334,#49335,#49336,#49337)) ;
#21573=EDGE_LOOP('',(#49338,#49339,#49340,#49341)) ;
#21574=EDGE_LOOP('',(#49342,#49343,#49344,#49345)) ;
#21575=EDGE_LOOP('',(#49346,#49347,#49348)) ;
#21576=EDGE_LOOP('',(#49349,#49350,#49351,#49352)) ;
#21577=EDGE_LOOP('',(#49353,#49354,#49355,#49356)) ;
#21578=EDGE_LOOP('',(#49357,#49358,#49359)) ;
#21579=EDGE_LOOP('',(#49360,#49361,#49362,#49363,#49364)) ;
#21580=EDGE_LOOP('',(#49365,#49366,#49367,#49368,#49369)) ;
#21581=EDGE_LOOP('',(#49370,#49371,#49372,#49373)) ;
#21582=EDGE_LOOP('',(#49374,#49375,#49376,#49377,#49378,#49379)) ;
#21583=EDGE_LOOP('',(#49380,#49381,#49382,#49383,#49384,#49385)) ;
#21584=EDGE_LOOP('',(#49386,#49387,#49388,#49389)) ;
#21585=EDGE_LOOP('',(#49390,#49391,#49392,#49393)) ;
#21586=EDGE_LOOP('',(#49394,#49395,#49396)) ;
#21587=EDGE_LOOP('',(#49397,#49398,#49399,#49400,#49401)) ;
#21588=EDGE_LOOP('',(#49402,#49403,#49404,#49405,#49406)) ;
#21589=EDGE_LOOP('',(#49407,#49408,#49409,#49410)) ;
#21590=EDGE_LOOP('',(#49411,#49412,#49413,#49414,#49415)) ;
#21591=EDGE_LOOP('',(#49416,#49417,#49418,#49419)) ;
#21592=EDGE_LOOP('',(#49420,#49421,#49422,#49423)) ;
#21593=EDGE_LOOP('',(#49424,#49425,#49426)) ;
#21594=EDGE_LOOP('',(#49427,#49428,#49429)) ;
#21595=EDGE_LOOP('',(#49430,#49431,#49432,#49433,#49434)) ;
#21596=EDGE_LOOP('',(#49435,#49436,#49437,#49438)) ;
#21597=EDGE_LOOP('',(#49439,#49440,#49441)) ;
#21598=EDGE_LOOP('',(#49442,#49443,#49444,#49445)) ;
#21599=EDGE_LOOP('',(#49446,#49447,#49448,#49449)) ;
#21600=EDGE_LOOP('',(#49450,#49451,#49452,#49453)) ;
#21601=EDGE_LOOP('',(#49454,#49455,#49456,#49457)) ;
#21602=EDGE_LOOP('',(#49458,#49459,#49460,#49461)) ;
#21603=EDGE_LOOP('',(#49462,#49463,#49464,#49465)) ;
#21604=EDGE_LOOP('',(#49466,#49467,#49468)) ;
#21605=EDGE_LOOP('',(#49469,#49470,#49471,#49472)) ;
#21606=EDGE_LOOP('',(#49473,#49474,#49475,#49476,#49477)) ;
#21607=EDGE_LOOP('',(#49478,#49479,#49480,#49481)) ;
#21608=EDGE_LOOP('',(#49482,#49483,#49484,#49485)) ;
#21609=EDGE_LOOP('',(#49486,#49487,#49488,#49489,#49490)) ;
#21610=EDGE_LOOP('',(#49491,#49492,#49493,#49494)) ;
#21611=EDGE_LOOP('',(#49495,#49496,#49497)) ;
#21612=EDGE_LOOP('',(#49498,#49499,#49500,#49501)) ;
#21613=EDGE_LOOP('',(#49502,#49503,#49504,#49505)) ;
#21614=EDGE_LOOP('',(#49506,#49507,#49508,#49509)) ;
#21615=EDGE_LOOP('',(#49510,#49511,#49512,#49513)) ;
#21616=EDGE_LOOP('',(#49514,#49515,#49516,#49517)) ;
#21617=EDGE_LOOP('',(#49518,#49519,#49520,#49521)) ;
#21618=EDGE_LOOP('',(#49522,#49523,#49524)) ;
#21619=EDGE_LOOP('',(#49525,#49526,#49527,#49528)) ;
#21620=EDGE_LOOP('',(#49529,#49530,#49531,#49532)) ;
#21621=EDGE_LOOP('',(#49533,#49534,#49535,#49536)) ;
#21622=EDGE_LOOP('',(#49537,#49538,#49539,#49540)) ;
#21623=EDGE_LOOP('',(#49541,#49542,#49543,#49544)) ;
#21624=EDGE_LOOP('',(#49545,#49546,#49547,#49548)) ;
#21625=EDGE_LOOP('',(#49549,#49550,#49551,#49552)) ;
#21626=EDGE_LOOP('',(#49553,#49554,#49555,#49556)) ;
#21627=EDGE_LOOP('',(#49557,#49558,#49559,#49560)) ;
#21628=EDGE_LOOP('',(#49561,#49562,#49563)) ;
#21629=EDGE_LOOP('',(#49564,#49565,#49566,#49567)) ;
#21630=EDGE_LOOP('',(#49568,#49569,#49570)) ;
#21631=EDGE_LOOP('',(#49571,#49572,#49573,#49574)) ;
#21632=EDGE_LOOP('',(#49575,#49576,#49577,#49578)) ;
#21633=EDGE_LOOP('',(#49579,#49580,#49581,#49582)) ;
#21634=EDGE_LOOP('',(#49583,#49584,#49585,#49586)) ;
#21635=EDGE_LOOP('',(#49587,#49588,#49589,#49590)) ;
#21636=EDGE_LOOP('',(#49591,#49592,#49593,#49594)) ;
#21637=EDGE_LOOP('',(#49595,#49596,#49597,#49598)) ;
#21638=EDGE_LOOP('',(#49599,#49600,#49601,#49602,#49603,#49604)) ;
#21639=EDGE_LOOP('',(#49605,#49606,#49607)) ;
#21640=EDGE_LOOP('',(#49608,#49609,#49610,#49611)) ;
#21641=EDGE_LOOP('',(#49612,#49613,#49614,#49615)) ;
#21642=EDGE_LOOP('',(#49616,#49617,#49618,#49619)) ;
#21643=EDGE_LOOP('',(#49620,#49621,#49622,#49623)) ;
#21644=EDGE_LOOP('',(#49624,#49625,#49626,#49627)) ;
#21645=EDGE_LOOP('',(#49628,#49629,#49630,#49631)) ;
#21646=EDGE_LOOP('',(#49632,#49633,#49634,#49635)) ;
#21647=EDGE_LOOP('',(#49636,#49637,#49638,#49639,#49640)) ;
#21648=EDGE_LOOP('',(#49641,#49642,#49643,#49644)) ;
#21649=EDGE_LOOP('',(#49645,#49646,#49647,#49648,#49649)) ;
#21650=EDGE_LOOP('',(#49650,#49651,#49652,#49653)) ;
#21651=EDGE_LOOP('',(#49654,#49655,#49656,#49657,#49658)) ;
#21652=EDGE_LOOP('',(#49659,#49660,#49661,#49662)) ;
#21653=EDGE_LOOP('',(#49663,#49664,#49665)) ;
#21654=EDGE_LOOP('',(#49666,#49667,#49668,#49669)) ;
#21655=EDGE_LOOP('',(#49670,#49671,#49672,#49673)) ;
#21656=EDGE_LOOP('',(#49674,#49675,#49676,#49677)) ;
#21657=EDGE_LOOP('',(#49678,#49679,#49680,#49681)) ;
#21658=EDGE_LOOP('',(#49682,#49683,#49684,#49685)) ;
#21659=EDGE_LOOP('',(#49686,#49687,#49688)) ;
#21660=EDGE_LOOP('',(#49689,#49690,#49691)) ;
#21661=EDGE_LOOP('',(#49692,#49693,#49694,#49695)) ;
#21662=EDGE_LOOP('',(#49696,#49697,#49698,#49699)) ;
#21663=EDGE_LOOP('',(#49700,#49701,#49702)) ;
#21664=EDGE_LOOP('',(#49703,#49704,#49705,#49706)) ;
#21665=EDGE_LOOP('',(#49707,#49708,#49709,#49710)) ;
#21666=EDGE_LOOP('',(#49711,#49712,#49713,#49714,#49715)) ;
#21667=EDGE_LOOP('',(#49716,#49717,#49718,#49719)) ;
#21668=EDGE_LOOP('',(#49720,#49721,#49722,#49723)) ;
#21669=EDGE_LOOP('',(#49724,#49725,#49726,#49727)) ;
#21670=EDGE_LOOP('',(#49728,#49729,#49730,#49731)) ;
#21671=EDGE_LOOP('',(#49732,#49733,#49734,#49735)) ;
#21672=EDGE_LOOP('',(#49736,#49737,#49738)) ;
#21673=EDGE_LOOP('',(#49739,#49740,#49741,#49742)) ;
#21674=EDGE_LOOP('',(#49743,#49744,#49745,#49746)) ;
#21675=EDGE_LOOP('',(#49747,#49748,#49749)) ;
#21676=EDGE_LOOP('',(#49750,#49751,#49752,#49753)) ;
#21677=EDGE_LOOP('',(#49754,#49755,#49756,#49757)) ;
#21678=EDGE_LOOP('',(#49758,#49759,#49760,#49761)) ;
#21679=EDGE_LOOP('',(#49762,#49763,#49764,#49765)) ;
#21680=EDGE_LOOP('',(#49766,#49767,#49768)) ;
#21681=EDGE_LOOP('',(#49769,#49770,#49771)) ;
#21682=EDGE_LOOP('',(#49772,#49773,#49774,#49775)) ;
#21683=EDGE_LOOP('',(#49776,#49777,#49778,#49779)) ;
#21684=EDGE_LOOP('',(#49780,#49781,#49782,#49783)) ;
#21685=EDGE_LOOP('',(#49784,#49785,#49786)) ;
#21686=EDGE_LOOP('',(#49787,#49788,#49789,#49790)) ;
#21687=EDGE_LOOP('',(#49791,#49792,#49793,#49794)) ;
#21688=EDGE_LOOP('',(#49795,#49796,#49797)) ;
#21689=EDGE_LOOP('',(#49798,#49799,#49800,#49801)) ;
#21690=EDGE_LOOP('',(#49802,#49803,#49804,#49805,#49806)) ;
#21691=EDGE_LOOP('',(#49807,#49808,#49809,#49810)) ;
#21692=EDGE_LOOP('',(#49811,#49812,#49813)) ;
#21693=EDGE_LOOP('',(#49814,#49815,#49816,#49817)) ;
#21694=EDGE_LOOP('',(#49818,#49819,#49820,#49821)) ;
#21695=EDGE_LOOP('',(#49822,#49823,#49824)) ;
#21696=EDGE_LOOP('',(#49825,#49826,#49827,#49828,#49829)) ;
#21697=EDGE_LOOP('',(#49830,#49831,#49832,#49833)) ;
#21698=EDGE_LOOP('',(#49834,#49835,#49836,#49837)) ;
#21699=EDGE_LOOP('',(#49838,#49839,#49840,#49841)) ;
#21700=EDGE_LOOP('',(#49842,#49843,#49844,#49845)) ;
#21701=EDGE_LOOP('',(#49846,#49847,#49848,#49849)) ;
#21702=EDGE_LOOP('',(#49850,#49851,#49852,#49853)) ;
#21703=EDGE_LOOP('',(#49854,#49855,#49856,#49857)) ;
#21704=EDGE_LOOP('',(#49858,#49859,#49860,#49861)) ;
#21705=EDGE_LOOP('',(#49862,#49863,#49864,#49865,#49866)) ;
#21706=EDGE_LOOP('',(#49867,#49868,#49869,#49870,#49871,#49872,#49873,#49874)) ;
#21707=EDGE_LOOP('',(#49875,#49876,#49877)) ;
#21708=EDGE_LOOP('',(#49878,#49879,#49880,#49881)) ;
#21709=EDGE_LOOP('',(#49882,#49883,#49884,#49885,#49886)) ;
#21710=EDGE_LOOP('',(#49887,#49888,#49889,#49890,#49891)) ;
#21711=EDGE_LOOP('',(#49892,#49893,#49894,#49895)) ;
#21712=EDGE_LOOP('',(#49896,#49897,#49898)) ;
#21713=EDGE_LOOP('',(#49899,#49900,#49901,#49902,#49903,#49904,#49905,#49906)) ;
#21714=EDGE_LOOP('',(#49907,#49908,#49909,#49910,#49911)) ;
#21715=EDGE_LOOP('',(#49912,#49913,#49914,#49915,#49916)) ;
#21716=EDGE_LOOP('',(#49917,#49918,#49919,#49920)) ;
#21717=EDGE_LOOP('',(#49921,#49922,#49923,#49924,#49925,#49926,#49927,#49928)) ;
#21718=EDGE_LOOP('',(#49929,#49930,#49931,#49932)) ;
#21719=EDGE_LOOP('',(#49933,#49934,#49935,#49936,#49937,#49938,#49939,#49940)) ;
#21720=EDGE_LOOP('',(#49941,#49942,#49943,#49944)) ;
#21721=EDGE_LOOP('',(#49945,#49946,#49947,#49948)) ;
#21722=EDGE_LOOP('',(#49949,#49950,#49951,#49952)) ;
#21723=EDGE_LOOP('',(#49953,#49954,#49955,#49956)) ;
#21724=EDGE_LOOP('',(#49957,#49958,#49959,#49960,#49961,#49962,#49963,#49964,
#49965)) ;
#21725=EDGE_LOOP('',(#49966,#49967,#49968,#49969,#49970,#49971,#49972)) ;
#21726=EDGE_LOOP('',(#49973,#49974,#49975,#49976)) ;
#21727=EDGE_LOOP('',(#49977,#49978,#49979,#49980)) ;
#21728=EDGE_LOOP('',(#49981,#49982,#49983,#49984)) ;
#21729=EDGE_LOOP('',(#49985,#49986,#49987)) ;
#21730=EDGE_LOOP('',(#49988,#49989,#49990,#49991)) ;
#21731=EDGE_LOOP('',(#49992,#49993,#49994,#49995)) ;
#21732=EDGE_LOOP('',(#49996,#49997,#49998,#49999)) ;
#21733=EDGE_LOOP('',(#50000,#50001,#50002,#50003)) ;
#21734=EDGE_LOOP('',(#50004,#50005,#50006,#50007)) ;
#21735=EDGE_LOOP('',(#50008,#50009,#50010,#50011)) ;
#21736=EDGE_LOOP('',(#50012,#50013,#50014,#50015)) ;
#21737=EDGE_LOOP('',(#50016,#50017,#50018,#50019)) ;
#21738=EDGE_LOOP('',(#50020,#50021,#50022,#50023)) ;
#21739=EDGE_LOOP('',(#50024,#50025,#50026,#50027)) ;
#21740=EDGE_LOOP('',(#50028,#50029,#50030,#50031)) ;
#21741=EDGE_LOOP('',(#50032,#50033,#50034,#50035)) ;
#21742=EDGE_LOOP('',(#50036,#50037,#50038,#50039)) ;
#21743=EDGE_LOOP('',(#50040,#50041,#50042,#50043)) ;
#21744=EDGE_LOOP('',(#50044,#50045,#50046,#50047)) ;
#21745=EDGE_LOOP('',(#50048,#50049,#50050,#50051)) ;
#21746=EDGE_LOOP('',(#50052,#50053,#50054,#50055)) ;
#21747=EDGE_LOOP('',(#50056,#50057,#50058,#50059)) ;
#21748=EDGE_LOOP('',(#50060,#50061,#50062,#50063)) ;
#21749=EDGE_LOOP('',(#50064,#50065,#50066)) ;
#21750=EDGE_LOOP('',(#50067,#50068,#50069,#50070)) ;
#21751=EDGE_LOOP('',(#50071,#50072,#50073,#50074,#50075,#50076)) ;
#21752=EDGE_LOOP('',(#50077,#50078,#50079,#50080)) ;
#21753=EDGE_LOOP('',(#50081,#50082,#50083,#50084,#50085)) ;
#21754=EDGE_LOOP('',(#50086,#50087,#50088,#50089)) ;
#21755=EDGE_LOOP('',(#50090,#50091,#50092,#50093,#50094)) ;
#21756=EDGE_LOOP('',(#50095,#50096,#50097,#50098,#50099)) ;
#21757=EDGE_LOOP('',(#50100,#50101,#50102,#50103)) ;
#21758=EDGE_LOOP('',(#50104,#50105,#50106,#50107)) ;
#21759=EDGE_LOOP('',(#50108,#50109,#50110,#50111,#50112)) ;
#21760=EDGE_LOOP('',(#50113,#50114,#50115,#50116)) ;
#21761=EDGE_LOOP('',(#50117,#50118,#50119,#50120)) ;
#21762=EDGE_LOOP('',(#50121,#50122,#50123,#50124)) ;
#21763=EDGE_LOOP('',(#50125,#50126,#50127,#50128,#50129,#50130,#50131,#50132,
#50133,#50134)) ;
#21764=EDGE_LOOP('',(#50135,#50136,#50137,#50138,#50139,#50140)) ;
#21765=EDGE_LOOP('',(#50141,#50142,#50143,#50144,#50145,#50146)) ;
#21766=EDGE_LOOP('',(#50147,#50148,#50149,#50150)) ;
#21767=EDGE_LOOP('',(#50151,#50152,#50153,#50154,#50155,#50156)) ;
#21768=EDGE_LOOP('',(#50157,#50158,#50159,#50160)) ;
#21769=EDGE_LOOP('',(#50161,#50162,#50163,#50164)) ;
#21770=EDGE_LOOP('',(#50165,#50166,#50167,#50168,#50169,#50170)) ;
#21771=EDGE_LOOP('',(#50171,#50172,#50173,#50174,#50175,#50176,#50177,#50178,
#50179,#50180,#50181,#50182,#50183,#50184,#50185,#50186,#50187,#50188,#50189,
#50190,#50191,#50192,#50193,#50194,#50195,#50196,#50197,#50198,#50199,#50200,
#50201,#50202,#50203)) ;
#21772=EDGE_LOOP('',(#50204,#50205,#50206,#50207,#50208,#50209,#50210,#50211,
#50212,#50213,#50214,#50215,#50216,#50217,#50218,#50219,#50220,#50221,#50222,
#50223,#50224,#50225,#50226,#50227,#50228,#50229,#50230,#50231,#50232,#50233,
#50234,#50235,#50236)) ;
#21773=EDGE_LOOP('',(#50237,#50238,#50239,#50240)) ;
#21774=EDGE_LOOP('',(#50241,#50242,#50243,#50244)) ;
#21775=EDGE_LOOP('',(#50245,#50246,#50247,#50248,#50249,#50250,#50251,#50252)) ;
#21776=EDGE_LOOP('',(#50253,#50254,#50255,#50256,#50257,#50258)) ;
#21777=EDGE_LOOP('',(#50259,#50260,#50261,#50262)) ;
#21778=EDGE_LOOP('',(#50263,#50264,#50265,#50266,#50267,#50268)) ;
#21779=EDGE_LOOP('',(#50269,#50270,#50271,#50272,#50273,#50274,#50275,#50276,
#50277,#50278,#50279,#50280,#50281,#50282)) ;
#21780=EDGE_LOOP('',(#50283,#50284,#50285,#50286,#50287,#50288,#50289,#50290,
#50291,#50292,#50293,#50294,#50295,#50296,#50297,#50298,#50299,#50300,#50301,
#50302,#50303,#50304,#50305,#50306)) ;
#21781=EDGE_LOOP('',(#50307)) ;
#21782=EDGE_LOOP('',(#50308,#50309,#50310,#50311,#50312,#50313,#50314,#50315,
#50316,#50317)) ;
#21783=EDGE_LOOP('',(#50318,#50319,#50320,#50321,#50322,#50323,#50324,#50325,
#50326,#50327)) ;
#21784=EDGE_LOOP('',(#50328,#50329,#50330)) ;
#21785=EDGE_LOOP('',(#50331,#50332,#50333)) ;
#21786=EDGE_LOOP('',(#50334,#50335,#50336,#50337,#50338,#50339,#50340,#50341)) ;
#21787=EDGE_LOOP('',(#50342,#50343,#50344,#50345)) ;
#21788=EDGE_LOOP('',(#50346,#50347,#50348,#50349)) ;
#21789=EDGE_LOOP('',(#50350,#50351,#50352,#50353)) ;
#21790=EDGE_LOOP('',(#50354,#50355,#50356,#50357,#50358,#50359)) ;
#21791=EDGE_LOOP('',(#50360,#50361,#50362,#50363,#50364,#50365,#50366,#50367)) ;
#21792=EDGE_LOOP('',(#50368)) ;
#21793=EDGE_LOOP('',(#50369,#50370,#50371,#50372,#50373,#50374,#50375,#50376)) ;
#21794=EDGE_LOOP('',(#50377,#50378,#50379,#50380,#50381,#50382,#50383)) ;
#21795=EDGE_LOOP('',(#50384,#50385,#50386,#50387)) ;
#21796=EDGE_LOOP('',(#50388,#50389,#50390,#50391)) ;
#21797=EDGE_LOOP('',(#50392,#50393,#50394,#50395)) ;
#21798=EDGE_LOOP('',(#50396,#50397,#50398,#50399)) ;
#21799=EDGE_LOOP('',(#50400,#50401,#50402,#50403)) ;
#21800=EDGE_LOOP('',(#50404,#50405,#50406,#50407)) ;
#21801=EDGE_LOOP('',(#50408,#50409,#50410,#50411,#50412,#50413,#50414)) ;
#21802=EDGE_LOOP('',(#50415,#50416,#50417,#50418,#50419)) ;
#21803=EDGE_LOOP('',(#50420,#50421,#50422,#50423)) ;
#21804=EDGE_LOOP('',(#50424,#50425,#50426,#50427)) ;
#21805=EDGE_LOOP('',(#50428,#50429,#50430,#50431)) ;
#21806=EDGE_LOOP('',(#50432,#50433,#50434,#50435)) ;
#21807=EDGE_LOOP('',(#50436,#50437,#50438,#50439)) ;
#21808=EDGE_LOOP('',(#50440,#50441,#50442,#50443)) ;
#21809=EDGE_LOOP('',(#50444,#50445,#50446,#50447,#50448)) ;
#21810=EDGE_LOOP('',(#50449,#50450,#50451,#50452)) ;
#21811=EDGE_LOOP('',(#50453,#50454,#50455,#50456,#50457,#50458,#50459,#50460)) ;
#21812=EDGE_LOOP('',(#50461,#50462,#50463,#50464)) ;
#21813=EDGE_LOOP('',(#50465,#50466,#50467,#50468)) ;
#21814=EDGE_LOOP('',(#50469,#50470,#50471,#50472)) ;
#21815=EDGE_LOOP('',(#50473,#50474,#50475,#50476)) ;
#21816=EDGE_LOOP('',(#50477,#50478,#50479,#50480)) ;
#21817=EDGE_LOOP('',(#50481,#50482,#50483,#50484)) ;
#21818=EDGE_LOOP('',(#50485,#50486,#50487,#50488)) ;
#21819=EDGE_LOOP('',(#50489,#50490,#50491,#50492)) ;
#21820=EDGE_LOOP('',(#50493,#50494,#50495,#50496,#50497,#50498)) ;
#21821=EDGE_LOOP('',(#50499,#50500,#50501,#50502,#50503,#50504)) ;
#21822=EDGE_LOOP('',(#50505,#50506,#50507,#50508)) ;
#21823=EDGE_LOOP('',(#50509,#50510,#50511,#50512)) ;
#21824=EDGE_LOOP('',(#50513,#50514,#50515,#50516)) ;
#21825=EDGE_LOOP('',(#50517,#50518,#50519,#50520)) ;
#21826=EDGE_LOOP('',(#50521,#50522,#50523,#50524)) ;
#21827=EDGE_LOOP('',(#50525,#50526,#50527,#50528)) ;
#21828=EDGE_LOOP('',(#50529,#50530,#50531,#50532)) ;
#21829=EDGE_LOOP('',(#50533,#50534,#50535,#50536)) ;
#21830=EDGE_LOOP('',(#50537,#50538,#50539,#50540)) ;
#21831=EDGE_LOOP('',(#50541,#50542,#50543,#50544)) ;
#21832=EDGE_LOOP('',(#50545,#50546,#50547,#50548)) ;
#21833=EDGE_LOOP('',(#50549,#50550,#50551,#50552)) ;
#21834=EDGE_LOOP('',(#50553,#50554,#50555,#50556)) ;
#21835=EDGE_LOOP('',(#50557,#50558,#50559,#50560)) ;
#21836=EDGE_LOOP('',(#50561,#50562,#50563,#50564)) ;
#21837=EDGE_LOOP('',(#50565,#50566,#50567)) ;
#21838=EDGE_LOOP('',(#50568,#50569,#50570,#50571)) ;
#21839=EDGE_LOOP('',(#50572,#50573,#50574,#50575)) ;
#21840=EDGE_LOOP('',(#50576,#50577,#50578,#50579)) ;
#21841=EDGE_LOOP('',(#50580,#50581,#50582,#50583)) ;
#21842=EDGE_LOOP('',(#50584,#50585,#50586)) ;
#21843=EDGE_LOOP('',(#50587,#50588,#50589,#50590)) ;
#21844=EDGE_LOOP('',(#50591,#50592,#50593,#50594)) ;
#21845=EDGE_LOOP('',(#50595,#50596,#50597,#50598)) ;
#21846=EDGE_LOOP('',(#50599,#50600,#50601,#50602)) ;
#21847=EDGE_LOOP('',(#50603,#50604,#50605,#50606)) ;
#21848=EDGE_LOOP('',(#50607,#50608,#50609,#50610)) ;
#21849=EDGE_LOOP('',(#50611,#50612,#50613,#50614)) ;
#21850=EDGE_LOOP('',(#50615,#50616,#50617)) ;
#21851=EDGE_LOOP('',(#50618,#50619,#50620,#50621)) ;
#21852=EDGE_LOOP('',(#50622,#50623,#50624,#50625)) ;
#21853=EDGE_LOOP('',(#50626,#50627,#50628)) ;
#21854=EDGE_LOOP('',(#50629,#50630,#50631,#50632)) ;
#21855=EDGE_LOOP('',(#50633,#50634,#50635,#50636)) ;
#21856=EDGE_LOOP('',(#50637,#50638,#50639,#50640)) ;
#21857=EDGE_LOOP('',(#50641,#50642,#50643,#50644)) ;
#21858=EDGE_LOOP('',(#50645,#50646,#50647,#50648)) ;
#21859=EDGE_LOOP('',(#50649,#50650,#50651)) ;
#21860=EDGE_LOOP('',(#50652,#50653,#50654,#50655)) ;
#21861=EDGE_LOOP('',(#50656,#50657,#50658,#50659)) ;
#21862=EDGE_LOOP('',(#50660,#50661,#50662,#50663)) ;
#21863=EDGE_LOOP('',(#50664,#50665,#50666,#50667)) ;
#21864=EDGE_LOOP('',(#50668,#50669,#50670,#50671)) ;
#21865=EDGE_LOOP('',(#50672,#50673,#50674,#50675)) ;
#21866=EDGE_LOOP('',(#50676,#50677,#50678)) ;
#21867=EDGE_LOOP('',(#50679,#50680,#50681,#50682)) ;
#21868=EDGE_LOOP('',(#50683,#50684,#50685,#50686)) ;
#21869=EDGE_LOOP('',(#50687,#50688,#50689)) ;
#21870=EDGE_LOOP('',(#50690,#50691,#50692,#50693,#50694)) ;
#21871=EDGE_LOOP('',(#50695,#50696,#50697,#50698,#50699)) ;
#21872=EDGE_LOOP('',(#50700,#50701,#50702,#50703)) ;
#21873=EDGE_LOOP('',(#50704,#50705,#50706,#50707,#50708,#50709)) ;
#21874=EDGE_LOOP('',(#50710,#50711,#50712,#50713,#50714,#50715)) ;
#21875=EDGE_LOOP('',(#50716,#50717,#50718,#50719)) ;
#21876=EDGE_LOOP('',(#50720,#50721,#50722,#50723)) ;
#21877=EDGE_LOOP('',(#50724,#50725,#50726)) ;
#21878=EDGE_LOOP('',(#50727,#50728,#50729,#50730,#50731)) ;
#21879=EDGE_LOOP('',(#50732,#50733,#50734,#50735,#50736)) ;
#21880=EDGE_LOOP('',(#50737,#50738,#50739,#50740)) ;
#21881=EDGE_LOOP('',(#50741,#50742,#50743,#50744,#50745)) ;
#21882=EDGE_LOOP('',(#50746,#50747,#50748,#50749)) ;
#21883=EDGE_LOOP('',(#50750,#50751,#50752,#50753)) ;
#21884=EDGE_LOOP('',(#50754,#50755,#50756)) ;
#21885=EDGE_LOOP('',(#50757,#50758,#50759)) ;
#21886=EDGE_LOOP('',(#50760,#50761,#50762,#50763,#50764)) ;
#21887=EDGE_LOOP('',(#50765,#50766,#50767,#50768)) ;
#21888=EDGE_LOOP('',(#50769,#50770,#50771)) ;
#21889=EDGE_LOOP('',(#50772,#50773,#50774,#50775)) ;
#21890=EDGE_LOOP('',(#50776,#50777,#50778,#50779)) ;
#21891=EDGE_LOOP('',(#50780,#50781,#50782,#50783)) ;
#21892=EDGE_LOOP('',(#50784,#50785,#50786,#50787)) ;
#21893=EDGE_LOOP('',(#50788,#50789,#50790,#50791)) ;
#21894=EDGE_LOOP('',(#50792,#50793,#50794,#50795)) ;
#21895=EDGE_LOOP('',(#50796,#50797,#50798)) ;
#21896=EDGE_LOOP('',(#50799,#50800,#50801,#50802)) ;
#21897=EDGE_LOOP('',(#50803,#50804,#50805,#50806,#50807)) ;
#21898=EDGE_LOOP('',(#50808,#50809,#50810,#50811)) ;
#21899=EDGE_LOOP('',(#50812,#50813,#50814,#50815)) ;
#21900=EDGE_LOOP('',(#50816,#50817,#50818,#50819,#50820)) ;
#21901=EDGE_LOOP('',(#50821,#50822,#50823,#50824)) ;
#21902=EDGE_LOOP('',(#50825,#50826,#50827)) ;
#21903=EDGE_LOOP('',(#50828,#50829,#50830,#50831)) ;
#21904=EDGE_LOOP('',(#50832,#50833,#50834,#50835)) ;
#21905=EDGE_LOOP('',(#50836,#50837,#50838,#50839)) ;
#21906=EDGE_LOOP('',(#50840,#50841,#50842,#50843)) ;
#21907=EDGE_LOOP('',(#50844,#50845,#50846,#50847)) ;
#21908=EDGE_LOOP('',(#50848,#50849,#50850,#50851)) ;
#21909=EDGE_LOOP('',(#50852,#50853,#50854)) ;
#21910=EDGE_LOOP('',(#50855,#50856,#50857,#50858)) ;
#21911=EDGE_LOOP('',(#50859,#50860,#50861,#50862)) ;
#21912=EDGE_LOOP('',(#50863,#50864,#50865,#50866)) ;
#21913=EDGE_LOOP('',(#50867,#50868,#50869,#50870)) ;
#21914=EDGE_LOOP('',(#50871,#50872,#50873,#50874)) ;
#21915=EDGE_LOOP('',(#50875,#50876,#50877,#50878)) ;
#21916=EDGE_LOOP('',(#50879,#50880,#50881,#50882)) ;
#21917=EDGE_LOOP('',(#50883,#50884,#50885,#50886)) ;
#21918=EDGE_LOOP('',(#50887,#50888,#50889,#50890)) ;
#21919=EDGE_LOOP('',(#50891,#50892,#50893)) ;
#21920=EDGE_LOOP('',(#50894,#50895,#50896,#50897)) ;
#21921=EDGE_LOOP('',(#50898,#50899,#50900)) ;
#21922=EDGE_LOOP('',(#50901,#50902,#50903,#50904)) ;
#21923=EDGE_LOOP('',(#50905,#50906,#50907,#50908)) ;
#21924=EDGE_LOOP('',(#50909,#50910,#50911,#50912)) ;
#21925=EDGE_LOOP('',(#50913,#50914,#50915,#50916)) ;
#21926=EDGE_LOOP('',(#50917,#50918,#50919,#50920)) ;
#21927=EDGE_LOOP('',(#50921,#50922,#50923,#50924)) ;
#21928=EDGE_LOOP('',(#50925,#50926,#50927,#50928)) ;
#21929=EDGE_LOOP('',(#50929,#50930,#50931,#50932,#50933,#50934)) ;
#21930=EDGE_LOOP('',(#50935,#50936,#50937)) ;
#21931=EDGE_LOOP('',(#50938,#50939,#50940,#50941)) ;
#21932=EDGE_LOOP('',(#50942,#50943,#50944,#50945)) ;
#21933=EDGE_LOOP('',(#50946,#50947,#50948,#50949)) ;
#21934=EDGE_LOOP('',(#50950,#50951,#50952,#50953)) ;
#21935=EDGE_LOOP('',(#50954,#50955,#50956,#50957)) ;
#21936=EDGE_LOOP('',(#50958,#50959,#50960,#50961)) ;
#21937=EDGE_LOOP('',(#50962,#50963,#50964,#50965)) ;
#21938=EDGE_LOOP('',(#50966,#50967,#50968,#50969,#50970)) ;
#21939=EDGE_LOOP('',(#50971,#50972,#50973,#50974)) ;
#21940=EDGE_LOOP('',(#50975,#50976,#50977,#50978,#50979)) ;
#21941=EDGE_LOOP('',(#50980,#50981,#50982,#50983)) ;
#21942=EDGE_LOOP('',(#50984,#50985,#50986,#50987,#50988)) ;
#21943=EDGE_LOOP('',(#50989,#50990,#50991,#50992)) ;
#21944=EDGE_LOOP('',(#50993,#50994,#50995)) ;
#21945=EDGE_LOOP('',(#50996,#50997,#50998,#50999)) ;
#21946=EDGE_LOOP('',(#51000,#51001,#51002,#51003)) ;
#21947=EDGE_LOOP('',(#51004,#51005,#51006,#51007)) ;
#21948=EDGE_LOOP('',(#51008,#51009,#51010,#51011)) ;
#21949=EDGE_LOOP('',(#51012,#51013,#51014,#51015)) ;
#21950=EDGE_LOOP('',(#51016,#51017,#51018)) ;
#21951=EDGE_LOOP('',(#51019,#51020,#51021)) ;
#21952=EDGE_LOOP('',(#51022,#51023,#51024,#51025)) ;
#21953=EDGE_LOOP('',(#51026,#51027,#51028,#51029)) ;
#21954=EDGE_LOOP('',(#51030,#51031,#51032)) ;
#21955=EDGE_LOOP('',(#51033,#51034,#51035,#51036)) ;
#21956=EDGE_LOOP('',(#51037,#51038,#51039,#51040)) ;
#21957=EDGE_LOOP('',(#51041,#51042,#51043,#51044,#51045)) ;
#21958=EDGE_LOOP('',(#51046,#51047,#51048,#51049)) ;
#21959=EDGE_LOOP('',(#51050,#51051,#51052,#51053)) ;
#21960=EDGE_LOOP('',(#51054,#51055,#51056,#51057)) ;
#21961=EDGE_LOOP('',(#51058,#51059,#51060,#51061)) ;
#21962=EDGE_LOOP('',(#51062,#51063,#51064,#51065)) ;
#21963=EDGE_LOOP('',(#51066,#51067,#51068)) ;
#21964=EDGE_LOOP('',(#51069,#51070,#51071,#51072)) ;
#21965=EDGE_LOOP('',(#51073,#51074,#51075,#51076)) ;
#21966=EDGE_LOOP('',(#51077,#51078,#51079)) ;
#21967=EDGE_LOOP('',(#51080,#51081,#51082,#51083)) ;
#21968=EDGE_LOOP('',(#51084,#51085,#51086,#51087)) ;
#21969=EDGE_LOOP('',(#51088,#51089,#51090,#51091)) ;
#21970=EDGE_LOOP('',(#51092,#51093,#51094,#51095)) ;
#21971=EDGE_LOOP('',(#51096,#51097,#51098)) ;
#21972=EDGE_LOOP('',(#51099,#51100,#51101)) ;
#21973=EDGE_LOOP('',(#51102,#51103,#51104,#51105)) ;
#21974=EDGE_LOOP('',(#51106,#51107,#51108,#51109)) ;
#21975=EDGE_LOOP('',(#51110,#51111,#51112,#51113)) ;
#21976=EDGE_LOOP('',(#51114,#51115,#51116)) ;
#21977=EDGE_LOOP('',(#51117,#51118,#51119,#51120)) ;
#21978=EDGE_LOOP('',(#51121,#51122,#51123,#51124)) ;
#21979=EDGE_LOOP('',(#51125,#51126,#51127)) ;
#21980=EDGE_LOOP('',(#51128,#51129,#51130,#51131)) ;
#21981=EDGE_LOOP('',(#51132,#51133,#51134,#51135,#51136)) ;
#21982=EDGE_LOOP('',(#51137,#51138,#51139,#51140)) ;
#21983=EDGE_LOOP('',(#51141,#51142,#51143)) ;
#21984=EDGE_LOOP('',(#51144,#51145,#51146,#51147)) ;
#21985=EDGE_LOOP('',(#51148,#51149,#51150,#51151)) ;
#21986=EDGE_LOOP('',(#51152,#51153,#51154)) ;
#21987=EDGE_LOOP('',(#51155,#51156,#51157,#51158,#51159)) ;
#21988=EDGE_LOOP('',(#51160,#51161,#51162,#51163)) ;
#21989=EDGE_LOOP('',(#51164,#51165,#51166,#51167)) ;
#21990=EDGE_LOOP('',(#51168,#51169,#51170,#51171)) ;
#21991=EDGE_LOOP('',(#51172,#51173,#51174,#51175)) ;
#21992=EDGE_LOOP('',(#51176,#51177,#51178,#51179)) ;
#21993=EDGE_LOOP('',(#51180,#51181,#51182,#51183)) ;
#21994=EDGE_LOOP('',(#51184,#51185,#51186,#51187)) ;
#21995=EDGE_LOOP('',(#51188,#51189,#51190,#51191)) ;
#21996=EDGE_LOOP('',(#51192,#51193,#51194,#51195,#51196)) ;
#21997=EDGE_LOOP('',(#51197,#51198,#51199,#51200,#51201,#51202,#51203,#51204)) ;
#21998=EDGE_LOOP('',(#51205,#51206,#51207)) ;
#21999=EDGE_LOOP('',(#51208,#51209,#51210,#51211)) ;
#22000=EDGE_LOOP('',(#51212,#51213,#51214,#51215,#51216)) ;
#22001=EDGE_LOOP('',(#51217,#51218,#51219,#51220,#51221)) ;
#22002=EDGE_LOOP('',(#51222,#51223,#51224,#51225)) ;
#22003=EDGE_LOOP('',(#51226,#51227,#51228)) ;
#22004=EDGE_LOOP('',(#51229,#51230,#51231,#51232,#51233,#51234,#51235,#51236)) ;
#22005=EDGE_LOOP('',(#51237,#51238,#51239,#51240,#51241)) ;
#22006=EDGE_LOOP('',(#51242,#51243,#51244,#51245,#51246)) ;
#22007=EDGE_LOOP('',(#51247,#51248,#51249,#51250)) ;
#22008=EDGE_LOOP('',(#51251,#51252,#51253,#51254,#51255,#51256,#51257,#51258)) ;
#22009=EDGE_LOOP('',(#51259,#51260,#51261,#51262)) ;
#22010=EDGE_LOOP('',(#51263,#51264,#51265,#51266,#51267,#51268,#51269,#51270)) ;
#22011=EDGE_LOOP('',(#51271,#51272,#51273,#51274)) ;
#22012=EDGE_LOOP('',(#51275,#51276,#51277,#51278)) ;
#22013=EDGE_LOOP('',(#51279,#51280,#51281,#51282)) ;
#22014=EDGE_LOOP('',(#51283,#51284,#51285,#51286)) ;
#22015=EDGE_LOOP('',(#51287,#51288,#51289,#51290,#51291,#51292,#51293,#51294,
#51295)) ;
#22016=EDGE_LOOP('',(#51296,#51297,#51298,#51299,#51300,#51301,#51302)) ;
#22017=EDGE_LOOP('',(#51303,#51304,#51305,#51306)) ;
#22018=EDGE_LOOP('',(#51307,#51308,#51309,#51310)) ;
#22019=EDGE_LOOP('',(#51311,#51312,#51313,#51314)) ;
#22020=EDGE_LOOP('',(#51315,#51316,#51317)) ;
#22021=EDGE_LOOP('',(#51318,#51319,#51320,#51321)) ;
#22022=EDGE_LOOP('',(#51322,#51323,#51324,#51325)) ;
#22023=EDGE_LOOP('',(#51326,#51327,#51328,#51329)) ;
#22024=EDGE_LOOP('',(#51330,#51331,#51332,#51333)) ;
#22025=EDGE_LOOP('',(#51334,#51335,#51336,#51337)) ;
#22026=EDGE_LOOP('',(#51338,#51339,#51340,#51341)) ;
#22027=EDGE_LOOP('',(#51342,#51343,#51344,#51345)) ;
#22028=EDGE_LOOP('',(#51346,#51347,#51348,#51349)) ;
#22029=EDGE_LOOP('',(#51350,#51351,#51352,#51353)) ;
#22030=EDGE_LOOP('',(#51354,#51355,#51356,#51357)) ;
#22031=EDGE_LOOP('',(#51358,#51359,#51360,#51361)) ;
#22032=EDGE_LOOP('',(#51362,#51363,#51364,#51365)) ;
#22033=EDGE_LOOP('',(#51366,#51367,#51368,#51369)) ;
#22034=EDGE_LOOP('',(#51370,#51371,#51372,#51373)) ;
#22035=EDGE_LOOP('',(#51374,#51375,#51376,#51377)) ;
#22036=EDGE_LOOP('',(#51378,#51379,#51380,#51381)) ;
#22037=EDGE_LOOP('',(#51382,#51383,#51384,#51385)) ;
#22038=EDGE_LOOP('',(#51386,#51387,#51388,#51389)) ;
#22039=EDGE_LOOP('',(#51390,#51391,#51392,#51393)) ;
#22040=EDGE_LOOP('',(#51394,#51395,#51396)) ;
#22041=EDGE_LOOP('',(#51397,#51398,#51399,#51400)) ;
#22042=EDGE_LOOP('',(#51401,#51402,#51403,#51404,#51405,#51406)) ;
#22043=EDGE_LOOP('',(#51407,#51408,#51409,#51410)) ;
#22044=EDGE_LOOP('',(#51411,#51412,#51413,#51414,#51415)) ;
#22045=EDGE_LOOP('',(#51416,#51417,#51418,#51419)) ;
#22046=EDGE_LOOP('',(#51420,#51421,#51422,#51423,#51424)) ;
#22047=EDGE_LOOP('',(#51425,#51426,#51427,#51428,#51429)) ;
#22048=EDGE_LOOP('',(#51430,#51431,#51432,#51433)) ;
#22049=EDGE_LOOP('',(#51434,#51435,#51436,#51437)) ;
#22050=EDGE_LOOP('',(#51438,#51439,#51440,#51441,#51442)) ;
#22051=EDGE_LOOP('',(#51443,#51444,#51445,#51446)) ;
#22052=EDGE_LOOP('',(#51447,#51448,#51449,#51450)) ;
#22053=EDGE_LOOP('',(#51451,#51452,#51453,#51454)) ;
#22054=EDGE_LOOP('',(#51455,#51456,#51457,#51458,#51459,#51460,#51461,#51462,
#51463,#51464)) ;
#22055=EDGE_LOOP('',(#51465,#51466,#51467,#51468,#51469,#51470)) ;
#22056=EDGE_LOOP('',(#51471,#51472,#51473,#51474,#51475,#51476)) ;
#22057=EDGE_LOOP('',(#51477,#51478,#51479,#51480)) ;
#22058=EDGE_LOOP('',(#51481,#51482,#51483,#51484,#51485,#51486)) ;
#22059=EDGE_LOOP('',(#51487,#51488,#51489,#51490)) ;
#22060=EDGE_LOOP('',(#51491,#51492,#51493,#51494)) ;
#22061=EDGE_LOOP('',(#51495,#51496,#51497,#51498,#51499,#51500)) ;
#22062=EDGE_LOOP('',(#51501,#51502,#51503,#51504,#51505,#51506,#51507,#51508,
#51509,#51510,#51511,#51512,#51513,#51514,#51515,#51516,#51517,#51518,#51519,
#51520,#51521,#51522,#51523,#51524,#51525,#51526,#51527,#51528,#51529,#51530,
#51531,#51532,#51533)) ;
#22063=EDGE_LOOP('',(#51534,#51535,#51536,#51537,#51538,#51539,#51540,#51541,
#51542,#51543,#51544,#51545,#51546,#51547,#51548,#51549,#51550,#51551,#51552,
#51553,#51554,#51555,#51556,#51557,#51558,#51559,#51560,#51561,#51562,#51563,
#51564,#51565,#51566)) ;
#22064=EDGE_LOOP('',(#51567,#51568,#51569,#51570)) ;
#22065=EDGE_LOOP('',(#51571,#51572,#51573,#51574)) ;
#22066=EDGE_LOOP('',(#51575,#51576,#51577,#51578,#51579,#51580,#51581,#51582)) ;
#22067=EDGE_LOOP('',(#51583,#51584,#51585,#51586,#51587,#51588)) ;
#22068=EDGE_LOOP('',(#51589,#51590,#51591,#51592)) ;
#22069=EDGE_LOOP('',(#51593,#51594,#51595,#51596,#51597,#51598)) ;
#22070=EDGE_LOOP('',(#51599,#51600,#51601,#51602,#51603,#51604,#51605,#51606,
#51607,#51608,#51609,#51610,#51611,#51612)) ;
#22071=EDGE_LOOP('',(#51613,#51614,#51615,#51616,#51617,#51618,#51619,#51620,
#51621,#51622,#51623,#51624,#51625,#51626,#51627,#51628,#51629,#51630,#51631,
#51632,#51633,#51634,#51635,#51636)) ;
#22072=EDGE_LOOP('',(#51637)) ;
#22073=EDGE_LOOP('',(#51638,#51639,#51640,#51641,#51642,#51643,#51644,#51645,
#51646,#51647)) ;
#22074=EDGE_LOOP('',(#51648,#51649,#51650,#51651,#51652,#51653,#51654,#51655,
#51656,#51657)) ;
#22075=EDGE_LOOP('',(#51658,#51659,#51660)) ;
#22076=EDGE_LOOP('',(#51661,#51662,#51663)) ;
#22077=EDGE_LOOP('',(#51664,#51665,#51666,#51667,#51668,#51669,#51670,#51671)) ;
#22078=EDGE_LOOP('',(#51672,#51673,#51674,#51675)) ;
#22079=EDGE_LOOP('',(#51676,#51677,#51678,#51679)) ;
#22080=EDGE_LOOP('',(#51680,#51681,#51682,#51683)) ;
#22081=EDGE_LOOP('',(#51684,#51685,#51686,#51687,#51688,#51689)) ;
#22082=EDGE_LOOP('',(#51690,#51691,#51692,#51693,#51694,#51695,#51696,#51697)) ;
#22083=EDGE_LOOP('',(#51698)) ;
#22084=EDGE_LOOP('',(#51699,#51700,#51701,#51702,#51703,#51704,#51705,#51706)) ;
#22085=EDGE_LOOP('',(#51707,#51708,#51709,#51710,#51711,#51712,#51713)) ;
#22086=EDGE_LOOP('',(#51714,#51715,#51716,#51717)) ;
#22087=EDGE_LOOP('',(#51718,#51719,#51720,#51721)) ;
#22088=EDGE_LOOP('',(#51722,#51723,#51724,#51725)) ;
#22089=EDGE_LOOP('',(#51726,#51727,#51728,#51729)) ;
#22090=EDGE_LOOP('',(#51730,#51731,#51732,#51733)) ;
#22091=EDGE_LOOP('',(#51734,#51735,#51736,#51737)) ;
#22092=EDGE_LOOP('',(#51738,#51739,#51740,#51741,#51742,#51743,#51744)) ;
#22093=EDGE_LOOP('',(#51745,#51746,#51747,#51748,#51749)) ;
#22094=EDGE_LOOP('',(#51750,#51751,#51752,#51753)) ;
#22095=EDGE_LOOP('',(#51754,#51755,#51756,#51757)) ;
#22096=EDGE_LOOP('',(#51758,#51759,#51760,#51761)) ;
#22097=EDGE_LOOP('',(#51762,#51763,#51764,#51765)) ;
#22098=EDGE_LOOP('',(#51766,#51767,#51768,#51769)) ;
#22099=EDGE_LOOP('',(#51770,#51771,#51772,#51773)) ;
#22100=EDGE_LOOP('',(#51774,#51775,#51776,#51777,#51778)) ;
#22101=EDGE_LOOP('',(#51779,#51780,#51781,#51782)) ;
#22102=EDGE_LOOP('',(#51783,#51784,#51785,#51786,#51787,#51788,#51789,#51790)) ;
#22103=EDGE_LOOP('',(#51791,#51792,#51793,#51794)) ;
#22104=EDGE_LOOP('',(#51795,#51796,#51797,#51798)) ;
#22105=EDGE_LOOP('',(#51799,#51800,#51801,#51802)) ;
#22106=EDGE_LOOP('',(#51803,#51804,#51805,#51806)) ;
#22107=EDGE_LOOP('',(#51807,#51808,#51809,#51810)) ;
#22108=EDGE_LOOP('',(#51811,#51812,#51813,#51814)) ;
#22109=EDGE_LOOP('',(#51815,#51816,#51817,#51818)) ;
#22110=EDGE_LOOP('',(#51819,#51820,#51821,#51822)) ;
#22111=EDGE_LOOP('',(#51823,#51824,#51825,#51826,#51827,#51828)) ;
#22112=EDGE_LOOP('',(#51829,#51830,#51831,#51832,#51833,#51834)) ;
#22113=EDGE_LOOP('',(#51835,#51836,#51837,#51838)) ;
#22114=EDGE_LOOP('',(#51839,#51840,#51841,#51842)) ;
#22115=EDGE_LOOP('',(#51843,#51844,#51845,#51846)) ;
#22116=EDGE_LOOP('',(#51847,#51848,#51849,#51850)) ;
#22117=EDGE_LOOP('',(#51851,#51852,#51853,#51854)) ;
#22118=EDGE_LOOP('',(#51855,#51856,#51857,#51858)) ;
#22119=EDGE_LOOP('',(#51859,#51860,#51861,#51862)) ;
#22120=EDGE_LOOP('',(#51863,#51864,#51865,#51866)) ;
#22121=EDGE_LOOP('',(#51867,#51868,#51869,#51870)) ;
#22122=EDGE_LOOP('',(#51871,#51872,#51873,#51874)) ;
#22123=EDGE_LOOP('',(#51875,#51876,#51877,#51878)) ;
#22124=EDGE_LOOP('',(#51879,#51880,#51881,#51882)) ;
#22125=EDGE_LOOP('',(#51883,#51884,#51885,#51886)) ;
#22126=EDGE_LOOP('',(#51887,#51888,#51889,#51890)) ;
#22127=EDGE_LOOP('',(#51891,#51892,#51893,#51894)) ;
#22128=EDGE_LOOP('',(#51895,#51896,#51897)) ;
#22129=EDGE_LOOP('',(#51898,#51899,#51900,#51901)) ;
#22130=EDGE_LOOP('',(#51902,#51903,#51904,#51905)) ;
#22131=EDGE_LOOP('',(#51906,#51907,#51908,#51909)) ;
#22132=EDGE_LOOP('',(#51910,#51911,#51912,#51913)) ;
#22133=EDGE_LOOP('',(#51914,#51915,#51916)) ;
#22134=EDGE_LOOP('',(#51917,#51918,#51919,#51920)) ;
#22135=EDGE_LOOP('',(#51921,#51922,#51923,#51924)) ;
#22136=EDGE_LOOP('',(#51925,#51926,#51927,#51928)) ;
#22137=EDGE_LOOP('',(#51929,#51930,#51931,#51932)) ;
#22138=EDGE_LOOP('',(#51933,#51934,#51935,#51936)) ;
#22139=EDGE_LOOP('',(#51937,#51938,#51939,#51940)) ;
#22140=EDGE_LOOP('',(#51941,#51942,#51943,#51944)) ;
#22141=EDGE_LOOP('',(#51945,#51946,#51947)) ;
#22142=EDGE_LOOP('',(#51948,#51949,#51950,#51951)) ;
#22143=EDGE_LOOP('',(#51952,#51953,#51954,#51955)) ;
#22144=EDGE_LOOP('',(#51956,#51957,#51958)) ;
#22145=EDGE_LOOP('',(#51959,#51960,#51961,#51962)) ;
#22146=EDGE_LOOP('',(#51963,#51964,#51965,#51966)) ;
#22147=EDGE_LOOP('',(#51967,#51968,#51969,#51970)) ;
#22148=EDGE_LOOP('',(#51971,#51972,#51973,#51974)) ;
#22149=EDGE_LOOP('',(#51975,#51976,#51977,#51978)) ;
#22150=EDGE_LOOP('',(#51979,#51980,#51981)) ;
#22151=EDGE_LOOP('',(#51982,#51983,#51984,#51985)) ;
#22152=EDGE_LOOP('',(#51986,#51987,#51988,#51989)) ;
#22153=EDGE_LOOP('',(#51990,#51991,#51992,#51993)) ;
#22154=EDGE_LOOP('',(#51994,#51995,#51996,#51997)) ;
#22155=EDGE_LOOP('',(#51998,#51999,#52000,#52001)) ;
#22156=EDGE_LOOP('',(#52002,#52003,#52004,#52005)) ;
#22157=EDGE_LOOP('',(#52006,#52007,#52008)) ;
#22158=EDGE_LOOP('',(#52009,#52010,#52011,#52012)) ;
#22159=EDGE_LOOP('',(#52013,#52014,#52015,#52016)) ;
#22160=EDGE_LOOP('',(#52017,#52018,#52019)) ;
#22161=EDGE_LOOP('',(#52020,#52021,#52022,#52023,#52024)) ;
#22162=EDGE_LOOP('',(#52025,#52026,#52027,#52028,#52029)) ;
#22163=EDGE_LOOP('',(#52030,#52031,#52032,#52033)) ;
#22164=EDGE_LOOP('',(#52034,#52035,#52036,#52037,#52038,#52039)) ;
#22165=EDGE_LOOP('',(#52040,#52041,#52042,#52043,#52044,#52045)) ;
#22166=EDGE_LOOP('',(#52046,#52047,#52048,#52049)) ;
#22167=EDGE_LOOP('',(#52050,#52051,#52052,#52053)) ;
#22168=EDGE_LOOP('',(#52054,#52055,#52056)) ;
#22169=EDGE_LOOP('',(#52057,#52058,#52059,#52060,#52061)) ;
#22170=EDGE_LOOP('',(#52062,#52063,#52064,#52065,#52066)) ;
#22171=EDGE_LOOP('',(#52067,#52068,#52069,#52070)) ;
#22172=EDGE_LOOP('',(#52071,#52072,#52073,#52074,#52075)) ;
#22173=EDGE_LOOP('',(#52076,#52077,#52078,#52079)) ;
#22174=EDGE_LOOP('',(#52080,#52081,#52082,#52083)) ;
#22175=EDGE_LOOP('',(#52084,#52085,#52086)) ;
#22176=EDGE_LOOP('',(#52087,#52088,#52089)) ;
#22177=EDGE_LOOP('',(#52090,#52091,#52092,#52093,#52094)) ;
#22178=EDGE_LOOP('',(#52095,#52096,#52097,#52098)) ;
#22179=EDGE_LOOP('',(#52099,#52100,#52101)) ;
#22180=EDGE_LOOP('',(#52102,#52103,#52104,#52105)) ;
#22181=EDGE_LOOP('',(#52106,#52107,#52108,#52109)) ;
#22182=EDGE_LOOP('',(#52110,#52111,#52112,#52113)) ;
#22183=EDGE_LOOP('',(#52114,#52115,#52116,#52117)) ;
#22184=EDGE_LOOP('',(#52118,#52119,#52120,#52121)) ;
#22185=EDGE_LOOP('',(#52122,#52123,#52124,#52125)) ;
#22186=EDGE_LOOP('',(#52126,#52127,#52128)) ;
#22187=EDGE_LOOP('',(#52129,#52130,#52131,#52132)) ;
#22188=EDGE_LOOP('',(#52133,#52134,#52135,#52136,#52137)) ;
#22189=EDGE_LOOP('',(#52138,#52139,#52140,#52141)) ;
#22190=EDGE_LOOP('',(#52142,#52143,#52144,#52145)) ;
#22191=EDGE_LOOP('',(#52146,#52147,#52148,#52149,#52150)) ;
#22192=EDGE_LOOP('',(#52151,#52152,#52153,#52154)) ;
#22193=EDGE_LOOP('',(#52155,#52156,#52157)) ;
#22194=EDGE_LOOP('',(#52158,#52159,#52160,#52161)) ;
#22195=EDGE_LOOP('',(#52162,#52163,#52164,#52165)) ;
#22196=EDGE_LOOP('',(#52166,#52167,#52168,#52169)) ;
#22197=EDGE_LOOP('',(#52170,#52171,#52172,#52173)) ;
#22198=EDGE_LOOP('',(#52174,#52175,#52176,#52177)) ;
#22199=EDGE_LOOP('',(#52178,#52179,#52180,#52181)) ;
#22200=EDGE_LOOP('',(#52182,#52183,#52184)) ;
#22201=EDGE_LOOP('',(#52185,#52186,#52187,#52188)) ;
#22202=EDGE_LOOP('',(#52189,#52190,#52191,#52192)) ;
#22203=EDGE_LOOP('',(#52193,#52194,#52195,#52196)) ;
#22204=EDGE_LOOP('',(#52197,#52198,#52199,#52200)) ;
#22205=EDGE_LOOP('',(#52201,#52202,#52203,#52204)) ;
#22206=EDGE_LOOP('',(#52205,#52206,#52207,#52208)) ;
#22207=EDGE_LOOP('',(#52209,#52210,#52211,#52212)) ;
#22208=EDGE_LOOP('',(#52213,#52214,#52215,#52216)) ;
#22209=EDGE_LOOP('',(#52217,#52218,#52219,#52220)) ;
#22210=EDGE_LOOP('',(#52221,#52222,#52223)) ;
#22211=EDGE_LOOP('',(#52224,#52225,#52226,#52227)) ;
#22212=EDGE_LOOP('',(#52228,#52229,#52230)) ;
#22213=EDGE_LOOP('',(#52231,#52232,#52233,#52234)) ;
#22214=EDGE_LOOP('',(#52235,#52236,#52237,#52238)) ;
#22215=EDGE_LOOP('',(#52239,#52240,#52241,#52242)) ;
#22216=EDGE_LOOP('',(#52243,#52244,#52245,#52246)) ;
#22217=EDGE_LOOP('',(#52247,#52248,#52249,#52250)) ;
#22218=EDGE_LOOP('',(#52251,#52252,#52253,#52254)) ;
#22219=EDGE_LOOP('',(#52255,#52256,#52257,#52258)) ;
#22220=EDGE_LOOP('',(#52259,#52260,#52261,#52262,#52263,#52264)) ;
#22221=EDGE_LOOP('',(#52265,#52266,#52267)) ;
#22222=EDGE_LOOP('',(#52268,#52269,#52270,#52271)) ;
#22223=EDGE_LOOP('',(#52272,#52273,#52274,#52275)) ;
#22224=EDGE_LOOP('',(#52276,#52277,#52278,#52279)) ;
#22225=EDGE_LOOP('',(#52280,#52281,#52282,#52283)) ;
#22226=EDGE_LOOP('',(#52284,#52285,#52286,#52287)) ;
#22227=EDGE_LOOP('',(#52288,#52289,#52290,#52291)) ;
#22228=EDGE_LOOP('',(#52292,#52293,#52294,#52295)) ;
#22229=EDGE_LOOP('',(#52296,#52297,#52298,#52299,#52300)) ;
#22230=EDGE_LOOP('',(#52301,#52302,#52303,#52304)) ;
#22231=EDGE_LOOP('',(#52305,#52306,#52307,#52308,#52309)) ;
#22232=EDGE_LOOP('',(#52310,#52311,#52312,#52313)) ;
#22233=EDGE_LOOP('',(#52314,#52315,#52316,#52317,#52318)) ;
#22234=EDGE_LOOP('',(#52319,#52320,#52321,#52322)) ;
#22235=EDGE_LOOP('',(#52323,#52324,#52325)) ;
#22236=EDGE_LOOP('',(#52326,#52327,#52328,#52329)) ;
#22237=EDGE_LOOP('',(#52330,#52331,#52332,#52333)) ;
#22238=EDGE_LOOP('',(#52334,#52335,#52336,#52337)) ;
#22239=EDGE_LOOP('',(#52338,#52339,#52340,#52341)) ;
#22240=EDGE_LOOP('',(#52342,#52343,#52344,#52345)) ;
#22241=EDGE_LOOP('',(#52346,#52347,#52348)) ;
#22242=EDGE_LOOP('',(#52349,#52350,#52351)) ;
#22243=EDGE_LOOP('',(#52352,#52353,#52354,#52355)) ;
#22244=EDGE_LOOP('',(#52356,#52357,#52358,#52359)) ;
#22245=EDGE_LOOP('',(#52360,#52361,#52362)) ;
#22246=EDGE_LOOP('',(#52363,#52364,#52365,#52366)) ;
#22247=EDGE_LOOP('',(#52367,#52368,#52369,#52370)) ;
#22248=EDGE_LOOP('',(#52371,#52372,#52373,#52374,#52375)) ;
#22249=EDGE_LOOP('',(#52376,#52377,#52378,#52379)) ;
#22250=EDGE_LOOP('',(#52380,#52381,#52382,#52383)) ;
#22251=EDGE_LOOP('',(#52384,#52385,#52386,#52387)) ;
#22252=EDGE_LOOP('',(#52388,#52389,#52390,#52391)) ;
#22253=EDGE_LOOP('',(#52392,#52393,#52394,#52395)) ;
#22254=EDGE_LOOP('',(#52396,#52397,#52398)) ;
#22255=EDGE_LOOP('',(#52399,#52400,#52401,#52402)) ;
#22256=EDGE_LOOP('',(#52403,#52404,#52405,#52406)) ;
#22257=EDGE_LOOP('',(#52407,#52408,#52409)) ;
#22258=EDGE_LOOP('',(#52410,#52411,#52412,#52413)) ;
#22259=EDGE_LOOP('',(#52414,#52415,#52416,#52417)) ;
#22260=EDGE_LOOP('',(#52418,#52419,#52420,#52421)) ;
#22261=EDGE_LOOP('',(#52422,#52423,#52424,#52425)) ;
#22262=EDGE_LOOP('',(#52426,#52427,#52428)) ;
#22263=EDGE_LOOP('',(#52429,#52430,#52431)) ;
#22264=EDGE_LOOP('',(#52432,#52433,#52434,#52435)) ;
#22265=EDGE_LOOP('',(#52436,#52437,#52438,#52439)) ;
#22266=EDGE_LOOP('',(#52440,#52441,#52442,#52443)) ;
#22267=EDGE_LOOP('',(#52444,#52445,#52446)) ;
#22268=EDGE_LOOP('',(#52447,#52448,#52449,#52450)) ;
#22269=EDGE_LOOP('',(#52451,#52452,#52453,#52454)) ;
#22270=EDGE_LOOP('',(#52455,#52456,#52457)) ;
#22271=EDGE_LOOP('',(#52458,#52459,#52460,#52461)) ;
#22272=EDGE_LOOP('',(#52462,#52463,#52464,#52465,#52466)) ;
#22273=EDGE_LOOP('',(#52467,#52468,#52469,#52470)) ;
#22274=EDGE_LOOP('',(#52471,#52472,#52473)) ;
#22275=EDGE_LOOP('',(#52474,#52475,#52476,#52477)) ;
#22276=EDGE_LOOP('',(#52478,#52479,#52480,#52481)) ;
#22277=EDGE_LOOP('',(#52482,#52483,#52484)) ;
#22278=EDGE_LOOP('',(#52485,#52486,#52487,#52488,#52489)) ;
#22279=EDGE_LOOP('',(#52490,#52491,#52492,#52493)) ;
#22280=EDGE_LOOP('',(#52494,#52495,#52496,#52497)) ;
#22281=EDGE_LOOP('',(#52498,#52499,#52500,#52501)) ;
#22282=EDGE_LOOP('',(#52502,#52503,#52504,#52505)) ;
#22283=EDGE_LOOP('',(#52506,#52507,#52508,#52509)) ;
#22284=EDGE_LOOP('',(#52510,#52511,#52512,#52513)) ;
#22285=EDGE_LOOP('',(#52514,#52515,#52516,#52517)) ;
#22286=EDGE_LOOP('',(#52518,#52519,#52520,#52521)) ;
#22287=EDGE_LOOP('',(#52522,#52523,#52524,#52525,#52526)) ;
#22288=EDGE_LOOP('',(#52527,#52528,#52529,#52530,#52531,#52532,#52533,#52534)) ;
#22289=EDGE_LOOP('',(#52535,#52536,#52537)) ;
#22290=EDGE_LOOP('',(#52538,#52539,#52540,#52541)) ;
#22291=EDGE_LOOP('',(#52542,#52543,#52544,#52545,#52546)) ;
#22292=EDGE_LOOP('',(#52547,#52548,#52549,#52550,#52551)) ;
#22293=EDGE_LOOP('',(#52552,#52553,#52554,#52555)) ;
#22294=EDGE_LOOP('',(#52556,#52557,#52558)) ;
#22295=EDGE_LOOP('',(#52559,#52560,#52561,#52562,#52563,#52564,#52565,#52566)) ;
#22296=EDGE_LOOP('',(#52567,#52568,#52569,#52570,#52571)) ;
#22297=EDGE_LOOP('',(#52572,#52573,#52574,#52575,#52576)) ;
#22298=EDGE_LOOP('',(#52577,#52578,#52579,#52580)) ;
#22299=EDGE_LOOP('',(#52581,#52582,#52583,#52584,#52585,#52586,#52587,#52588)) ;
#22300=EDGE_LOOP('',(#52589,#52590,#52591,#52592)) ;
#22301=EDGE_LOOP('',(#52593,#52594,#52595,#52596,#52597,#52598,#52599,#52600)) ;
#22302=EDGE_LOOP('',(#52601,#52602,#52603,#52604)) ;
#22303=EDGE_LOOP('',(#52605,#52606,#52607,#52608)) ;
#22304=EDGE_LOOP('',(#52609,#52610,#52611,#52612)) ;
#22305=EDGE_LOOP('',(#52613,#52614,#52615,#52616)) ;
#22306=EDGE_LOOP('',(#52617,#52618,#52619,#52620,#52621,#52622,#52623,#52624,
#52625)) ;
#22307=EDGE_LOOP('',(#52626,#52627,#52628,#52629,#52630,#52631,#52632)) ;
#22308=EDGE_LOOP('',(#52633,#52634,#52635,#52636)) ;
#22309=EDGE_LOOP('',(#52637,#52638,#52639,#52640)) ;
#22310=EDGE_LOOP('',(#52641,#52642,#52643,#52644)) ;
#22311=EDGE_LOOP('',(#52645,#52646,#52647)) ;
#22312=EDGE_LOOP('',(#52648,#52649,#52650,#52651)) ;
#22313=EDGE_LOOP('',(#52652,#52653,#52654,#52655)) ;
#22314=EDGE_LOOP('',(#52656,#52657,#52658,#52659)) ;
#22315=EDGE_LOOP('',(#52660,#52661,#52662,#52663)) ;
#22316=EDGE_LOOP('',(#52664,#52665,#52666,#52667)) ;
#22317=EDGE_LOOP('',(#52668,#52669,#52670,#52671)) ;
#22318=EDGE_LOOP('',(#52672,#52673,#52674,#52675)) ;
#22319=EDGE_LOOP('',(#52676,#52677,#52678,#52679)) ;
#22320=EDGE_LOOP('',(#52680,#52681,#52682,#52683)) ;
#22321=EDGE_LOOP('',(#52684,#52685,#52686,#52687)) ;
#22322=EDGE_LOOP('',(#52688,#52689,#52690,#52691)) ;
#22323=EDGE_LOOP('',(#52692,#52693,#52694,#52695)) ;
#22324=EDGE_LOOP('',(#52696,#52697,#52698,#52699)) ;
#22325=EDGE_LOOP('',(#52700,#52701,#52702,#52703)) ;
#22326=EDGE_LOOP('',(#52704,#52705,#52706,#52707)) ;
#22327=EDGE_LOOP('',(#52708,#52709,#52710,#52711)) ;
#22328=EDGE_LOOP('',(#52712,#52713,#52714,#52715)) ;
#22329=EDGE_LOOP('',(#52716,#52717,#52718,#52719)) ;
#22330=EDGE_LOOP('',(#52720,#52721,#52722,#52723)) ;
#22331=EDGE_LOOP('',(#52724,#52725,#52726)) ;
#22332=EDGE_LOOP('',(#52727,#52728,#52729,#52730)) ;
#22333=EDGE_LOOP('',(#52731,#52732,#52733,#52734,#52735,#52736)) ;
#22334=EDGE_LOOP('',(#52737,#52738,#52739,#52740)) ;
#22335=EDGE_LOOP('',(#52741,#52742,#52743,#52744,#52745)) ;
#22336=EDGE_LOOP('',(#52746,#52747,#52748,#52749)) ;
#25273=CIRCLE('',#68780,0.1) ;
#25274=CIRCLE('',#68782,0.1) ;
#25275=CIRCLE('',#68784,0.1) ;
#25276=CIRCLE('',#68787,1.4) ;
#25277=CIRCLE('',#68788,0.1) ;
#25278=CIRCLE('',#68789,1.5) ;
#25279=CIRCLE('',#68791,1.5) ;
#25280=CIRCLE('',#68792,0.1) ;
#25281=CIRCLE('',#68793,1.6) ;
#25282=CIRCLE('',#68795,0.1) ;
#25283=CIRCLE('',#68796,0.1) ;
#25284=CIRCLE('',#68797,0.1) ;
#25285=CIRCLE('',#68799,0.1) ;
#25286=CIRCLE('',#68800,0.1) ;
#25287=CIRCLE('',#68802,3.) ;
#25288=CIRCLE('',#68803,0.1) ;
#25289=CIRCLE('',#68804,3.00136060761679) ;
#25290=CIRCLE('',#68805,0.1) ;
#25291=CIRCLE('',#68808,3.) ;
#25292=CIRCLE('',#68809,3.) ;
#25293=CIRCLE('',#68810,3.) ;
#25294=CIRCLE('',#68819,3.33471270883832) ;
#25295=CIRCLE('',#68821,0.0999999999999994) ;
#25296=CIRCLE('',#68822,0.0999999999999994) ;
#25297=CIRCLE('',#68823,0.0999999999999994) ;
#25298=CIRCLE('',#68824,0.0999999999999994) ;
#25299=CIRCLE('',#68825,0.1) ;
#25300=CIRCLE('',#68826,0.1) ;
#25301=CIRCLE('',#68827,0.1) ;
#25302=CIRCLE('',#68828,0.1) ;
#25303=CIRCLE('',#68829,0.1) ;
#25304=CIRCLE('',#68830,0.1) ;
#25305=CIRCLE('',#68831,0.0999999999999994) ;
#25306=CIRCLE('',#68832,0.0999999999999994) ;
#25307=CIRCLE('',#68833,0.0999999999999994) ;
#25308=CIRCLE('',#68834,0.1) ;
#25309=CIRCLE('',#68835,0.1) ;
#25310=CIRCLE('',#68836,0.1) ;
#25311=CIRCLE('',#68838,0.0999999999999994) ;
#25312=CIRCLE('',#68839,0.1) ;
#25313=CIRCLE('',#68840,0.1) ;
#25314=CIRCLE('',#68841,0.1) ;
#25315=CIRCLE('',#68842,0.0999999999999994) ;
#25316=CIRCLE('',#68843,0.0999999999999994) ;
#25317=CIRCLE('',#68844,0.0999999999999994) ;
#25318=CIRCLE('',#68845,0.1) ;
#25319=CIRCLE('',#68846,0.1) ;
#25320=CIRCLE('',#68847,0.1) ;
#25321=CIRCLE('',#68848,0.1) ;
#25322=CIRCLE('',#68849,0.1) ;
#25323=CIRCLE('',#68850,0.1) ;
#25324=CIRCLE('',#68851,0.0999999999999994) ;
#25325=CIRCLE('',#68852,0.0999999999999994) ;
#25326=CIRCLE('',#68853,0.0999999999999994) ;
#25327=CIRCLE('',#68862,0.2) ;
#25328=CIRCLE('',#68863,0.2) ;
#25329=CIRCLE('',#68865,0.2) ;
#25330=CIRCLE('',#68866,0.2) ;
#25331=CIRCLE('',#68867,1.65) ;
#25332=CIRCLE('',#68868,0.2) ;
#25333=CIRCLE('',#68869,0.2) ;
#25334=CIRCLE('',#68870,1.65) ;
#25335=CIRCLE('',#68871,0.2) ;
#25336=CIRCLE('',#68872,0.2) ;
#25337=CIRCLE('',#68873,1.65) ;
#25338=CIRCLE('',#68874,0.2) ;
#25339=CIRCLE('',#68875,2.9) ;
#25340=CIRCLE('',#68876,0.2) ;
#25341=CIRCLE('',#68877,1.65) ;
#25342=CIRCLE('',#68879,0.2) ;
#25343=CIRCLE('',#68880,0.2) ;
#25344=CIRCLE('',#68882,0.2) ;
#25345=CIRCLE('',#68883,0.2) ;
#25346=CIRCLE('',#68885,0.2) ;
#25347=CIRCLE('',#68887,0.2) ;
#25348=CIRCLE('',#68895,0.1) ;
#25349=CIRCLE('',#68896,0.1) ;
#25350=CIRCLE('',#68897,0.0999999999999998) ;
#25351=CIRCLE('',#68898,0.0999999999999998) ;
#25352=CIRCLE('',#68900,0.2) ;
#25353=CIRCLE('',#68901,1.85) ;
#25354=CIRCLE('',#68902,2.9) ;
#25355=CIRCLE('',#68906,1.75) ;
#25356=CIRCLE('',#68907,1.75) ;
#25357=CIRCLE('',#68909,1.75) ;
#25358=CIRCLE('',#68910,1.75) ;
#25359=CIRCLE('',#68914,1.85) ;
#25360=CIRCLE('',#68915,0.2) ;
#25361=CIRCLE('',#68916,2.9) ;
#25362=CIRCLE('',#68918,1.85) ;
#25363=CIRCLE('',#68921,1.75) ;
#25364=CIRCLE('',#68922,1.75) ;
#25365=CIRCLE('',#68925,1.75) ;
#25366=CIRCLE('',#68926,1.75) ;
#25367=CIRCLE('',#68930,1.85) ;
#25368=CIRCLE('',#68945,1.1) ;
#25369=CIRCLE('',#68946,1.9) ;
#25370=CIRCLE('',#68948,1.9) ;
#25371=CIRCLE('',#68949,1.1) ;
#25372=CIRCLE('',#68951,2.) ;
#25373=CIRCLE('',#68952,2.) ;
#25374=CIRCLE('',#68959,1.) ;
#25375=CIRCLE('',#68960,1.) ;
#25376=CIRCLE('',#68966,609.695407949973) ;
#25377=CIRCLE('',#68968,3.23607331645511) ;
#25378=CIRCLE('',#68969,576.383429116614) ;
#25379=CIRCLE('',#68970,576.383429126766) ;
#25380=CIRCLE('',#68972,609.695407938939) ;
#25381=CIRCLE('',#68974,0.1) ;
#25382=CIRCLE('',#68976,0.1) ;
#25383=CIRCLE('',#68977,0.1) ;
#25384=CIRCLE('',#68979,0.1) ;
#25385=CIRCLE('',#68981,0.1) ;
#25386=CIRCLE('',#68983,0.1) ;
#25387=CIRCLE('',#68985,0.1) ;
#25388=CIRCLE('',#68987,0.1) ;
#25389=CIRCLE('',#68988,0.1) ;
#25390=CIRCLE('',#68990,0.1) ;
#25391=CIRCLE('',#68992,0.1) ;
#25392=CIRCLE('',#68993,0.1) ;
#25393=CIRCLE('',#68995,0.1) ;
#25394=CIRCLE('',#68997,0.1) ;
#25395=CIRCLE('',#68999,0.1) ;
#25396=CIRCLE('',#69001,0.1) ;
#25397=CIRCLE('',#69003,0.1) ;
#25398=CIRCLE('',#69005,0.1) ;
#25399=CIRCLE('',#69007,0.1) ;
#25400=CIRCLE('',#69009,0.1) ;
#25401=CIRCLE('',#69011,0.1) ;
#25402=CIRCLE('',#69013,0.1) ;
#25403=CIRCLE('',#69015,0.1) ;
#25404=CIRCLE('',#69016,0.1) ;
#25405=CIRCLE('',#69018,0.1) ;
#25406=CIRCLE('',#69020,0.1) ;
#25407=CIRCLE('',#69022,0.1) ;
#25408=CIRCLE('',#69024,0.1) ;
#25409=CIRCLE('',#69026,0.1) ;
#25410=CIRCLE('',#69028,0.1) ;
#25411=CIRCLE('',#69030,0.1) ;
#25412=CIRCLE('',#69032,0.1) ;
#25413=CIRCLE('',#69034,0.1) ;
#25414=CIRCLE('',#69036,0.1) ;
#25415=CIRCLE('',#69038,0.1) ;
#25416=CIRCLE('',#69040,0.1) ;
#25417=CIRCLE('',#69043,0.1) ;
#25418=CIRCLE('',#69044,0.1) ;
#25419=CIRCLE('',#69045,0.1) ;
#25420=CIRCLE('',#69051,0.1) ;
#25421=CIRCLE('',#69059,0.1) ;
#25422=CIRCLE('',#69060,0.1) ;
#25423=CIRCLE('',#69062,0.1) ;
#25424=CIRCLE('',#69064,0.1) ;
#25425=CIRCLE('',#69065,0.1) ;
#25426=CIRCLE('',#69068,0.1) ;
#25427=CIRCLE('',#69071,0.1) ;
#25428=CIRCLE('',#69073,0.1) ;
#25429=CIRCLE('',#69076,0.1) ;
#25430=CIRCLE('',#69078,0.1) ;
#25431=CIRCLE('',#69080,0.1) ;
#25432=CIRCLE('',#69082,0.1) ;
#25433=CIRCLE('',#69084,0.1) ;
#25434=CIRCLE('',#69085,0.1) ;
#25435=CIRCLE('',#69087,0.1) ;
#25436=CIRCLE('',#69089,0.1) ;
#25437=CIRCLE('',#69091,0.1) ;
#25438=CIRCLE('',#69092,0.1) ;
#25439=CIRCLE('',#69094,0.1) ;
#25440=CIRCLE('',#69096,0.1) ;
#25441=CIRCLE('',#69098,0.1) ;
#25442=CIRCLE('',#69100,0.1) ;
#25443=CIRCLE('',#69102,0.1) ;
#25444=CIRCLE('',#69104,0.1) ;
#25445=CIRCLE('',#69106,0.1) ;
#25446=CIRCLE('',#69107,0.1) ;
#25447=CIRCLE('',#69109,0.1) ;
#25448=CIRCLE('',#69114,0.1) ;
#25449=CIRCLE('',#69117,0.0999999999999998) ;
#25450=CIRCLE('',#69119,0.1) ;
#25451=CIRCLE('',#69120,0.1) ;
#25452=CIRCLE('',#69122,0.1) ;
#25453=CIRCLE('',#69124,0.0999999999999998) ;
#25454=CIRCLE('',#69126,0.1) ;
#25455=CIRCLE('',#69128,0.1) ;
#25456=CIRCLE('',#69130,0.1) ;
#25457=CIRCLE('',#69131,0.1) ;
#25458=CIRCLE('',#69133,0.0999999999999999) ;
#25459=CIRCLE('',#69135,0.1) ;
#25460=CIRCLE('',#69136,0.1) ;
#25461=CIRCLE('',#69138,0.1) ;
#25462=CIRCLE('',#69140,0.0999999999999999) ;
#25463=CIRCLE('',#69142,0.0999999999999998) ;
#25464=CIRCLE('',#69144,0.1) ;
#25465=CIRCLE('',#69146,0.1) ;
#25466=CIRCLE('',#69148,0.1) ;
#25467=CIRCLE('',#69149,0.1) ;
#25468=CIRCLE('',#69151,0.1) ;
#25469=CIRCLE('',#69153,0.1) ;
#25470=CIRCLE('',#69155,0.1) ;
#25471=CIRCLE('',#69158,0.1) ;
#25472=CIRCLE('',#69160,0.1) ;
#25473=CIRCLE('',#69161,0.1) ;
#25474=CIRCLE('',#69164,0.1) ;
#25475=CIRCLE('',#69166,0.1) ;
#25476=CIRCLE('',#69167,0.1) ;
#25477=CIRCLE('',#69169,0.0999999999999999) ;
#25478=CIRCLE('',#69171,0.0999999999999998) ;
#25479=CIRCLE('',#69173,0.1) ;
#25480=CIRCLE('',#69174,0.1) ;
#25481=CIRCLE('',#69176,0.1) ;
#25482=CIRCLE('',#69178,0.1) ;
#25483=CIRCLE('',#69180,0.1) ;
#25484=CIRCLE('',#69182,0.1) ;
#25485=CIRCLE('',#69184,0.0999999999999998) ;
#25486=CIRCLE('',#69186,0.0999999999999999) ;
#25487=CIRCLE('',#69188,0.1) ;
#25488=CIRCLE('',#69191,0.1) ;
#25489=CIRCLE('',#69193,0.1) ;
#25490=CIRCLE('',#69195,0.1) ;
#25491=CIRCLE('',#69197,0.1) ;
#25492=CIRCLE('',#69198,0.1) ;
#25493=CIRCLE('',#69200,0.1) ;
#25494=CIRCLE('',#69202,0.1) ;
#25495=CIRCLE('',#69204,0.1) ;
#25496=CIRCLE('',#69205,0.0999999999999998) ;
#25497=CIRCLE('',#69207,0.1) ;
#25498=CIRCLE('',#69209,0.1) ;
#25499=CIRCLE('',#69210,0.1) ;
#25500=CIRCLE('',#69212,0.1) ;
#25501=CIRCLE('',#69214,0.0999999999999998) ;
#25502=CIRCLE('',#69216,0.1) ;
#25503=CIRCLE('',#69217,0.1) ;
#25504=CIRCLE('',#69219,0.0999999999999998) ;
#25505=CIRCLE('',#69221,0.1) ;
#25506=CIRCLE('',#69223,0.1) ;
#25507=CIRCLE('',#69225,0.0999999999999998) ;
#25508=CIRCLE('',#69227,0.1) ;
#25509=CIRCLE('',#69229,0.1) ;
#25510=CIRCLE('',#69231,0.1) ;
#25511=CIRCLE('',#69232,0.1) ;
#25512=CIRCLE('',#69235,0.0999999999999998) ;
#25513=CIRCLE('',#69237,0.1) ;
#25514=CIRCLE('',#69239,0.1) ;
#25515=CIRCLE('',#69240,0.1) ;
#25516=CIRCLE('',#69242,0.1) ;
#25517=CIRCLE('',#69243,0.0999999999999998) ;
#25518=CIRCLE('',#69245,0.0999999999999994) ;
#25519=CIRCLE('',#69246,0.1) ;
#25520=CIRCLE('',#69248,0.0999999999999998) ;
#25521=CIRCLE('',#69250,0.0999999999999998) ;
#25522=CIRCLE('',#69252,0.1) ;
#25523=CIRCLE('',#69254,0.0999999999999994) ;
#25524=CIRCLE('',#69256,0.0999999999999994) ;
#25525=CIRCLE('',#69258,0.1) ;
#25526=CIRCLE('',#69259,0.1) ;
#25527=CIRCLE('',#69261,0.1) ;
#25528=CIRCLE('',#69262,0.1) ;
#25529=CIRCLE('',#69264,0.0999999999999998) ;
#25530=CIRCLE('',#69266,0.1) ;
#25531=CIRCLE('',#69268,0.0999999999999994) ;
#25532=CIRCLE('',#69271,0.0999999999999994) ;
#25533=CIRCLE('',#69273,0.0999999999999999) ;
#25534=CIRCLE('',#69275,0.1) ;
#25535=CIRCLE('',#69277,0.1) ;
#25536=CIRCLE('',#69279,0.0999999999999994) ;
#25537=CIRCLE('',#69281,0.0999999999999998) ;
#25538=CIRCLE('',#69285,0.1) ;
#25539=CIRCLE('',#69287,0.1) ;
#25540=CIRCLE('',#69289,0.0999999999999994) ;
#25541=CIRCLE('',#69291,0.1) ;
#25542=CIRCLE('',#69293,0.0999999999999994) ;
#25543=CIRCLE('',#69295,0.100000000000001) ;
#25544=CIRCLE('',#69299,0.1) ;
#25545=CIRCLE('',#69300,0.1) ;
#25546=CIRCLE('',#69306,0.0999999999999994) ;
#25547=CIRCLE('',#69308,0.1) ;
#25548=CIRCLE('',#69309,0.0999999999999999) ;
#25549=CIRCLE('',#69311,0.0999999999999994) ;
#25550=CIRCLE('',#69312,0.1) ;
#25551=CIRCLE('',#69314,0.1) ;
#25552=CIRCLE('',#69316,0.1) ;
#25553=CIRCLE('',#69318,0.1) ;
#25554=CIRCLE('',#69319,0.1) ;
#25555=CIRCLE('',#69321,0.1) ;
#25556=CIRCLE('',#69323,0.1) ;
#25557=CIRCLE('',#69325,0.1) ;
#25558=CIRCLE('',#69326,0.1) ;
#25559=CIRCLE('',#69328,0.1) ;
#25560=CIRCLE('',#69331,0.0999999999999994) ;
#25561=CIRCLE('',#69333,0.0999999999999994) ;
#25562=CIRCLE('',#69337,0.1) ;
#25563=CIRCLE('',#69339,0.0999999999999994) ;
#25564=CIRCLE('',#69341,0.0999999999999999) ;
#25565=CIRCLE('',#69342,0.1) ;
#25566=CIRCLE('',#69345,0.1) ;
#25567=CIRCLE('',#69346,0.0999999999999998) ;
#25568=CIRCLE('',#69348,0.1) ;
#25569=CIRCLE('',#69350,0.1) ;
#25570=CIRCLE('',#69352,0.0999999999999998) ;
#25571=CIRCLE('',#69354,0.1) ;
#25572=CIRCLE('',#69356,0.1) ;
#25573=CIRCLE('',#69358,0.1) ;
#25574=CIRCLE('',#69361,0.0999999999999994) ;
#25575=CIRCLE('',#69362,0.1) ;
#25576=CIRCLE('',#69364,0.0999999999999994) ;
#25577=CIRCLE('',#69366,0.1) ;
#25578=CIRCLE('',#69368,0.1) ;
#25579=CIRCLE('',#69370,0.1) ;
#25580=CIRCLE('',#69372,0.1) ;
#25581=CIRCLE('',#69374,0.0999999999999994) ;
#25582=CIRCLE('',#69377,0.0999999999999994) ;
#25583=CIRCLE('',#69379,0.0999999999999999) ;
#25584=CIRCLE('',#69380,0.0999999999999999) ;
#25585=CIRCLE('',#69384,0.0999999999999994) ;
#25586=CIRCLE('',#69386,0.0999999999999994) ;
#25587=CIRCLE('',#69390,0.1) ;
#25588=CIRCLE('',#69392,0.1) ;
#25589=CIRCLE('',#69394,0.1) ;
#25590=CIRCLE('',#69397,1.4) ;
#25591=CIRCLE('',#69398,0.1) ;
#25592=CIRCLE('',#69399,1.5) ;
#25593=CIRCLE('',#69401,1.5) ;
#25594=CIRCLE('',#69402,0.1) ;
#25595=CIRCLE('',#69403,1.6) ;
#25596=CIRCLE('',#69405,0.1) ;
#25597=CIRCLE('',#69406,0.1) ;
#25598=CIRCLE('',#69407,0.1) ;
#25599=CIRCLE('',#69409,0.1) ;
#25600=CIRCLE('',#69410,0.1) ;
#25601=CIRCLE('',#69412,3.) ;
#25602=CIRCLE('',#69413,0.1) ;
#25603=CIRCLE('',#69414,3.00136060761679) ;
#25604=CIRCLE('',#69415,0.1) ;
#25605=CIRCLE('',#69418,3.) ;
#25606=CIRCLE('',#69419,3.) ;
#25607=CIRCLE('',#69420,3.) ;
#25608=CIRCLE('',#69429,3.33471270883832) ;
#25609=CIRCLE('',#69431,0.0999999999999994) ;
#25610=CIRCLE('',#69432,0.0999999999999994) ;
#25611=CIRCLE('',#69433,0.0999999999999994) ;
#25612=CIRCLE('',#69434,0.0999999999999994) ;
#25613=CIRCLE('',#69435,0.1) ;
#25614=CIRCLE('',#69436,0.1) ;
#25615=CIRCLE('',#69437,0.1) ;
#25616=CIRCLE('',#69438,0.1) ;
#25617=CIRCLE('',#69439,0.1) ;
#25618=CIRCLE('',#69440,0.1) ;
#25619=CIRCLE('',#69441,0.0999999999999994) ;
#25620=CIRCLE('',#69442,0.0999999999999994) ;
#25621=CIRCLE('',#69443,0.0999999999999994) ;
#25622=CIRCLE('',#69444,0.1) ;
#25623=CIRCLE('',#69445,0.1) ;
#25624=CIRCLE('',#69446,0.1) ;
#25625=CIRCLE('',#69448,0.0999999999999994) ;
#25626=CIRCLE('',#69449,0.1) ;
#25627=CIRCLE('',#69450,0.1) ;
#25628=CIRCLE('',#69451,0.1) ;
#25629=CIRCLE('',#69452,0.0999999999999994) ;
#25630=CIRCLE('',#69453,0.0999999999999994) ;
#25631=CIRCLE('',#69454,0.0999999999999994) ;
#25632=CIRCLE('',#69455,0.1) ;
#25633=CIRCLE('',#69456,0.1) ;
#25634=CIRCLE('',#69457,0.1) ;
#25635=CIRCLE('',#69458,0.1) ;
#25636=CIRCLE('',#69459,0.1) ;
#25637=CIRCLE('',#69460,0.1) ;
#25638=CIRCLE('',#69461,0.0999999999999994) ;
#25639=CIRCLE('',#69462,0.0999999999999994) ;
#25640=CIRCLE('',#69463,0.0999999999999994) ;
#25641=CIRCLE('',#69472,0.2) ;
#25642=CIRCLE('',#69473,0.2) ;
#25643=CIRCLE('',#69475,0.2) ;
#25644=CIRCLE('',#69476,0.2) ;
#25645=CIRCLE('',#69477,1.65) ;
#25646=CIRCLE('',#69478,0.2) ;
#25647=CIRCLE('',#69479,0.2) ;
#25648=CIRCLE('',#69480,1.65) ;
#25649=CIRCLE('',#69481,0.2) ;
#25650=CIRCLE('',#69482,0.2) ;
#25651=CIRCLE('',#69483,1.65) ;
#25652=CIRCLE('',#69484,0.2) ;
#25653=CIRCLE('',#69485,2.9) ;
#25654=CIRCLE('',#69486,0.2) ;
#25655=CIRCLE('',#69487,1.65) ;
#25656=CIRCLE('',#69489,0.2) ;
#25657=CIRCLE('',#69490,0.2) ;
#25658=CIRCLE('',#69492,0.2) ;
#25659=CIRCLE('',#69493,0.2) ;
#25660=CIRCLE('',#69495,0.2) ;
#25661=CIRCLE('',#69497,0.2) ;
#25662=CIRCLE('',#69505,0.1) ;
#25663=CIRCLE('',#69506,0.1) ;
#25664=CIRCLE('',#69507,0.0999999999999998) ;
#25665=CIRCLE('',#69508,0.0999999999999998) ;
#25666=CIRCLE('',#69510,0.2) ;
#25667=CIRCLE('',#69511,1.85) ;
#25668=CIRCLE('',#69512,2.9) ;
#25669=CIRCLE('',#69516,1.75) ;
#25670=CIRCLE('',#69517,1.75) ;
#25671=CIRCLE('',#69519,1.75) ;
#25672=CIRCLE('',#69520,1.75) ;
#25673=CIRCLE('',#69524,1.85) ;
#25674=CIRCLE('',#69525,0.2) ;
#25675=CIRCLE('',#69526,2.9) ;
#25676=CIRCLE('',#69528,1.85) ;
#25677=CIRCLE('',#69531,1.75) ;
#25678=CIRCLE('',#69532,1.75) ;
#25679=CIRCLE('',#69535,1.75) ;
#25680=CIRCLE('',#69536,1.75) ;
#25681=CIRCLE('',#69540,1.85) ;
#25682=CIRCLE('',#69555,1.1) ;
#25683=CIRCLE('',#69556,1.9) ;
#25684=CIRCLE('',#69558,1.9) ;
#25685=CIRCLE('',#69559,1.1) ;
#25686=CIRCLE('',#69561,2.) ;
#25687=CIRCLE('',#69562,2.) ;
#25688=CIRCLE('',#69569,1.) ;
#25689=CIRCLE('',#69570,1.) ;
#25690=CIRCLE('',#69576,609.695407951934) ;
#25691=CIRCLE('',#69578,3.23607331645511) ;
#25692=CIRCLE('',#69579,576.383429245353) ;
#25693=CIRCLE('',#69580,576.383429191305) ;
#25694=CIRCLE('',#69582,609.695408159653) ;
#25695=CIRCLE('',#69584,0.1) ;
#25696=CIRCLE('',#69586,0.0999999999999999) ;
#25697=CIRCLE('',#69587,0.0999999999999998) ;
#25698=CIRCLE('',#69589,0.1) ;
#25699=CIRCLE('',#69591,0.1) ;
#25700=CIRCLE('',#69593,0.1) ;
#25701=CIRCLE('',#69595,0.0999999999999999) ;
#25702=CIRCLE('',#69597,0.1) ;
#25703=CIRCLE('',#69598,0.1) ;
#25704=CIRCLE('',#69600,0.1) ;
#25705=CIRCLE('',#69602,0.1) ;
#25706=CIRCLE('',#69603,0.1) ;
#25707=CIRCLE('',#69605,0.1) ;
#25708=CIRCLE('',#69607,0.1) ;
#25709=CIRCLE('',#69609,0.1) ;
#25710=CIRCLE('',#69611,0.1) ;
#25711=CIRCLE('',#69613,0.1) ;
#25712=CIRCLE('',#69615,0.1) ;
#25713=CIRCLE('',#69617,0.1) ;
#25714=CIRCLE('',#69619,0.1) ;
#25715=CIRCLE('',#69621,0.1) ;
#25716=CIRCLE('',#69623,0.1) ;
#25717=CIRCLE('',#69625,0.1) ;
#25718=CIRCLE('',#69626,0.1) ;
#25719=CIRCLE('',#69628,0.1) ;
#25720=CIRCLE('',#69630,0.1) ;
#25721=CIRCLE('',#69632,0.1) ;
#25722=CIRCLE('',#69634,0.1) ;
#25723=CIRCLE('',#69636,0.1) ;
#25724=CIRCLE('',#69638,0.1) ;
#25725=CIRCLE('',#69640,0.1) ;
#25726=CIRCLE('',#69642,0.1) ;
#25727=CIRCLE('',#69644,0.1) ;
#25728=CIRCLE('',#69646,0.1) ;
#25729=CIRCLE('',#69648,0.1) ;
#25730=CIRCLE('',#69650,0.1) ;
#25731=CIRCLE('',#69653,0.1) ;
#25732=CIRCLE('',#69654,0.1) ;
#25733=CIRCLE('',#69655,0.1) ;
#25734=CIRCLE('',#69661,0.1) ;
#25735=CIRCLE('',#69669,0.1) ;
#25736=CIRCLE('',#69670,0.1) ;
#25737=CIRCLE('',#69672,0.1) ;
#25738=CIRCLE('',#69674,0.1) ;
#25739=CIRCLE('',#69675,0.1) ;
#25740=CIRCLE('',#69678,0.1) ;
#25741=CIRCLE('',#69681,0.1) ;
#25742=CIRCLE('',#69683,0.1) ;
#25743=CIRCLE('',#69686,0.1) ;
#25744=CIRCLE('',#69688,0.1) ;
#25745=CIRCLE('',#69690,0.1) ;
#25746=CIRCLE('',#69692,0.1) ;
#25747=CIRCLE('',#69694,0.1) ;
#25748=CIRCLE('',#69695,0.1) ;
#25749=CIRCLE('',#69697,0.1) ;
#25750=CIRCLE('',#69699,0.1) ;
#25751=CIRCLE('',#69701,0.0999999999999998) ;
#25752=CIRCLE('',#69702,0.1) ;
#25753=CIRCLE('',#69704,0.1) ;
#25754=CIRCLE('',#69706,0.1) ;
#25755=CIRCLE('',#69708,0.1) ;
#25756=CIRCLE('',#69710,0.0999999999999998) ;
#25757=CIRCLE('',#69712,0.0999999999999998) ;
#25758=CIRCLE('',#69714,0.0999999999999998) ;
#25759=CIRCLE('',#69716,0.0999999999999998) ;
#25760=CIRCLE('',#69717,0.0999999999999998) ;
#25761=CIRCLE('',#69719,0.1) ;
#25762=CIRCLE('',#69724,0.0999999999999998) ;
#25763=CIRCLE('',#69727,0.0999999999999998) ;
#25764=CIRCLE('',#69729,0.1) ;
#25765=CIRCLE('',#69730,0.1) ;
#25766=CIRCLE('',#69732,0.1) ;
#25767=CIRCLE('',#69734,0.0999999999999998) ;
#25768=CIRCLE('',#69736,0.1) ;
#25769=CIRCLE('',#69738,0.1) ;
#25770=CIRCLE('',#69740,0.1) ;
#25771=CIRCLE('',#69741,0.1) ;
#25772=CIRCLE('',#69743,0.1) ;
#25773=CIRCLE('',#69745,0.1) ;
#25774=CIRCLE('',#69746,0.1) ;
#25775=CIRCLE('',#69748,0.0999999999999999) ;
#25776=CIRCLE('',#69750,0.0999999999999999) ;
#25777=CIRCLE('',#69752,0.0999999999999998) ;
#25778=CIRCLE('',#69754,0.1) ;
#25779=CIRCLE('',#69756,0.1) ;
#25780=CIRCLE('',#69758,0.1) ;
#25781=CIRCLE('',#69759,0.1) ;
#25782=CIRCLE('',#69761,0.1) ;
#25783=CIRCLE('',#69763,0.1) ;
#25784=CIRCLE('',#69765,0.1) ;
#25785=CIRCLE('',#69768,0.1) ;
#25786=CIRCLE('',#69770,0.0999999999999998) ;
#25787=CIRCLE('',#69771,0.1) ;
#25788=CIRCLE('',#69774,0.1) ;
#25789=CIRCLE('',#69776,0.1) ;
#25790=CIRCLE('',#69777,0.1) ;
#25791=CIRCLE('',#69779,0.0999999999999999) ;
#25792=CIRCLE('',#69781,0.0999999999999998) ;
#25793=CIRCLE('',#69783,0.1) ;
#25794=CIRCLE('',#69784,0.1) ;
#25795=CIRCLE('',#69786,0.1) ;
#25796=CIRCLE('',#69788,0.1) ;
#25797=CIRCLE('',#69790,0.0999999999999999) ;
#25798=CIRCLE('',#69792,0.1) ;
#25799=CIRCLE('',#69794,0.0999999999999998) ;
#25800=CIRCLE('',#69796,0.0999999999999999) ;
#25801=CIRCLE('',#69798,0.1) ;
#25802=CIRCLE('',#69801,0.1) ;
#25803=CIRCLE('',#69803,0.1) ;
#25804=CIRCLE('',#69805,0.1) ;
#25805=CIRCLE('',#69807,0.1) ;
#25806=CIRCLE('',#69808,0.1) ;
#25807=CIRCLE('',#69810,0.1) ;
#25808=CIRCLE('',#69812,0.1) ;
#25809=CIRCLE('',#69814,0.1) ;
#25810=CIRCLE('',#69815,0.0999999999999998) ;
#25811=CIRCLE('',#69817,0.1) ;
#25812=CIRCLE('',#69819,0.1) ;
#25813=CIRCLE('',#69820,0.1) ;
#25814=CIRCLE('',#69822,0.1) ;
#25815=CIRCLE('',#69824,0.0999999999999998) ;
#25816=CIRCLE('',#69826,0.1) ;
#25817=CIRCLE('',#69827,0.1) ;
#25818=CIRCLE('',#69829,0.0999999999999998) ;
#25819=CIRCLE('',#69831,0.1) ;
#25820=CIRCLE('',#69833,0.1) ;
#25821=CIRCLE('',#69835,0.0999999999999998) ;
#25822=CIRCLE('',#69837,0.1) ;
#25823=CIRCLE('',#69839,0.1) ;
#25824=CIRCLE('',#69841,0.1) ;
#25825=CIRCLE('',#69842,0.1) ;
#25826=CIRCLE('',#69845,0.0999999999999998) ;
#25827=CIRCLE('',#69847,0.1) ;
#25828=CIRCLE('',#69849,0.1) ;
#25829=CIRCLE('',#69850,0.1) ;
#25830=CIRCLE('',#69852,0.1) ;
#25831=CIRCLE('',#69853,0.0999999999999998) ;
#25832=CIRCLE('',#69855,0.0999999999999994) ;
#25833=CIRCLE('',#69856,0.1) ;
#25834=CIRCLE('',#69858,0.0999999999999998) ;
#25835=CIRCLE('',#69860,0.0999999999999998) ;
#25836=CIRCLE('',#69862,0.1) ;
#25837=CIRCLE('',#69864,0.0999999999999994) ;
#25838=CIRCLE('',#69866,0.0999999999999994) ;
#25839=CIRCLE('',#69868,0.1) ;
#25840=CIRCLE('',#69869,0.1) ;
#25841=CIRCLE('',#69871,0.1) ;
#25842=CIRCLE('',#69872,0.1) ;
#25843=CIRCLE('',#69874,0.0999999999999998) ;
#25844=CIRCLE('',#69876,0.1) ;
#25845=CIRCLE('',#69878,0.0999999999999994) ;
#25846=CIRCLE('',#69881,0.0999999999999994) ;
#25847=CIRCLE('',#69883,0.1) ;
#25848=CIRCLE('',#69885,0.1) ;
#25849=CIRCLE('',#69887,0.1) ;
#25850=CIRCLE('',#69889,0.0999999999999994) ;
#25851=CIRCLE('',#69891,0.0999999999999998) ;
#25852=CIRCLE('',#69895,0.1) ;
#25853=CIRCLE('',#69897,0.1) ;
#25854=CIRCLE('',#69899,0.0999999999999994) ;
#25855=CIRCLE('',#69901,0.1) ;
#25856=CIRCLE('',#69903,0.0999999999999994) ;
#25857=CIRCLE('',#69905,0.100000000000001) ;
#25858=CIRCLE('',#69909,0.1) ;
#25859=CIRCLE('',#69910,0.1) ;
#25860=CIRCLE('',#69916,0.0999999999999994) ;
#25861=CIRCLE('',#69918,0.1) ;
#25862=CIRCLE('',#69919,0.0999999999999997) ;
#25863=CIRCLE('',#69921,0.0999999999999994) ;
#25864=CIRCLE('',#69922,0.1) ;
#25865=CIRCLE('',#69924,0.1) ;
#25866=CIRCLE('',#69926,0.1) ;
#25867=CIRCLE('',#69928,0.1) ;
#25868=CIRCLE('',#69929,0.1) ;
#25869=CIRCLE('',#69931,0.1) ;
#25870=CIRCLE('',#69933,0.1) ;
#25871=CIRCLE('',#69935,0.1) ;
#25872=CIRCLE('',#69936,0.1) ;
#25873=CIRCLE('',#69938,0.1) ;
#25874=CIRCLE('',#69941,0.0999999999999994) ;
#25875=CIRCLE('',#69943,0.0999999999999994) ;
#25876=CIRCLE('',#69947,0.1) ;
#25877=CIRCLE('',#69949,0.0999999999999994) ;
#25878=CIRCLE('',#69951,0.0999999999999999) ;
#25879=CIRCLE('',#69952,0.1) ;
#25880=CIRCLE('',#69955,0.1) ;
#25881=CIRCLE('',#69956,0.0999999999999998) ;
#25882=CIRCLE('',#69958,0.1) ;
#25883=CIRCLE('',#69960,0.1) ;
#25884=CIRCLE('',#69962,0.0999999999999998) ;
#25885=CIRCLE('',#69964,0.1) ;
#25886=CIRCLE('',#69966,0.1) ;
#25887=CIRCLE('',#69968,0.1) ;
#25888=CIRCLE('',#69971,0.0999999999999994) ;
#25889=CIRCLE('',#69972,0.1) ;
#25890=CIRCLE('',#69974,0.0999999999999994) ;
#25891=CIRCLE('',#69976,0.1) ;
#25892=CIRCLE('',#69978,0.1) ;
#25893=CIRCLE('',#69980,0.1) ;
#25894=CIRCLE('',#69982,0.1) ;
#25895=CIRCLE('',#69984,0.0999999999999994) ;
#25896=CIRCLE('',#69987,0.0999999999999994) ;
#25897=CIRCLE('',#69989,0.0999999999999999) ;
#25898=CIRCLE('',#69990,0.0999999999999999) ;
#25899=CIRCLE('',#69994,0.0999999999999994) ;
#25900=CIRCLE('',#69996,0.0999999999999994) ;
#25901=CIRCLE('',#70000,0.1) ;
#25902=CIRCLE('',#70002,0.0999999999999997) ;
#25903=CIRCLE('',#70004,0.0999999999999994) ;
#25904=CIRCLE('',#70007,1.4) ;
#25905=CIRCLE('',#70008,0.1) ;
#25906=CIRCLE('',#70009,1.5) ;
#25907=CIRCLE('',#70011,1.5) ;
#25908=CIRCLE('',#70012,0.1) ;
#25909=CIRCLE('',#70013,1.6) ;
#25910=CIRCLE('',#70015,0.0999999999999994) ;
#25911=CIRCLE('',#70016,0.0999999999999994) ;
#25912=CIRCLE('',#70017,0.0999999999999994) ;
#25913=CIRCLE('',#70019,0.0999999999999994) ;
#25914=CIRCLE('',#70020,0.1) ;
#25915=CIRCLE('',#70022,3.) ;
#25916=CIRCLE('',#70023,0.1) ;
#25917=CIRCLE('',#70024,3.00136060761679) ;
#25918=CIRCLE('',#70025,0.1) ;
#25919=CIRCLE('',#70028,3.) ;
#25920=CIRCLE('',#70029,3.) ;
#25921=CIRCLE('',#70030,3.) ;
#25922=CIRCLE('',#70039,3.33471270883832) ;
#25923=CIRCLE('',#70041,0.0999999999999994) ;
#25924=CIRCLE('',#70042,0.0999999999999994) ;
#25925=CIRCLE('',#70043,0.0999999999999994) ;
#25926=CIRCLE('',#70044,0.0999999999999994) ;
#25927=CIRCLE('',#70045,0.1) ;
#25928=CIRCLE('',#70046,0.1) ;
#25929=CIRCLE('',#70047,0.1) ;
#25930=CIRCLE('',#70048,0.1) ;
#25931=CIRCLE('',#70049,0.1) ;
#25932=CIRCLE('',#70050,0.1) ;
#25933=CIRCLE('',#70051,0.0999999999999994) ;
#25934=CIRCLE('',#70052,0.0999999999999994) ;
#25935=CIRCLE('',#70053,0.0999999999999994) ;
#25936=CIRCLE('',#70054,0.1) ;
#25937=CIRCLE('',#70055,0.1) ;
#25938=CIRCLE('',#70056,0.1) ;
#25939=CIRCLE('',#70058,0.0999999999999994) ;
#25940=CIRCLE('',#70059,0.1) ;
#25941=CIRCLE('',#70060,0.1) ;
#25942=CIRCLE('',#70061,0.1) ;
#25943=CIRCLE('',#70062,0.0999999999999994) ;
#25944=CIRCLE('',#70063,0.0999999999999994) ;
#25945=CIRCLE('',#70064,0.0999999999999994) ;
#25946=CIRCLE('',#70065,0.1) ;
#25947=CIRCLE('',#70066,0.1) ;
#25948=CIRCLE('',#70067,0.1) ;
#25949=CIRCLE('',#70068,0.1) ;
#25950=CIRCLE('',#70069,0.1) ;
#25951=CIRCLE('',#70070,0.1) ;
#25952=CIRCLE('',#70071,0.0999999999999994) ;
#25953=CIRCLE('',#70072,0.0999999999999994) ;
#25954=CIRCLE('',#70073,0.0999999999999994) ;
#25955=CIRCLE('',#70082,0.200000000000001) ;
#25956=CIRCLE('',#70083,0.200000000000001) ;
#25957=CIRCLE('',#70085,0.2) ;
#25958=CIRCLE('',#70086,0.2) ;
#25959=CIRCLE('',#70087,1.65) ;
#25960=CIRCLE('',#70088,0.2) ;
#25961=CIRCLE('',#70089,0.2) ;
#25962=CIRCLE('',#70090,1.65) ;
#25963=CIRCLE('',#70091,0.2) ;
#25964=CIRCLE('',#70092,0.2) ;
#25965=CIRCLE('',#70093,1.65) ;
#25966=CIRCLE('',#70094,0.2) ;
#25967=CIRCLE('',#70095,2.9) ;
#25968=CIRCLE('',#70096,0.2) ;
#25969=CIRCLE('',#70097,1.65) ;
#25970=CIRCLE('',#70099,0.200000000000001) ;
#25971=CIRCLE('',#70100,0.200000000000001) ;
#25972=CIRCLE('',#70102,0.2) ;
#25973=CIRCLE('',#70103,0.2) ;
#25974=CIRCLE('',#70105,0.2) ;
#25975=CIRCLE('',#70107,0.2) ;
#25976=CIRCLE('',#70115,0.1) ;
#25977=CIRCLE('',#70116,0.1) ;
#25978=CIRCLE('',#70117,0.0999999999999998) ;
#25979=CIRCLE('',#70118,0.0999999999999998) ;
#25980=CIRCLE('',#70120,0.2) ;
#25981=CIRCLE('',#70121,1.85) ;
#25982=CIRCLE('',#70122,2.9) ;
#25983=CIRCLE('',#70126,1.75) ;
#25984=CIRCLE('',#70127,1.75) ;
#25985=CIRCLE('',#70129,1.75) ;
#25986=CIRCLE('',#70130,1.75) ;
#25987=CIRCLE('',#70134,1.85) ;
#25988=CIRCLE('',#70135,0.2) ;
#25989=CIRCLE('',#70136,2.9) ;
#25990=CIRCLE('',#70138,1.85) ;
#25991=CIRCLE('',#70141,1.75) ;
#25992=CIRCLE('',#70142,1.75) ;
#25993=CIRCLE('',#70145,1.75) ;
#25994=CIRCLE('',#70146,1.75) ;
#25995=CIRCLE('',#70150,1.85) ;
#25996=CIRCLE('',#70165,1.1) ;
#25997=CIRCLE('',#70166,1.9) ;
#25998=CIRCLE('',#70168,1.9) ;
#25999=CIRCLE('',#70169,1.1) ;
#26000=CIRCLE('',#70171,2.) ;
#26001=CIRCLE('',#70172,2.) ;
#26002=CIRCLE('',#70179,1.) ;
#26003=CIRCLE('',#70180,1.) ;
#26004=CIRCLE('',#70186,609.695408627795) ;
#26005=CIRCLE('',#70188,3.23607331645511) ;
#26006=CIRCLE('',#70189,576.383428977096) ;
#26007=CIRCLE('',#70190,576.383429600196) ;
#26008=CIRCLE('',#70192,609.695407714902) ;
#26009=CIRCLE('',#70194,0.1) ;
#26010=CIRCLE('',#70196,0.0999999999999995) ;
#26011=CIRCLE('',#70197,0.0999999999999994) ;
#26012=CIRCLE('',#70199,0.1) ;
#26013=CIRCLE('',#70201,0.1) ;
#26014=CIRCLE('',#70203,0.0999999999999999) ;
#26015=CIRCLE('',#70205,0.0999999999999995) ;
#26016=CIRCLE('',#70207,0.0999999999999994) ;
#26017=CIRCLE('',#70208,0.0999999999999994) ;
#26018=CIRCLE('',#70210,0.1) ;
#26019=CIRCLE('',#70212,0.1) ;
#26020=CIRCLE('',#70213,0.0999999999999994) ;
#26021=CIRCLE('',#70215,0.1) ;
#26022=CIRCLE('',#70217,0.0999999999999999) ;
#26023=CIRCLE('',#70219,0.1) ;
#26024=CIRCLE('',#70221,0.0999999999999994) ;
#26025=CIRCLE('',#70223,0.1) ;
#26026=CIRCLE('',#70225,0.0999999999999995) ;
#26027=CIRCLE('',#70227,0.0999999999999995) ;
#26028=CIRCLE('',#70229,0.0999999999999994) ;
#26029=CIRCLE('',#70231,0.0999999999999994) ;
#26030=CIRCLE('',#70233,0.0999999999999999) ;
#26031=CIRCLE('',#70235,0.1) ;
#26032=CIRCLE('',#70236,0.0999999999999994) ;
#26033=CIRCLE('',#70238,0.0999999999999999) ;
#26034=CIRCLE('',#70240,0.0999999999999994) ;
#26035=CIRCLE('',#70242,0.0999999999999994) ;
#26036=CIRCLE('',#70244,0.0999999999999994) ;
#26037=CIRCLE('',#70246,0.0999999999999994) ;
#26038=CIRCLE('',#70248,0.1) ;
#26039=CIRCLE('',#70250,0.1) ;
#26040=CIRCLE('',#70252,0.0999999999999994) ;
#26041=CIRCLE('',#70254,0.0999999999999994) ;
#26042=CIRCLE('',#70256,0.1) ;
#26043=CIRCLE('',#70258,0.0999999999999994) ;
#26044=CIRCLE('',#70260,0.0999999999999994) ;
#26045=CIRCLE('',#70263,0.1) ;
#26046=CIRCLE('',#70264,0.0999999999999994) ;
#26047=CIRCLE('',#70265,0.1) ;
#26048=CIRCLE('',#70271,0.1) ;
#26049=CIRCLE('',#70279,0.0999999999999994) ;
#26050=CIRCLE('',#70280,0.0999999999999994) ;
#26051=CIRCLE('',#70282,0.0999999999999994) ;
#26052=CIRCLE('',#70284,0.0999999999999994) ;
#26053=CIRCLE('',#70285,0.1) ;
#26054=CIRCLE('',#70288,0.0999999999999994) ;
#26055=CIRCLE('',#70291,0.0999999999999994) ;
#26056=CIRCLE('',#70293,0.0999999999999994) ;
#26057=CIRCLE('',#70296,0.0999999999999994) ;
#26058=CIRCLE('',#70298,0.1) ;
#26059=CIRCLE('',#70300,0.1) ;
#26060=CIRCLE('',#70302,0.1) ;
#26061=CIRCLE('',#70304,0.0999999999999994) ;
#26062=CIRCLE('',#70305,0.1) ;
#26063=CIRCLE('',#70307,0.0999999999999994) ;
#26064=CIRCLE('',#70309,0.1) ;
#26065=CIRCLE('',#70311,0.0999999999999994) ;
#26066=CIRCLE('',#70312,0.1) ;
#26067=CIRCLE('',#70314,0.1) ;
#26068=CIRCLE('',#70316,0.1) ;
#26069=CIRCLE('',#70318,0.1) ;
#26070=CIRCLE('',#70320,0.0999999999999994) ;
#26071=CIRCLE('',#70322,0.0999999999999994) ;
#26072=CIRCLE('',#70324,0.0999999999999994) ;
#26073=CIRCLE('',#70326,0.0999999999999994) ;
#26074=CIRCLE('',#70327,0.0999999999999994) ;
#26075=CIRCLE('',#70329,0.1) ;
#26076=CIRCLE('',#70334,0.0999999999999994) ;
#26077=CIRCLE('',#70337,0.0999999999999998) ;
#26078=CIRCLE('',#70339,0.0999999999999995) ;
#26079=CIRCLE('',#70340,0.0999999999999994) ;
#26080=CIRCLE('',#70342,0.1) ;
#26081=CIRCLE('',#70344,0.0999999999999998) ;
#26082=CIRCLE('',#70346,0.0999999999999999) ;
#26083=CIRCLE('',#70348,0.1) ;
#26084=CIRCLE('',#70350,0.1) ;
#26085=CIRCLE('',#70351,0.1) ;
#26086=CIRCLE('',#70353,0.0999999999999995) ;
#26087=CIRCLE('',#70355,0.0999999999999994) ;
#26088=CIRCLE('',#70356,0.0999999999999994) ;
#26089=CIRCLE('',#70358,0.0999999999999999) ;
#26090=CIRCLE('',#70360,0.0999999999999995) ;
#26091=CIRCLE('',#70362,0.0999999999999998) ;
#26092=CIRCLE('',#70364,0.0999999999999994) ;
#26093=CIRCLE('',#70366,0.1) ;
#26094=CIRCLE('',#70368,0.1) ;
#26095=CIRCLE('',#70369,0.1) ;
#26096=CIRCLE('',#70371,0.1) ;
#26097=CIRCLE('',#70373,0.1) ;
#26098=CIRCLE('',#70375,0.0999999999999994) ;
#26099=CIRCLE('',#70378,0.0999999999999999) ;
#26100=CIRCLE('',#70380,0.0999999999999994) ;
#26101=CIRCLE('',#70381,0.0999999999999993) ;
#26102=CIRCLE('',#70384,0.1) ;
#26103=CIRCLE('',#70386,0.0999999999999994) ;
#26104=CIRCLE('',#70387,0.0999999999999994) ;
#26105=CIRCLE('',#70389,0.0999999999999995) ;
#26106=CIRCLE('',#70391,0.0999999999999998) ;
#26107=CIRCLE('',#70393,0.1) ;
#26108=CIRCLE('',#70394,0.1) ;
#26109=CIRCLE('',#70396,0.1) ;
#26110=CIRCLE('',#70398,0.0999999999999994) ;
#26111=CIRCLE('',#70400,0.0999999999999995) ;
#26112=CIRCLE('',#70402,0.1) ;
#26113=CIRCLE('',#70404,0.0999999999999998) ;
#26114=CIRCLE('',#70406,0.0999999999999995) ;
#26115=CIRCLE('',#70408,0.0999999999999994) ;
#26116=CIRCLE('',#70411,0.0999999999999994) ;
#26117=CIRCLE('',#70413,0.0999999999999994) ;
#26118=CIRCLE('',#70415,0.1) ;
#26119=CIRCLE('',#70417,0.1) ;
#26120=CIRCLE('',#70418,0.0999999999999995) ;
#26121=CIRCLE('',#70420,0.0999999999999994) ;
#26122=CIRCLE('',#70422,0.0999999999999994) ;
#26123=CIRCLE('',#70424,0.1) ;
#26124=CIRCLE('',#70425,0.0999999999999998) ;
#26125=CIRCLE('',#70427,0.0999999999999994) ;
#26126=CIRCLE('',#70429,0.1) ;
#26127=CIRCLE('',#70430,0.1) ;
#26128=CIRCLE('',#70432,0.0999999999999994) ;
#26129=CIRCLE('',#70434,0.0999999999999998) ;
#26130=CIRCLE('',#70436,0.1) ;
#26131=CIRCLE('',#70437,0.1) ;
#26132=CIRCLE('',#70439,0.0999999999999998) ;
#26133=CIRCLE('',#70441,0.0999999999999994) ;
#26134=CIRCLE('',#70443,0.1) ;
#26135=CIRCLE('',#70445,0.0999999999999998) ;
#26136=CIRCLE('',#70447,0.100000000000001) ;
#26137=CIRCLE('',#70449,0.1) ;
#26138=CIRCLE('',#70451,0.0999999999999994) ;
#26139=CIRCLE('',#70452,0.1) ;
#26140=CIRCLE('',#70455,0.0999999999999998) ;
#26141=CIRCLE('',#70457,0.1) ;
#26142=CIRCLE('',#70459,0.1) ;
#26143=CIRCLE('',#70460,0.0999999999999995) ;
#26144=CIRCLE('',#70462,0.0999999999999995) ;
#26145=CIRCLE('',#70463,0.0999999999999998) ;
#26146=CIRCLE('',#70465,0.0999999999999994) ;
#26147=CIRCLE('',#70466,0.0999999999999994) ;
#26148=CIRCLE('',#70468,0.0999999999999998) ;
#26149=CIRCLE('',#70470,0.0999999999999998) ;
#26150=CIRCLE('',#70472,0.1) ;
#26151=CIRCLE('',#70474,0.0999999999999994) ;
#26152=CIRCLE('',#70476,0.0999999999999994) ;
#26153=CIRCLE('',#70478,0.1) ;
#26154=CIRCLE('',#70479,0.0999999999999995) ;
#26155=CIRCLE('',#70481,0.1) ;
#26156=CIRCLE('',#70482,0.0999999999999995) ;
#26157=CIRCLE('',#70484,0.0999999999999998) ;
#26158=CIRCLE('',#70486,0.0999999999999994) ;
#26159=CIRCLE('',#70488,0.0999999999999994) ;
#26160=CIRCLE('',#70491,0.0999999999999994) ;
#26161=CIRCLE('',#70493,0.0999999999999995) ;
#26162=CIRCLE('',#70495,0.0999999999999994) ;
#26163=CIRCLE('',#70497,0.1) ;
#26164=CIRCLE('',#70499,0.0999999999999994) ;
#26165=CIRCLE('',#70501,0.0999999999999998) ;
#26166=CIRCLE('',#70505,0.0999999999999995) ;
#26167=CIRCLE('',#70507,0.1) ;
#26168=CIRCLE('',#70509,0.0999999999999994) ;
#26169=CIRCLE('',#70511,0.0999999999999994) ;
#26170=CIRCLE('',#70513,0.0999999999999994) ;
#26171=CIRCLE('',#70515,0.100000000000001) ;
#26172=CIRCLE('',#70519,0.1) ;
#26173=CIRCLE('',#70520,0.1) ;
#26174=CIRCLE('',#70526,0.0999999999999994) ;
#26175=CIRCLE('',#70528,0.1) ;
#26176=CIRCLE('',#70529,0.1) ;
#26177=CIRCLE('',#70531,0.0999999999999994) ;
#26178=CIRCLE('',#70532,0.1) ;
#26179=CIRCLE('',#70534,0.0999999999999994) ;
#26180=CIRCLE('',#70536,0.0999999999999994) ;
#26181=CIRCLE('',#70538,0.0999999999999994) ;
#26182=CIRCLE('',#70539,0.0999999999999994) ;
#26183=CIRCLE('',#70541,0.0999999999999994) ;
#26184=CIRCLE('',#70543,0.0999999999999994) ;
#26185=CIRCLE('',#70545,0.1) ;
#26186=CIRCLE('',#70546,0.0999999999999994) ;
#26187=CIRCLE('',#70548,0.0999999999999994) ;
#26188=CIRCLE('',#70551,0.0999999999999994) ;
#26189=CIRCLE('',#70553,0.0999999999999994) ;
#26190=CIRCLE('',#70557,0.0999999999999994) ;
#26191=CIRCLE('',#70559,0.0999999999999994) ;
#26192=CIRCLE('',#70561,0.0999999999999999) ;
#26193=CIRCLE('',#70562,0.1) ;
#26194=CIRCLE('',#70565,0.1) ;
#26195=CIRCLE('',#70566,0.0999999999999998) ;
#26196=CIRCLE('',#70568,0.1) ;
#26197=CIRCLE('',#70570,0.0999999999999994) ;
#26198=CIRCLE('',#70572,0.0999999999999998) ;
#26199=CIRCLE('',#70574,0.1) ;
#26200=CIRCLE('',#70576,0.0999999999999994) ;
#26201=CIRCLE('',#70578,0.1) ;
#26202=CIRCLE('',#70581,0.0999999999999994) ;
#26203=CIRCLE('',#70582,0.0999999999999994) ;
#26204=CIRCLE('',#70584,0.0999999999999994) ;
#26205=CIRCLE('',#70586,0.0999999999999994) ;
#26206=CIRCLE('',#70588,0.0999999999999994) ;
#26207=CIRCLE('',#70590,0.1) ;
#26208=CIRCLE('',#70592,0.0999999999999994) ;
#26209=CIRCLE('',#70594,0.0999999999999994) ;
#26210=CIRCLE('',#70597,0.0999999999999994) ;
#26211=CIRCLE('',#70599,0.0999999999999999) ;
#26212=CIRCLE('',#70600,0.0999999999999999) ;
#26213=CIRCLE('',#70604,0.0999999999999994) ;
#26214=CIRCLE('',#70606,0.0999999999999994) ;
#26215=CIRCLE('',#70610,0.1) ;
#26216=CIRCLE('',#70612,0.0999999999999997) ;
#26217=CIRCLE('',#70614,0.0999999999999994) ;
#26218=CIRCLE('',#70617,1.4) ;
#26219=CIRCLE('',#70618,0.1) ;
#26220=CIRCLE('',#70619,1.5) ;
#26221=CIRCLE('',#70621,1.5) ;
#26222=CIRCLE('',#70622,0.1) ;
#26223=CIRCLE('',#70623,1.6) ;
#26224=CIRCLE('',#70625,0.0999999999999994) ;
#26225=CIRCLE('',#70626,0.0999999999999994) ;
#26226=CIRCLE('',#70627,0.0999999999999994) ;
#26227=CIRCLE('',#70629,0.0999999999999994) ;
#26228=CIRCLE('',#70630,0.1) ;
#26229=CIRCLE('',#70632,3.) ;
#26230=CIRCLE('',#70633,0.1) ;
#26231=CIRCLE('',#70634,3.00136060761679) ;
#26232=CIRCLE('',#70635,0.100000000000001) ;
#26233=CIRCLE('',#70638,3.) ;
#26234=CIRCLE('',#70639,3.) ;
#26235=CIRCLE('',#70640,3.) ;
#26236=CIRCLE('',#70649,3.33471270883832) ;
#26237=CIRCLE('',#70651,0.0999999999999994) ;
#26238=CIRCLE('',#70652,0.0999999999999994) ;
#26239=CIRCLE('',#70653,0.0999999999999994) ;
#26240=CIRCLE('',#70654,0.0999999999999994) ;
#26241=CIRCLE('',#70655,0.1) ;
#26242=CIRCLE('',#70656,0.1) ;
#26243=CIRCLE('',#70657,0.1) ;
#26244=CIRCLE('',#70658,0.1) ;
#26245=CIRCLE('',#70659,0.1) ;
#26246=CIRCLE('',#70660,0.1) ;
#26247=CIRCLE('',#70661,0.0999999999999994) ;
#26248=CIRCLE('',#70662,0.0999999999999994) ;
#26249=CIRCLE('',#70663,0.0999999999999994) ;
#26250=CIRCLE('',#70664,0.1) ;
#26251=CIRCLE('',#70665,0.1) ;
#26252=CIRCLE('',#70666,0.1) ;
#26253=CIRCLE('',#70668,0.0999999999999994) ;
#26254=CIRCLE('',#70669,0.1) ;
#26255=CIRCLE('',#70670,0.1) ;
#26256=CIRCLE('',#70671,0.1) ;
#26257=CIRCLE('',#70672,0.0999999999999994) ;
#26258=CIRCLE('',#70673,0.0999999999999994) ;
#26259=CIRCLE('',#70674,0.0999999999999994) ;
#26260=CIRCLE('',#70675,0.1) ;
#26261=CIRCLE('',#70676,0.1) ;
#26262=CIRCLE('',#70677,0.1) ;
#26263=CIRCLE('',#70678,0.1) ;
#26264=CIRCLE('',#70679,0.1) ;
#26265=CIRCLE('',#70680,0.1) ;
#26266=CIRCLE('',#70681,0.0999999999999994) ;
#26267=CIRCLE('',#70682,0.0999999999999994) ;
#26268=CIRCLE('',#70683,0.0999999999999994) ;
#26269=CIRCLE('',#70692,0.200000000000001) ;
#26270=CIRCLE('',#70693,0.199999999999999) ;
#26271=CIRCLE('',#70695,0.2) ;
#26272=CIRCLE('',#70696,0.2) ;
#26273=CIRCLE('',#70697,1.65) ;
#26274=CIRCLE('',#70698,0.2) ;
#26275=CIRCLE('',#70699,0.2) ;
#26276=CIRCLE('',#70700,1.65) ;
#26277=CIRCLE('',#70701,0.2) ;
#26278=CIRCLE('',#70702,0.2) ;
#26279=CIRCLE('',#70703,1.65) ;
#26280=CIRCLE('',#70704,0.2) ;
#26281=CIRCLE('',#70705,2.9) ;
#26282=CIRCLE('',#70706,0.2) ;
#26283=CIRCLE('',#70707,1.65) ;
#26284=CIRCLE('',#70709,0.199999999999999) ;
#26285=CIRCLE('',#70710,0.200000000000001) ;
#26286=CIRCLE('',#70712,0.2) ;
#26287=CIRCLE('',#70713,0.2) ;
#26288=CIRCLE('',#70715,0.2) ;
#26289=CIRCLE('',#70717,0.2) ;
#26290=CIRCLE('',#70725,0.1) ;
#26291=CIRCLE('',#70726,0.1) ;
#26292=CIRCLE('',#70727,0.0999999999999998) ;
#26293=CIRCLE('',#70728,0.0999999999999998) ;
#26294=CIRCLE('',#70730,0.2) ;
#26295=CIRCLE('',#70731,1.85) ;
#26296=CIRCLE('',#70732,2.9) ;
#26297=CIRCLE('',#70736,1.75) ;
#26298=CIRCLE('',#70737,1.75) ;
#26299=CIRCLE('',#70739,1.75) ;
#26300=CIRCLE('',#70740,1.75) ;
#26301=CIRCLE('',#70744,1.85) ;
#26302=CIRCLE('',#70745,0.2) ;
#26303=CIRCLE('',#70746,2.9) ;
#26304=CIRCLE('',#70748,1.85) ;
#26305=CIRCLE('',#70751,1.75) ;
#26306=CIRCLE('',#70752,1.75) ;
#26307=CIRCLE('',#70755,1.75) ;
#26308=CIRCLE('',#70756,1.75) ;
#26309=CIRCLE('',#70760,1.85) ;
#26310=CIRCLE('',#70775,1.1) ;
#26311=CIRCLE('',#70776,1.9) ;
#26312=CIRCLE('',#70778,1.9) ;
#26313=CIRCLE('',#70779,1.1) ;
#26314=CIRCLE('',#70781,2.) ;
#26315=CIRCLE('',#70782,2.) ;
#26316=CIRCLE('',#70789,1.) ;
#26317=CIRCLE('',#70790,1.) ;
#26318=CIRCLE('',#70796,609.695408630063) ;
#26319=CIRCLE('',#70798,3.23607331645511) ;
#26320=CIRCLE('',#70799,576.383429457373) ;
#26321=CIRCLE('',#70800,576.38342959882) ;
#26322=CIRCLE('',#70802,609.695409345007) ;
#26323=CIRCLE('',#70804,0.1) ;
#26324=CIRCLE('',#70806,0.0999999999999995) ;
#26325=CIRCLE('',#70807,0.0999999999999994) ;
#26326=CIRCLE('',#70809,0.1) ;
#26327=CIRCLE('',#70811,0.1) ;
#26328=CIRCLE('',#70813,0.0999999999999999) ;
#26329=CIRCLE('',#70815,0.0999999999999995) ;
#26330=CIRCLE('',#70817,0.0999999999999994) ;
#26331=CIRCLE('',#70818,0.0999999999999994) ;
#26332=CIRCLE('',#70820,0.1) ;
#26333=CIRCLE('',#70822,0.1) ;
#26334=CIRCLE('',#70823,0.0999999999999994) ;
#26335=CIRCLE('',#70825,0.1) ;
#26336=CIRCLE('',#70827,0.0999999999999999) ;
#26337=CIRCLE('',#70829,0.1) ;
#26338=CIRCLE('',#70831,0.0999999999999994) ;
#26339=CIRCLE('',#70833,0.1) ;
#26340=CIRCLE('',#70835,0.0999999999999995) ;
#26341=CIRCLE('',#70837,0.0999999999999995) ;
#26342=CIRCLE('',#70839,0.0999999999999994) ;
#26343=CIRCLE('',#70841,0.0999999999999994) ;
#26344=CIRCLE('',#70843,0.0999999999999999) ;
#26345=CIRCLE('',#70845,0.1) ;
#26346=CIRCLE('',#70846,0.0999999999999994) ;
#26347=CIRCLE('',#70848,0.0999999999999999) ;
#26348=CIRCLE('',#70850,0.0999999999999994) ;
#26349=CIRCLE('',#70852,0.0999999999999994) ;
#26350=CIRCLE('',#70854,0.0999999999999994) ;
#26351=CIRCLE('',#70856,0.0999999999999994) ;
#26352=CIRCLE('',#70858,0.1) ;
#26353=CIRCLE('',#70860,0.1) ;
#26354=CIRCLE('',#70862,0.0999999999999994) ;
#26355=CIRCLE('',#70864,0.0999999999999994) ;
#26356=CIRCLE('',#70866,0.1) ;
#26357=CIRCLE('',#70868,0.0999999999999994) ;
#26358=CIRCLE('',#70870,0.0999999999999994) ;
#26359=CIRCLE('',#70873,0.1) ;
#26360=CIRCLE('',#70874,0.0999999999999994) ;
#26361=CIRCLE('',#70875,0.1) ;
#26362=CIRCLE('',#70881,0.1) ;
#26363=CIRCLE('',#70889,0.0999999999999994) ;
#26364=CIRCLE('',#70890,0.0999999999999994) ;
#26365=CIRCLE('',#70892,0.0999999999999994) ;
#26366=CIRCLE('',#70894,0.0999999999999994) ;
#26367=CIRCLE('',#70895,0.1) ;
#26368=CIRCLE('',#70898,0.0999999999999994) ;
#26369=CIRCLE('',#70901,0.0999999999999994) ;
#26370=CIRCLE('',#70903,0.0999999999999994) ;
#26371=CIRCLE('',#70906,0.0999999999999994) ;
#26372=CIRCLE('',#70908,0.1) ;
#26373=CIRCLE('',#70910,0.1) ;
#26374=CIRCLE('',#70912,0.1) ;
#26375=CIRCLE('',#70914,0.0999999999999994) ;
#26376=CIRCLE('',#70915,0.1) ;
#26377=CIRCLE('',#70917,0.0999999999999994) ;
#26378=CIRCLE('',#70919,0.1) ;
#26379=CIRCLE('',#70921,0.0999999999999994) ;
#26380=CIRCLE('',#70922,0.1) ;
#26381=CIRCLE('',#70924,0.1) ;
#26382=CIRCLE('',#70926,0.1) ;
#26383=CIRCLE('',#70928,0.1) ;
#26384=CIRCLE('',#70930,0.0999999999999994) ;
#26385=CIRCLE('',#70932,0.0999999999999994) ;
#26386=CIRCLE('',#70934,0.0999999999999994) ;
#26387=CIRCLE('',#70936,0.0999999999999994) ;
#26388=CIRCLE('',#70937,0.0999999999999994) ;
#26389=CIRCLE('',#70939,0.1) ;
#26390=CIRCLE('',#70944,0.0999999999999994) ;
#26391=CIRCLE('',#70947,0.0999999999999998) ;
#26392=CIRCLE('',#70949,0.0999999999999995) ;
#26393=CIRCLE('',#70950,0.0999999999999994) ;
#26394=CIRCLE('',#70952,0.1) ;
#26395=CIRCLE('',#70954,0.0999999999999998) ;
#26396=CIRCLE('',#70956,0.0999999999999999) ;
#26397=CIRCLE('',#70958,0.1) ;
#26398=CIRCLE('',#70960,0.1) ;
#26399=CIRCLE('',#70961,0.1) ;
#26400=CIRCLE('',#70963,0.0999999999999995) ;
#26401=CIRCLE('',#70965,0.0999999999999994) ;
#26402=CIRCLE('',#70966,0.0999999999999994) ;
#26403=CIRCLE('',#70968,0.100000000000001) ;
#26404=CIRCLE('',#70970,0.0999999999999995) ;
#26405=CIRCLE('',#70972,0.0999999999999998) ;
#26406=CIRCLE('',#70974,0.0999999999999994) ;
#26407=CIRCLE('',#70976,0.100000000000001) ;
#26408=CIRCLE('',#70978,0.1) ;
#26409=CIRCLE('',#70979,0.1) ;
#26410=CIRCLE('',#70981,0.1) ;
#26411=CIRCLE('',#70983,0.1) ;
#26412=CIRCLE('',#70985,0.0999999999999994) ;
#26413=CIRCLE('',#70988,0.0999999999999999) ;
#26414=CIRCLE('',#70990,0.0999999999999994) ;
#26415=CIRCLE('',#70991,0.0999999999999993) ;
#26416=CIRCLE('',#70994,0.1) ;
#26417=CIRCLE('',#70996,0.0999999999999994) ;
#26418=CIRCLE('',#70997,0.0999999999999994) ;
#26419=CIRCLE('',#70999,0.0999999999999995) ;
#26420=CIRCLE('',#71001,0.0999999999999998) ;
#26421=CIRCLE('',#71003,0.1) ;
#26422=CIRCLE('',#71004,0.1) ;
#26423=CIRCLE('',#71006,0.1) ;
#26424=CIRCLE('',#71008,0.0999999999999994) ;
#26425=CIRCLE('',#71010,0.0999999999999995) ;
#26426=CIRCLE('',#71012,0.1) ;
#26427=CIRCLE('',#71014,0.0999999999999998) ;
#26428=CIRCLE('',#71016,0.0999999999999995) ;
#26429=CIRCLE('',#71018,0.0999999999999994) ;
#26430=CIRCLE('',#71021,0.0999999999999994) ;
#26431=CIRCLE('',#71023,0.0999999999999994) ;
#26432=CIRCLE('',#71025,0.1) ;
#26433=CIRCLE('',#71027,0.1) ;
#26434=CIRCLE('',#71028,0.0999999999999995) ;
#26435=CIRCLE('',#71030,0.0999999999999994) ;
#26436=CIRCLE('',#71032,0.0999999999999994) ;
#26437=CIRCLE('',#71034,0.1) ;
#26438=CIRCLE('',#71035,0.0999999999999998) ;
#26439=CIRCLE('',#71037,0.0999999999999994) ;
#26440=CIRCLE('',#71039,0.1) ;
#26441=CIRCLE('',#71040,0.1) ;
#26442=CIRCLE('',#71042,0.0999999999999994) ;
#26443=CIRCLE('',#71044,0.0999999999999998) ;
#26444=CIRCLE('',#71046,0.1) ;
#26445=CIRCLE('',#71047,0.1) ;
#26446=CIRCLE('',#71049,0.0999999999999998) ;
#26447=CIRCLE('',#71051,0.0999999999999994) ;
#26448=CIRCLE('',#71053,0.1) ;
#26449=CIRCLE('',#71055,0.0999999999999998) ;
#26450=CIRCLE('',#71057,0.100000000000001) ;
#26451=CIRCLE('',#71059,0.1) ;
#26452=CIRCLE('',#71061,0.0999999999999994) ;
#26453=CIRCLE('',#71062,0.1) ;
#26454=CIRCLE('',#71065,0.0999999999999998) ;
#26455=CIRCLE('',#71067,0.1) ;
#26456=CIRCLE('',#71069,0.1) ;
#26457=CIRCLE('',#71070,0.0999999999999995) ;
#26458=CIRCLE('',#71072,0.1) ;
#26459=CIRCLE('',#71073,0.0999999999999998) ;
#26460=CIRCLE('',#71075,0.0999999999999994) ;
#26461=CIRCLE('',#71076,0.0999999999999994) ;
#26462=CIRCLE('',#71078,0.0999999999999998) ;
#26463=CIRCLE('',#71080,0.0999999999999998) ;
#26464=CIRCLE('',#71082,0.1) ;
#26465=CIRCLE('',#71084,0.0999999999999994) ;
#26466=CIRCLE('',#71086,0.0999999999999994) ;
#26467=CIRCLE('',#71088,0.1) ;
#26468=CIRCLE('',#71089,0.0999999999999995) ;
#26469=CIRCLE('',#71091,0.1) ;
#26470=CIRCLE('',#71092,0.0999999999999995) ;
#26471=CIRCLE('',#71094,0.0999999999999998) ;
#26472=CIRCLE('',#71096,0.0999999999999994) ;
#26473=CIRCLE('',#71098,0.0999999999999994) ;
#26474=CIRCLE('',#71101,0.0999999999999994) ;
#26475=CIRCLE('',#71103,0.0999999999999995) ;
#26476=CIRCLE('',#71105,0.0999999999999994) ;
#26477=CIRCLE('',#71107,0.1) ;
#26478=CIRCLE('',#71109,0.0999999999999994) ;
#26479=CIRCLE('',#71111,0.0999999999999998) ;
#26480=CIRCLE('',#71115,0.0999999999999995) ;
#26481=CIRCLE('',#71117,0.1) ;
#26482=CIRCLE('',#71119,0.0999999999999994) ;
#26483=CIRCLE('',#71121,0.0999999999999994) ;
#26484=CIRCLE('',#71123,0.0999999999999994) ;
#26485=CIRCLE('',#71125,0.100000000000001) ;
#26486=CIRCLE('',#71129,0.1) ;
#26487=CIRCLE('',#71130,0.1) ;
#26488=CIRCLE('',#71136,0.0999999999999994) ;
#26489=CIRCLE('',#71138,0.1) ;
#26490=CIRCLE('',#71139,0.1) ;
#26491=CIRCLE('',#71141,0.0999999999999994) ;
#26492=CIRCLE('',#71142,0.1) ;
#26493=CIRCLE('',#71144,0.0999999999999994) ;
#26494=CIRCLE('',#71146,0.0999999999999994) ;
#26495=CIRCLE('',#71148,0.0999999999999994) ;
#26496=CIRCLE('',#71149,0.0999999999999994) ;
#26497=CIRCLE('',#71151,0.0999999999999994) ;
#26498=CIRCLE('',#71153,0.0999999999999994) ;
#26499=CIRCLE('',#71155,0.1) ;
#26500=CIRCLE('',#71156,0.0999999999999994) ;
#26501=CIRCLE('',#71158,0.0999999999999994) ;
#26502=CIRCLE('',#71161,0.0999999999999994) ;
#26503=CIRCLE('',#71163,0.0999999999999994) ;
#26504=CIRCLE('',#71167,0.0999999999999994) ;
#26505=CIRCLE('',#71169,0.0999999999999994) ;
#26506=CIRCLE('',#71171,0.0999999999999999) ;
#26507=CIRCLE('',#71172,0.1) ;
#26508=CIRCLE('',#71175,0.1) ;
#26509=CIRCLE('',#71176,0.0999999999999998) ;
#26510=CIRCLE('',#71178,0.1) ;
#26511=CIRCLE('',#71180,0.0999999999999994) ;
#26512=CIRCLE('',#71182,0.0999999999999998) ;
#26513=CIRCLE('',#71184,0.1) ;
#26514=CIRCLE('',#71186,0.0999999999999994) ;
#26515=CIRCLE('',#71188,0.1) ;
#26516=CIRCLE('',#71191,0.0999999999999994) ;
#26517=CIRCLE('',#71192,0.0999999999999994) ;
#26518=CIRCLE('',#71194,0.0999999999999994) ;
#26519=CIRCLE('',#71196,0.0999999999999994) ;
#26520=CIRCLE('',#71198,0.0999999999999994) ;
#26521=CIRCLE('',#71200,0.1) ;
#26522=CIRCLE('',#71202,0.0999999999999994) ;
#26523=CIRCLE('',#71204,0.0999999999999994) ;
#26524=CIRCLE('',#71207,0.0999999999999994) ;
#26525=CIRCLE('',#71209,0.0999999999999999) ;
#26526=CIRCLE('',#71210,0.0999999999999999) ;
#26527=CIRCLE('',#71214,0.0999999999999994) ;
#26528=CIRCLE('',#71216,0.0999999999999994) ;
#26529=CIRCLE('',#71220,0.100000000000001) ;
#26530=CIRCLE('',#71222,0.0999999999999997) ;
#26531=CIRCLE('',#71224,0.0999999999999994) ;
#26532=CIRCLE('',#71227,1.4) ;
#26533=CIRCLE('',#71228,0.1) ;
#26534=CIRCLE('',#71229,1.5) ;
#26535=CIRCLE('',#71231,1.5) ;
#26536=CIRCLE('',#71232,0.1) ;
#26537=CIRCLE('',#71233,1.6) ;
#26538=CIRCLE('',#71235,0.0999999999999994) ;
#26539=CIRCLE('',#71236,0.0999999999999994) ;
#26540=CIRCLE('',#71237,0.0999999999999994) ;
#26541=CIRCLE('',#71239,0.0999999999999994) ;
#26542=CIRCLE('',#71240,0.1) ;
#26543=CIRCLE('',#71242,3.) ;
#26544=CIRCLE('',#71243,0.100000000000001) ;
#26545=CIRCLE('',#71244,3.00136060761679) ;
#26546=CIRCLE('',#71245,0.100000000000001) ;
#26547=CIRCLE('',#71248,3.) ;
#26548=CIRCLE('',#71249,3.) ;
#26549=CIRCLE('',#71250,3.) ;
#26550=CIRCLE('',#71259,3.33471270883832) ;
#26551=CIRCLE('',#71261,0.0999999999999994) ;
#26552=CIRCLE('',#71262,0.0999999999999994) ;
#26553=CIRCLE('',#71263,0.0999999999999994) ;
#26554=CIRCLE('',#71264,0.0999999999999994) ;
#26555=CIRCLE('',#71265,0.1) ;
#26556=CIRCLE('',#71266,0.1) ;
#26557=CIRCLE('',#71267,0.1) ;
#26558=CIRCLE('',#71268,0.1) ;
#26559=CIRCLE('',#71269,0.1) ;
#26560=CIRCLE('',#71270,0.1) ;
#26561=CIRCLE('',#71271,0.0999999999999994) ;
#26562=CIRCLE('',#71272,0.0999999999999994) ;
#26563=CIRCLE('',#71273,0.0999999999999994) ;
#26564=CIRCLE('',#71274,0.1) ;
#26565=CIRCLE('',#71275,0.1) ;
#26566=CIRCLE('',#71276,0.1) ;
#26567=CIRCLE('',#71278,0.0999999999999994) ;
#26568=CIRCLE('',#71279,0.1) ;
#26569=CIRCLE('',#71280,0.1) ;
#26570=CIRCLE('',#71281,0.1) ;
#26571=CIRCLE('',#71282,0.0999999999999994) ;
#26572=CIRCLE('',#71283,0.0999999999999994) ;
#26573=CIRCLE('',#71284,0.0999999999999994) ;
#26574=CIRCLE('',#71285,0.1) ;
#26575=CIRCLE('',#71286,0.1) ;
#26576=CIRCLE('',#71287,0.1) ;
#26577=CIRCLE('',#71288,0.1) ;
#26578=CIRCLE('',#71289,0.1) ;
#26579=CIRCLE('',#71290,0.1) ;
#26580=CIRCLE('',#71291,0.0999999999999994) ;
#26581=CIRCLE('',#71292,0.0999999999999994) ;
#26582=CIRCLE('',#71293,0.0999999999999994) ;
#26583=CIRCLE('',#71302,0.199999999999999) ;
#26584=CIRCLE('',#71303,0.199999999999999) ;
#26585=CIRCLE('',#71305,0.2) ;
#26586=CIRCLE('',#71306,0.2) ;
#26587=CIRCLE('',#71307,1.65) ;
#26588=CIRCLE('',#71308,0.2) ;
#26589=CIRCLE('',#71309,0.2) ;
#26590=CIRCLE('',#71310,1.65) ;
#26591=CIRCLE('',#71311,0.2) ;
#26592=CIRCLE('',#71312,0.2) ;
#26593=CIRCLE('',#71313,1.65) ;
#26594=CIRCLE('',#71314,0.2) ;
#26595=CIRCLE('',#71315,2.9) ;
#26596=CIRCLE('',#71316,0.2) ;
#26597=CIRCLE('',#71317,1.65) ;
#26598=CIRCLE('',#71319,0.199999999999999) ;
#26599=CIRCLE('',#71320,0.199999999999999) ;
#26600=CIRCLE('',#71322,0.2) ;
#26601=CIRCLE('',#71323,0.2) ;
#26602=CIRCLE('',#71325,0.2) ;
#26603=CIRCLE('',#71327,0.2) ;
#26604=CIRCLE('',#71335,0.1) ;
#26605=CIRCLE('',#71336,0.1) ;
#26606=CIRCLE('',#71337,0.0999999999999998) ;
#26607=CIRCLE('',#71338,0.0999999999999998) ;
#26608=CIRCLE('',#71340,0.2) ;
#26609=CIRCLE('',#71341,1.85) ;
#26610=CIRCLE('',#71342,2.9) ;
#26611=CIRCLE('',#71346,1.75) ;
#26612=CIRCLE('',#71347,1.75) ;
#26613=CIRCLE('',#71349,1.75) ;
#26614=CIRCLE('',#71350,1.75) ;
#26615=CIRCLE('',#71354,1.85) ;
#26616=CIRCLE('',#71355,0.2) ;
#26617=CIRCLE('',#71356,2.9) ;
#26618=CIRCLE('',#71358,1.85) ;
#26619=CIRCLE('',#71361,1.75) ;
#26620=CIRCLE('',#71362,1.75) ;
#26621=CIRCLE('',#71365,1.75) ;
#26622=CIRCLE('',#71366,1.75) ;
#26623=CIRCLE('',#71370,1.85) ;
#26624=CIRCLE('',#71385,1.1) ;
#26625=CIRCLE('',#71386,1.9) ;
#26626=CIRCLE('',#71388,1.9) ;
#26627=CIRCLE('',#71389,1.1) ;
#26628=CIRCLE('',#71391,2.) ;
#26629=CIRCLE('',#71392,2.) ;
#26630=CIRCLE('',#71399,1.) ;
#26631=CIRCLE('',#71400,1.) ;
#26632=CIRCLE('',#71406,609.695407994444) ;
#26633=CIRCLE('',#71408,3.23607331645511) ;
#26634=CIRCLE('',#71409,576.383429460242) ;
#26635=CIRCLE('',#71410,576.383428783031) ;
#26636=CIRCLE('',#71412,609.695409343247) ;
#26637=CIRCLE('',#71414,0.1) ;
#26638=CIRCLE('',#71416,0.0999999999999995) ;
#26639=CIRCLE('',#71417,0.0999999999999994) ;
#26640=CIRCLE('',#71419,0.1) ;
#26641=CIRCLE('',#71421,0.1) ;
#26642=CIRCLE('',#71423,0.0999999999999999) ;
#26643=CIRCLE('',#71425,0.0999999999999995) ;
#26644=CIRCLE('',#71427,0.0999999999999994) ;
#26645=CIRCLE('',#71428,0.0999999999999994) ;
#26646=CIRCLE('',#71430,0.1) ;
#26647=CIRCLE('',#71432,0.1) ;
#26648=CIRCLE('',#71433,0.0999999999999994) ;
#26649=CIRCLE('',#71435,0.1) ;
#26650=CIRCLE('',#71437,0.0999999999999999) ;
#26651=CIRCLE('',#71439,0.1) ;
#26652=CIRCLE('',#71441,0.0999999999999994) ;
#26653=CIRCLE('',#71443,0.1) ;
#26654=CIRCLE('',#71445,0.0999999999999995) ;
#26655=CIRCLE('',#71447,0.0999999999999995) ;
#26656=CIRCLE('',#71449,0.0999999999999994) ;
#26657=CIRCLE('',#71451,0.0999999999999994) ;
#26658=CIRCLE('',#71453,0.0999999999999999) ;
#26659=CIRCLE('',#71455,0.1) ;
#26660=CIRCLE('',#71456,0.0999999999999994) ;
#26661=CIRCLE('',#71458,0.0999999999999999) ;
#26662=CIRCLE('',#71460,0.0999999999999994) ;
#26663=CIRCLE('',#71462,0.0999999999999994) ;
#26664=CIRCLE('',#71464,0.0999999999999994) ;
#26665=CIRCLE('',#71466,0.0999999999999994) ;
#26666=CIRCLE('',#71468,0.1) ;
#26667=CIRCLE('',#71470,0.1) ;
#26668=CIRCLE('',#71472,0.0999999999999994) ;
#26669=CIRCLE('',#71474,0.0999999999999994) ;
#26670=CIRCLE('',#71476,0.1) ;
#26671=CIRCLE('',#71478,0.0999999999999994) ;
#26672=CIRCLE('',#71480,0.0999999999999994) ;
#26673=CIRCLE('',#71483,0.1) ;
#26674=CIRCLE('',#71484,0.0999999999999994) ;
#26675=CIRCLE('',#71485,0.1) ;
#26676=CIRCLE('',#71491,0.1) ;
#26677=CIRCLE('',#71499,0.0999999999999994) ;
#26678=CIRCLE('',#71500,0.0999999999999994) ;
#26679=CIRCLE('',#71502,0.0999999999999994) ;
#26680=CIRCLE('',#71504,0.0999999999999994) ;
#26681=CIRCLE('',#71505,0.1) ;
#26682=CIRCLE('',#71508,0.0999999999999994) ;
#26683=CIRCLE('',#71511,0.0999999999999994) ;
#26684=CIRCLE('',#71513,0.0999999999999994) ;
#26685=CIRCLE('',#71516,0.0999999999999994) ;
#26686=CIRCLE('',#71518,0.1) ;
#26687=CIRCLE('',#71520,0.1) ;
#26688=CIRCLE('',#71522,0.1) ;
#26689=CIRCLE('',#71524,0.0999999999999994) ;
#26690=CIRCLE('',#71525,0.1) ;
#26691=CIRCLE('',#71527,0.0999999999999994) ;
#26692=CIRCLE('',#71529,0.1) ;
#26693=CIRCLE('',#71531,0.0999999999999994) ;
#26694=CIRCLE('',#71532,0.1) ;
#26695=CIRCLE('',#71534,0.1) ;
#26696=CIRCLE('',#71536,0.1) ;
#26697=CIRCLE('',#71538,0.1) ;
#26698=CIRCLE('',#71540,0.0999999999999994) ;
#26699=CIRCLE('',#71542,0.0999999999999994) ;
#26700=CIRCLE('',#71544,0.0999999999999994) ;
#26701=CIRCLE('',#71546,0.0999999999999994) ;
#26702=CIRCLE('',#71547,0.0999999999999994) ;
#26703=CIRCLE('',#71549,0.1) ;
#26704=CIRCLE('',#71554,0.0999999999999994) ;
#26705=CIRCLE('',#71557,0.0999999999999998) ;
#26706=CIRCLE('',#71559,0.0999999999999995) ;
#26707=CIRCLE('',#71560,0.0999999999999994) ;
#26708=CIRCLE('',#71562,0.1) ;
#26709=CIRCLE('',#71564,0.0999999999999998) ;
#26710=CIRCLE('',#71566,0.0999999999999999) ;
#26711=CIRCLE('',#71568,0.1) ;
#26712=CIRCLE('',#71570,0.1) ;
#26713=CIRCLE('',#71571,0.1) ;
#26714=CIRCLE('',#71573,0.0999999999999995) ;
#26715=CIRCLE('',#71575,0.0999999999999994) ;
#26716=CIRCLE('',#71576,0.0999999999999994) ;
#26717=CIRCLE('',#71578,0.100000000000001) ;
#26718=CIRCLE('',#71580,0.0999999999999995) ;
#26719=CIRCLE('',#71582,0.0999999999999998) ;
#26720=CIRCLE('',#71584,0.0999999999999994) ;
#26721=CIRCLE('',#71586,0.100000000000001) ;
#26722=CIRCLE('',#71588,0.1) ;
#26723=CIRCLE('',#71589,0.1) ;
#26724=CIRCLE('',#71591,0.1) ;
#26725=CIRCLE('',#71593,0.1) ;
#26726=CIRCLE('',#71595,0.0999999999999994) ;
#26727=CIRCLE('',#71598,0.100000000000001) ;
#26728=CIRCLE('',#71600,0.0999999999999994) ;
#26729=CIRCLE('',#71601,0.0999999999999993) ;
#26730=CIRCLE('',#71604,0.1) ;
#26731=CIRCLE('',#71606,0.0999999999999994) ;
#26732=CIRCLE('',#71607,0.0999999999999994) ;
#26733=CIRCLE('',#71609,0.0999999999999995) ;
#26734=CIRCLE('',#71611,0.0999999999999998) ;
#26735=CIRCLE('',#71613,0.1) ;
#26736=CIRCLE('',#71614,0.1) ;
#26737=CIRCLE('',#71616,0.1) ;
#26738=CIRCLE('',#71618,0.0999999999999994) ;
#26739=CIRCLE('',#71620,0.0999999999999995) ;
#26740=CIRCLE('',#71622,0.1) ;
#26741=CIRCLE('',#71624,0.0999999999999998) ;
#26742=CIRCLE('',#71626,0.0999999999999995) ;
#26743=CIRCLE('',#71628,0.0999999999999994) ;
#26744=CIRCLE('',#71631,0.0999999999999994) ;
#26745=CIRCLE('',#71633,0.0999999999999994) ;
#26746=CIRCLE('',#71635,0.1) ;
#26747=CIRCLE('',#71637,0.1) ;
#26748=CIRCLE('',#71638,0.0999999999999995) ;
#26749=CIRCLE('',#71640,0.0999999999999994) ;
#26750=CIRCLE('',#71642,0.0999999999999994) ;
#26751=CIRCLE('',#71644,0.1) ;
#26752=CIRCLE('',#71645,0.0999999999999998) ;
#26753=CIRCLE('',#71647,0.0999999999999994) ;
#26754=CIRCLE('',#71649,0.1) ;
#26755=CIRCLE('',#71650,0.1) ;
#26756=CIRCLE('',#71652,0.0999999999999994) ;
#26757=CIRCLE('',#71654,0.0999999999999998) ;
#26758=CIRCLE('',#71656,0.1) ;
#26759=CIRCLE('',#71657,0.1) ;
#26760=CIRCLE('',#71659,0.0999999999999998) ;
#26761=CIRCLE('',#71661,0.0999999999999994) ;
#26762=CIRCLE('',#71663,0.1) ;
#26763=CIRCLE('',#71665,0.0999999999999998) ;
#26764=CIRCLE('',#71667,0.099999999999999) ;
#26765=CIRCLE('',#71669,0.1) ;
#26766=CIRCLE('',#71671,0.0999999999999994) ;
#26767=CIRCLE('',#71672,0.1) ;
#26768=CIRCLE('',#71675,0.0999999999999998) ;
#26769=CIRCLE('',#71677,0.1) ;
#26770=CIRCLE('',#71679,0.1) ;
#26771=CIRCLE('',#71680,0.0999999999999995) ;
#26772=CIRCLE('',#71682,0.1) ;
#26773=CIRCLE('',#71683,0.0999999999999998) ;
#26774=CIRCLE('',#71685,0.0999999999999994) ;
#26775=CIRCLE('',#71686,0.0999999999999994) ;
#26776=CIRCLE('',#71688,0.0999999999999998) ;
#26777=CIRCLE('',#71690,0.0999999999999998) ;
#26778=CIRCLE('',#71692,0.1) ;
#26779=CIRCLE('',#71694,0.0999999999999994) ;
#26780=CIRCLE('',#71696,0.0999999999999994) ;
#26781=CIRCLE('',#71698,0.1) ;
#26782=CIRCLE('',#71699,0.0999999999999995) ;
#26783=CIRCLE('',#71701,0.1) ;
#26784=CIRCLE('',#71702,0.0999999999999995) ;
#26785=CIRCLE('',#71704,0.0999999999999998) ;
#26786=CIRCLE('',#71706,0.0999999999999994) ;
#26787=CIRCLE('',#71708,0.0999999999999994) ;
#26788=CIRCLE('',#71711,0.0999999999999994) ;
#26789=CIRCLE('',#71713,0.0999999999999995) ;
#26790=CIRCLE('',#71715,0.0999999999999994) ;
#26791=CIRCLE('',#71717,0.1) ;
#26792=CIRCLE('',#71719,0.0999999999999994) ;
#26793=CIRCLE('',#71721,0.0999999999999998) ;
#26794=CIRCLE('',#71725,0.0999999999999995) ;
#26795=CIRCLE('',#71727,0.1) ;
#26796=CIRCLE('',#71729,0.0999999999999994) ;
#26797=CIRCLE('',#71731,0.0999999999999994) ;
#26798=CIRCLE('',#71733,0.0999999999999994) ;
#26799=CIRCLE('',#71735,0.100000000000001) ;
#26800=CIRCLE('',#71739,0.1) ;
#26801=CIRCLE('',#71740,0.1) ;
#26802=CIRCLE('',#71746,0.0999999999999994) ;
#26803=CIRCLE('',#71748,0.1) ;
#26804=CIRCLE('',#71749,0.1) ;
#26805=CIRCLE('',#71751,0.0999999999999994) ;
#26806=CIRCLE('',#71752,0.1) ;
#26807=CIRCLE('',#71754,0.0999999999999994) ;
#26808=CIRCLE('',#71756,0.0999999999999994) ;
#26809=CIRCLE('',#71758,0.0999999999999994) ;
#26810=CIRCLE('',#71759,0.0999999999999994) ;
#26811=CIRCLE('',#71761,0.0999999999999994) ;
#26812=CIRCLE('',#71763,0.0999999999999994) ;
#26813=CIRCLE('',#71765,0.1) ;
#26814=CIRCLE('',#71766,0.0999999999999994) ;
#26815=CIRCLE('',#71768,0.0999999999999994) ;
#26816=CIRCLE('',#71771,0.0999999999999994) ;
#26817=CIRCLE('',#71773,0.0999999999999994) ;
#26818=CIRCLE('',#71777,0.0999999999999994) ;
#26819=CIRCLE('',#71779,0.0999999999999994) ;
#26820=CIRCLE('',#71781,0.0999999999999999) ;
#26821=CIRCLE('',#71782,0.1) ;
#26822=CIRCLE('',#71785,0.1) ;
#26823=CIRCLE('',#71786,0.0999999999999998) ;
#26824=CIRCLE('',#71788,0.1) ;
#26825=CIRCLE('',#71790,0.0999999999999994) ;
#26826=CIRCLE('',#71792,0.0999999999999998) ;
#26827=CIRCLE('',#71794,0.1) ;
#26828=CIRCLE('',#71796,0.0999999999999994) ;
#26829=CIRCLE('',#71798,0.1) ;
#26830=CIRCLE('',#71801,0.0999999999999994) ;
#26831=CIRCLE('',#71802,0.0999999999999994) ;
#26832=CIRCLE('',#71804,0.0999999999999994) ;
#26833=CIRCLE('',#71806,0.0999999999999994) ;
#26834=CIRCLE('',#71808,0.0999999999999994) ;
#26835=CIRCLE('',#71810,0.1) ;
#26836=CIRCLE('',#71812,0.0999999999999994) ;
#26837=CIRCLE('',#71814,0.0999999999999994) ;
#26838=CIRCLE('',#71817,0.0999999999999994) ;
#26839=CIRCLE('',#71819,0.0999999999999999) ;
#26840=CIRCLE('',#71820,0.0999999999999999) ;
#26841=CIRCLE('',#71824,0.0999999999999994) ;
#26842=CIRCLE('',#71826,0.0999999999999994) ;
#30062=VERTEX_POINT('',#101197) ;
#30063=VERTEX_POINT('',#101198) ;
#30064=VERTEX_POINT('',#101209) ;
#30065=VERTEX_POINT('',#101211) ;
#30066=VERTEX_POINT('',#101213) ;
#30067=VERTEX_POINT('',#101234) ;
#30068=VERTEX_POINT('',#101235) ;
#30069=VERTEX_POINT('',#101252) ;
#30070=VERTEX_POINT('',#101254) ;
#30071=VERTEX_POINT('',#101256) ;
#30072=VERTEX_POINT('',#101260) ;
#30073=VERTEX_POINT('',#101262) ;
#30074=VERTEX_POINT('',#101266) ;
#30075=VERTEX_POINT('',#101268) ;
#30076=VERTEX_POINT('',#101272) ;
#30077=VERTEX_POINT('',#101273) ;
#30078=VERTEX_POINT('',#101275) ;
#30079=VERTEX_POINT('',#101277) ;
#30080=VERTEX_POINT('',#101279) ;
#30081=VERTEX_POINT('',#101283) ;
#30082=VERTEX_POINT('',#101284) ;
#30083=VERTEX_POINT('',#101286) ;
#30084=VERTEX_POINT('',#101288) ;
#30085=VERTEX_POINT('',#101292) ;
#30086=VERTEX_POINT('',#101293) ;
#30087=VERTEX_POINT('',#101295) ;
#30088=VERTEX_POINT('',#101297) ;
#30089=VERTEX_POINT('',#101303) ;
#30090=VERTEX_POINT('',#101306) ;
#30091=VERTEX_POINT('',#101313) ;
#30092=VERTEX_POINT('',#101321) ;
#30093=VERTEX_POINT('',#101325) ;
#30094=VERTEX_POINT('',#101326) ;
#30095=VERTEX_POINT('',#101328) ;
#30096=VERTEX_POINT('',#101330) ;
#30097=VERTEX_POINT('',#101337) ;
#30098=VERTEX_POINT('',#101339) ;
#30099=VERTEX_POINT('',#101343) ;
#30100=VERTEX_POINT('',#101344) ;
#30101=VERTEX_POINT('',#101346) ;
#30102=VERTEX_POINT('',#101348) ;
#30103=VERTEX_POINT('',#101377) ;
#30104=VERTEX_POINT('',#101388) ;
#30105=VERTEX_POINT('',#101392) ;
#30106=VERTEX_POINT('',#101393) ;
#30107=VERTEX_POINT('',#101395) ;
#30108=VERTEX_POINT('',#101397) ;
#30109=VERTEX_POINT('',#101401) ;
#30110=VERTEX_POINT('',#101402) ;
#30111=VERTEX_POINT('',#101404) ;
#30112=VERTEX_POINT('',#101412) ;
#30113=VERTEX_POINT('',#101425) ;
#30114=VERTEX_POINT('',#101427) ;
#30115=VERTEX_POINT('',#101431) ;
#30116=VERTEX_POINT('',#101432) ;
#30117=VERTEX_POINT('',#101434) ;
#30118=VERTEX_POINT('',#101436) ;
#30119=VERTEX_POINT('',#101440) ;
#30120=VERTEX_POINT('',#101441) ;
#30121=VERTEX_POINT('',#101443) ;
#30122=VERTEX_POINT('',#101445) ;
#30123=VERTEX_POINT('',#101449) ;
#30124=VERTEX_POINT('',#101450) ;
#30125=VERTEX_POINT('',#101452) ;
#30126=VERTEX_POINT('',#101454) ;
#30127=VERTEX_POINT('',#101456) ;
#30128=VERTEX_POINT('',#101458) ;
#30129=VERTEX_POINT('',#101462) ;
#30130=VERTEX_POINT('',#101463) ;
#30131=VERTEX_POINT('',#101468) ;
#30132=VERTEX_POINT('',#101470) ;
#30133=VERTEX_POINT('',#101472) ;
#30134=VERTEX_POINT('',#101474) ;
#30135=VERTEX_POINT('',#101476) ;
#30136=VERTEX_POINT('',#101478) ;
#30137=VERTEX_POINT('',#101480) ;
#30138=VERTEX_POINT('',#101482) ;
#30139=VERTEX_POINT('',#101484) ;
#30140=VERTEX_POINT('',#101486) ;
#30141=VERTEX_POINT('',#101488) ;
#30142=VERTEX_POINT('',#101490) ;
#30143=VERTEX_POINT('',#101493) ;
#30144=VERTEX_POINT('',#101495) ;
#30145=VERTEX_POINT('',#101498) ;
#30146=VERTEX_POINT('',#101500) ;
#30147=VERTEX_POINT('',#101502) ;
#30148=VERTEX_POINT('',#101504) ;
#30149=VERTEX_POINT('',#101506) ;
#30150=VERTEX_POINT('',#101508) ;
#30151=VERTEX_POINT('',#101510) ;
#30152=VERTEX_POINT('',#101514) ;
#30153=VERTEX_POINT('',#101515) ;
#30154=VERTEX_POINT('',#101517) ;
#30155=VERTEX_POINT('',#101519) ;
#30156=VERTEX_POINT('',#101521) ;
#30157=VERTEX_POINT('',#101523) ;
#30158=VERTEX_POINT('',#101525) ;
#30159=VERTEX_POINT('',#101527) ;
#30160=VERTEX_POINT('',#101529) ;
#30161=VERTEX_POINT('',#101531) ;
#30162=VERTEX_POINT('',#101533) ;
#30163=VERTEX_POINT('',#101536) ;
#30164=VERTEX_POINT('',#101538) ;
#30165=VERTEX_POINT('',#101541) ;
#30166=VERTEX_POINT('',#101543) ;
#30167=VERTEX_POINT('',#101545) ;
#30168=VERTEX_POINT('',#101547) ;
#30169=VERTEX_POINT('',#101549) ;
#30170=VERTEX_POINT('',#101551) ;
#30171=VERTEX_POINT('',#101553) ;
#30172=VERTEX_POINT('',#101555) ;
#30173=VERTEX_POINT('',#101557) ;
#30174=VERTEX_POINT('',#101559) ;
#30175=VERTEX_POINT('',#101561) ;
#30176=VERTEX_POINT('',#101563) ;
#30177=VERTEX_POINT('',#101565) ;
#30178=VERTEX_POINT('',#101567) ;
#30179=VERTEX_POINT('',#101569) ;
#30180=VERTEX_POINT('',#101571) ;
#30181=VERTEX_POINT('',#101581) ;
#30182=VERTEX_POINT('',#101582) ;
#30183=VERTEX_POINT('',#101625) ;
#30184=VERTEX_POINT('',#101627) ;
#30185=VERTEX_POINT('',#101670) ;
#30186=VERTEX_POINT('',#101671) ;
#30187=VERTEX_POINT('',#101679) ;
#30188=VERTEX_POINT('',#101682) ;
#30189=VERTEX_POINT('',#101686) ;
#30190=VERTEX_POINT('',#101687) ;
#30191=VERTEX_POINT('',#101692) ;
#30192=VERTEX_POINT('',#101707) ;
#30193=VERTEX_POINT('',#101712) ;
#30194=VERTEX_POINT('',#101714) ;
#30195=VERTEX_POINT('',#101749) ;
#30196=VERTEX_POINT('',#101751) ;
#30197=VERTEX_POINT('',#101805) ;
#30198=VERTEX_POINT('',#101807) ;
#30199=VERTEX_POINT('',#101809) ;
#30200=VERTEX_POINT('',#101811) ;
#30201=VERTEX_POINT('',#101813) ;
#30202=VERTEX_POINT('',#101815) ;
#30203=VERTEX_POINT('',#101819) ;
#30204=VERTEX_POINT('',#101820) ;
#30205=VERTEX_POINT('',#101823) ;
#30206=VERTEX_POINT('',#101825) ;
#30207=VERTEX_POINT('',#101827) ;
#30208=VERTEX_POINT('',#101829) ;
#30209=VERTEX_POINT('',#101831) ;
#30210=VERTEX_POINT('',#101833) ;
#30211=VERTEX_POINT('',#101835) ;
#30212=VERTEX_POINT('',#101837) ;
#30213=VERTEX_POINT('',#101839) ;
#30214=VERTEX_POINT('',#101841) ;
#30215=VERTEX_POINT('',#101844) ;
#30216=VERTEX_POINT('',#101846) ;
#30217=VERTEX_POINT('',#101848) ;
#30218=VERTEX_POINT('',#101850) ;
#30219=VERTEX_POINT('',#101852) ;
#30220=VERTEX_POINT('',#101854) ;
#30221=VERTEX_POINT('',#101856) ;
#30222=VERTEX_POINT('',#101858) ;
#30223=VERTEX_POINT('',#101862) ;
#30224=VERTEX_POINT('',#101863) ;
#30225=VERTEX_POINT('',#101865) ;
#30226=VERTEX_POINT('',#101869) ;
#30227=VERTEX_POINT('',#101871) ;
#30228=VERTEX_POINT('',#101873) ;
#30229=VERTEX_POINT('',#101877) ;
#30230=VERTEX_POINT('',#101878) ;
#30231=VERTEX_POINT('',#101882) ;
#30232=VERTEX_POINT('',#101884) ;
#30233=VERTEX_POINT('',#101888) ;
#30234=VERTEX_POINT('',#101889) ;
#30235=VERTEX_POINT('',#101891) ;
#30236=VERTEX_POINT('',#101895) ;
#30237=VERTEX_POINT('',#101896) ;
#30238=VERTEX_POINT('',#101898) ;
#30239=VERTEX_POINT('',#101902) ;
#30240=VERTEX_POINT('',#101903) ;
#30241=VERTEX_POINT('',#101905) ;
#30242=VERTEX_POINT('',#101907) ;
#30243=VERTEX_POINT('',#101909) ;
#30244=VERTEX_POINT('',#101911) ;
#30245=VERTEX_POINT('',#101913) ;
#30246=VERTEX_POINT('',#101915) ;
#30247=VERTEX_POINT('',#101919) ;
#30248=VERTEX_POINT('',#101920) ;
#30249=VERTEX_POINT('',#101922) ;
#30250=VERTEX_POINT('',#101924) ;
#30251=VERTEX_POINT('',#101928) ;
#30252=VERTEX_POINT('',#101929) ;
#30253=VERTEX_POINT('',#101931) ;
#30254=VERTEX_POINT('',#101933) ;
#30255=VERTEX_POINT('',#101937) ;
#30256=VERTEX_POINT('',#101938) ;
#30257=VERTEX_POINT('',#101940) ;
#30258=VERTEX_POINT('',#101942) ;
#30259=VERTEX_POINT('',#101946) ;
#30260=VERTEX_POINT('',#101947) ;
#30261=VERTEX_POINT('',#101956) ;
#30262=VERTEX_POINT('',#101958) ;
#30263=VERTEX_POINT('',#101960) ;
#30264=VERTEX_POINT('',#101962) ;
#30265=VERTEX_POINT('',#101973) ;
#30266=VERTEX_POINT('',#101974) ;
#30267=VERTEX_POINT('',#101976) ;
#30268=VERTEX_POINT('',#101978) ;
#30269=VERTEX_POINT('',#101980) ;
#30270=VERTEX_POINT('',#101982) ;
#30271=VERTEX_POINT('',#101984) ;
#30272=VERTEX_POINT('',#101986) ;
#30273=VERTEX_POINT('',#101990) ;
#30274=VERTEX_POINT('',#101991) ;
#30275=VERTEX_POINT('',#101993) ;
#30276=VERTEX_POINT('',#101995) ;
#30277=VERTEX_POINT('',#101997) ;
#30278=VERTEX_POINT('',#101999) ;
#30279=VERTEX_POINT('',#102001) ;
#30280=VERTEX_POINT('',#102003) ;
#30281=VERTEX_POINT('',#102007) ;
#30282=VERTEX_POINT('',#102008) ;
#30283=VERTEX_POINT('',#102011) ;
#30284=VERTEX_POINT('',#102013) ;
#30285=VERTEX_POINT('',#102015) ;
#30286=VERTEX_POINT('',#102019) ;
#30287=VERTEX_POINT('',#102021) ;
#30288=VERTEX_POINT('',#102025) ;
#30289=VERTEX_POINT('',#102026) ;
#30290=VERTEX_POINT('',#102031) ;
#30291=VERTEX_POINT('',#102032) ;
#30292=VERTEX_POINT('',#102034) ;
#30293=VERTEX_POINT('',#102036) ;
#30294=VERTEX_POINT('',#102040) ;
#30295=VERTEX_POINT('',#102041) ;
#30296=VERTEX_POINT('',#102043) ;
#30297=VERTEX_POINT('',#102045) ;
#30298=VERTEX_POINT('',#102049) ;
#30299=VERTEX_POINT('',#102051) ;
#30300=VERTEX_POINT('',#102055) ;
#30301=VERTEX_POINT('',#102056) ;
#30302=VERTEX_POINT('',#102061) ;
#30303=VERTEX_POINT('',#102062) ;
#30304=VERTEX_POINT('',#102065) ;
#30305=VERTEX_POINT('',#102067) ;
#30306=VERTEX_POINT('',#102069) ;
#30307=VERTEX_POINT('',#102073) ;
#30308=VERTEX_POINT('',#102074) ;
#30309=VERTEX_POINT('',#102077) ;
#30310=VERTEX_POINT('',#102081) ;
#30311=VERTEX_POINT('',#102082) ;
#30312=VERTEX_POINT('',#102087) ;
#30313=VERTEX_POINT('',#102088) ;
#30314=VERTEX_POINT('',#102090) ;
#30315=VERTEX_POINT('',#102092) ;
#30316=VERTEX_POINT('',#102096) ;
#30317=VERTEX_POINT('',#102097) ;
#30318=VERTEX_POINT('',#102099) ;
#30319=VERTEX_POINT('',#102101) ;
#30320=VERTEX_POINT('',#102105) ;
#30321=VERTEX_POINT('',#102106) ;
#30322=VERTEX_POINT('',#102108) ;
#30323=VERTEX_POINT('',#102110) ;
#30324=VERTEX_POINT('',#102114) ;
#30325=VERTEX_POINT('',#102116) ;
#30326=VERTEX_POINT('',#102120) ;
#30327=VERTEX_POINT('',#102121) ;
#30328=VERTEX_POINT('',#102123) ;
#30329=VERTEX_POINT('',#102125) ;
#30330=VERTEX_POINT('',#102129) ;
#30331=VERTEX_POINT('',#102130) ;
#30332=VERTEX_POINT('',#102133) ;
#30333=VERTEX_POINT('',#102137) ;
#30334=VERTEX_POINT('',#102138) ;
#30335=VERTEX_POINT('',#102140) ;
#30336=VERTEX_POINT('',#102142) ;
#30337=VERTEX_POINT('',#102146) ;
#30338=VERTEX_POINT('',#102147) ;
#30339=VERTEX_POINT('',#102150) ;
#30340=VERTEX_POINT('',#102152) ;
#30341=VERTEX_POINT('',#102154) ;
#30342=VERTEX_POINT('',#102156) ;
#30343=VERTEX_POINT('',#102160) ;
#30344=VERTEX_POINT('',#102161) ;
#30345=VERTEX_POINT('',#102164) ;
#30346=VERTEX_POINT('',#102168) ;
#30347=VERTEX_POINT('',#102169) ;
#30348=VERTEX_POINT('',#102171) ;
#30349=VERTEX_POINT('',#102173) ;
#30350=VERTEX_POINT('',#102177) ;
#30351=VERTEX_POINT('',#102178) ;
#30352=VERTEX_POINT('',#102180) ;
#30353=VERTEX_POINT('',#102182) ;
#30354=VERTEX_POINT('',#102186) ;
#30355=VERTEX_POINT('',#102187) ;
#30356=VERTEX_POINT('',#102189) ;
#30357=VERTEX_POINT('',#102191) ;
#30358=VERTEX_POINT('',#102195) ;
#30359=VERTEX_POINT('',#102197) ;
#30360=VERTEX_POINT('',#102201) ;
#30361=VERTEX_POINT('',#102203) ;
#30362=VERTEX_POINT('',#102207) ;
#30363=VERTEX_POINT('',#102209) ;
#30364=VERTEX_POINT('',#102213) ;
#30365=VERTEX_POINT('',#102215) ;
#30366=VERTEX_POINT('',#102219) ;
#30367=VERTEX_POINT('',#102220) ;
#30368=VERTEX_POINT('',#102222) ;
#30369=VERTEX_POINT('',#102224) ;
#30370=VERTEX_POINT('',#102226) ;
#30371=VERTEX_POINT('',#102228) ;
#30372=VERTEX_POINT('',#102232) ;
#30373=VERTEX_POINT('',#102233) ;
#30374=VERTEX_POINT('',#102235) ;
#30375=VERTEX_POINT('',#102237) ;
#30376=VERTEX_POINT('',#102239) ;
#30377=VERTEX_POINT('',#102241) ;
#30378=VERTEX_POINT('',#102245) ;
#30379=VERTEX_POINT('',#102246) ;
#30380=VERTEX_POINT('',#102251) ;
#30381=VERTEX_POINT('',#102253) ;
#30382=VERTEX_POINT('',#102257) ;
#30383=VERTEX_POINT('',#102258) ;
#30384=VERTEX_POINT('',#102260) ;
#30385=VERTEX_POINT('',#102262) ;
#30386=VERTEX_POINT('',#102266) ;
#30387=VERTEX_POINT('',#102267) ;
#30388=VERTEX_POINT('',#102269) ;
#30389=VERTEX_POINT('',#102271) ;
#30390=VERTEX_POINT('',#102275) ;
#30391=VERTEX_POINT('',#102276) ;
#30392=VERTEX_POINT('',#102278) ;
#30393=VERTEX_POINT('',#102280) ;
#30394=VERTEX_POINT('',#102284) ;
#30395=VERTEX_POINT('',#102285) ;
#30396=VERTEX_POINT('',#102287) ;
#30397=VERTEX_POINT('',#102289) ;
#30398=VERTEX_POINT('',#102296) ;
#30399=VERTEX_POINT('',#102297) ;
#30400=VERTEX_POINT('',#102299) ;
#30401=VERTEX_POINT('',#102301) ;
#30402=VERTEX_POINT('',#102305) ;
#30403=VERTEX_POINT('',#102306) ;
#30404=VERTEX_POINT('',#102308) ;
#30405=VERTEX_POINT('',#102310) ;
#30406=VERTEX_POINT('',#102314) ;
#30407=VERTEX_POINT('',#102315) ;
#30408=VERTEX_POINT('',#102317) ;
#30409=VERTEX_POINT('',#102319) ;
#30410=VERTEX_POINT('',#102323) ;
#30411=VERTEX_POINT('',#102324) ;
#30412=VERTEX_POINT('',#102326) ;
#30413=VERTEX_POINT('',#102328) ;
#30414=VERTEX_POINT('',#102332) ;
#30415=VERTEX_POINT('',#102334) ;
#30416=VERTEX_POINT('',#102338) ;
#30417=VERTEX_POINT('',#102339) ;
#30418=VERTEX_POINT('',#102344) ;
#30419=VERTEX_POINT('',#102346) ;
#30420=VERTEX_POINT('',#102423) ;
#30421=VERTEX_POINT('',#102440) ;
#30422=VERTEX_POINT('',#102459) ;
#30423=VERTEX_POINT('',#102475) ;
#30424=VERTEX_POINT('',#102492) ;
#30425=VERTEX_POINT('',#102508) ;
#30426=VERTEX_POINT('',#102528) ;
#30427=VERTEX_POINT('',#102532) ;
#30428=VERTEX_POINT('',#102536) ;
#30429=VERTEX_POINT('',#102554) ;
#30430=VERTEX_POINT('',#102572) ;
#30431=VERTEX_POINT('',#102581) ;
#30432=VERTEX_POINT('',#102587) ;
#30433=VERTEX_POINT('',#102595) ;
#30434=VERTEX_POINT('',#102601) ;
#30435=VERTEX_POINT('',#102614) ;
#30436=VERTEX_POINT('',#102720) ;
#30437=VERTEX_POINT('',#103147) ;
#30438=VERTEX_POINT('',#103227) ;
#30439=VERTEX_POINT('',#103238) ;
#30440=VERTEX_POINT('',#103464) ;
#30441=VERTEX_POINT('',#103481) ;
#30442=VERTEX_POINT('',#103709) ;
#30443=VERTEX_POINT('',#103710) ;
#30444=VERTEX_POINT('',#103721) ;
#30445=VERTEX_POINT('',#103723) ;
#30446=VERTEX_POINT('',#103725) ;
#30447=VERTEX_POINT('',#103746) ;
#30448=VERTEX_POINT('',#103747) ;
#30449=VERTEX_POINT('',#103764) ;
#30450=VERTEX_POINT('',#103766) ;
#30451=VERTEX_POINT('',#103768) ;
#30452=VERTEX_POINT('',#103772) ;
#30453=VERTEX_POINT('',#103774) ;
#30454=VERTEX_POINT('',#103778) ;
#30455=VERTEX_POINT('',#103780) ;
#30456=VERTEX_POINT('',#103784) ;
#30457=VERTEX_POINT('',#103785) ;
#30458=VERTEX_POINT('',#103787) ;
#30459=VERTEX_POINT('',#103789) ;
#30460=VERTEX_POINT('',#103791) ;
#30461=VERTEX_POINT('',#103795) ;
#30462=VERTEX_POINT('',#103796) ;
#30463=VERTEX_POINT('',#103798) ;
#30464=VERTEX_POINT('',#103800) ;
#30465=VERTEX_POINT('',#103804) ;
#30466=VERTEX_POINT('',#103805) ;
#30467=VERTEX_POINT('',#103807) ;
#30468=VERTEX_POINT('',#103809) ;
#30469=VERTEX_POINT('',#103815) ;
#30470=VERTEX_POINT('',#103818) ;
#30471=VERTEX_POINT('',#103825) ;
#30472=VERTEX_POINT('',#103833) ;
#30473=VERTEX_POINT('',#103837) ;
#30474=VERTEX_POINT('',#103838) ;
#30475=VERTEX_POINT('',#103840) ;
#30476=VERTEX_POINT('',#103842) ;
#30477=VERTEX_POINT('',#103849) ;
#30478=VERTEX_POINT('',#103851) ;
#30479=VERTEX_POINT('',#103855) ;
#30480=VERTEX_POINT('',#103856) ;
#30481=VERTEX_POINT('',#103858) ;
#30482=VERTEX_POINT('',#103860) ;
#30483=VERTEX_POINT('',#103889) ;
#30484=VERTEX_POINT('',#103900) ;
#30485=VERTEX_POINT('',#103904) ;
#30486=VERTEX_POINT('',#103905) ;
#30487=VERTEX_POINT('',#103907) ;
#30488=VERTEX_POINT('',#103909) ;
#30489=VERTEX_POINT('',#103913) ;
#30490=VERTEX_POINT('',#103914) ;
#30491=VERTEX_POINT('',#103916) ;
#30492=VERTEX_POINT('',#103924) ;
#30493=VERTEX_POINT('',#103937) ;
#30494=VERTEX_POINT('',#103939) ;
#30495=VERTEX_POINT('',#103943) ;
#30496=VERTEX_POINT('',#103944) ;
#30497=VERTEX_POINT('',#103946) ;
#30498=VERTEX_POINT('',#103948) ;
#30499=VERTEX_POINT('',#103952) ;
#30500=VERTEX_POINT('',#103953) ;
#30501=VERTEX_POINT('',#103955) ;
#30502=VERTEX_POINT('',#103957) ;
#30503=VERTEX_POINT('',#103961) ;
#30504=VERTEX_POINT('',#103962) ;
#30505=VERTEX_POINT('',#103964) ;
#30506=VERTEX_POINT('',#103966) ;
#30507=VERTEX_POINT('',#103968) ;
#30508=VERTEX_POINT('',#103970) ;
#30509=VERTEX_POINT('',#103974) ;
#30510=VERTEX_POINT('',#103975) ;
#30511=VERTEX_POINT('',#103980) ;
#30512=VERTEX_POINT('',#103982) ;
#30513=VERTEX_POINT('',#103984) ;
#30514=VERTEX_POINT('',#103986) ;
#30515=VERTEX_POINT('',#103988) ;
#30516=VERTEX_POINT('',#103990) ;
#30517=VERTEX_POINT('',#103992) ;
#30518=VERTEX_POINT('',#103994) ;
#30519=VERTEX_POINT('',#103996) ;
#30520=VERTEX_POINT('',#103998) ;
#30521=VERTEX_POINT('',#104000) ;
#30522=VERTEX_POINT('',#104002) ;
#30523=VERTEX_POINT('',#104005) ;
#30524=VERTEX_POINT('',#104007) ;
#30525=VERTEX_POINT('',#104010) ;
#30526=VERTEX_POINT('',#104012) ;
#30527=VERTEX_POINT('',#104014) ;
#30528=VERTEX_POINT('',#104016) ;
#30529=VERTEX_POINT('',#104018) ;
#30530=VERTEX_POINT('',#104020) ;
#30531=VERTEX_POINT('',#104022) ;
#30532=VERTEX_POINT('',#104026) ;
#30533=VERTEX_POINT('',#104027) ;
#30534=VERTEX_POINT('',#104029) ;
#30535=VERTEX_POINT('',#104031) ;
#30536=VERTEX_POINT('',#104033) ;
#30537=VERTEX_POINT('',#104035) ;
#30538=VERTEX_POINT('',#104037) ;
#30539=VERTEX_POINT('',#104039) ;
#30540=VERTEX_POINT('',#104041) ;
#30541=VERTEX_POINT('',#104043) ;
#30542=VERTEX_POINT('',#104045) ;
#30543=VERTEX_POINT('',#104048) ;
#30544=VERTEX_POINT('',#104050) ;
#30545=VERTEX_POINT('',#104053) ;
#30546=VERTEX_POINT('',#104055) ;
#30547=VERTEX_POINT('',#104057) ;
#30548=VERTEX_POINT('',#104059) ;
#30549=VERTEX_POINT('',#104061) ;
#30550=VERTEX_POINT('',#104063) ;
#30551=VERTEX_POINT('',#104065) ;
#30552=VERTEX_POINT('',#104067) ;
#30553=VERTEX_POINT('',#104069) ;
#30554=VERTEX_POINT('',#104071) ;
#30555=VERTEX_POINT('',#104073) ;
#30556=VERTEX_POINT('',#104075) ;
#30557=VERTEX_POINT('',#104077) ;
#30558=VERTEX_POINT('',#104079) ;
#30559=VERTEX_POINT('',#104081) ;
#30560=VERTEX_POINT('',#104083) ;
#30561=VERTEX_POINT('',#104093) ;
#30562=VERTEX_POINT('',#104094) ;
#30563=VERTEX_POINT('',#104137) ;
#30564=VERTEX_POINT('',#104139) ;
#30565=VERTEX_POINT('',#104182) ;
#30566=VERTEX_POINT('',#104183) ;
#30567=VERTEX_POINT('',#104191) ;
#30568=VERTEX_POINT('',#104194) ;
#30569=VERTEX_POINT('',#104198) ;
#30570=VERTEX_POINT('',#104199) ;
#30571=VERTEX_POINT('',#104204) ;
#30572=VERTEX_POINT('',#104219) ;
#30573=VERTEX_POINT('',#104224) ;
#30574=VERTEX_POINT('',#104226) ;
#30575=VERTEX_POINT('',#104261) ;
#30576=VERTEX_POINT('',#104263) ;
#30577=VERTEX_POINT('',#104317) ;
#30578=VERTEX_POINT('',#104319) ;
#30579=VERTEX_POINT('',#104321) ;
#30580=VERTEX_POINT('',#104323) ;
#30581=VERTEX_POINT('',#104325) ;
#30582=VERTEX_POINT('',#104327) ;
#30583=VERTEX_POINT('',#104331) ;
#30584=VERTEX_POINT('',#104332) ;
#30585=VERTEX_POINT('',#104335) ;
#30586=VERTEX_POINT('',#104337) ;
#30587=VERTEX_POINT('',#104339) ;
#30588=VERTEX_POINT('',#104341) ;
#30589=VERTEX_POINT('',#104343) ;
#30590=VERTEX_POINT('',#104345) ;
#30591=VERTEX_POINT('',#104347) ;
#30592=VERTEX_POINT('',#104349) ;
#30593=VERTEX_POINT('',#104351) ;
#30594=VERTEX_POINT('',#104353) ;
#30595=VERTEX_POINT('',#104356) ;
#30596=VERTEX_POINT('',#104358) ;
#30597=VERTEX_POINT('',#104360) ;
#30598=VERTEX_POINT('',#104362) ;
#30599=VERTEX_POINT('',#104364) ;
#30600=VERTEX_POINT('',#104366) ;
#30601=VERTEX_POINT('',#104368) ;
#30602=VERTEX_POINT('',#104370) ;
#30603=VERTEX_POINT('',#104374) ;
#30604=VERTEX_POINT('',#104375) ;
#30605=VERTEX_POINT('',#104377) ;
#30606=VERTEX_POINT('',#104381) ;
#30607=VERTEX_POINT('',#104383) ;
#30608=VERTEX_POINT('',#104385) ;
#30609=VERTEX_POINT('',#104389) ;
#30610=VERTEX_POINT('',#104390) ;
#30611=VERTEX_POINT('',#104394) ;
#30612=VERTEX_POINT('',#104396) ;
#30613=VERTEX_POINT('',#104400) ;
#30614=VERTEX_POINT('',#104401) ;
#30615=VERTEX_POINT('',#104403) ;
#30616=VERTEX_POINT('',#104407) ;
#30617=VERTEX_POINT('',#104408) ;
#30618=VERTEX_POINT('',#104410) ;
#30619=VERTEX_POINT('',#104414) ;
#30620=VERTEX_POINT('',#104415) ;
#30621=VERTEX_POINT('',#104417) ;
#30622=VERTEX_POINT('',#104419) ;
#30623=VERTEX_POINT('',#104421) ;
#30624=VERTEX_POINT('',#104423) ;
#30625=VERTEX_POINT('',#104425) ;
#30626=VERTEX_POINT('',#104427) ;
#30627=VERTEX_POINT('',#104431) ;
#30628=VERTEX_POINT('',#104432) ;
#30629=VERTEX_POINT('',#104434) ;
#30630=VERTEX_POINT('',#104436) ;
#30631=VERTEX_POINT('',#104440) ;
#30632=VERTEX_POINT('',#104441) ;
#30633=VERTEX_POINT('',#104443) ;
#30634=VERTEX_POINT('',#104445) ;
#30635=VERTEX_POINT('',#104449) ;
#30636=VERTEX_POINT('',#104450) ;
#30637=VERTEX_POINT('',#104452) ;
#30638=VERTEX_POINT('',#104454) ;
#30639=VERTEX_POINT('',#104458) ;
#30640=VERTEX_POINT('',#104459) ;
#30641=VERTEX_POINT('',#104468) ;
#30642=VERTEX_POINT('',#104470) ;
#30643=VERTEX_POINT('',#104472) ;
#30644=VERTEX_POINT('',#104474) ;
#30645=VERTEX_POINT('',#104485) ;
#30646=VERTEX_POINT('',#104486) ;
#30647=VERTEX_POINT('',#104488) ;
#30648=VERTEX_POINT('',#104490) ;
#30649=VERTEX_POINT('',#104492) ;
#30650=VERTEX_POINT('',#104494) ;
#30651=VERTEX_POINT('',#104496) ;
#30652=VERTEX_POINT('',#104498) ;
#30653=VERTEX_POINT('',#104502) ;
#30654=VERTEX_POINT('',#104503) ;
#30655=VERTEX_POINT('',#104505) ;
#30656=VERTEX_POINT('',#104507) ;
#30657=VERTEX_POINT('',#104509) ;
#30658=VERTEX_POINT('',#104511) ;
#30659=VERTEX_POINT('',#104513) ;
#30660=VERTEX_POINT('',#104515) ;
#30661=VERTEX_POINT('',#104519) ;
#30662=VERTEX_POINT('',#104520) ;
#30663=VERTEX_POINT('',#104523) ;
#30664=VERTEX_POINT('',#104525) ;
#30665=VERTEX_POINT('',#104527) ;
#30666=VERTEX_POINT('',#104531) ;
#30667=VERTEX_POINT('',#104533) ;
#30668=VERTEX_POINT('',#104537) ;
#30669=VERTEX_POINT('',#104538) ;
#30670=VERTEX_POINT('',#104543) ;
#30671=VERTEX_POINT('',#104544) ;
#30672=VERTEX_POINT('',#104546) ;
#30673=VERTEX_POINT('',#104548) ;
#30674=VERTEX_POINT('',#104552) ;
#30675=VERTEX_POINT('',#104553) ;
#30676=VERTEX_POINT('',#104555) ;
#30677=VERTEX_POINT('',#104557) ;
#30678=VERTEX_POINT('',#104561) ;
#30679=VERTEX_POINT('',#104563) ;
#30680=VERTEX_POINT('',#104567) ;
#30681=VERTEX_POINT('',#104568) ;
#30682=VERTEX_POINT('',#104573) ;
#30683=VERTEX_POINT('',#104574) ;
#30684=VERTEX_POINT('',#104577) ;
#30685=VERTEX_POINT('',#104579) ;
#30686=VERTEX_POINT('',#104581) ;
#30687=VERTEX_POINT('',#104585) ;
#30688=VERTEX_POINT('',#104586) ;
#30689=VERTEX_POINT('',#104589) ;
#30690=VERTEX_POINT('',#104593) ;
#30691=VERTEX_POINT('',#104594) ;
#30692=VERTEX_POINT('',#104599) ;
#30693=VERTEX_POINT('',#104600) ;
#30694=VERTEX_POINT('',#104602) ;
#30695=VERTEX_POINT('',#104604) ;
#30696=VERTEX_POINT('',#104608) ;
#30697=VERTEX_POINT('',#104609) ;
#30698=VERTEX_POINT('',#104611) ;
#30699=VERTEX_POINT('',#104613) ;
#30700=VERTEX_POINT('',#104617) ;
#30701=VERTEX_POINT('',#104618) ;
#30702=VERTEX_POINT('',#104620) ;
#30703=VERTEX_POINT('',#104622) ;
#30704=VERTEX_POINT('',#104626) ;
#30705=VERTEX_POINT('',#104628) ;
#30706=VERTEX_POINT('',#104632) ;
#30707=VERTEX_POINT('',#104633) ;
#30708=VERTEX_POINT('',#104635) ;
#30709=VERTEX_POINT('',#104637) ;
#30710=VERTEX_POINT('',#104641) ;
#30711=VERTEX_POINT('',#104642) ;
#30712=VERTEX_POINT('',#104645) ;
#30713=VERTEX_POINT('',#104649) ;
#30714=VERTEX_POINT('',#104650) ;
#30715=VERTEX_POINT('',#104652) ;
#30716=VERTEX_POINT('',#104654) ;
#30717=VERTEX_POINT('',#104658) ;
#30718=VERTEX_POINT('',#104659) ;
#30719=VERTEX_POINT('',#104662) ;
#30720=VERTEX_POINT('',#104664) ;
#30721=VERTEX_POINT('',#104666) ;
#30722=VERTEX_POINT('',#104668) ;
#30723=VERTEX_POINT('',#104672) ;
#30724=VERTEX_POINT('',#104673) ;
#30725=VERTEX_POINT('',#104676) ;
#30726=VERTEX_POINT('',#104680) ;
#30727=VERTEX_POINT('',#104681) ;
#30728=VERTEX_POINT('',#104683) ;
#30729=VERTEX_POINT('',#104685) ;
#30730=VERTEX_POINT('',#104689) ;
#30731=VERTEX_POINT('',#104690) ;
#30732=VERTEX_POINT('',#104692) ;
#30733=VERTEX_POINT('',#104694) ;
#30734=VERTEX_POINT('',#104698) ;
#30735=VERTEX_POINT('',#104699) ;
#30736=VERTEX_POINT('',#104701) ;
#30737=VERTEX_POINT('',#104703) ;
#30738=VERTEX_POINT('',#104707) ;
#30739=VERTEX_POINT('',#104709) ;
#30740=VERTEX_POINT('',#104713) ;
#30741=VERTEX_POINT('',#104715) ;
#30742=VERTEX_POINT('',#104719) ;
#30743=VERTEX_POINT('',#104721) ;
#30744=VERTEX_POINT('',#104725) ;
#30745=VERTEX_POINT('',#104727) ;
#30746=VERTEX_POINT('',#104731) ;
#30747=VERTEX_POINT('',#104732) ;
#30748=VERTEX_POINT('',#104734) ;
#30749=VERTEX_POINT('',#104736) ;
#30750=VERTEX_POINT('',#104738) ;
#30751=VERTEX_POINT('',#104740) ;
#30752=VERTEX_POINT('',#104744) ;
#30753=VERTEX_POINT('',#104745) ;
#30754=VERTEX_POINT('',#104747) ;
#30755=VERTEX_POINT('',#104749) ;
#30756=VERTEX_POINT('',#104751) ;
#30757=VERTEX_POINT('',#104753) ;
#30758=VERTEX_POINT('',#104757) ;
#30759=VERTEX_POINT('',#104758) ;
#30760=VERTEX_POINT('',#104763) ;
#30761=VERTEX_POINT('',#104765) ;
#30762=VERTEX_POINT('',#104769) ;
#30763=VERTEX_POINT('',#104770) ;
#30764=VERTEX_POINT('',#104772) ;
#30765=VERTEX_POINT('',#104774) ;
#30766=VERTEX_POINT('',#104778) ;
#30767=VERTEX_POINT('',#104779) ;
#30768=VERTEX_POINT('',#104781) ;
#30769=VERTEX_POINT('',#104783) ;
#30770=VERTEX_POINT('',#104787) ;
#30771=VERTEX_POINT('',#104788) ;
#30772=VERTEX_POINT('',#104790) ;
#30773=VERTEX_POINT('',#104792) ;
#30774=VERTEX_POINT('',#104796) ;
#30775=VERTEX_POINT('',#104797) ;
#30776=VERTEX_POINT('',#104799) ;
#30777=VERTEX_POINT('',#104801) ;
#30778=VERTEX_POINT('',#104808) ;
#30779=VERTEX_POINT('',#104809) ;
#30780=VERTEX_POINT('',#104811) ;
#30781=VERTEX_POINT('',#104813) ;
#30782=VERTEX_POINT('',#104817) ;
#30783=VERTEX_POINT('',#104818) ;
#30784=VERTEX_POINT('',#104820) ;
#30785=VERTEX_POINT('',#104822) ;
#30786=VERTEX_POINT('',#104826) ;
#30787=VERTEX_POINT('',#104827) ;
#30788=VERTEX_POINT('',#104829) ;
#30789=VERTEX_POINT('',#104831) ;
#30790=VERTEX_POINT('',#104835) ;
#30791=VERTEX_POINT('',#104836) ;
#30792=VERTEX_POINT('',#104838) ;
#30793=VERTEX_POINT('',#104840) ;
#30794=VERTEX_POINT('',#104844) ;
#30795=VERTEX_POINT('',#104846) ;
#30796=VERTEX_POINT('',#104850) ;
#30797=VERTEX_POINT('',#104851) ;
#30798=VERTEX_POINT('',#104856) ;
#30799=VERTEX_POINT('',#104858) ;
#30800=VERTEX_POINT('',#104935) ;
#30801=VERTEX_POINT('',#104952) ;
#30802=VERTEX_POINT('',#104971) ;
#30803=VERTEX_POINT('',#104987) ;
#30804=VERTEX_POINT('',#105004) ;
#30805=VERTEX_POINT('',#105020) ;
#30806=VERTEX_POINT('',#105040) ;
#30807=VERTEX_POINT('',#105044) ;
#30808=VERTEX_POINT('',#105048) ;
#30809=VERTEX_POINT('',#105066) ;
#30810=VERTEX_POINT('',#105084) ;
#30811=VERTEX_POINT('',#105093) ;
#30812=VERTEX_POINT('',#105099) ;
#30813=VERTEX_POINT('',#105107) ;
#30814=VERTEX_POINT('',#105113) ;
#30815=VERTEX_POINT('',#105126) ;
#30816=VERTEX_POINT('',#105232) ;
#30817=VERTEX_POINT('',#105659) ;
#30818=VERTEX_POINT('',#105739) ;
#30819=VERTEX_POINT('',#105750) ;
#30820=VERTEX_POINT('',#105976) ;
#30821=VERTEX_POINT('',#105993) ;
#30822=VERTEX_POINT('',#106221) ;
#30823=VERTEX_POINT('',#106222) ;
#30824=VERTEX_POINT('',#106233) ;
#30825=VERTEX_POINT('',#106235) ;
#30826=VERTEX_POINT('',#106237) ;
#30827=VERTEX_POINT('',#106258) ;
#30828=VERTEX_POINT('',#106259) ;
#30829=VERTEX_POINT('',#106276) ;
#30830=VERTEX_POINT('',#106278) ;
#30831=VERTEX_POINT('',#106280) ;
#30832=VERTEX_POINT('',#106284) ;
#30833=VERTEX_POINT('',#106286) ;
#30834=VERTEX_POINT('',#106290) ;
#30835=VERTEX_POINT('',#106292) ;
#30836=VERTEX_POINT('',#106296) ;
#30837=VERTEX_POINT('',#106297) ;
#30838=VERTEX_POINT('',#106299) ;
#30839=VERTEX_POINT('',#106301) ;
#30840=VERTEX_POINT('',#106303) ;
#30841=VERTEX_POINT('',#106307) ;
#30842=VERTEX_POINT('',#106308) ;
#30843=VERTEX_POINT('',#106310) ;
#30844=VERTEX_POINT('',#106312) ;
#30845=VERTEX_POINT('',#106316) ;
#30846=VERTEX_POINT('',#106317) ;
#30847=VERTEX_POINT('',#106319) ;
#30848=VERTEX_POINT('',#106321) ;
#30849=VERTEX_POINT('',#106327) ;
#30850=VERTEX_POINT('',#106330) ;
#30851=VERTEX_POINT('',#106337) ;
#30852=VERTEX_POINT('',#106345) ;
#30853=VERTEX_POINT('',#106349) ;
#30854=VERTEX_POINT('',#106350) ;
#30855=VERTEX_POINT('',#106352) ;
#30856=VERTEX_POINT('',#106354) ;
#30857=VERTEX_POINT('',#106361) ;
#30858=VERTEX_POINT('',#106363) ;
#30859=VERTEX_POINT('',#106367) ;
#30860=VERTEX_POINT('',#106368) ;
#30861=VERTEX_POINT('',#106370) ;
#30862=VERTEX_POINT('',#106372) ;
#30863=VERTEX_POINT('',#106401) ;
#30864=VERTEX_POINT('',#106412) ;
#30865=VERTEX_POINT('',#106416) ;
#30866=VERTEX_POINT('',#106417) ;
#30867=VERTEX_POINT('',#106419) ;
#30868=VERTEX_POINT('',#106421) ;
#30869=VERTEX_POINT('',#106425) ;
#30870=VERTEX_POINT('',#106426) ;
#30871=VERTEX_POINT('',#106428) ;
#30872=VERTEX_POINT('',#106436) ;
#30873=VERTEX_POINT('',#106449) ;
#30874=VERTEX_POINT('',#106451) ;
#30875=VERTEX_POINT('',#106455) ;
#30876=VERTEX_POINT('',#106456) ;
#30877=VERTEX_POINT('',#106458) ;
#30878=VERTEX_POINT('',#106460) ;
#30879=VERTEX_POINT('',#106464) ;
#30880=VERTEX_POINT('',#106465) ;
#30881=VERTEX_POINT('',#106467) ;
#30882=VERTEX_POINT('',#106469) ;
#30883=VERTEX_POINT('',#106473) ;
#30884=VERTEX_POINT('',#106474) ;
#30885=VERTEX_POINT('',#106476) ;
#30886=VERTEX_POINT('',#106478) ;
#30887=VERTEX_POINT('',#106480) ;
#30888=VERTEX_POINT('',#106482) ;
#30889=VERTEX_POINT('',#106486) ;
#30890=VERTEX_POINT('',#106487) ;
#30891=VERTEX_POINT('',#106492) ;
#30892=VERTEX_POINT('',#106494) ;
#30893=VERTEX_POINT('',#106496) ;
#30894=VERTEX_POINT('',#106498) ;
#30895=VERTEX_POINT('',#106500) ;
#30896=VERTEX_POINT('',#106502) ;
#30897=VERTEX_POINT('',#106504) ;
#30898=VERTEX_POINT('',#106506) ;
#30899=VERTEX_POINT('',#106508) ;
#30900=VERTEX_POINT('',#106510) ;
#30901=VERTEX_POINT('',#106512) ;
#30902=VERTEX_POINT('',#106514) ;
#30903=VERTEX_POINT('',#106517) ;
#30904=VERTEX_POINT('',#106519) ;
#30905=VERTEX_POINT('',#106522) ;
#30906=VERTEX_POINT('',#106524) ;
#30907=VERTEX_POINT('',#106526) ;
#30908=VERTEX_POINT('',#106528) ;
#30909=VERTEX_POINT('',#106530) ;
#30910=VERTEX_POINT('',#106532) ;
#30911=VERTEX_POINT('',#106534) ;
#30912=VERTEX_POINT('',#106538) ;
#30913=VERTEX_POINT('',#106539) ;
#30914=VERTEX_POINT('',#106541) ;
#30915=VERTEX_POINT('',#106543) ;
#30916=VERTEX_POINT('',#106545) ;
#30917=VERTEX_POINT('',#106547) ;
#30918=VERTEX_POINT('',#106549) ;
#30919=VERTEX_POINT('',#106551) ;
#30920=VERTEX_POINT('',#106553) ;
#30921=VERTEX_POINT('',#106555) ;
#30922=VERTEX_POINT('',#106557) ;
#30923=VERTEX_POINT('',#106560) ;
#30924=VERTEX_POINT('',#106562) ;
#30925=VERTEX_POINT('',#106565) ;
#30926=VERTEX_POINT('',#106567) ;
#30927=VERTEX_POINT('',#106569) ;
#30928=VERTEX_POINT('',#106571) ;
#30929=VERTEX_POINT('',#106573) ;
#30930=VERTEX_POINT('',#106575) ;
#30931=VERTEX_POINT('',#106577) ;
#30932=VERTEX_POINT('',#106579) ;
#30933=VERTEX_POINT('',#106581) ;
#30934=VERTEX_POINT('',#106583) ;
#30935=VERTEX_POINT('',#106585) ;
#30936=VERTEX_POINT('',#106587) ;
#30937=VERTEX_POINT('',#106589) ;
#30938=VERTEX_POINT('',#106591) ;
#30939=VERTEX_POINT('',#106593) ;
#30940=VERTEX_POINT('',#106595) ;
#30941=VERTEX_POINT('',#106605) ;
#30942=VERTEX_POINT('',#106606) ;
#30943=VERTEX_POINT('',#106649) ;
#30944=VERTEX_POINT('',#106651) ;
#30945=VERTEX_POINT('',#106694) ;
#30946=VERTEX_POINT('',#106695) ;
#30947=VERTEX_POINT('',#106703) ;
#30948=VERTEX_POINT('',#106706) ;
#30949=VERTEX_POINT('',#106710) ;
#30950=VERTEX_POINT('',#106711) ;
#30951=VERTEX_POINT('',#106716) ;
#30952=VERTEX_POINT('',#106731) ;
#30953=VERTEX_POINT('',#106736) ;
#30954=VERTEX_POINT('',#106738) ;
#30955=VERTEX_POINT('',#106773) ;
#30956=VERTEX_POINT('',#106775) ;
#30957=VERTEX_POINT('',#106829) ;
#30958=VERTEX_POINT('',#106831) ;
#30959=VERTEX_POINT('',#106833) ;
#30960=VERTEX_POINT('',#106835) ;
#30961=VERTEX_POINT('',#106837) ;
#30962=VERTEX_POINT('',#106839) ;
#30963=VERTEX_POINT('',#106843) ;
#30964=VERTEX_POINT('',#106844) ;
#30965=VERTEX_POINT('',#106847) ;
#30966=VERTEX_POINT('',#106849) ;
#30967=VERTEX_POINT('',#106851) ;
#30968=VERTEX_POINT('',#106853) ;
#30969=VERTEX_POINT('',#106855) ;
#30970=VERTEX_POINT('',#106857) ;
#30971=VERTEX_POINT('',#106859) ;
#30972=VERTEX_POINT('',#106861) ;
#30973=VERTEX_POINT('',#106863) ;
#30974=VERTEX_POINT('',#106865) ;
#30975=VERTEX_POINT('',#106868) ;
#30976=VERTEX_POINT('',#106870) ;
#30977=VERTEX_POINT('',#106872) ;
#30978=VERTEX_POINT('',#106874) ;
#30979=VERTEX_POINT('',#106876) ;
#30980=VERTEX_POINT('',#106878) ;
#30981=VERTEX_POINT('',#106880) ;
#30982=VERTEX_POINT('',#106882) ;
#30983=VERTEX_POINT('',#106886) ;
#30984=VERTEX_POINT('',#106887) ;
#30985=VERTEX_POINT('',#106889) ;
#30986=VERTEX_POINT('',#106893) ;
#30987=VERTEX_POINT('',#106895) ;
#30988=VERTEX_POINT('',#106897) ;
#30989=VERTEX_POINT('',#106901) ;
#30990=VERTEX_POINT('',#106902) ;
#30991=VERTEX_POINT('',#106906) ;
#30992=VERTEX_POINT('',#106908) ;
#30993=VERTEX_POINT('',#106912) ;
#30994=VERTEX_POINT('',#106913) ;
#30995=VERTEX_POINT('',#106915) ;
#30996=VERTEX_POINT('',#106919) ;
#30997=VERTEX_POINT('',#106920) ;
#30998=VERTEX_POINT('',#106922) ;
#30999=VERTEX_POINT('',#106926) ;
#31000=VERTEX_POINT('',#106927) ;
#31001=VERTEX_POINT('',#106929) ;
#31002=VERTEX_POINT('',#106931) ;
#31003=VERTEX_POINT('',#106933) ;
#31004=VERTEX_POINT('',#106935) ;
#31005=VERTEX_POINT('',#106937) ;
#31006=VERTEX_POINT('',#106939) ;
#31007=VERTEX_POINT('',#106943) ;
#31008=VERTEX_POINT('',#106944) ;
#31009=VERTEX_POINT('',#106946) ;
#31010=VERTEX_POINT('',#106948) ;
#31011=VERTEX_POINT('',#106952) ;
#31012=VERTEX_POINT('',#106953) ;
#31013=VERTEX_POINT('',#106955) ;
#31014=VERTEX_POINT('',#106957) ;
#31015=VERTEX_POINT('',#106961) ;
#31016=VERTEX_POINT('',#106962) ;
#31017=VERTEX_POINT('',#106964) ;
#31018=VERTEX_POINT('',#106966) ;
#31019=VERTEX_POINT('',#106970) ;
#31020=VERTEX_POINT('',#106971) ;
#31021=VERTEX_POINT('',#106980) ;
#31022=VERTEX_POINT('',#106982) ;
#31023=VERTEX_POINT('',#106984) ;
#31024=VERTEX_POINT('',#106986) ;
#31025=VERTEX_POINT('',#106997) ;
#31026=VERTEX_POINT('',#106998) ;
#31027=VERTEX_POINT('',#107000) ;
#31028=VERTEX_POINT('',#107002) ;
#31029=VERTEX_POINT('',#107004) ;
#31030=VERTEX_POINT('',#107006) ;
#31031=VERTEX_POINT('',#107008) ;
#31032=VERTEX_POINT('',#107010) ;
#31033=VERTEX_POINT('',#107014) ;
#31034=VERTEX_POINT('',#107015) ;
#31035=VERTEX_POINT('',#107017) ;
#31036=VERTEX_POINT('',#107019) ;
#31037=VERTEX_POINT('',#107021) ;
#31038=VERTEX_POINT('',#107023) ;
#31039=VERTEX_POINT('',#107025) ;
#31040=VERTEX_POINT('',#107027) ;
#31041=VERTEX_POINT('',#107031) ;
#31042=VERTEX_POINT('',#107032) ;
#31043=VERTEX_POINT('',#107035) ;
#31044=VERTEX_POINT('',#107037) ;
#31045=VERTEX_POINT('',#107039) ;
#31046=VERTEX_POINT('',#107043) ;
#31047=VERTEX_POINT('',#107045) ;
#31048=VERTEX_POINT('',#107049) ;
#31049=VERTEX_POINT('',#107050) ;
#31050=VERTEX_POINT('',#107055) ;
#31051=VERTEX_POINT('',#107056) ;
#31052=VERTEX_POINT('',#107058) ;
#31053=VERTEX_POINT('',#107060) ;
#31054=VERTEX_POINT('',#107064) ;
#31055=VERTEX_POINT('',#107065) ;
#31056=VERTEX_POINT('',#107067) ;
#31057=VERTEX_POINT('',#107069) ;
#31058=VERTEX_POINT('',#107073) ;
#31059=VERTEX_POINT('',#107075) ;
#31060=VERTEX_POINT('',#107079) ;
#31061=VERTEX_POINT('',#107080) ;
#31062=VERTEX_POINT('',#107085) ;
#31063=VERTEX_POINT('',#107086) ;
#31064=VERTEX_POINT('',#107089) ;
#31065=VERTEX_POINT('',#107091) ;
#31066=VERTEX_POINT('',#107093) ;
#31067=VERTEX_POINT('',#107097) ;
#31068=VERTEX_POINT('',#107098) ;
#31069=VERTEX_POINT('',#107101) ;
#31070=VERTEX_POINT('',#107105) ;
#31071=VERTEX_POINT('',#107106) ;
#31072=VERTEX_POINT('',#107111) ;
#31073=VERTEX_POINT('',#107112) ;
#31074=VERTEX_POINT('',#107114) ;
#31075=VERTEX_POINT('',#107116) ;
#31076=VERTEX_POINT('',#107120) ;
#31077=VERTEX_POINT('',#107121) ;
#31078=VERTEX_POINT('',#107123) ;
#31079=VERTEX_POINT('',#107125) ;
#31080=VERTEX_POINT('',#107129) ;
#31081=VERTEX_POINT('',#107130) ;
#31082=VERTEX_POINT('',#107132) ;
#31083=VERTEX_POINT('',#107134) ;
#31084=VERTEX_POINT('',#107138) ;
#31085=VERTEX_POINT('',#107140) ;
#31086=VERTEX_POINT('',#107144) ;
#31087=VERTEX_POINT('',#107145) ;
#31088=VERTEX_POINT('',#107147) ;
#31089=VERTEX_POINT('',#107149) ;
#31090=VERTEX_POINT('',#107153) ;
#31091=VERTEX_POINT('',#107154) ;
#31092=VERTEX_POINT('',#107157) ;
#31093=VERTEX_POINT('',#107161) ;
#31094=VERTEX_POINT('',#107162) ;
#31095=VERTEX_POINT('',#107164) ;
#31096=VERTEX_POINT('',#107166) ;
#31097=VERTEX_POINT('',#107170) ;
#31098=VERTEX_POINT('',#107171) ;
#31099=VERTEX_POINT('',#107174) ;
#31100=VERTEX_POINT('',#107176) ;
#31101=VERTEX_POINT('',#107178) ;
#31102=VERTEX_POINT('',#107180) ;
#31103=VERTEX_POINT('',#107184) ;
#31104=VERTEX_POINT('',#107185) ;
#31105=VERTEX_POINT('',#107188) ;
#31106=VERTEX_POINT('',#107192) ;
#31107=VERTEX_POINT('',#107193) ;
#31108=VERTEX_POINT('',#107195) ;
#31109=VERTEX_POINT('',#107197) ;
#31110=VERTEX_POINT('',#107201) ;
#31111=VERTEX_POINT('',#107202) ;
#31112=VERTEX_POINT('',#107204) ;
#31113=VERTEX_POINT('',#107206) ;
#31114=VERTEX_POINT('',#107210) ;
#31115=VERTEX_POINT('',#107211) ;
#31116=VERTEX_POINT('',#107213) ;
#31117=VERTEX_POINT('',#107215) ;
#31118=VERTEX_POINT('',#107219) ;
#31119=VERTEX_POINT('',#107221) ;
#31120=VERTEX_POINT('',#107225) ;
#31121=VERTEX_POINT('',#107227) ;
#31122=VERTEX_POINT('',#107231) ;
#31123=VERTEX_POINT('',#107233) ;
#31124=VERTEX_POINT('',#107237) ;
#31125=VERTEX_POINT('',#107239) ;
#31126=VERTEX_POINT('',#107243) ;
#31127=VERTEX_POINT('',#107244) ;
#31128=VERTEX_POINT('',#107246) ;
#31129=VERTEX_POINT('',#107248) ;
#31130=VERTEX_POINT('',#107250) ;
#31131=VERTEX_POINT('',#107252) ;
#31132=VERTEX_POINT('',#107256) ;
#31133=VERTEX_POINT('',#107257) ;
#31134=VERTEX_POINT('',#107259) ;
#31135=VERTEX_POINT('',#107261) ;
#31136=VERTEX_POINT('',#107263) ;
#31137=VERTEX_POINT('',#107265) ;
#31138=VERTEX_POINT('',#107269) ;
#31139=VERTEX_POINT('',#107270) ;
#31140=VERTEX_POINT('',#107275) ;
#31141=VERTEX_POINT('',#107277) ;
#31142=VERTEX_POINT('',#107281) ;
#31143=VERTEX_POINT('',#107282) ;
#31144=VERTEX_POINT('',#107284) ;
#31145=VERTEX_POINT('',#107286) ;
#31146=VERTEX_POINT('',#107290) ;
#31147=VERTEX_POINT('',#107291) ;
#31148=VERTEX_POINT('',#107293) ;
#31149=VERTEX_POINT('',#107295) ;
#31150=VERTEX_POINT('',#107299) ;
#31151=VERTEX_POINT('',#107300) ;
#31152=VERTEX_POINT('',#107302) ;
#31153=VERTEX_POINT('',#107304) ;
#31154=VERTEX_POINT('',#107308) ;
#31155=VERTEX_POINT('',#107309) ;
#31156=VERTEX_POINT('',#107311) ;
#31157=VERTEX_POINT('',#107313) ;
#31158=VERTEX_POINT('',#107320) ;
#31159=VERTEX_POINT('',#107321) ;
#31160=VERTEX_POINT('',#107323) ;
#31161=VERTEX_POINT('',#107325) ;
#31162=VERTEX_POINT('',#107329) ;
#31163=VERTEX_POINT('',#107330) ;
#31164=VERTEX_POINT('',#107332) ;
#31165=VERTEX_POINT('',#107334) ;
#31166=VERTEX_POINT('',#107338) ;
#31167=VERTEX_POINT('',#107339) ;
#31168=VERTEX_POINT('',#107341) ;
#31169=VERTEX_POINT('',#107343) ;
#31170=VERTEX_POINT('',#107347) ;
#31171=VERTEX_POINT('',#107348) ;
#31172=VERTEX_POINT('',#107350) ;
#31173=VERTEX_POINT('',#107352) ;
#31174=VERTEX_POINT('',#107356) ;
#31175=VERTEX_POINT('',#107358) ;
#31176=VERTEX_POINT('',#107362) ;
#31177=VERTEX_POINT('',#107363) ;
#31178=VERTEX_POINT('',#107368) ;
#31179=VERTEX_POINT('',#107370) ;
#31180=VERTEX_POINT('',#107447) ;
#31181=VERTEX_POINT('',#107464) ;
#31182=VERTEX_POINT('',#107483) ;
#31183=VERTEX_POINT('',#107499) ;
#31184=VERTEX_POINT('',#107516) ;
#31185=VERTEX_POINT('',#107532) ;
#31186=VERTEX_POINT('',#107552) ;
#31187=VERTEX_POINT('',#107556) ;
#31188=VERTEX_POINT('',#107560) ;
#31189=VERTEX_POINT('',#107578) ;
#31190=VERTEX_POINT('',#107596) ;
#31191=VERTEX_POINT('',#107605) ;
#31192=VERTEX_POINT('',#107611) ;
#31193=VERTEX_POINT('',#107619) ;
#31194=VERTEX_POINT('',#107625) ;
#31195=VERTEX_POINT('',#107638) ;
#31196=VERTEX_POINT('',#107744) ;
#31197=VERTEX_POINT('',#108171) ;
#31198=VERTEX_POINT('',#108251) ;
#31199=VERTEX_POINT('',#108262) ;
#31200=VERTEX_POINT('',#108488) ;
#31201=VERTEX_POINT('',#108505) ;
#31202=VERTEX_POINT('',#108733) ;
#31203=VERTEX_POINT('',#108734) ;
#31204=VERTEX_POINT('',#108745) ;
#31205=VERTEX_POINT('',#108747) ;
#31206=VERTEX_POINT('',#108749) ;
#31207=VERTEX_POINT('',#108770) ;
#31208=VERTEX_POINT('',#108771) ;
#31209=VERTEX_POINT('',#108788) ;
#31210=VERTEX_POINT('',#108790) ;
#31211=VERTEX_POINT('',#108792) ;
#31212=VERTEX_POINT('',#108796) ;
#31213=VERTEX_POINT('',#108798) ;
#31214=VERTEX_POINT('',#108802) ;
#31215=VERTEX_POINT('',#108804) ;
#31216=VERTEX_POINT('',#108808) ;
#31217=VERTEX_POINT('',#108809) ;
#31218=VERTEX_POINT('',#108811) ;
#31219=VERTEX_POINT('',#108813) ;
#31220=VERTEX_POINT('',#108815) ;
#31221=VERTEX_POINT('',#108819) ;
#31222=VERTEX_POINT('',#108820) ;
#31223=VERTEX_POINT('',#108822) ;
#31224=VERTEX_POINT('',#108824) ;
#31225=VERTEX_POINT('',#108828) ;
#31226=VERTEX_POINT('',#108829) ;
#31227=VERTEX_POINT('',#108831) ;
#31228=VERTEX_POINT('',#108833) ;
#31229=VERTEX_POINT('',#108839) ;
#31230=VERTEX_POINT('',#108842) ;
#31231=VERTEX_POINT('',#108849) ;
#31232=VERTEX_POINT('',#108857) ;
#31233=VERTEX_POINT('',#108861) ;
#31234=VERTEX_POINT('',#108862) ;
#31235=VERTEX_POINT('',#108864) ;
#31236=VERTEX_POINT('',#108866) ;
#31237=VERTEX_POINT('',#108873) ;
#31238=VERTEX_POINT('',#108875) ;
#31239=VERTEX_POINT('',#108879) ;
#31240=VERTEX_POINT('',#108880) ;
#31241=VERTEX_POINT('',#108882) ;
#31242=VERTEX_POINT('',#108884) ;
#31243=VERTEX_POINT('',#108913) ;
#31244=VERTEX_POINT('',#108924) ;
#31245=VERTEX_POINT('',#108928) ;
#31246=VERTEX_POINT('',#108929) ;
#31247=VERTEX_POINT('',#108931) ;
#31248=VERTEX_POINT('',#108933) ;
#31249=VERTEX_POINT('',#108937) ;
#31250=VERTEX_POINT('',#108938) ;
#31251=VERTEX_POINT('',#108940) ;
#31252=VERTEX_POINT('',#108948) ;
#31253=VERTEX_POINT('',#108961) ;
#31254=VERTEX_POINT('',#108963) ;
#31255=VERTEX_POINT('',#108967) ;
#31256=VERTEX_POINT('',#108968) ;
#31257=VERTEX_POINT('',#108970) ;
#31258=VERTEX_POINT('',#108972) ;
#31259=VERTEX_POINT('',#108976) ;
#31260=VERTEX_POINT('',#108977) ;
#31261=VERTEX_POINT('',#108979) ;
#31262=VERTEX_POINT('',#108981) ;
#31263=VERTEX_POINT('',#108985) ;
#31264=VERTEX_POINT('',#108986) ;
#31265=VERTEX_POINT('',#108988) ;
#31266=VERTEX_POINT('',#108990) ;
#31267=VERTEX_POINT('',#108992) ;
#31268=VERTEX_POINT('',#108994) ;
#31269=VERTEX_POINT('',#108998) ;
#31270=VERTEX_POINT('',#108999) ;
#31271=VERTEX_POINT('',#109004) ;
#31272=VERTEX_POINT('',#109006) ;
#31273=VERTEX_POINT('',#109008) ;
#31274=VERTEX_POINT('',#109010) ;
#31275=VERTEX_POINT('',#109012) ;
#31276=VERTEX_POINT('',#109014) ;
#31277=VERTEX_POINT('',#109016) ;
#31278=VERTEX_POINT('',#109018) ;
#31279=VERTEX_POINT('',#109020) ;
#31280=VERTEX_POINT('',#109022) ;
#31281=VERTEX_POINT('',#109024) ;
#31282=VERTEX_POINT('',#109026) ;
#31283=VERTEX_POINT('',#109029) ;
#31284=VERTEX_POINT('',#109031) ;
#31285=VERTEX_POINT('',#109034) ;
#31286=VERTEX_POINT('',#109036) ;
#31287=VERTEX_POINT('',#109038) ;
#31288=VERTEX_POINT('',#109040) ;
#31289=VERTEX_POINT('',#109042) ;
#31290=VERTEX_POINT('',#109044) ;
#31291=VERTEX_POINT('',#109046) ;
#31292=VERTEX_POINT('',#109050) ;
#31293=VERTEX_POINT('',#109051) ;
#31294=VERTEX_POINT('',#109053) ;
#31295=VERTEX_POINT('',#109055) ;
#31296=VERTEX_POINT('',#109057) ;
#31297=VERTEX_POINT('',#109059) ;
#31298=VERTEX_POINT('',#109061) ;
#31299=VERTEX_POINT('',#109063) ;
#31300=VERTEX_POINT('',#109065) ;
#31301=VERTEX_POINT('',#109067) ;
#31302=VERTEX_POINT('',#109069) ;
#31303=VERTEX_POINT('',#109072) ;
#31304=VERTEX_POINT('',#109074) ;
#31305=VERTEX_POINT('',#109077) ;
#31306=VERTEX_POINT('',#109079) ;
#31307=VERTEX_POINT('',#109081) ;
#31308=VERTEX_POINT('',#109083) ;
#31309=VERTEX_POINT('',#109085) ;
#31310=VERTEX_POINT('',#109087) ;
#31311=VERTEX_POINT('',#109089) ;
#31312=VERTEX_POINT('',#109091) ;
#31313=VERTEX_POINT('',#109093) ;
#31314=VERTEX_POINT('',#109095) ;
#31315=VERTEX_POINT('',#109097) ;
#31316=VERTEX_POINT('',#109099) ;
#31317=VERTEX_POINT('',#109101) ;
#31318=VERTEX_POINT('',#109103) ;
#31319=VERTEX_POINT('',#109105) ;
#31320=VERTEX_POINT('',#109107) ;
#31321=VERTEX_POINT('',#109117) ;
#31322=VERTEX_POINT('',#109118) ;
#31323=VERTEX_POINT('',#109161) ;
#31324=VERTEX_POINT('',#109163) ;
#31325=VERTEX_POINT('',#109206) ;
#31326=VERTEX_POINT('',#109207) ;
#31327=VERTEX_POINT('',#109215) ;
#31328=VERTEX_POINT('',#109218) ;
#31329=VERTEX_POINT('',#109222) ;
#31330=VERTEX_POINT('',#109223) ;
#31331=VERTEX_POINT('',#109228) ;
#31332=VERTEX_POINT('',#109243) ;
#31333=VERTEX_POINT('',#109248) ;
#31334=VERTEX_POINT('',#109250) ;
#31335=VERTEX_POINT('',#109285) ;
#31336=VERTEX_POINT('',#109287) ;
#31337=VERTEX_POINT('',#109341) ;
#31338=VERTEX_POINT('',#109343) ;
#31339=VERTEX_POINT('',#109345) ;
#31340=VERTEX_POINT('',#109347) ;
#31341=VERTEX_POINT('',#109349) ;
#31342=VERTEX_POINT('',#109351) ;
#31343=VERTEX_POINT('',#109355) ;
#31344=VERTEX_POINT('',#109356) ;
#31345=VERTEX_POINT('',#109359) ;
#31346=VERTEX_POINT('',#109361) ;
#31347=VERTEX_POINT('',#109363) ;
#31348=VERTEX_POINT('',#109365) ;
#31349=VERTEX_POINT('',#109367) ;
#31350=VERTEX_POINT('',#109369) ;
#31351=VERTEX_POINT('',#109371) ;
#31352=VERTEX_POINT('',#109373) ;
#31353=VERTEX_POINT('',#109375) ;
#31354=VERTEX_POINT('',#109377) ;
#31355=VERTEX_POINT('',#109380) ;
#31356=VERTEX_POINT('',#109382) ;
#31357=VERTEX_POINT('',#109384) ;
#31358=VERTEX_POINT('',#109386) ;
#31359=VERTEX_POINT('',#109388) ;
#31360=VERTEX_POINT('',#109390) ;
#31361=VERTEX_POINT('',#109392) ;
#31362=VERTEX_POINT('',#109394) ;
#31363=VERTEX_POINT('',#109398) ;
#31364=VERTEX_POINT('',#109399) ;
#31365=VERTEX_POINT('',#109401) ;
#31366=VERTEX_POINT('',#109405) ;
#31367=VERTEX_POINT('',#109407) ;
#31368=VERTEX_POINT('',#109409) ;
#31369=VERTEX_POINT('',#109413) ;
#31370=VERTEX_POINT('',#109414) ;
#31371=VERTEX_POINT('',#109418) ;
#31372=VERTEX_POINT('',#109420) ;
#31373=VERTEX_POINT('',#109424) ;
#31374=VERTEX_POINT('',#109425) ;
#31375=VERTEX_POINT('',#109427) ;
#31376=VERTEX_POINT('',#109431) ;
#31377=VERTEX_POINT('',#109432) ;
#31378=VERTEX_POINT('',#109434) ;
#31379=VERTEX_POINT('',#109438) ;
#31380=VERTEX_POINT('',#109439) ;
#31381=VERTEX_POINT('',#109441) ;
#31382=VERTEX_POINT('',#109443) ;
#31383=VERTEX_POINT('',#109445) ;
#31384=VERTEX_POINT('',#109447) ;
#31385=VERTEX_POINT('',#109449) ;
#31386=VERTEX_POINT('',#109451) ;
#31387=VERTEX_POINT('',#109455) ;
#31388=VERTEX_POINT('',#109456) ;
#31389=VERTEX_POINT('',#109458) ;
#31390=VERTEX_POINT('',#109460) ;
#31391=VERTEX_POINT('',#109464) ;
#31392=VERTEX_POINT('',#109465) ;
#31393=VERTEX_POINT('',#109467) ;
#31394=VERTEX_POINT('',#109469) ;
#31395=VERTEX_POINT('',#109473) ;
#31396=VERTEX_POINT('',#109474) ;
#31397=VERTEX_POINT('',#109476) ;
#31398=VERTEX_POINT('',#109478) ;
#31399=VERTEX_POINT('',#109482) ;
#31400=VERTEX_POINT('',#109483) ;
#31401=VERTEX_POINT('',#109492) ;
#31402=VERTEX_POINT('',#109494) ;
#31403=VERTEX_POINT('',#109496) ;
#31404=VERTEX_POINT('',#109498) ;
#31405=VERTEX_POINT('',#109509) ;
#31406=VERTEX_POINT('',#109510) ;
#31407=VERTEX_POINT('',#109512) ;
#31408=VERTEX_POINT('',#109514) ;
#31409=VERTEX_POINT('',#109516) ;
#31410=VERTEX_POINT('',#109518) ;
#31411=VERTEX_POINT('',#109520) ;
#31412=VERTEX_POINT('',#109522) ;
#31413=VERTEX_POINT('',#109526) ;
#31414=VERTEX_POINT('',#109527) ;
#31415=VERTEX_POINT('',#109529) ;
#31416=VERTEX_POINT('',#109531) ;
#31417=VERTEX_POINT('',#109533) ;
#31418=VERTEX_POINT('',#109535) ;
#31419=VERTEX_POINT('',#109537) ;
#31420=VERTEX_POINT('',#109539) ;
#31421=VERTEX_POINT('',#109543) ;
#31422=VERTEX_POINT('',#109544) ;
#31423=VERTEX_POINT('',#109547) ;
#31424=VERTEX_POINT('',#109549) ;
#31425=VERTEX_POINT('',#109551) ;
#31426=VERTEX_POINT('',#109555) ;
#31427=VERTEX_POINT('',#109557) ;
#31428=VERTEX_POINT('',#109561) ;
#31429=VERTEX_POINT('',#109562) ;
#31430=VERTEX_POINT('',#109567) ;
#31431=VERTEX_POINT('',#109568) ;
#31432=VERTEX_POINT('',#109570) ;
#31433=VERTEX_POINT('',#109572) ;
#31434=VERTEX_POINT('',#109576) ;
#31435=VERTEX_POINT('',#109577) ;
#31436=VERTEX_POINT('',#109579) ;
#31437=VERTEX_POINT('',#109581) ;
#31438=VERTEX_POINT('',#109585) ;
#31439=VERTEX_POINT('',#109587) ;
#31440=VERTEX_POINT('',#109591) ;
#31441=VERTEX_POINT('',#109592) ;
#31442=VERTEX_POINT('',#109597) ;
#31443=VERTEX_POINT('',#109598) ;
#31444=VERTEX_POINT('',#109601) ;
#31445=VERTEX_POINT('',#109603) ;
#31446=VERTEX_POINT('',#109605) ;
#31447=VERTEX_POINT('',#109609) ;
#31448=VERTEX_POINT('',#109610) ;
#31449=VERTEX_POINT('',#109613) ;
#31450=VERTEX_POINT('',#109617) ;
#31451=VERTEX_POINT('',#109618) ;
#31452=VERTEX_POINT('',#109623) ;
#31453=VERTEX_POINT('',#109624) ;
#31454=VERTEX_POINT('',#109626) ;
#31455=VERTEX_POINT('',#109628) ;
#31456=VERTEX_POINT('',#109632) ;
#31457=VERTEX_POINT('',#109633) ;
#31458=VERTEX_POINT('',#109635) ;
#31459=VERTEX_POINT('',#109637) ;
#31460=VERTEX_POINT('',#109641) ;
#31461=VERTEX_POINT('',#109642) ;
#31462=VERTEX_POINT('',#109644) ;
#31463=VERTEX_POINT('',#109646) ;
#31464=VERTEX_POINT('',#109650) ;
#31465=VERTEX_POINT('',#109652) ;
#31466=VERTEX_POINT('',#109656) ;
#31467=VERTEX_POINT('',#109657) ;
#31468=VERTEX_POINT('',#109659) ;
#31469=VERTEX_POINT('',#109661) ;
#31470=VERTEX_POINT('',#109665) ;
#31471=VERTEX_POINT('',#109666) ;
#31472=VERTEX_POINT('',#109669) ;
#31473=VERTEX_POINT('',#109673) ;
#31474=VERTEX_POINT('',#109674) ;
#31475=VERTEX_POINT('',#109676) ;
#31476=VERTEX_POINT('',#109678) ;
#31477=VERTEX_POINT('',#109682) ;
#31478=VERTEX_POINT('',#109683) ;
#31479=VERTEX_POINT('',#109686) ;
#31480=VERTEX_POINT('',#109688) ;
#31481=VERTEX_POINT('',#109690) ;
#31482=VERTEX_POINT('',#109692) ;
#31483=VERTEX_POINT('',#109696) ;
#31484=VERTEX_POINT('',#109697) ;
#31485=VERTEX_POINT('',#109700) ;
#31486=VERTEX_POINT('',#109704) ;
#31487=VERTEX_POINT('',#109705) ;
#31488=VERTEX_POINT('',#109707) ;
#31489=VERTEX_POINT('',#109709) ;
#31490=VERTEX_POINT('',#109713) ;
#31491=VERTEX_POINT('',#109714) ;
#31492=VERTEX_POINT('',#109716) ;
#31493=VERTEX_POINT('',#109718) ;
#31494=VERTEX_POINT('',#109722) ;
#31495=VERTEX_POINT('',#109723) ;
#31496=VERTEX_POINT('',#109725) ;
#31497=VERTEX_POINT('',#109727) ;
#31498=VERTEX_POINT('',#109731) ;
#31499=VERTEX_POINT('',#109733) ;
#31500=VERTEX_POINT('',#109737) ;
#31501=VERTEX_POINT('',#109739) ;
#31502=VERTEX_POINT('',#109743) ;
#31503=VERTEX_POINT('',#109745) ;
#31504=VERTEX_POINT('',#109749) ;
#31505=VERTEX_POINT('',#109751) ;
#31506=VERTEX_POINT('',#109755) ;
#31507=VERTEX_POINT('',#109756) ;
#31508=VERTEX_POINT('',#109758) ;
#31509=VERTEX_POINT('',#109760) ;
#31510=VERTEX_POINT('',#109762) ;
#31511=VERTEX_POINT('',#109764) ;
#31512=VERTEX_POINT('',#109768) ;
#31513=VERTEX_POINT('',#109769) ;
#31514=VERTEX_POINT('',#109771) ;
#31515=VERTEX_POINT('',#109773) ;
#31516=VERTEX_POINT('',#109775) ;
#31517=VERTEX_POINT('',#109777) ;
#31518=VERTEX_POINT('',#109781) ;
#31519=VERTEX_POINT('',#109782) ;
#31520=VERTEX_POINT('',#109787) ;
#31521=VERTEX_POINT('',#109789) ;
#31522=VERTEX_POINT('',#109793) ;
#31523=VERTEX_POINT('',#109794) ;
#31524=VERTEX_POINT('',#109796) ;
#31525=VERTEX_POINT('',#109798) ;
#31526=VERTEX_POINT('',#109802) ;
#31527=VERTEX_POINT('',#109803) ;
#31528=VERTEX_POINT('',#109805) ;
#31529=VERTEX_POINT('',#109807) ;
#31530=VERTEX_POINT('',#109811) ;
#31531=VERTEX_POINT('',#109812) ;
#31532=VERTEX_POINT('',#109814) ;
#31533=VERTEX_POINT('',#109816) ;
#31534=VERTEX_POINT('',#109820) ;
#31535=VERTEX_POINT('',#109821) ;
#31536=VERTEX_POINT('',#109823) ;
#31537=VERTEX_POINT('',#109825) ;
#31538=VERTEX_POINT('',#109832) ;
#31539=VERTEX_POINT('',#109833) ;
#31540=VERTEX_POINT('',#109835) ;
#31541=VERTEX_POINT('',#109837) ;
#31542=VERTEX_POINT('',#109841) ;
#31543=VERTEX_POINT('',#109842) ;
#31544=VERTEX_POINT('',#109844) ;
#31545=VERTEX_POINT('',#109846) ;
#31546=VERTEX_POINT('',#109850) ;
#31547=VERTEX_POINT('',#109851) ;
#31548=VERTEX_POINT('',#109853) ;
#31549=VERTEX_POINT('',#109855) ;
#31550=VERTEX_POINT('',#109859) ;
#31551=VERTEX_POINT('',#109860) ;
#31552=VERTEX_POINT('',#109862) ;
#31553=VERTEX_POINT('',#109864) ;
#31554=VERTEX_POINT('',#109868) ;
#31555=VERTEX_POINT('',#109870) ;
#31556=VERTEX_POINT('',#109874) ;
#31557=VERTEX_POINT('',#109875) ;
#31558=VERTEX_POINT('',#109880) ;
#31559=VERTEX_POINT('',#109882) ;
#31560=VERTEX_POINT('',#109959) ;
#31561=VERTEX_POINT('',#109976) ;
#31562=VERTEX_POINT('',#109995) ;
#31563=VERTEX_POINT('',#110011) ;
#31564=VERTEX_POINT('',#110028) ;
#31565=VERTEX_POINT('',#110044) ;
#31566=VERTEX_POINT('',#110064) ;
#31567=VERTEX_POINT('',#110068) ;
#31568=VERTEX_POINT('',#110072) ;
#31569=VERTEX_POINT('',#110090) ;
#31570=VERTEX_POINT('',#110108) ;
#31571=VERTEX_POINT('',#110117) ;
#31572=VERTEX_POINT('',#110123) ;
#31573=VERTEX_POINT('',#110131) ;
#31574=VERTEX_POINT('',#110137) ;
#31575=VERTEX_POINT('',#110150) ;
#31576=VERTEX_POINT('',#110256) ;
#31577=VERTEX_POINT('',#110683) ;
#31578=VERTEX_POINT('',#110763) ;
#31579=VERTEX_POINT('',#110774) ;
#31580=VERTEX_POINT('',#111000) ;
#31581=VERTEX_POINT('',#111017) ;
#31582=VERTEX_POINT('',#111245) ;
#31583=VERTEX_POINT('',#111246) ;
#31584=VERTEX_POINT('',#111257) ;
#31585=VERTEX_POINT('',#111259) ;
#31586=VERTEX_POINT('',#111261) ;
#31587=VERTEX_POINT('',#111282) ;
#31588=VERTEX_POINT('',#111283) ;
#31589=VERTEX_POINT('',#111300) ;
#31590=VERTEX_POINT('',#111302) ;
#31591=VERTEX_POINT('',#111304) ;
#31592=VERTEX_POINT('',#111308) ;
#31593=VERTEX_POINT('',#111310) ;
#31594=VERTEX_POINT('',#111314) ;
#31595=VERTEX_POINT('',#111316) ;
#31596=VERTEX_POINT('',#111320) ;
#31597=VERTEX_POINT('',#111321) ;
#31598=VERTEX_POINT('',#111323) ;
#31599=VERTEX_POINT('',#111325) ;
#31600=VERTEX_POINT('',#111327) ;
#31601=VERTEX_POINT('',#111331) ;
#31602=VERTEX_POINT('',#111332) ;
#31603=VERTEX_POINT('',#111334) ;
#31604=VERTEX_POINT('',#111336) ;
#31605=VERTEX_POINT('',#111340) ;
#31606=VERTEX_POINT('',#111341) ;
#31607=VERTEX_POINT('',#111343) ;
#31608=VERTEX_POINT('',#111345) ;
#31609=VERTEX_POINT('',#111351) ;
#31610=VERTEX_POINT('',#111354) ;
#31611=VERTEX_POINT('',#111361) ;
#31612=VERTEX_POINT('',#111369) ;
#31613=VERTEX_POINT('',#111373) ;
#31614=VERTEX_POINT('',#111374) ;
#31615=VERTEX_POINT('',#111376) ;
#31616=VERTEX_POINT('',#111378) ;
#31617=VERTEX_POINT('',#111385) ;
#31618=VERTEX_POINT('',#111387) ;
#31619=VERTEX_POINT('',#111391) ;
#31620=VERTEX_POINT('',#111392) ;
#31621=VERTEX_POINT('',#111394) ;
#31622=VERTEX_POINT('',#111396) ;
#31623=VERTEX_POINT('',#111425) ;
#31624=VERTEX_POINT('',#111436) ;
#31625=VERTEX_POINT('',#111440) ;
#31626=VERTEX_POINT('',#111441) ;
#31627=VERTEX_POINT('',#111443) ;
#31628=VERTEX_POINT('',#111445) ;
#31629=VERTEX_POINT('',#111449) ;
#31630=VERTEX_POINT('',#111450) ;
#31631=VERTEX_POINT('',#111452) ;
#31632=VERTEX_POINT('',#111460) ;
#31633=VERTEX_POINT('',#111473) ;
#31634=VERTEX_POINT('',#111475) ;
#31635=VERTEX_POINT('',#111479) ;
#31636=VERTEX_POINT('',#111480) ;
#31637=VERTEX_POINT('',#111482) ;
#31638=VERTEX_POINT('',#111484) ;
#31639=VERTEX_POINT('',#111488) ;
#31640=VERTEX_POINT('',#111489) ;
#31641=VERTEX_POINT('',#111491) ;
#31642=VERTEX_POINT('',#111493) ;
#31643=VERTEX_POINT('',#111497) ;
#31644=VERTEX_POINT('',#111498) ;
#31645=VERTEX_POINT('',#111500) ;
#31646=VERTEX_POINT('',#111502) ;
#31647=VERTEX_POINT('',#111504) ;
#31648=VERTEX_POINT('',#111506) ;
#31649=VERTEX_POINT('',#111510) ;
#31650=VERTEX_POINT('',#111511) ;
#31651=VERTEX_POINT('',#111516) ;
#31652=VERTEX_POINT('',#111518) ;
#31653=VERTEX_POINT('',#111520) ;
#31654=VERTEX_POINT('',#111522) ;
#31655=VERTEX_POINT('',#111524) ;
#31656=VERTEX_POINT('',#111526) ;
#31657=VERTEX_POINT('',#111528) ;
#31658=VERTEX_POINT('',#111530) ;
#31659=VERTEX_POINT('',#111532) ;
#31660=VERTEX_POINT('',#111534) ;
#31661=VERTEX_POINT('',#111536) ;
#31662=VERTEX_POINT('',#111538) ;
#31663=VERTEX_POINT('',#111541) ;
#31664=VERTEX_POINT('',#111543) ;
#31665=VERTEX_POINT('',#111546) ;
#31666=VERTEX_POINT('',#111548) ;
#31667=VERTEX_POINT('',#111550) ;
#31668=VERTEX_POINT('',#111552) ;
#31669=VERTEX_POINT('',#111554) ;
#31670=VERTEX_POINT('',#111556) ;
#31671=VERTEX_POINT('',#111558) ;
#31672=VERTEX_POINT('',#111562) ;
#31673=VERTEX_POINT('',#111563) ;
#31674=VERTEX_POINT('',#111565) ;
#31675=VERTEX_POINT('',#111567) ;
#31676=VERTEX_POINT('',#111569) ;
#31677=VERTEX_POINT('',#111571) ;
#31678=VERTEX_POINT('',#111573) ;
#31679=VERTEX_POINT('',#111575) ;
#31680=VERTEX_POINT('',#111577) ;
#31681=VERTEX_POINT('',#111579) ;
#31682=VERTEX_POINT('',#111581) ;
#31683=VERTEX_POINT('',#111584) ;
#31684=VERTEX_POINT('',#111586) ;
#31685=VERTEX_POINT('',#111589) ;
#31686=VERTEX_POINT('',#111591) ;
#31687=VERTEX_POINT('',#111593) ;
#31688=VERTEX_POINT('',#111595) ;
#31689=VERTEX_POINT('',#111597) ;
#31690=VERTEX_POINT('',#111599) ;
#31691=VERTEX_POINT('',#111601) ;
#31692=VERTEX_POINT('',#111603) ;
#31693=VERTEX_POINT('',#111605) ;
#31694=VERTEX_POINT('',#111607) ;
#31695=VERTEX_POINT('',#111609) ;
#31696=VERTEX_POINT('',#111611) ;
#31697=VERTEX_POINT('',#111613) ;
#31698=VERTEX_POINT('',#111615) ;
#31699=VERTEX_POINT('',#111617) ;
#31700=VERTEX_POINT('',#111619) ;
#31701=VERTEX_POINT('',#111629) ;
#31702=VERTEX_POINT('',#111630) ;
#31703=VERTEX_POINT('',#111673) ;
#31704=VERTEX_POINT('',#111675) ;
#31705=VERTEX_POINT('',#111718) ;
#31706=VERTEX_POINT('',#111719) ;
#31707=VERTEX_POINT('',#111727) ;
#31708=VERTEX_POINT('',#111730) ;
#31709=VERTEX_POINT('',#111734) ;
#31710=VERTEX_POINT('',#111735) ;
#31711=VERTEX_POINT('',#111740) ;
#31712=VERTEX_POINT('',#111755) ;
#31713=VERTEX_POINT('',#111760) ;
#31714=VERTEX_POINT('',#111762) ;
#31715=VERTEX_POINT('',#111797) ;
#31716=VERTEX_POINT('',#111799) ;
#31717=VERTEX_POINT('',#111853) ;
#31718=VERTEX_POINT('',#111855) ;
#31719=VERTEX_POINT('',#111857) ;
#31720=VERTEX_POINT('',#111859) ;
#31721=VERTEX_POINT('',#111861) ;
#31722=VERTEX_POINT('',#111863) ;
#31723=VERTEX_POINT('',#111867) ;
#31724=VERTEX_POINT('',#111868) ;
#31725=VERTEX_POINT('',#111871) ;
#31726=VERTEX_POINT('',#111873) ;
#31727=VERTEX_POINT('',#111875) ;
#31728=VERTEX_POINT('',#111877) ;
#31729=VERTEX_POINT('',#111879) ;
#31730=VERTEX_POINT('',#111881) ;
#31731=VERTEX_POINT('',#111883) ;
#31732=VERTEX_POINT('',#111885) ;
#31733=VERTEX_POINT('',#111887) ;
#31734=VERTEX_POINT('',#111889) ;
#31735=VERTEX_POINT('',#111892) ;
#31736=VERTEX_POINT('',#111894) ;
#31737=VERTEX_POINT('',#111896) ;
#31738=VERTEX_POINT('',#111898) ;
#31739=VERTEX_POINT('',#111900) ;
#31740=VERTEX_POINT('',#111902) ;
#31741=VERTEX_POINT('',#111904) ;
#31742=VERTEX_POINT('',#111906) ;
#31743=VERTEX_POINT('',#111910) ;
#31744=VERTEX_POINT('',#111911) ;
#31745=VERTEX_POINT('',#111913) ;
#31746=VERTEX_POINT('',#111917) ;
#31747=VERTEX_POINT('',#111919) ;
#31748=VERTEX_POINT('',#111921) ;
#31749=VERTEX_POINT('',#111925) ;
#31750=VERTEX_POINT('',#111926) ;
#31751=VERTEX_POINT('',#111930) ;
#31752=VERTEX_POINT('',#111932) ;
#31753=VERTEX_POINT('',#111936) ;
#31754=VERTEX_POINT('',#111937) ;
#31755=VERTEX_POINT('',#111939) ;
#31756=VERTEX_POINT('',#111943) ;
#31757=VERTEX_POINT('',#111944) ;
#31758=VERTEX_POINT('',#111946) ;
#31759=VERTEX_POINT('',#111950) ;
#31760=VERTEX_POINT('',#111951) ;
#31761=VERTEX_POINT('',#111953) ;
#31762=VERTEX_POINT('',#111955) ;
#31763=VERTEX_POINT('',#111957) ;
#31764=VERTEX_POINT('',#111959) ;
#31765=VERTEX_POINT('',#111961) ;
#31766=VERTEX_POINT('',#111963) ;
#31767=VERTEX_POINT('',#111967) ;
#31768=VERTEX_POINT('',#111968) ;
#31769=VERTEX_POINT('',#111970) ;
#31770=VERTEX_POINT('',#111972) ;
#31771=VERTEX_POINT('',#111976) ;
#31772=VERTEX_POINT('',#111977) ;
#31773=VERTEX_POINT('',#111979) ;
#31774=VERTEX_POINT('',#111981) ;
#31775=VERTEX_POINT('',#111985) ;
#31776=VERTEX_POINT('',#111986) ;
#31777=VERTEX_POINT('',#111988) ;
#31778=VERTEX_POINT('',#111990) ;
#31779=VERTEX_POINT('',#111994) ;
#31780=VERTEX_POINT('',#111995) ;
#31781=VERTEX_POINT('',#112004) ;
#31782=VERTEX_POINT('',#112006) ;
#31783=VERTEX_POINT('',#112008) ;
#31784=VERTEX_POINT('',#112010) ;
#31785=VERTEX_POINT('',#112021) ;
#31786=VERTEX_POINT('',#112022) ;
#31787=VERTEX_POINT('',#112024) ;
#31788=VERTEX_POINT('',#112026) ;
#31789=VERTEX_POINT('',#112028) ;
#31790=VERTEX_POINT('',#112030) ;
#31791=VERTEX_POINT('',#112032) ;
#31792=VERTEX_POINT('',#112034) ;
#31793=VERTEX_POINT('',#112038) ;
#31794=VERTEX_POINT('',#112039) ;
#31795=VERTEX_POINT('',#112041) ;
#31796=VERTEX_POINT('',#112043) ;
#31797=VERTEX_POINT('',#112045) ;
#31798=VERTEX_POINT('',#112047) ;
#31799=VERTEX_POINT('',#112049) ;
#31800=VERTEX_POINT('',#112051) ;
#31801=VERTEX_POINT('',#112055) ;
#31802=VERTEX_POINT('',#112056) ;
#31803=VERTEX_POINT('',#112059) ;
#31804=VERTEX_POINT('',#112061) ;
#31805=VERTEX_POINT('',#112063) ;
#31806=VERTEX_POINT('',#112067) ;
#31807=VERTEX_POINT('',#112069) ;
#31808=VERTEX_POINT('',#112073) ;
#31809=VERTEX_POINT('',#112074) ;
#31810=VERTEX_POINT('',#112079) ;
#31811=VERTEX_POINT('',#112080) ;
#31812=VERTEX_POINT('',#112082) ;
#31813=VERTEX_POINT('',#112084) ;
#31814=VERTEX_POINT('',#112088) ;
#31815=VERTEX_POINT('',#112089) ;
#31816=VERTEX_POINT('',#112091) ;
#31817=VERTEX_POINT('',#112093) ;
#31818=VERTEX_POINT('',#112097) ;
#31819=VERTEX_POINT('',#112099) ;
#31820=VERTEX_POINT('',#112103) ;
#31821=VERTEX_POINT('',#112104) ;
#31822=VERTEX_POINT('',#112109) ;
#31823=VERTEX_POINT('',#112110) ;
#31824=VERTEX_POINT('',#112113) ;
#31825=VERTEX_POINT('',#112115) ;
#31826=VERTEX_POINT('',#112117) ;
#31827=VERTEX_POINT('',#112121) ;
#31828=VERTEX_POINT('',#112122) ;
#31829=VERTEX_POINT('',#112125) ;
#31830=VERTEX_POINT('',#112129) ;
#31831=VERTEX_POINT('',#112130) ;
#31832=VERTEX_POINT('',#112135) ;
#31833=VERTEX_POINT('',#112136) ;
#31834=VERTEX_POINT('',#112138) ;
#31835=VERTEX_POINT('',#112140) ;
#31836=VERTEX_POINT('',#112144) ;
#31837=VERTEX_POINT('',#112145) ;
#31838=VERTEX_POINT('',#112147) ;
#31839=VERTEX_POINT('',#112149) ;
#31840=VERTEX_POINT('',#112153) ;
#31841=VERTEX_POINT('',#112154) ;
#31842=VERTEX_POINT('',#112156) ;
#31843=VERTEX_POINT('',#112158) ;
#31844=VERTEX_POINT('',#112162) ;
#31845=VERTEX_POINT('',#112164) ;
#31846=VERTEX_POINT('',#112168) ;
#31847=VERTEX_POINT('',#112169) ;
#31848=VERTEX_POINT('',#112171) ;
#31849=VERTEX_POINT('',#112173) ;
#31850=VERTEX_POINT('',#112177) ;
#31851=VERTEX_POINT('',#112178) ;
#31852=VERTEX_POINT('',#112181) ;
#31853=VERTEX_POINT('',#112185) ;
#31854=VERTEX_POINT('',#112186) ;
#31855=VERTEX_POINT('',#112188) ;
#31856=VERTEX_POINT('',#112190) ;
#31857=VERTEX_POINT('',#112194) ;
#31858=VERTEX_POINT('',#112195) ;
#31859=VERTEX_POINT('',#112198) ;
#31860=VERTEX_POINT('',#112200) ;
#31861=VERTEX_POINT('',#112202) ;
#31862=VERTEX_POINT('',#112204) ;
#31863=VERTEX_POINT('',#112208) ;
#31864=VERTEX_POINT('',#112209) ;
#31865=VERTEX_POINT('',#112212) ;
#31866=VERTEX_POINT('',#112216) ;
#31867=VERTEX_POINT('',#112217) ;
#31868=VERTEX_POINT('',#112219) ;
#31869=VERTEX_POINT('',#112221) ;
#31870=VERTEX_POINT('',#112225) ;
#31871=VERTEX_POINT('',#112226) ;
#31872=VERTEX_POINT('',#112228) ;
#31873=VERTEX_POINT('',#112230) ;
#31874=VERTEX_POINT('',#112234) ;
#31875=VERTEX_POINT('',#112235) ;
#31876=VERTEX_POINT('',#112237) ;
#31877=VERTEX_POINT('',#112239) ;
#31878=VERTEX_POINT('',#112243) ;
#31879=VERTEX_POINT('',#112245) ;
#31880=VERTEX_POINT('',#112249) ;
#31881=VERTEX_POINT('',#112251) ;
#31882=VERTEX_POINT('',#112255) ;
#31883=VERTEX_POINT('',#112257) ;
#31884=VERTEX_POINT('',#112261) ;
#31885=VERTEX_POINT('',#112263) ;
#31886=VERTEX_POINT('',#112267) ;
#31887=VERTEX_POINT('',#112268) ;
#31888=VERTEX_POINT('',#112270) ;
#31889=VERTEX_POINT('',#112272) ;
#31890=VERTEX_POINT('',#112274) ;
#31891=VERTEX_POINT('',#112276) ;
#31892=VERTEX_POINT('',#112280) ;
#31893=VERTEX_POINT('',#112281) ;
#31894=VERTEX_POINT('',#112283) ;
#31895=VERTEX_POINT('',#112285) ;
#31896=VERTEX_POINT('',#112287) ;
#31897=VERTEX_POINT('',#112289) ;
#31898=VERTEX_POINT('',#112293) ;
#31899=VERTEX_POINT('',#112294) ;
#31900=VERTEX_POINT('',#112299) ;
#31901=VERTEX_POINT('',#112301) ;
#31902=VERTEX_POINT('',#112305) ;
#31903=VERTEX_POINT('',#112306) ;
#31904=VERTEX_POINT('',#112308) ;
#31905=VERTEX_POINT('',#112310) ;
#31906=VERTEX_POINT('',#112314) ;
#31907=VERTEX_POINT('',#112315) ;
#31908=VERTEX_POINT('',#112317) ;
#31909=VERTEX_POINT('',#112319) ;
#31910=VERTEX_POINT('',#112323) ;
#31911=VERTEX_POINT('',#112324) ;
#31912=VERTEX_POINT('',#112326) ;
#31913=VERTEX_POINT('',#112328) ;
#31914=VERTEX_POINT('',#112332) ;
#31915=VERTEX_POINT('',#112333) ;
#31916=VERTEX_POINT('',#112335) ;
#31917=VERTEX_POINT('',#112337) ;
#31918=VERTEX_POINT('',#112344) ;
#31919=VERTEX_POINT('',#112345) ;
#31920=VERTEX_POINT('',#112347) ;
#31921=VERTEX_POINT('',#112349) ;
#31922=VERTEX_POINT('',#112353) ;
#31923=VERTEX_POINT('',#112354) ;
#31924=VERTEX_POINT('',#112356) ;
#31925=VERTEX_POINT('',#112358) ;
#31926=VERTEX_POINT('',#112362) ;
#31927=VERTEX_POINT('',#112363) ;
#31928=VERTEX_POINT('',#112365) ;
#31929=VERTEX_POINT('',#112367) ;
#31930=VERTEX_POINT('',#112371) ;
#31931=VERTEX_POINT('',#112372) ;
#31932=VERTEX_POINT('',#112374) ;
#31933=VERTEX_POINT('',#112376) ;
#31934=VERTEX_POINT('',#112380) ;
#31935=VERTEX_POINT('',#112382) ;
#31936=VERTEX_POINT('',#112386) ;
#31937=VERTEX_POINT('',#112387) ;
#31938=VERTEX_POINT('',#112392) ;
#31939=VERTEX_POINT('',#112394) ;
#31940=VERTEX_POINT('',#112471) ;
#31941=VERTEX_POINT('',#112488) ;
#31942=VERTEX_POINT('',#112507) ;
#31943=VERTEX_POINT('',#112523) ;
#31944=VERTEX_POINT('',#112540) ;
#31945=VERTEX_POINT('',#112556) ;
#31946=VERTEX_POINT('',#112576) ;
#31947=VERTEX_POINT('',#112580) ;
#31948=VERTEX_POINT('',#112584) ;
#31949=VERTEX_POINT('',#112602) ;
#31950=VERTEX_POINT('',#112620) ;
#31951=VERTEX_POINT('',#112629) ;
#31952=VERTEX_POINT('',#112635) ;
#31953=VERTEX_POINT('',#112643) ;
#31954=VERTEX_POINT('',#112649) ;
#31955=VERTEX_POINT('',#112662) ;
#31956=VERTEX_POINT('',#112768) ;
#31957=VERTEX_POINT('',#113195) ;
#31958=VERTEX_POINT('',#113275) ;
#31959=VERTEX_POINT('',#113286) ;
#31960=VERTEX_POINT('',#113512) ;
#31961=VERTEX_POINT('',#113529) ;
#35709=EDGE_CURVE('',#30062,#30063,#75,.T.) ;
#35710=EDGE_CURVE('',#30063,#30064,#4848,.T.) ;
#35711=EDGE_CURVE('',#30064,#30065,#25273,.T.) ;
#35712=EDGE_CURVE('',#30066,#30065,#4849,.T.) ;
#35713=EDGE_CURVE('',#30062,#30066,#76,.T.) ;
#35714=EDGE_CURVE('',#30067,#30068,#77,.T.) ;
#35715=EDGE_CURVE('',#30068,#30069,#25274,.T.) ;
#35716=EDGE_CURVE('',#30070,#30069,#4850,.T.) ;
#35717=EDGE_CURVE('',#30071,#30070,#25275,.T.) ;
#35718=EDGE_CURVE('',#30067,#30071,#4851,.T.) ;
#35719=EDGE_CURVE('',#30072,#30072,#25276,.T.) ;
#35720=EDGE_CURVE('',#30072,#30073,#25277,.T.) ;
#35721=EDGE_CURVE('',#30073,#30073,#25278,.T.) ;
#35722=EDGE_CURVE('',#30074,#30074,#25279,.T.) ;
#35723=EDGE_CURVE('',#30074,#30075,#25280,.T.) ;
#35724=EDGE_CURVE('',#30075,#30075,#25281,.T.) ;
#35725=EDGE_CURVE('',#30076,#30077,#25282,.T.) ;
#35726=EDGE_CURVE('',#30078,#30076,#8351,.T.) ;
#35727=EDGE_CURVE('',#30078,#30079,#25283,.T.) ;
#35728=EDGE_CURVE('',#30079,#30080,#25284,.T.) ;
#35729=EDGE_CURVE('',#30077,#30080,#8352,.T.) ;
#35730=EDGE_CURVE('',#30081,#30082,#25285,.T.) ;
#35731=EDGE_CURVE('',#30083,#30081,#8353,.T.) ;
#35732=EDGE_CURVE('',#30083,#30084,#25286,.T.) ;
#35733=EDGE_CURVE('',#30082,#30084,#8354,.T.) ;
#35734=EDGE_CURVE('',#30085,#30086,#25287,.T.) ;
#35735=EDGE_CURVE('',#30085,#30087,#25288,.T.) ;
#35736=EDGE_CURVE('',#30088,#30087,#25289,.T.) ;
#35737=EDGE_CURVE('',#30088,#30086,#25290,.T.) ;
#35738=EDGE_CURVE('',#30073,#30074,#8355,.T.) ;
#35739=EDGE_CURVE('',#30086,#30089,#8356,.T.) ;
#35740=EDGE_CURVE('',#30089,#30083,#25291,.T.) ;
#35741=EDGE_CURVE('',#30090,#30081,#78,.T.) ;
#35742=EDGE_CURVE('',#30090,#30091,#25292,.T.) ;
#35743=EDGE_CURVE('',#30077,#30091,#79,.T.) ;
#35744=EDGE_CURVE('',#30080,#30092,#25293,.T.) ;
#35745=EDGE_CURVE('',#30092,#30085,#8357,.T.) ;
#35746=EDGE_CURVE('',#30093,#30094,#8358,.T.) ;
#35747=EDGE_CURVE('',#30094,#30095,#8359,.T.) ;
#35748=EDGE_CURVE('',#30095,#30096,#80,.T.) ;
#35749=EDGE_CURVE('',#30096,#30097,#8360,.T.) ;
#35750=EDGE_CURVE('',#30097,#30098,#4852,.T.) ;
#35751=EDGE_CURVE('',#30098,#30093,#8361,.T.) ;
#35752=EDGE_CURVE('',#30099,#30100,#8362,.T.) ;
#35753=EDGE_CURVE('',#30100,#30101,#8363,.T.) ;
#35754=EDGE_CURVE('',#30101,#30102,#81,.T.) ;
#35755=EDGE_CURVE('',#30102,#30103,#82,.T.) ;
#35756=EDGE_CURVE('',#30103,#30104,#8364,.T.) ;
#35757=EDGE_CURVE('',#30104,#30099,#8365,.T.) ;
#35758=EDGE_CURVE('',#30105,#30106,#8366,.T.) ;
#35759=EDGE_CURVE('',#30106,#30107,#8367,.T.) ;
#35760=EDGE_CURVE('',#30107,#30108,#8368,.T.) ;
#35761=EDGE_CURVE('',#30108,#30105,#8369,.T.) ;
#35762=EDGE_CURVE('',#30109,#30110,#8370,.T.) ;
#35763=EDGE_CURVE('',#30110,#30111,#83,.T.) ;
#35764=EDGE_CURVE('',#30111,#30112,#84,.T.) ;
#35765=EDGE_CURVE('',#30112,#30113,#8371,.T.) ;
#35766=EDGE_CURVE('',#30113,#30114,#8372,.T.) ;
#35767=EDGE_CURVE('',#30114,#30109,#8373,.T.) ;
#35768=EDGE_CURVE('',#30115,#30116,#8374,.T.) ;
#35769=EDGE_CURVE('',#30116,#30117,#8375,.T.) ;
#35770=EDGE_CURVE('',#30117,#30118,#8376,.T.) ;
#35771=EDGE_CURVE('',#30118,#30115,#8377,.T.) ;
#35772=EDGE_CURVE('',#30119,#30120,#8378,.T.) ;
#35773=EDGE_CURVE('',#30119,#30121,#8379,.T.) ;
#35774=EDGE_CURVE('',#30121,#30122,#8380,.T.) ;
#35775=EDGE_CURVE('',#30122,#30120,#8381,.T.) ;
#35776=EDGE_CURVE('',#30123,#30124,#8382,.T.) ;
#35777=EDGE_CURVE('',#30123,#30125,#8383,.T.) ;
#35778=EDGE_CURVE('',#30125,#30126,#8384,.T.) ;
#35779=EDGE_CURVE('',#30126,#30127,#8385,.T.) ;
#35780=EDGE_CURVE('',#30127,#30128,#25294,.T.) ;
#35781=EDGE_CURVE('',#30128,#30124,#8386,.T.) ;
#35782=EDGE_CURVE('',#30129,#30130,#8387,.T.) ;
#35783=EDGE_CURVE('',#30129,#30100,#25295,.T.) ;
#35784=EDGE_CURVE('',#30099,#30106,#25296,.T.) ;
#35785=EDGE_CURVE('',#30105,#30114,#25297,.T.) ;
#35786=EDGE_CURVE('',#30113,#30131,#25298,.T.) ;
#35787=EDGE_CURVE('',#30132,#30131,#8388,.T.) ;
#35788=EDGE_CURVE('',#30132,#30133,#25299,.T.) ;
#35789=EDGE_CURVE('',#30134,#30133,#8389,.T.) ;
#35790=EDGE_CURVE('',#30134,#30135,#25300,.T.) ;
#35791=EDGE_CURVE('',#30135,#30136,#8390,.T.) ;
#35792=EDGE_CURVE('',#30136,#30137,#25301,.T.) ;
#35793=EDGE_CURVE('',#30138,#30137,#8391,.T.) ;
#35794=EDGE_CURVE('',#30138,#30139,#25302,.T.) ;
#35795=EDGE_CURVE('',#30139,#30140,#8392,.T.) ;
#35796=EDGE_CURVE('',#30140,#30141,#25303,.T.) ;
#35797=EDGE_CURVE('',#30142,#30141,#8393,.T.) ;
#35798=EDGE_CURVE('',#30142,#30118,#25304,.T.) ;
#35799=EDGE_CURVE('',#30117,#30143,#25305,.T.) ;
#35800=EDGE_CURVE('',#30143,#30144,#8394,.T.) ;
#35801=EDGE_CURVE('',#30144,#30126,#25306,.T.) ;
#35802=EDGE_CURVE('',#30125,#30145,#25307,.T.) ;
#35803=EDGE_CURVE('',#30146,#30145,#8395,.T.) ;
#35804=EDGE_CURVE('',#30147,#30146,#8396,.T.) ;
#35805=EDGE_CURVE('',#30147,#30148,#25308,.T.) ;
#35806=EDGE_CURVE('',#30149,#30148,#8397,.T.) ;
#35807=EDGE_CURVE('',#30149,#30150,#25309,.T.) ;
#35808=EDGE_CURVE('',#30151,#30150,#8398,.T.) ;
#35809=EDGE_CURVE('',#30151,#30130,#25310,.T.) ;
#35810=EDGE_CURVE('',#30152,#30153,#8399,.T.) ;
#35811=EDGE_CURVE('',#30153,#30154,#25311,.T.) ;
#35812=EDGE_CURVE('',#30154,#30155,#8400,.T.) ;
#35813=EDGE_CURVE('',#30155,#30156,#25312,.T.) ;
#35814=EDGE_CURVE('',#30156,#30157,#8401,.T.) ;
#35815=EDGE_CURVE('',#30157,#30158,#25313,.T.) ;
#35816=EDGE_CURVE('',#30158,#30159,#8402,.T.) ;
#35817=EDGE_CURVE('',#30159,#30160,#25314,.T.) ;
#35818=EDGE_CURVE('',#30160,#30161,#8403,.T.) ;
#35819=EDGE_CURVE('',#30161,#30162,#8404,.T.) ;
#35820=EDGE_CURVE('',#30162,#30123,#25315,.T.) ;
#35821=EDGE_CURVE('',#30124,#30163,#25316,.T.) ;
#35822=EDGE_CURVE('',#30163,#30164,#8405,.T.) ;
#35823=EDGE_CURVE('',#30164,#30119,#25317,.T.) ;
#35824=EDGE_CURVE('',#30120,#30165,#25318,.T.) ;
#35825=EDGE_CURVE('',#30166,#30165,#8406,.T.) ;
#35826=EDGE_CURVE('',#30166,#30167,#25319,.T.) ;
#35827=EDGE_CURVE('',#30168,#30167,#8407,.T.) ;
#35828=EDGE_CURVE('',#30168,#30169,#25320,.T.) ;
#35829=EDGE_CURVE('',#30169,#30170,#8408,.T.) ;
#35830=EDGE_CURVE('',#30170,#30171,#25321,.T.) ;
#35831=EDGE_CURVE('',#30172,#30171,#8409,.T.) ;
#35832=EDGE_CURVE('',#30172,#30173,#25322,.T.) ;
#35833=EDGE_CURVE('',#30174,#30173,#8410,.T.) ;
#35834=EDGE_CURVE('',#30174,#30175,#25323,.T.) ;
#35835=EDGE_CURVE('',#30175,#30176,#8411,.T.) ;
#35836=EDGE_CURVE('',#30176,#30177,#25324,.T.) ;
#35837=EDGE_CURVE('',#30177,#30178,#8412,.T.) ;
#35838=EDGE_CURVE('',#30178,#30179,#25325,.T.) ;
#35839=EDGE_CURVE('',#30179,#30180,#8413,.T.) ;
#35840=EDGE_CURVE('',#30180,#30152,#25326,.T.) ;
#35841=EDGE_CURVE('',#30148,#30159,#8414,.T.) ;
#35842=EDGE_CURVE('',#30158,#30149,#8415,.T.) ;
#35843=EDGE_CURVE('',#30150,#30157,#8416,.T.) ;
#35844=EDGE_CURVE('',#30156,#30151,#8417,.T.) ;
#35845=EDGE_CURVE('',#30181,#30182,#85,.T.) ;
#35846=EDGE_CURVE('',#30182,#30129,#8418,.T.) ;
#35847=EDGE_CURVE('',#30130,#30155,#8419,.T.) ;
#35848=EDGE_CURVE('',#30154,#30183,#8420,.T.) ;
#35849=EDGE_CURVE('',#30183,#30184,#86,.T.) ;
#35850=EDGE_CURVE('',#30184,#30181,#8421,.T.) ;
#35851=EDGE_CURVE('',#30185,#30186,#87,.T.) ;
#35852=EDGE_CURVE('',#30186,#30187,#4853,.T.) ;
#35853=EDGE_CURVE('',#30187,#30153,#8422,.T.) ;
#35854=EDGE_CURVE('',#30152,#30188,#8423,.T.) ;
#35855=EDGE_CURVE('',#30188,#30185,#8424,.T.) ;
#35856=EDGE_CURVE('',#30189,#30190,#8425,.T.) ;
#35857=EDGE_CURVE('',#30190,#30180,#8426,.T.) ;
#35858=EDGE_CURVE('',#30179,#30189,#8427,.T.) ;
#35859=EDGE_CURVE('',#30191,#30062,#88,.T.) ;
#35860=EDGE_CURVE('',#30066,#30192,#8428,.T.) ;
#35861=EDGE_CURVE('',#30192,#30178,#8429,.T.) ;
#35862=EDGE_CURVE('',#30177,#30191,#8430,.T.) ;
#35863=EDGE_CURVE('',#30131,#30193,#8431,.T.) ;
#35864=EDGE_CURVE('',#30193,#30194,#89,.T.) ;
#35865=EDGE_CURVE('',#30194,#30195,#8432,.T.) ;
#35866=EDGE_CURVE('',#30195,#30196,#90,.T.) ;
#35867=EDGE_CURVE('',#30196,#30176,#8433,.T.) ;
#35868=EDGE_CURVE('',#30175,#30197,#8434,.T.) ;
#35869=EDGE_CURVE('',#30197,#30198,#8435,.T.) ;
#35870=EDGE_CURVE('',#30199,#30198,#25327,.T.) ;
#35871=EDGE_CURVE('',#30199,#30200,#8436,.T.) ;
#35872=EDGE_CURVE('',#30201,#30200,#25328,.T.) ;
#35873=EDGE_CURVE('',#30201,#30202,#8437,.T.) ;
#35874=EDGE_CURVE('',#30202,#30132,#8438,.T.) ;
#35875=EDGE_CURVE('',#30203,#30204,#25329,.T.) ;
#35876=EDGE_CURVE('',#30203,#30138,#8439,.T.) ;
#35877=EDGE_CURVE('',#30137,#30205,#8440,.T.) ;
#35878=EDGE_CURVE('',#30206,#30205,#25330,.T.) ;
#35879=EDGE_CURVE('',#30206,#30207,#25331,.T.) ;
#35880=EDGE_CURVE('',#30208,#30207,#25332,.T.) ;
#35881=EDGE_CURVE('',#30208,#30209,#8441,.T.) ;
#35882=EDGE_CURVE('',#30209,#30210,#8442,.T.) ;
#35883=EDGE_CURVE('',#30210,#30211,#8443,.T.) ;
#35884=EDGE_CURVE('',#30212,#30211,#25333,.T.) ;
#35885=EDGE_CURVE('',#30212,#30213,#25334,.T.) ;
#35886=EDGE_CURVE('',#30214,#30213,#25335,.T.) ;
#35887=EDGE_CURVE('',#30214,#30170,#8444,.T.) ;
#35888=EDGE_CURVE('',#30169,#30215,#8445,.T.) ;
#35889=EDGE_CURVE('',#30216,#30215,#25336,.T.) ;
#35890=EDGE_CURVE('',#30216,#30217,#25337,.T.) ;
#35891=EDGE_CURVE('',#30218,#30217,#25338,.T.) ;
#35892=EDGE_CURVE('',#30218,#30219,#8446,.T.) ;
#35893=EDGE_CURVE('',#30219,#30220,#25339,.T.) ;
#35894=EDGE_CURVE('',#30220,#30221,#8447,.T.) ;
#35895=EDGE_CURVE('',#30222,#30221,#25340,.T.) ;
#35896=EDGE_CURVE('',#30222,#30204,#25341,.T.) ;
#35897=EDGE_CURVE('',#30223,#30224,#25342,.T.) ;
#35898=EDGE_CURVE('',#30223,#30225,#8448,.T.) ;
#35899=EDGE_CURVE('',#30146,#30225,#8449,.T.) ;
#35900=EDGE_CURVE('',#30145,#30162,#8450,.T.) ;
#35901=EDGE_CURVE('',#30226,#30161,#8451,.T.) ;
#35902=EDGE_CURVE('',#30226,#30227,#8452,.T.) ;
#35903=EDGE_CURVE('',#30228,#30227,#25343,.T.) ;
#35904=EDGE_CURVE('',#30228,#30224,#8453,.T.) ;
#35905=EDGE_CURVE('',#30229,#30230,#25344,.T.) ;
#35906=EDGE_CURVE('',#30229,#30226,#8454,.T.) ;
#35907=EDGE_CURVE('',#30160,#30147,#8455,.T.) ;
#35908=EDGE_CURVE('',#30225,#30231,#8456,.T.) ;
#35909=EDGE_CURVE('',#30232,#30231,#25345,.T.) ;
#35910=EDGE_CURVE('',#30232,#30230,#8457,.T.) ;
#35911=EDGE_CURVE('',#30233,#30234,#8458,.T.) ;
#35912=EDGE_CURVE('',#30234,#30235,#8459,.T.) ;
#35913=EDGE_CURVE('',#30233,#30235,#25346,.T.) ;
#35914=EDGE_CURVE('',#30236,#30237,#25347,.T.) ;
#35915=EDGE_CURVE('',#30236,#30238,#8460,.T.) ;
#35916=EDGE_CURVE('',#30238,#30237,#8461,.T.) ;
#35917=EDGE_CURVE('',#30239,#30240,#8462,.T.) ;
#35918=EDGE_CURVE('',#30240,#30241,#8463,.T.) ;
#35919=EDGE_CURVE('',#30241,#30242,#8464,.T.) ;
#35920=EDGE_CURVE('',#30242,#30243,#8465,.T.) ;
#35921=EDGE_CURVE('',#30243,#30244,#8466,.T.) ;
#35922=EDGE_CURVE('',#30244,#30245,#8467,.T.) ;
#35923=EDGE_CURVE('',#30245,#30246,#8468,.T.) ;
#35924=EDGE_CURVE('',#30246,#30239,#8469,.T.) ;
#35925=EDGE_CURVE('',#30247,#30248,#8470,.T.) ;
#35926=EDGE_CURVE('',#30248,#30249,#8471,.T.) ;
#35927=EDGE_CURVE('',#30249,#30250,#8472,.T.) ;
#35928=EDGE_CURVE('',#30250,#30247,#8473,.T.) ;
#35929=EDGE_CURVE('',#30251,#30252,#8474,.T.) ;
#35930=EDGE_CURVE('',#30252,#30253,#8475,.T.) ;
#35931=EDGE_CURVE('',#30253,#30254,#8476,.T.) ;
#35932=EDGE_CURVE('',#30254,#30251,#8477,.T.) ;
#35933=EDGE_CURVE('',#30255,#30256,#8478,.T.) ;
#35934=EDGE_CURVE('',#30256,#30257,#8479,.T.) ;
#35935=EDGE_CURVE('',#30257,#30258,#8480,.T.) ;
#35936=EDGE_CURVE('',#30258,#30255,#8481,.T.) ;
#35937=EDGE_CURVE('',#30259,#30260,#91,.T.) ;
#35938=EDGE_CURVE('',#30260,#30261,#8482,.T.) ;
#35939=EDGE_CURVE('',#30261,#30262,#8483,.T.) ;
#35940=EDGE_CURVE('',#30262,#30263,#8484,.T.) ;
#35941=EDGE_CURVE('',#30263,#30264,#92,.T.) ;
#35942=EDGE_CURVE('',#30264,#30259,#8485,.T.) ;
#35943=EDGE_CURVE('',#30265,#30266,#8486,.T.) ;
#35944=EDGE_CURVE('',#30266,#30267,#8487,.T.) ;
#35945=EDGE_CURVE('',#30267,#30268,#8488,.T.) ;
#35946=EDGE_CURVE('',#30268,#30269,#8489,.T.) ;
#35947=EDGE_CURVE('',#30269,#30270,#8490,.T.) ;
#35948=EDGE_CURVE('',#30270,#30271,#8491,.T.) ;
#35949=EDGE_CURVE('',#30271,#30272,#8492,.T.) ;
#35950=EDGE_CURVE('',#30272,#30265,#8493,.T.) ;
#35951=EDGE_CURVE('',#30273,#30274,#8494,.T.) ;
#35952=EDGE_CURVE('',#30273,#30275,#25348,.T.) ;
#35953=EDGE_CURVE('',#30275,#30276,#8495,.T.) ;
#35954=EDGE_CURVE('',#30276,#30277,#25349,.T.) ;
#35955=EDGE_CURVE('',#30277,#30278,#8496,.T.) ;
#35956=EDGE_CURVE('',#30278,#30279,#25350,.T.) ;
#35957=EDGE_CURVE('',#30279,#30280,#8497,.T.) ;
#35958=EDGE_CURVE('',#30280,#30274,#25351,.T.) ;
#35959=EDGE_CURVE('',#30281,#30282,#25352,.T.) ;
#35960=EDGE_CURVE('',#30281,#30142,#8498,.T.) ;
#35961=EDGE_CURVE('',#30141,#30283,#8499,.T.) ;
#35962=EDGE_CURVE('',#30283,#30284,#25353,.T.) ;
#35963=EDGE_CURVE('',#30284,#30285,#8500,.T.) ;
#35964=EDGE_CURVE('',#30285,#30282,#25354,.T.) ;
#35965=EDGE_CURVE('',#30139,#30286,#8501,.T.) ;
#35966=EDGE_CURVE('',#30286,#30287,#8502,.T.) ;
#35967=EDGE_CURVE('',#30287,#30140,#8503,.T.) ;
#35968=EDGE_CURVE('',#30288,#30289,#8504,.T.) ;
#35969=EDGE_CURVE('',#30289,#30082,#8505,.T.) ;
#35970=EDGE_CURVE('',#30084,#30288,#8506,.T.) ;
#35971=EDGE_CURVE('',#30290,#30291,#25355,.T.) ;
#35972=EDGE_CURVE('',#30291,#30292,#8507,.T.) ;
#35973=EDGE_CURVE('',#30292,#30293,#25356,.T.) ;
#35974=EDGE_CURVE('',#30293,#30290,#8508,.T.) ;
#35975=EDGE_CURVE('',#30294,#30295,#25357,.T.) ;
#35976=EDGE_CURVE('',#30295,#30296,#8509,.T.) ;
#35977=EDGE_CURVE('',#30296,#30297,#25358,.T.) ;
#35978=EDGE_CURVE('',#30297,#30294,#8510,.T.) ;
#35979=EDGE_CURVE('',#30076,#30298,#8511,.T.) ;
#35980=EDGE_CURVE('',#30298,#30299,#8512,.T.) ;
#35981=EDGE_CURVE('',#30299,#30078,#8513,.T.) ;
#35982=EDGE_CURVE('',#30300,#30301,#8514,.T.) ;
#35983=EDGE_CURVE('',#30301,#30168,#8515,.T.) ;
#35984=EDGE_CURVE('',#30167,#30300,#8516,.T.) ;
#35985=EDGE_CURVE('',#30302,#30303,#25359,.T.) ;
#35986=EDGE_CURVE('',#30303,#30166,#8517,.T.) ;
#35987=EDGE_CURVE('',#30165,#30304,#8518,.T.) ;
#35988=EDGE_CURVE('',#30305,#30304,#25360,.T.) ;
#35989=EDGE_CURVE('',#30305,#30306,#25361,.T.) ;
#35990=EDGE_CURVE('',#30306,#30302,#8519,.T.) ;
#35991=EDGE_CURVE('',#30307,#30308,#25362,.T.) ;
#35992=EDGE_CURVE('',#30308,#30134,#8520,.T.) ;
#35993=EDGE_CURVE('',#30133,#30309,#8521,.T.) ;
#35994=EDGE_CURVE('',#30309,#30307,#8522,.T.) ;
#35995=EDGE_CURVE('',#30310,#30311,#8523,.T.) ;
#35996=EDGE_CURVE('',#30311,#30136,#8524,.T.) ;
#35997=EDGE_CURVE('',#30135,#30310,#8525,.T.) ;
#35998=EDGE_CURVE('',#30312,#30313,#25363,.T.) ;
#35999=EDGE_CURVE('',#30313,#30314,#8526,.T.) ;
#36000=EDGE_CURVE('',#30314,#30315,#25364,.T.) ;
#36001=EDGE_CURVE('',#30315,#30312,#8527,.T.) ;
#36002=EDGE_CURVE('',#30316,#30317,#8528,.T.) ;
#36003=EDGE_CURVE('',#30317,#30318,#8529,.T.) ;
#36004=EDGE_CURVE('',#30318,#30319,#8530,.T.) ;
#36005=EDGE_CURVE('',#30319,#30316,#8531,.T.) ;
#36006=EDGE_CURVE('',#30320,#30321,#25365,.T.) ;
#36007=EDGE_CURVE('',#30321,#30322,#8532,.T.) ;
#36008=EDGE_CURVE('',#30322,#30323,#25366,.T.) ;
#36009=EDGE_CURVE('',#30323,#30320,#8533,.T.) ;
#36010=EDGE_CURVE('',#30171,#30324,#8534,.T.) ;
#36011=EDGE_CURVE('',#30324,#30325,#8535,.T.) ;
#36012=EDGE_CURVE('',#30325,#30172,#8536,.T.) ;
#36013=EDGE_CURVE('',#30326,#30327,#8537,.T.) ;
#36014=EDGE_CURVE('',#30327,#30328,#8538,.T.) ;
#36015=EDGE_CURVE('',#30328,#30329,#8539,.T.) ;
#36016=EDGE_CURVE('',#30329,#30326,#8540,.T.) ;
#36017=EDGE_CURVE('',#30330,#30331,#8541,.T.) ;
#36018=EDGE_CURVE('',#30331,#30174,#8542,.T.) ;
#36019=EDGE_CURVE('',#30173,#30332,#8543,.T.) ;
#36020=EDGE_CURVE('',#30332,#30330,#25367,.T.) ;
#36021=EDGE_CURVE('',#30333,#30334,#8544,.T.) ;
#36022=EDGE_CURVE('',#30334,#30335,#8545,.T.) ;
#36023=EDGE_CURVE('',#30335,#30336,#8546,.T.) ;
#36024=EDGE_CURVE('',#30336,#30333,#8547,.T.) ;
#36025=EDGE_CURVE('',#30337,#30338,#4854,.T.) ;
#36026=EDGE_CURVE('',#30338,#30067,#8548,.T.) ;
#36027=EDGE_CURVE('',#30071,#30339,#8549,.T.) ;
#36028=EDGE_CURVE('',#30339,#30340,#4855,.T.) ;
#36029=EDGE_CURVE('',#30340,#30341,#8550,.T.) ;
#36030=EDGE_CURVE('',#30341,#30342,#4856,.T.) ;
#36031=EDGE_CURVE('',#30342,#30337,#8551,.T.) ;
#36032=EDGE_CURVE('',#30343,#30344,#8552,.T.) ;
#36033=EDGE_CURVE('',#30344,#30070,#8553,.T.) ;
#36034=EDGE_CURVE('',#30070,#30345,#8554,.T.) ;
#36035=EDGE_CURVE('',#30345,#30343,#8555,.T.) ;
#36036=EDGE_CURVE('',#30346,#30347,#8556,.T.) ;
#36037=EDGE_CURVE('',#30347,#30348,#8557,.T.) ;
#36038=EDGE_CURVE('',#30348,#30349,#8558,.T.) ;
#36039=EDGE_CURVE('',#30349,#30346,#8559,.T.) ;
#36040=EDGE_CURVE('',#30350,#30351,#8560,.T.) ;
#36041=EDGE_CURVE('',#30351,#30352,#8561,.T.) ;
#36042=EDGE_CURVE('',#30352,#30353,#8562,.T.) ;
#36043=EDGE_CURVE('',#30353,#30350,#8563,.T.) ;
#36044=EDGE_CURVE('',#30354,#30355,#8564,.T.) ;
#36045=EDGE_CURVE('',#30355,#30356,#8565,.T.) ;
#36046=EDGE_CURVE('',#30356,#30357,#8566,.T.) ;
#36047=EDGE_CURVE('',#30357,#30354,#8567,.T.) ;
#36048=EDGE_CURVE('',#30274,#30358,#8568,.T.) ;
#36049=EDGE_CURVE('',#30358,#30359,#8569,.T.) ;
#36050=EDGE_CURVE('',#30359,#30273,#8570,.T.) ;
#36051=EDGE_CURVE('',#30277,#30360,#8571,.T.) ;
#36052=EDGE_CURVE('',#30360,#30361,#8572,.T.) ;
#36053=EDGE_CURVE('',#30361,#30278,#8573,.T.) ;
#36054=EDGE_CURVE('',#30279,#30362,#8574,.T.) ;
#36055=EDGE_CURVE('',#30362,#30363,#8575,.T.) ;
#36056=EDGE_CURVE('',#30363,#30280,#8576,.T.) ;
#36057=EDGE_CURVE('',#30275,#30364,#8577,.T.) ;
#36058=EDGE_CURVE('',#30364,#30365,#8578,.T.) ;
#36059=EDGE_CURVE('',#30365,#30276,#8579,.T.) ;
#36060=EDGE_CURVE('',#30366,#30367,#8580,.T.) ;
#36061=EDGE_CURVE('',#30367,#30368,#8581,.T.) ;
#36062=EDGE_CURVE('',#30368,#30369,#8582,.T.) ;
#36063=EDGE_CURVE('',#30369,#30370,#25368,.T.) ;
#36064=EDGE_CURVE('',#30370,#30371,#8583,.T.) ;
#36065=EDGE_CURVE('',#30371,#30366,#25369,.T.) ;
#36066=EDGE_CURVE('',#30372,#30373,#8584,.T.) ;
#36067=EDGE_CURVE('',#30373,#30374,#8585,.T.) ;
#36068=EDGE_CURVE('',#30374,#30375,#8586,.T.) ;
#36069=EDGE_CURVE('',#30375,#30376,#25370,.T.) ;
#36070=EDGE_CURVE('',#30376,#30377,#8587,.T.) ;
#36071=EDGE_CURVE('',#30377,#30372,#25371,.T.) ;
#36072=EDGE_CURVE('',#30378,#30379,#8588,.T.) ;
#36073=EDGE_CURVE('',#30378,#30097,#25372,.T.) ;
#36074=EDGE_CURVE('',#30096,#30379,#25373,.T.) ;
#36075=EDGE_CURVE('',#30379,#30380,#8589,.T.) ;
#36076=EDGE_CURVE('',#30380,#30381,#8590,.T.) ;
#36077=EDGE_CURVE('',#30381,#30378,#8591,.T.) ;
#36078=EDGE_CURVE('',#30382,#30383,#8592,.T.) ;
#36079=EDGE_CURVE('',#30383,#30384,#8593,.T.) ;
#36080=EDGE_CURVE('',#30384,#30385,#8594,.T.) ;
#36081=EDGE_CURVE('',#30385,#30382,#8595,.T.) ;
#36082=EDGE_CURVE('',#30386,#30387,#8596,.T.) ;
#36083=EDGE_CURVE('',#30387,#30388,#8597,.T.) ;
#36084=EDGE_CURVE('',#30388,#30389,#8598,.T.) ;
#36085=EDGE_CURVE('',#30389,#30386,#8599,.T.) ;
#36086=EDGE_CURVE('',#30390,#30391,#8600,.T.) ;
#36087=EDGE_CURVE('',#30391,#30392,#8601,.T.) ;
#36088=EDGE_CURVE('',#30392,#30393,#8602,.T.) ;
#36089=EDGE_CURVE('',#30393,#30390,#8603,.T.) ;
#36090=EDGE_CURVE('',#30394,#30395,#8604,.T.) ;
#36091=EDGE_CURVE('',#30395,#30396,#8605,.T.) ;
#36092=EDGE_CURVE('',#30396,#30397,#8606,.T.) ;
#36093=EDGE_CURVE('',#30394,#30397,#8607,.T.) ;
#36094=EDGE_CURVE('',#30264,#30394,#25374,.T.) ;
#36095=EDGE_CURVE('',#30397,#30259,#25375,.T.) ;
#36096=EDGE_CURVE('',#30398,#30399,#8608,.T.) ;
#36097=EDGE_CURVE('',#30399,#30400,#8609,.T.) ;
#36098=EDGE_CURVE('',#30400,#30401,#8610,.T.) ;
#36099=EDGE_CURVE('',#30401,#30398,#8611,.T.) ;
#36100=EDGE_CURVE('',#30402,#30403,#8612,.T.) ;
#36101=EDGE_CURVE('',#30403,#30404,#8613,.T.) ;
#36102=EDGE_CURVE('',#30404,#30405,#8614,.T.) ;
#36103=EDGE_CURVE('',#30405,#30402,#8615,.T.) ;
#36104=EDGE_CURVE('',#30406,#30407,#8616,.T.) ;
#36105=EDGE_CURVE('',#30407,#30408,#8617,.T.) ;
#36106=EDGE_CURVE('',#30408,#30409,#8618,.T.) ;
#36107=EDGE_CURVE('',#30409,#30406,#8619,.T.) ;
#36108=EDGE_CURVE('',#30410,#30411,#8620,.T.) ;
#36109=EDGE_CURVE('',#30411,#30412,#8621,.T.) ;
#36110=EDGE_CURVE('',#30412,#30413,#8622,.T.) ;
#36111=EDGE_CURVE('',#30413,#30410,#8623,.T.) ;
#36112=EDGE_CURVE('',#30163,#30414,#8624,.T.) ;
#36113=EDGE_CURVE('',#30414,#30415,#25376,.T.) ;
#36114=EDGE_CURVE('',#30415,#30164,#8625,.T.) ;
#36115=EDGE_CURVE('',#30416,#30417,#25377,.T.) ;
#36116=EDGE_CURVE('',#30417,#30088,#25378,.T.) ;
#36117=EDGE_CURVE('',#30087,#30416,#25379,.T.) ;
#36118=EDGE_CURVE('',#30143,#30418,#8626,.T.) ;
#36119=EDGE_CURVE('',#30418,#30419,#25380,.T.) ;
#36120=EDGE_CURVE('',#30419,#30144,#8627,.T.) ;
#36121=EDGE_CURVE('',#30332,#30325,#25381,.T.) ;
#36122=EDGE_CURVE('',#30332,#30321,#25382,.T.) ;
#36123=EDGE_CURVE('',#30321,#30325,#25383,.T.) ;
#36124=EDGE_CURVE('',#30324,#30214,#25384,.T.) ;
#36125=EDGE_CURVE('',#30322,#30324,#25385,.T.) ;
#36126=EDGE_CURVE('',#30330,#30320,#25386,.T.) ;
#36127=EDGE_CURVE('',#30322,#30213,#25387,.T.) ;
#36128=EDGE_CURVE('',#30330,#30329,#25388,.T.) ;
#36129=EDGE_CURVE('',#30329,#30320,#25389,.T.) ;
#36130=EDGE_CURVE('',#30310,#30308,#25390,.T.) ;
#36131=EDGE_CURVE('',#30311,#30315,#25391,.T.) ;
#36132=EDGE_CURVE('',#30312,#30310,#25392,.T.) ;
#36133=EDGE_CURVE('',#30205,#30311,#25393,.T.) ;
#36134=EDGE_CURVE('',#30323,#30212,#25394,.T.) ;
#36135=EDGE_CURVE('',#30326,#30323,#25395,.T.) ;
#36136=EDGE_CURVE('',#30331,#30328,#25396,.T.) ;
#36137=EDGE_CURVE('',#30197,#30331,#25397,.T.) ;
#36138=EDGE_CURVE('',#30312,#30308,#25398,.T.) ;
#36139=EDGE_CURVE('',#30206,#30315,#25399,.T.) ;
#36140=EDGE_CURVE('',#30326,#30211,#25400,.T.) ;
#36141=EDGE_CURVE('',#30197,#30328,#25401,.T.) ;
#36142=EDGE_CURVE('',#30313,#30307,#25402,.T.) ;
#36143=EDGE_CURVE('',#30314,#30319,#25403,.T.) ;
#36144=EDGE_CURVE('',#30316,#30313,#25404,.T.) ;
#36145=EDGE_CURVE('',#30207,#30314,#25405,.T.) ;
#36146=EDGE_CURVE('',#30327,#30210,#25406,.T.) ;
#36147=EDGE_CURVE('',#30198,#30327,#25407,.T.) ;
#36148=EDGE_CURVE('',#30316,#30307,#25408,.T.) ;
#36149=EDGE_CURVE('',#30208,#30319,#25409,.T.) ;
#36150=EDGE_CURVE('',#30199,#30210,#25410,.T.) ;
#36151=EDGE_CURVE('',#30309,#30202,#25411,.T.) ;
#36152=EDGE_CURVE('',#30317,#30309,#25412,.T.) ;
#36153=EDGE_CURVE('',#30209,#30318,#25413,.T.) ;
#36154=EDGE_CURVE('',#30200,#30209,#25414,.T.) ;
#36155=EDGE_CURVE('',#30317,#30202,#25415,.T.) ;
#36156=EDGE_CURVE('',#30201,#30318,#25416,.T.) ;
#36157=EDGE_CURVE('',#30265,#30246,#25417,.T.) ;
#36158=EDGE_CURVE('',#30254,#30265,#25418,.T.) ;
#36159=EDGE_CURVE('',#30246,#30254,#25419,.T.) ;
#36160=EDGE_CURVE('',#30272,#30420,#93,.T.) ;
#36161=EDGE_CURVE('',#30420,#30251,#4857,.T.) ;
#36162=EDGE_CURVE('',#30253,#30421,#4858,.T.) ;
#36163=EDGE_CURVE('',#30421,#30239,#94,.T.) ;
#36164=EDGE_CURVE('',#30266,#30245,#25420,.T.) ;
#36165=EDGE_CURVE('',#30261,#30422,#4859,.T.) ;
#36166=EDGE_CURVE('',#30422,#30272,#95,.T.) ;
#36167=EDGE_CURVE('',#30271,#30423,#96,.T.) ;
#36168=EDGE_CURVE('',#30423,#30262,#4860,.T.) ;
#36169=EDGE_CURVE('',#30239,#30424,#97,.T.) ;
#36170=EDGE_CURVE('',#30424,#30256,#4861,.T.) ;
#36171=EDGE_CURVE('',#30255,#30425,#4862,.T.) ;
#36172=EDGE_CURVE('',#30425,#30240,#98,.T.) ;
#36173=EDGE_CURVE('',#30266,#30237,#25421,.T.) ;
#36174=EDGE_CURVE('',#30236,#30245,#25422,.T.) ;
#36175=EDGE_CURVE('',#30426,#30237,#8628,.T.) ;
#36176=EDGE_CURVE('',#30267,#30426,#25423,.T.) ;
#36177=EDGE_CURVE('',#30427,#30426,#25424,.T.) ;
#36178=EDGE_CURVE('',#30267,#30427,#25425,.T.) ;
#36179=EDGE_CURVE('',#30250,#30428,#4863,.T.) ;
#36180=EDGE_CURVE('',#30428,#30271,#99,.T.) ;
#36181=EDGE_CURVE('',#30247,#30270,#25426,.T.) ;
#36182=EDGE_CURVE('',#30240,#30429,#100,.T.) ;
#36183=EDGE_CURVE('',#30429,#30248,#4864,.T.) ;
#36184=EDGE_CURVE('',#30241,#30247,#25427,.T.) ;
#36185=EDGE_CURVE('',#30430,#30244,#25428,.T.) ;
#36186=EDGE_CURVE('',#30236,#30430,#8629,.T.) ;
#36187=EDGE_CURVE('',#30225,#30238,#4865,.T.) ;
#36188=EDGE_CURVE('',#30426,#30223,#25429,.T.) ;
#36189=EDGE_CURVE('',#30427,#30224,#25430,.T.) ;
#36190=EDGE_CURVE('',#30431,#30427,#8630,.T.) ;
#36191=EDGE_CURVE('',#30268,#30431,#25431,.T.) ;
#36192=EDGE_CURVE('',#30241,#30270,#25432,.T.) ;
#36193=EDGE_CURVE('',#30430,#30432,#25433,.T.) ;
#36194=EDGE_CURVE('',#30432,#30244,#25434,.T.) ;
#36195=EDGE_CURVE('',#30231,#30430,#25435,.T.) ;
#36196=EDGE_CURVE('',#30431,#30228,#25436,.T.) ;
#36197=EDGE_CURVE('',#30433,#30431,#25437,.T.) ;
#36198=EDGE_CURVE('',#30268,#30433,#25438,.T.) ;
#36199=EDGE_CURVE('',#30242,#30269,#25439,.T.) ;
#36200=EDGE_CURVE('',#30434,#30243,#25440,.T.) ;
#36201=EDGE_CURVE('',#30432,#30434,#8631,.T.) ;
#36202=EDGE_CURVE('',#30232,#30432,#25441,.T.) ;
#36203=EDGE_CURVE('',#30433,#30227,#25442,.T.) ;
#36204=EDGE_CURVE('',#30233,#30433,#8632,.T.) ;
#36205=EDGE_CURVE('',#30269,#30233,#25443,.T.) ;
#36206=EDGE_CURVE('',#30242,#30235,#25444,.T.) ;
#36207=EDGE_CURVE('',#30434,#30435,#25445,.T.) ;
#36208=EDGE_CURVE('',#30435,#30243,#25446,.T.) ;
#36209=EDGE_CURVE('',#30230,#30434,#25447,.T.) ;
#36210=EDGE_CURVE('',#30234,#30226,#4866,.T.) ;
#36211=EDGE_CURVE('',#30435,#30235,#8633,.T.) ;
#36212=EDGE_CURVE('',#30229,#30435,#25448,.T.) ;
#36213=EDGE_CURVE('',#30283,#30287,#25449,.T.) ;
#36214=EDGE_CURVE('',#30283,#30291,#25450,.T.) ;
#36215=EDGE_CURVE('',#30291,#30287,#25451,.T.) ;
#36216=EDGE_CURVE('',#30286,#30203,#25452,.T.) ;
#36217=EDGE_CURVE('',#30292,#30286,#25453,.T.) ;
#36218=EDGE_CURVE('',#30284,#30290,#25454,.T.) ;
#36219=EDGE_CURVE('',#30115,#30281,#25455,.T.) ;
#36220=EDGE_CURVE('',#30086,#30116,#25456,.T.) ;
#36221=EDGE_CURVE('',#30089,#30115,#25457,.T.) ;
#36222=EDGE_CURVE('',#30292,#30204,#25458,.T.) ;
#36223=EDGE_CURVE('',#30284,#30288,#25459,.T.) ;
#36224=EDGE_CURVE('',#30288,#30290,#25460,.T.) ;
#36225=EDGE_CURVE('',#30089,#30282,#25461,.T.) ;
#36226=EDGE_CURVE('',#30293,#30222,#25462,.T.) ;
#36227=EDGE_CURVE('',#30289,#30293,#25463,.T.) ;
#36228=EDGE_CURVE('',#30285,#30084,#25464,.T.) ;
#36229=EDGE_CURVE('',#30083,#30285,#25465,.T.) ;
#36230=EDGE_CURVE('',#30121,#30085,#25466,.T.) ;
#36231=EDGE_CURVE('',#30122,#30092,#25467,.T.) ;
#36232=EDGE_CURVE('',#30304,#30122,#25468,.T.) ;
#36233=EDGE_CURVE('',#30300,#30303,#25469,.T.) ;
#36234=EDGE_CURVE('',#30289,#30221,#25470,.T.) ;
#36235=EDGE_CURVE('',#30305,#30092,#25471,.T.) ;
#36236=EDGE_CURVE('',#30300,#30294,#25472,.T.) ;
#36237=EDGE_CURVE('',#30294,#30303,#25473,.T.) ;
#36238=EDGE_CURVE('',#30082,#30220,#101,.T.) ;
#36239=EDGE_CURVE('',#30306,#30080,#25474,.T.) ;
#36240=EDGE_CURVE('',#30302,#30299,#25475,.T.) ;
#36241=EDGE_CURVE('',#30078,#30306,#25476,.T.) ;
#36242=EDGE_CURVE('',#30295,#30302,#25477,.T.) ;
#36243=EDGE_CURVE('',#30301,#30297,#25478,.T.) ;
#36244=EDGE_CURVE('',#30215,#30301,#25479,.T.) ;
#36245=EDGE_CURVE('',#30090,#30220,#25480,.T.) ;
#36246=EDGE_CURVE('',#30436,#30079,#25481,.T.) ;
#36247=EDGE_CURVE('',#30295,#30299,#25482,.T.) ;
#36248=EDGE_CURVE('',#30216,#30297,#25483,.T.) ;
#36249=EDGE_CURVE('',#30091,#30219,#25484,.T.) ;
#36250=EDGE_CURVE('',#30296,#30298,#25485,.T.) ;
#36251=EDGE_CURVE('',#30217,#30296,#25486,.T.) ;
#36252=EDGE_CURVE('',#30076,#30219,#102,.T.) ;
#36253=EDGE_CURVE('',#30218,#30298,#25487,.T.) ;
#36254=EDGE_CURVE('',#30095,#30376,#103,.T.) ;
#36255=EDGE_CURVE('',#30379,#30375,#25488,.T.) ;
#36256=EDGE_CURVE('',#30374,#30380,#25489,.T.) ;
#36257=EDGE_CURVE('',#30377,#30260,#104,.T.) ;
#36258=EDGE_CURVE('',#30372,#30397,#25490,.T.) ;
#36259=EDGE_CURVE('',#30384,#30411,#25491,.T.) ;
#36260=EDGE_CURVE('',#30385,#30410,#25492,.T.) ;
#36261=EDGE_CURVE('',#30371,#30098,#105,.T.) ;
#36262=EDGE_CURVE('',#30366,#30378,#25493,.T.) ;
#36263=EDGE_CURVE('',#30396,#30373,#25494,.T.) ;
#36264=EDGE_CURVE('',#30385,#30389,#25495,.T.) ;
#36265=EDGE_CURVE('',#30389,#30410,#25496,.T.) ;
#36266=EDGE_CURVE('',#30381,#30367,#25497,.T.) ;
#36267=EDGE_CURVE('',#30412,#30391,#25498,.T.) ;
#36268=EDGE_CURVE('',#30413,#30390,#25499,.T.) ;
#36269=EDGE_CURVE('',#30386,#30413,#25500,.T.) ;
#36270=EDGE_CURVE('',#30382,#30388,#25501,.T.) ;
#36271=EDGE_CURVE('',#30408,#30383,#25502,.T.) ;
#36272=EDGE_CURVE('',#30409,#30382,#25503,.T.) ;
#36273=EDGE_CURVE('',#30386,#30390,#25504,.T.) ;
#36274=EDGE_CURVE('',#30409,#30388,#25505,.T.) ;
#36275=EDGE_CURVE('',#30387,#30393,#25506,.T.) ;
#36276=EDGE_CURVE('',#30406,#30387,#25507,.T.) ;
#36277=EDGE_CURVE('',#30406,#30393,#25508,.T.) ;
#36278=EDGE_CURVE('',#30392,#30407,#25509,.T.) ;
#36279=EDGE_CURVE('',#30368,#30395,#25510,.T.) ;
#36280=EDGE_CURVE('',#30369,#30394,#25511,.T.) ;
#36281=EDGE_CURVE('',#30263,#30370,#106,.T.) ;
#36282=EDGE_CURVE('',#30361,#30362,#25512,.T.) ;
#36283=EDGE_CURVE('',#30365,#30360,#25513,.T.) ;
#36284=EDGE_CURVE('',#30348,#30399,#25514,.T.) ;
#36285=EDGE_CURVE('',#30349,#30398,#25515,.T.) ;
#36286=EDGE_CURVE('',#30400,#30355,#25516,.T.) ;
#36287=EDGE_CURVE('',#30401,#30354,#25517,.T.) ;
#36288=EDGE_CURVE('',#30398,#30353,#25518,.T.) ;
#36289=EDGE_CURVE('',#30350,#30401,#25519,.T.) ;
#36290=EDGE_CURVE('',#30349,#30353,#25520,.T.) ;
#36291=EDGE_CURVE('',#30363,#30358,#25521,.T.) ;
#36292=EDGE_CURVE('',#30359,#30364,#25522,.T.) ;
#36293=EDGE_CURVE('',#30350,#30354,#25523,.T.) ;
#36294=EDGE_CURVE('',#30346,#30352,#25524,.T.) ;
#36295=EDGE_CURVE('',#30404,#30347,#25525,.T.) ;
#36296=EDGE_CURVE('',#30405,#30346,#25526,.T.) ;
#36297=EDGE_CURVE('',#30356,#30403,#25527,.T.) ;
#36298=EDGE_CURVE('',#30357,#30402,#25528,.T.) ;
#36299=EDGE_CURVE('',#30351,#30357,#25529,.T.) ;
#36300=EDGE_CURVE('',#30405,#30352,#25530,.T.) ;
#36301=EDGE_CURVE('',#30351,#30402,#25531,.T.) ;
#36302=EDGE_CURVE('',#30109,#30108,#25532,.T.) ;
#36303=EDGE_CURVE('',#30335,#30110,#107,.T.) ;
#36304=EDGE_CURVE('',#30336,#30109,#25533,.T.) ;
#36305=EDGE_CURVE('',#30336,#30108,#25534,.T.) ;
#36306=EDGE_CURVE('',#30107,#30104,#25535,.T.) ;
#36307=EDGE_CURVE('',#30333,#30107,#25536,.T.) ;
#36308=EDGE_CURVE('',#30333,#30104,#25537,.T.) ;
#36309=EDGE_CURVE('',#30103,#30334,#108,.T.) ;
#36310=EDGE_CURVE('',#30065,#30344,#4867,.T.) ;
#36311=EDGE_CURVE('',#30192,#30343,#25538,.T.) ;
#36312=EDGE_CURVE('',#30189,#30192,#25539,.T.) ;
#36313=EDGE_CURVE('',#30189,#30343,#25540,.T.) ;
#36314=EDGE_CURVE('',#30190,#30345,#25541,.T.) ;
#36315=EDGE_CURVE('',#30188,#30190,#25542,.T.) ;
#36316=EDGE_CURVE('',#30188,#30345,#25543,.T.) ;
#36317=EDGE_CURVE('',#30069,#30185,#4868,.T.) ;
#36318=EDGE_CURVE('',#30257,#30094,#25544,.T.) ;
#36319=EDGE_CURVE('',#30093,#30258,#25545,.T.) ;
#36320=EDGE_CURVE('',#30419,#30127,#25546,.T.) ;
#36321=EDGE_CURVE('',#30416,#30128,#25547,.T.) ;
#36322=EDGE_CURVE('',#30127,#30417,#25548,.T.) ;
#36323=EDGE_CURVE('',#30128,#30414,#25549,.T.) ;
#36324=EDGE_CURVE('',#30251,#30261,#25550,.T.) ;
#36325=EDGE_CURVE('',#30252,#30094,#25551,.T.) ;
#36326=EDGE_CURVE('',#30252,#30257,#25552,.T.) ;
#36327=EDGE_CURVE('',#30253,#30256,#25553,.T.) ;
#36328=EDGE_CURVE('',#30248,#30255,#25554,.T.) ;
#36329=EDGE_CURVE('',#30249,#30258,#25555,.T.) ;
#36330=EDGE_CURVE('',#30249,#30093,#25556,.T.) ;
#36331=EDGE_CURVE('',#30250,#30262,#25557,.T.) ;
#36332=EDGE_CURVE('',#30102,#30338,#109,.T.) ;
#36333=EDGE_CURVE('',#30334,#30337,#25558,.T.) ;
#36334=EDGE_CURVE('',#30335,#30342,#25559,.T.) ;
#36335=EDGE_CURVE('',#30437,#30341,#110,.T.) ;
#36336=EDGE_CURVE('',#30438,#30437,#111,.T.) ;
#36337=EDGE_CURVE('',#30439,#30438,#112,.T.) ;
#36338=EDGE_CURVE('',#30111,#30439,#113,.T.) ;
#36339=EDGE_CURVE('',#30193,#30112,#4869,.T.) ;
#36340=EDGE_CURVE('',#30194,#30341,#25560,.T.) ;
#36341=EDGE_CURVE('',#30068,#30186,#114,.T.) ;
#36342=EDGE_CURVE('',#30195,#30340,#25561,.T.) ;
#36343=EDGE_CURVE('',#30191,#30196,#4870,.T.) ;
#36344=EDGE_CURVE('',#30339,#30344,#25562,.T.) ;
#36345=EDGE_CURVE('',#30440,#30340,#115,.T.) ;
#36346=EDGE_CURVE('',#30441,#30440,#116,.T.) ;
#36347=EDGE_CURVE('',#30064,#30441,#117,.T.) ;
#36348=EDGE_CURVE('',#30121,#30415,#25563,.T.) ;
#36349=EDGE_CURVE('',#30087,#30415,#25564,.T.) ;
#36350=EDGE_CURVE('',#30416,#30414,#25565,.T.) ;
#36351=EDGE_CURVE('',#30384,#30380,#25566,.T.) ;
#36352=EDGE_CURVE('',#30411,#30374,#25567,.T.) ;
#36353=EDGE_CURVE('',#30381,#30383,#25568,.T.) ;
#36354=EDGE_CURVE('',#30412,#30373,#25569,.T.) ;
#36355=EDGE_CURVE('',#30367,#30408,#25570,.T.) ;
#36356=EDGE_CURVE('',#30391,#30396,#25571,.T.) ;
#36357=EDGE_CURVE('',#30368,#30407,#25572,.T.) ;
#36358=EDGE_CURVE('',#30392,#30395,#25573,.T.) ;
#36359=EDGE_CURVE('',#30348,#30362,#25574,.T.) ;
#36360=EDGE_CURVE('',#30399,#30361,#25575,.T.) ;
#36361=EDGE_CURVE('',#30363,#30347,#25576,.T.) ;
#36362=EDGE_CURVE('',#30400,#30360,#25577,.T.) ;
#36363=EDGE_CURVE('',#30358,#30404,#25578,.T.) ;
#36364=EDGE_CURVE('',#30355,#30365,#25579,.T.) ;
#36365=EDGE_CURVE('',#30359,#30403,#25580,.T.) ;
#36366=EDGE_CURVE('',#30356,#30364,#25581,.T.) ;
#36367=EDGE_CURVE('',#30418,#30116,#25582,.T.) ;
#36368=EDGE_CURVE('',#30418,#30088,#25583,.T.) ;
#36369=EDGE_CURVE('',#30419,#30417,#25584,.T.) ;
#36370=EDGE_CURVE('',#30183,#30187,#4871,.T.) ;
#36371=EDGE_CURVE('',#30184,#30067,#25585,.T.) ;
#36372=EDGE_CURVE('',#30181,#30338,#25586,.T.) ;
#36373=EDGE_CURVE('',#30182,#30101,#4872,.T.) ;
#36374=EDGE_CURVE('',#30442,#30443,#118,.T.) ;
#36375=EDGE_CURVE('',#30443,#30444,#4873,.T.) ;
#36376=EDGE_CURVE('',#30444,#30445,#25587,.T.) ;
#36377=EDGE_CURVE('',#30446,#30445,#4874,.T.) ;
#36378=EDGE_CURVE('',#30442,#30446,#119,.T.) ;
#36379=EDGE_CURVE('',#30447,#30448,#120,.T.) ;
#36380=EDGE_CURVE('',#30448,#30449,#25588,.T.) ;
#36381=EDGE_CURVE('',#30450,#30449,#4875,.T.) ;
#36382=EDGE_CURVE('',#30451,#30450,#25589,.T.) ;
#36383=EDGE_CURVE('',#30447,#30451,#4876,.T.) ;
#36384=EDGE_CURVE('',#30452,#30452,#25590,.T.) ;
#36385=EDGE_CURVE('',#30452,#30453,#25591,.T.) ;
#36386=EDGE_CURVE('',#30453,#30453,#25592,.T.) ;
#36387=EDGE_CURVE('',#30454,#30454,#25593,.T.) ;
#36388=EDGE_CURVE('',#30454,#30455,#25594,.T.) ;
#36389=EDGE_CURVE('',#30455,#30455,#25595,.T.) ;
#36390=EDGE_CURVE('',#30456,#30457,#25596,.T.) ;
#36391=EDGE_CURVE('',#30458,#30456,#8634,.T.) ;
#36392=EDGE_CURVE('',#30458,#30459,#25597,.T.) ;
#36393=EDGE_CURVE('',#30459,#30460,#25598,.T.) ;
#36394=EDGE_CURVE('',#30457,#30460,#8635,.T.) ;
#36395=EDGE_CURVE('',#30461,#30462,#25599,.T.) ;
#36396=EDGE_CURVE('',#30463,#30461,#8636,.T.) ;
#36397=EDGE_CURVE('',#30463,#30464,#25600,.T.) ;
#36398=EDGE_CURVE('',#30462,#30464,#8637,.T.) ;
#36399=EDGE_CURVE('',#30465,#30466,#25601,.T.) ;
#36400=EDGE_CURVE('',#30465,#30467,#25602,.T.) ;
#36401=EDGE_CURVE('',#30468,#30467,#25603,.T.) ;
#36402=EDGE_CURVE('',#30468,#30466,#25604,.T.) ;
#36403=EDGE_CURVE('',#30453,#30454,#8638,.T.) ;
#36404=EDGE_CURVE('',#30466,#30469,#8639,.T.) ;
#36405=EDGE_CURVE('',#30469,#30463,#25605,.T.) ;
#36406=EDGE_CURVE('',#30470,#30461,#121,.T.) ;
#36407=EDGE_CURVE('',#30470,#30471,#25606,.T.) ;
#36408=EDGE_CURVE('',#30457,#30471,#122,.T.) ;
#36409=EDGE_CURVE('',#30460,#30472,#25607,.T.) ;
#36410=EDGE_CURVE('',#30472,#30465,#8640,.T.) ;
#36411=EDGE_CURVE('',#30473,#30474,#8641,.T.) ;
#36412=EDGE_CURVE('',#30474,#30475,#8642,.T.) ;
#36413=EDGE_CURVE('',#30475,#30476,#123,.T.) ;
#36414=EDGE_CURVE('',#30476,#30477,#8643,.T.) ;
#36415=EDGE_CURVE('',#30477,#30478,#4877,.T.) ;
#36416=EDGE_CURVE('',#30478,#30473,#8644,.T.) ;
#36417=EDGE_CURVE('',#30479,#30480,#8645,.T.) ;
#36418=EDGE_CURVE('',#30480,#30481,#8646,.T.) ;
#36419=EDGE_CURVE('',#30481,#30482,#124,.T.) ;
#36420=EDGE_CURVE('',#30482,#30483,#125,.T.) ;
#36421=EDGE_CURVE('',#30483,#30484,#8647,.T.) ;
#36422=EDGE_CURVE('',#30484,#30479,#8648,.T.) ;
#36423=EDGE_CURVE('',#30485,#30486,#8649,.T.) ;
#36424=EDGE_CURVE('',#30486,#30487,#8650,.T.) ;
#36425=EDGE_CURVE('',#30487,#30488,#8651,.T.) ;
#36426=EDGE_CURVE('',#30488,#30485,#8652,.T.) ;
#36427=EDGE_CURVE('',#30489,#30490,#8653,.T.) ;
#36428=EDGE_CURVE('',#30490,#30491,#126,.T.) ;
#36429=EDGE_CURVE('',#30491,#30492,#127,.T.) ;
#36430=EDGE_CURVE('',#30492,#30493,#8654,.T.) ;
#36431=EDGE_CURVE('',#30493,#30494,#8655,.T.) ;
#36432=EDGE_CURVE('',#30494,#30489,#8656,.T.) ;
#36433=EDGE_CURVE('',#30495,#30496,#8657,.T.) ;
#36434=EDGE_CURVE('',#30496,#30497,#8658,.T.) ;
#36435=EDGE_CURVE('',#30497,#30498,#8659,.T.) ;
#36436=EDGE_CURVE('',#30498,#30495,#8660,.T.) ;
#36437=EDGE_CURVE('',#30499,#30500,#8661,.T.) ;
#36438=EDGE_CURVE('',#30499,#30501,#8662,.T.) ;
#36439=EDGE_CURVE('',#30501,#30502,#8663,.T.) ;
#36440=EDGE_CURVE('',#30502,#30500,#8664,.T.) ;
#36441=EDGE_CURVE('',#30503,#30504,#8665,.T.) ;
#36442=EDGE_CURVE('',#30503,#30505,#8666,.T.) ;
#36443=EDGE_CURVE('',#30505,#30506,#8667,.T.) ;
#36444=EDGE_CURVE('',#30506,#30507,#8668,.T.) ;
#36445=EDGE_CURVE('',#30507,#30508,#25608,.T.) ;
#36446=EDGE_CURVE('',#30508,#30504,#8669,.T.) ;
#36447=EDGE_CURVE('',#30509,#30510,#8670,.T.) ;
#36448=EDGE_CURVE('',#30509,#30480,#25609,.T.) ;
#36449=EDGE_CURVE('',#30479,#30486,#25610,.T.) ;
#36450=EDGE_CURVE('',#30485,#30494,#25611,.T.) ;
#36451=EDGE_CURVE('',#30493,#30511,#25612,.T.) ;
#36452=EDGE_CURVE('',#30512,#30511,#8671,.T.) ;
#36453=EDGE_CURVE('',#30512,#30513,#25613,.T.) ;
#36454=EDGE_CURVE('',#30514,#30513,#8672,.T.) ;
#36455=EDGE_CURVE('',#30514,#30515,#25614,.T.) ;
#36456=EDGE_CURVE('',#30515,#30516,#8673,.T.) ;
#36457=EDGE_CURVE('',#30516,#30517,#25615,.T.) ;
#36458=EDGE_CURVE('',#30518,#30517,#8674,.T.) ;
#36459=EDGE_CURVE('',#30518,#30519,#25616,.T.) ;
#36460=EDGE_CURVE('',#30519,#30520,#8675,.T.) ;
#36461=EDGE_CURVE('',#30520,#30521,#25617,.T.) ;
#36462=EDGE_CURVE('',#30522,#30521,#8676,.T.) ;
#36463=EDGE_CURVE('',#30522,#30498,#25618,.T.) ;
#36464=EDGE_CURVE('',#30497,#30523,#25619,.T.) ;
#36465=EDGE_CURVE('',#30523,#30524,#8677,.T.) ;
#36466=EDGE_CURVE('',#30524,#30506,#25620,.T.) ;
#36467=EDGE_CURVE('',#30505,#30525,#25621,.T.) ;
#36468=EDGE_CURVE('',#30526,#30525,#8678,.T.) ;
#36469=EDGE_CURVE('',#30527,#30526,#8679,.T.) ;
#36470=EDGE_CURVE('',#30527,#30528,#25622,.T.) ;
#36471=EDGE_CURVE('',#30529,#30528,#8680,.T.) ;
#36472=EDGE_CURVE('',#30529,#30530,#25623,.T.) ;
#36473=EDGE_CURVE('',#30531,#30530,#8681,.T.) ;
#36474=EDGE_CURVE('',#30531,#30510,#25624,.T.) ;
#36475=EDGE_CURVE('',#30532,#30533,#8682,.T.) ;
#36476=EDGE_CURVE('',#30533,#30534,#25625,.T.) ;
#36477=EDGE_CURVE('',#30534,#30535,#8683,.T.) ;
#36478=EDGE_CURVE('',#30535,#30536,#25626,.T.) ;
#36479=EDGE_CURVE('',#30536,#30537,#8684,.T.) ;
#36480=EDGE_CURVE('',#30537,#30538,#25627,.T.) ;
#36481=EDGE_CURVE('',#30538,#30539,#8685,.T.) ;
#36482=EDGE_CURVE('',#30539,#30540,#25628,.T.) ;
#36483=EDGE_CURVE('',#30540,#30541,#8686,.T.) ;
#36484=EDGE_CURVE('',#30541,#30542,#8687,.T.) ;
#36485=EDGE_CURVE('',#30542,#30503,#25629,.T.) ;
#36486=EDGE_CURVE('',#30504,#30543,#25630,.T.) ;
#36487=EDGE_CURVE('',#30543,#30544,#8688,.T.) ;
#36488=EDGE_CURVE('',#30544,#30499,#25631,.T.) ;
#36489=EDGE_CURVE('',#30500,#30545,#25632,.T.) ;
#36490=EDGE_CURVE('',#30546,#30545,#8689,.T.) ;
#36491=EDGE_CURVE('',#30546,#30547,#25633,.T.) ;
#36492=EDGE_CURVE('',#30548,#30547,#8690,.T.) ;
#36493=EDGE_CURVE('',#30548,#30549,#25634,.T.) ;
#36494=EDGE_CURVE('',#30549,#30550,#8691,.T.) ;
#36495=EDGE_CURVE('',#30550,#30551,#25635,.T.) ;
#36496=EDGE_CURVE('',#30552,#30551,#8692,.T.) ;
#36497=EDGE_CURVE('',#30552,#30553,#25636,.T.) ;
#36498=EDGE_CURVE('',#30554,#30553,#8693,.T.) ;
#36499=EDGE_CURVE('',#30554,#30555,#25637,.T.) ;
#36500=EDGE_CURVE('',#30555,#30556,#8694,.T.) ;
#36501=EDGE_CURVE('',#30556,#30557,#25638,.T.) ;
#36502=EDGE_CURVE('',#30557,#30558,#8695,.T.) ;
#36503=EDGE_CURVE('',#30558,#30559,#25639,.T.) ;
#36504=EDGE_CURVE('',#30559,#30560,#8696,.T.) ;
#36505=EDGE_CURVE('',#30560,#30532,#25640,.T.) ;
#36506=EDGE_CURVE('',#30528,#30539,#8697,.T.) ;
#36507=EDGE_CURVE('',#30538,#30529,#8698,.T.) ;
#36508=EDGE_CURVE('',#30530,#30537,#8699,.T.) ;
#36509=EDGE_CURVE('',#30536,#30531,#8700,.T.) ;
#36510=EDGE_CURVE('',#30561,#30562,#128,.T.) ;
#36511=EDGE_CURVE('',#30562,#30509,#8701,.T.) ;
#36512=EDGE_CURVE('',#30510,#30535,#8702,.T.) ;
#36513=EDGE_CURVE('',#30534,#30563,#8703,.T.) ;
#36514=EDGE_CURVE('',#30563,#30564,#129,.T.) ;
#36515=EDGE_CURVE('',#30564,#30561,#8704,.T.) ;
#36516=EDGE_CURVE('',#30565,#30566,#130,.T.) ;
#36517=EDGE_CURVE('',#30566,#30567,#4878,.T.) ;
#36518=EDGE_CURVE('',#30567,#30533,#8705,.T.) ;
#36519=EDGE_CURVE('',#30532,#30568,#8706,.T.) ;
#36520=EDGE_CURVE('',#30568,#30565,#8707,.T.) ;
#36521=EDGE_CURVE('',#30569,#30570,#8708,.T.) ;
#36522=EDGE_CURVE('',#30570,#30560,#8709,.T.) ;
#36523=EDGE_CURVE('',#30559,#30569,#8710,.T.) ;
#36524=EDGE_CURVE('',#30571,#30442,#131,.T.) ;
#36525=EDGE_CURVE('',#30446,#30572,#8711,.T.) ;
#36526=EDGE_CURVE('',#30572,#30558,#8712,.T.) ;
#36527=EDGE_CURVE('',#30557,#30571,#8713,.T.) ;
#36528=EDGE_CURVE('',#30511,#30573,#8714,.T.) ;
#36529=EDGE_CURVE('',#30573,#30574,#132,.T.) ;
#36530=EDGE_CURVE('',#30574,#30575,#8715,.T.) ;
#36531=EDGE_CURVE('',#30575,#30576,#133,.T.) ;
#36532=EDGE_CURVE('',#30576,#30556,#8716,.T.) ;
#36533=EDGE_CURVE('',#30555,#30577,#8717,.T.) ;
#36534=EDGE_CURVE('',#30577,#30578,#8718,.T.) ;
#36535=EDGE_CURVE('',#30579,#30578,#25641,.T.) ;
#36536=EDGE_CURVE('',#30579,#30580,#8719,.T.) ;
#36537=EDGE_CURVE('',#30581,#30580,#25642,.T.) ;
#36538=EDGE_CURVE('',#30581,#30582,#8720,.T.) ;
#36539=EDGE_CURVE('',#30582,#30512,#8721,.T.) ;
#36540=EDGE_CURVE('',#30583,#30584,#25643,.T.) ;
#36541=EDGE_CURVE('',#30583,#30518,#8722,.T.) ;
#36542=EDGE_CURVE('',#30517,#30585,#8723,.T.) ;
#36543=EDGE_CURVE('',#30586,#30585,#25644,.T.) ;
#36544=EDGE_CURVE('',#30586,#30587,#25645,.T.) ;
#36545=EDGE_CURVE('',#30588,#30587,#25646,.T.) ;
#36546=EDGE_CURVE('',#30588,#30589,#8724,.T.) ;
#36547=EDGE_CURVE('',#30589,#30590,#8725,.T.) ;
#36548=EDGE_CURVE('',#30590,#30591,#8726,.T.) ;
#36549=EDGE_CURVE('',#30592,#30591,#25647,.T.) ;
#36550=EDGE_CURVE('',#30592,#30593,#25648,.T.) ;
#36551=EDGE_CURVE('',#30594,#30593,#25649,.T.) ;
#36552=EDGE_CURVE('',#30594,#30550,#8727,.T.) ;
#36553=EDGE_CURVE('',#30549,#30595,#8728,.T.) ;
#36554=EDGE_CURVE('',#30596,#30595,#25650,.T.) ;
#36555=EDGE_CURVE('',#30596,#30597,#25651,.T.) ;
#36556=EDGE_CURVE('',#30598,#30597,#25652,.T.) ;
#36557=EDGE_CURVE('',#30598,#30599,#8729,.T.) ;
#36558=EDGE_CURVE('',#30599,#30600,#25653,.T.) ;
#36559=EDGE_CURVE('',#30600,#30601,#8730,.T.) ;
#36560=EDGE_CURVE('',#30602,#30601,#25654,.T.) ;
#36561=EDGE_CURVE('',#30602,#30584,#25655,.T.) ;
#36562=EDGE_CURVE('',#30603,#30604,#25656,.T.) ;
#36563=EDGE_CURVE('',#30603,#30605,#8731,.T.) ;
#36564=EDGE_CURVE('',#30526,#30605,#8732,.T.) ;
#36565=EDGE_CURVE('',#30525,#30542,#8733,.T.) ;
#36566=EDGE_CURVE('',#30606,#30541,#8734,.T.) ;
#36567=EDGE_CURVE('',#30606,#30607,#8735,.T.) ;
#36568=EDGE_CURVE('',#30608,#30607,#25657,.T.) ;
#36569=EDGE_CURVE('',#30608,#30604,#8736,.T.) ;
#36570=EDGE_CURVE('',#30609,#30610,#25658,.T.) ;
#36571=EDGE_CURVE('',#30609,#30606,#8737,.T.) ;
#36572=EDGE_CURVE('',#30540,#30527,#8738,.T.) ;
#36573=EDGE_CURVE('',#30605,#30611,#8739,.T.) ;
#36574=EDGE_CURVE('',#30612,#30611,#25659,.T.) ;
#36575=EDGE_CURVE('',#30612,#30610,#8740,.T.) ;
#36576=EDGE_CURVE('',#30613,#30614,#8741,.T.) ;
#36577=EDGE_CURVE('',#30614,#30615,#8742,.T.) ;
#36578=EDGE_CURVE('',#30613,#30615,#25660,.T.) ;
#36579=EDGE_CURVE('',#30616,#30617,#25661,.T.) ;
#36580=EDGE_CURVE('',#30616,#30618,#8743,.T.) ;
#36581=EDGE_CURVE('',#30618,#30617,#8744,.T.) ;
#36582=EDGE_CURVE('',#30619,#30620,#8745,.T.) ;
#36583=EDGE_CURVE('',#30620,#30621,#8746,.T.) ;
#36584=EDGE_CURVE('',#30621,#30622,#8747,.T.) ;
#36585=EDGE_CURVE('',#30622,#30623,#8748,.T.) ;
#36586=EDGE_CURVE('',#30623,#30624,#8749,.T.) ;
#36587=EDGE_CURVE('',#30624,#30625,#8750,.T.) ;
#36588=EDGE_CURVE('',#30625,#30626,#8751,.T.) ;
#36589=EDGE_CURVE('',#30626,#30619,#8752,.T.) ;
#36590=EDGE_CURVE('',#30627,#30628,#8753,.T.) ;
#36591=EDGE_CURVE('',#30628,#30629,#8754,.T.) ;
#36592=EDGE_CURVE('',#30629,#30630,#8755,.T.) ;
#36593=EDGE_CURVE('',#30630,#30627,#8756,.T.) ;
#36594=EDGE_CURVE('',#30631,#30632,#8757,.T.) ;
#36595=EDGE_CURVE('',#30632,#30633,#8758,.T.) ;
#36596=EDGE_CURVE('',#30633,#30634,#8759,.T.) ;
#36597=EDGE_CURVE('',#30634,#30631,#8760,.T.) ;
#36598=EDGE_CURVE('',#30635,#30636,#8761,.T.) ;
#36599=EDGE_CURVE('',#30636,#30637,#8762,.T.) ;
#36600=EDGE_CURVE('',#30637,#30638,#8763,.T.) ;
#36601=EDGE_CURVE('',#30638,#30635,#8764,.T.) ;
#36602=EDGE_CURVE('',#30639,#30640,#134,.T.) ;
#36603=EDGE_CURVE('',#30640,#30641,#8765,.T.) ;
#36604=EDGE_CURVE('',#30641,#30642,#8766,.T.) ;
#36605=EDGE_CURVE('',#30642,#30643,#8767,.T.) ;
#36606=EDGE_CURVE('',#30643,#30644,#135,.T.) ;
#36607=EDGE_CURVE('',#30644,#30639,#8768,.T.) ;
#36608=EDGE_CURVE('',#30645,#30646,#8769,.T.) ;
#36609=EDGE_CURVE('',#30646,#30647,#8770,.T.) ;
#36610=EDGE_CURVE('',#30647,#30648,#8771,.T.) ;
#36611=EDGE_CURVE('',#30648,#30649,#8772,.T.) ;
#36612=EDGE_CURVE('',#30649,#30650,#8773,.T.) ;
#36613=EDGE_CURVE('',#30650,#30651,#8774,.T.) ;
#36614=EDGE_CURVE('',#30651,#30652,#8775,.T.) ;
#36615=EDGE_CURVE('',#30652,#30645,#8776,.T.) ;
#36616=EDGE_CURVE('',#30653,#30654,#8777,.T.) ;
#36617=EDGE_CURVE('',#30653,#30655,#25662,.T.) ;
#36618=EDGE_CURVE('',#30655,#30656,#8778,.T.) ;
#36619=EDGE_CURVE('',#30656,#30657,#25663,.T.) ;
#36620=EDGE_CURVE('',#30657,#30658,#8779,.T.) ;
#36621=EDGE_CURVE('',#30658,#30659,#25664,.T.) ;
#36622=EDGE_CURVE('',#30659,#30660,#8780,.T.) ;
#36623=EDGE_CURVE('',#30660,#30654,#25665,.T.) ;
#36624=EDGE_CURVE('',#30661,#30662,#25666,.T.) ;
#36625=EDGE_CURVE('',#30661,#30522,#8781,.T.) ;
#36626=EDGE_CURVE('',#30521,#30663,#8782,.T.) ;
#36627=EDGE_CURVE('',#30663,#30664,#25667,.T.) ;
#36628=EDGE_CURVE('',#30664,#30665,#8783,.T.) ;
#36629=EDGE_CURVE('',#30665,#30662,#25668,.T.) ;
#36630=EDGE_CURVE('',#30519,#30666,#8784,.T.) ;
#36631=EDGE_CURVE('',#30666,#30667,#8785,.T.) ;
#36632=EDGE_CURVE('',#30667,#30520,#8786,.T.) ;
#36633=EDGE_CURVE('',#30668,#30669,#8787,.T.) ;
#36634=EDGE_CURVE('',#30669,#30462,#8788,.T.) ;
#36635=EDGE_CURVE('',#30464,#30668,#8789,.T.) ;
#36636=EDGE_CURVE('',#30670,#30671,#25669,.T.) ;
#36637=EDGE_CURVE('',#30671,#30672,#8790,.T.) ;
#36638=EDGE_CURVE('',#30672,#30673,#25670,.T.) ;
#36639=EDGE_CURVE('',#30673,#30670,#8791,.T.) ;
#36640=EDGE_CURVE('',#30674,#30675,#25671,.T.) ;
#36641=EDGE_CURVE('',#30675,#30676,#8792,.T.) ;
#36642=EDGE_CURVE('',#30676,#30677,#25672,.T.) ;
#36643=EDGE_CURVE('',#30677,#30674,#8793,.T.) ;
#36644=EDGE_CURVE('',#30456,#30678,#8794,.T.) ;
#36645=EDGE_CURVE('',#30678,#30679,#8795,.T.) ;
#36646=EDGE_CURVE('',#30679,#30458,#8796,.T.) ;
#36647=EDGE_CURVE('',#30680,#30681,#8797,.T.) ;
#36648=EDGE_CURVE('',#30681,#30548,#8798,.T.) ;
#36649=EDGE_CURVE('',#30547,#30680,#8799,.T.) ;
#36650=EDGE_CURVE('',#30682,#30683,#25673,.T.) ;
#36651=EDGE_CURVE('',#30683,#30546,#8800,.T.) ;
#36652=EDGE_CURVE('',#30545,#30684,#8801,.T.) ;
#36653=EDGE_CURVE('',#30685,#30684,#25674,.T.) ;
#36654=EDGE_CURVE('',#30685,#30686,#25675,.T.) ;
#36655=EDGE_CURVE('',#30686,#30682,#8802,.T.) ;
#36656=EDGE_CURVE('',#30687,#30688,#25676,.T.) ;
#36657=EDGE_CURVE('',#30688,#30514,#8803,.T.) ;
#36658=EDGE_CURVE('',#30513,#30689,#8804,.T.) ;
#36659=EDGE_CURVE('',#30689,#30687,#8805,.T.) ;
#36660=EDGE_CURVE('',#30690,#30691,#8806,.T.) ;
#36661=EDGE_CURVE('',#30691,#30516,#8807,.T.) ;
#36662=EDGE_CURVE('',#30515,#30690,#8808,.T.) ;
#36663=EDGE_CURVE('',#30692,#30693,#25677,.T.) ;
#36664=EDGE_CURVE('',#30693,#30694,#8809,.T.) ;
#36665=EDGE_CURVE('',#30694,#30695,#25678,.T.) ;
#36666=EDGE_CURVE('',#30695,#30692,#8810,.T.) ;
#36667=EDGE_CURVE('',#30696,#30697,#8811,.T.) ;
#36668=EDGE_CURVE('',#30697,#30698,#8812,.T.) ;
#36669=EDGE_CURVE('',#30698,#30699,#8813,.T.) ;
#36670=EDGE_CURVE('',#30699,#30696,#8814,.T.) ;
#36671=EDGE_CURVE('',#30700,#30701,#25679,.T.) ;
#36672=EDGE_CURVE('',#30701,#30702,#8815,.T.) ;
#36673=EDGE_CURVE('',#30702,#30703,#25680,.T.) ;
#36674=EDGE_CURVE('',#30703,#30700,#8816,.T.) ;
#36675=EDGE_CURVE('',#30551,#30704,#8817,.T.) ;
#36676=EDGE_CURVE('',#30704,#30705,#8818,.T.) ;
#36677=EDGE_CURVE('',#30705,#30552,#8819,.T.) ;
#36678=EDGE_CURVE('',#30706,#30707,#8820,.T.) ;
#36679=EDGE_CURVE('',#30707,#30708,#8821,.T.) ;
#36680=EDGE_CURVE('',#30708,#30709,#8822,.T.) ;
#36681=EDGE_CURVE('',#30709,#30706,#8823,.T.) ;
#36682=EDGE_CURVE('',#30710,#30711,#8824,.T.) ;
#36683=EDGE_CURVE('',#30711,#30554,#8825,.T.) ;
#36684=EDGE_CURVE('',#30553,#30712,#8826,.T.) ;
#36685=EDGE_CURVE('',#30712,#30710,#25681,.T.) ;
#36686=EDGE_CURVE('',#30713,#30714,#8827,.T.) ;
#36687=EDGE_CURVE('',#30714,#30715,#8828,.T.) ;
#36688=EDGE_CURVE('',#30715,#30716,#8829,.T.) ;
#36689=EDGE_CURVE('',#30716,#30713,#8830,.T.) ;
#36690=EDGE_CURVE('',#30717,#30718,#4879,.T.) ;
#36691=EDGE_CURVE('',#30718,#30447,#8831,.T.) ;
#36692=EDGE_CURVE('',#30451,#30719,#8832,.T.) ;
#36693=EDGE_CURVE('',#30719,#30720,#4880,.T.) ;
#36694=EDGE_CURVE('',#30720,#30721,#8833,.T.) ;
#36695=EDGE_CURVE('',#30721,#30722,#4881,.T.) ;
#36696=EDGE_CURVE('',#30722,#30717,#8834,.T.) ;
#36697=EDGE_CURVE('',#30723,#30724,#8835,.T.) ;
#36698=EDGE_CURVE('',#30724,#30450,#8836,.T.) ;
#36699=EDGE_CURVE('',#30450,#30725,#8837,.T.) ;
#36700=EDGE_CURVE('',#30725,#30723,#8838,.T.) ;
#36701=EDGE_CURVE('',#30726,#30727,#8839,.T.) ;
#36702=EDGE_CURVE('',#30727,#30728,#8840,.T.) ;
#36703=EDGE_CURVE('',#30728,#30729,#8841,.T.) ;
#36704=EDGE_CURVE('',#30729,#30726,#8842,.T.) ;
#36705=EDGE_CURVE('',#30730,#30731,#8843,.T.) ;
#36706=EDGE_CURVE('',#30731,#30732,#8844,.T.) ;
#36707=EDGE_CURVE('',#30732,#30733,#8845,.T.) ;
#36708=EDGE_CURVE('',#30733,#30730,#8846,.T.) ;
#36709=EDGE_CURVE('',#30734,#30735,#8847,.T.) ;
#36710=EDGE_CURVE('',#30735,#30736,#8848,.T.) ;
#36711=EDGE_CURVE('',#30736,#30737,#8849,.T.) ;
#36712=EDGE_CURVE('',#30737,#30734,#8850,.T.) ;
#36713=EDGE_CURVE('',#30654,#30738,#8851,.T.) ;
#36714=EDGE_CURVE('',#30738,#30739,#8852,.T.) ;
#36715=EDGE_CURVE('',#30739,#30653,#8853,.T.) ;
#36716=EDGE_CURVE('',#30657,#30740,#8854,.T.) ;
#36717=EDGE_CURVE('',#30740,#30741,#8855,.T.) ;
#36718=EDGE_CURVE('',#30741,#30658,#8856,.T.) ;
#36719=EDGE_CURVE('',#30659,#30742,#8857,.T.) ;
#36720=EDGE_CURVE('',#30742,#30743,#8858,.T.) ;
#36721=EDGE_CURVE('',#30743,#30660,#8859,.T.) ;
#36722=EDGE_CURVE('',#30655,#30744,#8860,.T.) ;
#36723=EDGE_CURVE('',#30744,#30745,#8861,.T.) ;
#36724=EDGE_CURVE('',#30745,#30656,#8862,.T.) ;
#36725=EDGE_CURVE('',#30746,#30747,#8863,.T.) ;
#36726=EDGE_CURVE('',#30747,#30748,#8864,.T.) ;
#36727=EDGE_CURVE('',#30748,#30749,#8865,.T.) ;
#36728=EDGE_CURVE('',#30749,#30750,#25682,.T.) ;
#36729=EDGE_CURVE('',#30750,#30751,#8866,.T.) ;
#36730=EDGE_CURVE('',#30751,#30746,#25683,.T.) ;
#36731=EDGE_CURVE('',#30752,#30753,#8867,.T.) ;
#36732=EDGE_CURVE('',#30753,#30754,#8868,.T.) ;
#36733=EDGE_CURVE('',#30754,#30755,#8869,.T.) ;
#36734=EDGE_CURVE('',#30755,#30756,#25684,.T.) ;
#36735=EDGE_CURVE('',#30756,#30757,#8870,.T.) ;
#36736=EDGE_CURVE('',#30757,#30752,#25685,.T.) ;
#36737=EDGE_CURVE('',#30758,#30759,#8871,.T.) ;
#36738=EDGE_CURVE('',#30758,#30477,#25686,.T.) ;
#36739=EDGE_CURVE('',#30476,#30759,#25687,.T.) ;
#36740=EDGE_CURVE('',#30759,#30760,#8872,.T.) ;
#36741=EDGE_CURVE('',#30760,#30761,#8873,.T.) ;
#36742=EDGE_CURVE('',#30761,#30758,#8874,.T.) ;
#36743=EDGE_CURVE('',#30762,#30763,#8875,.T.) ;
#36744=EDGE_CURVE('',#30763,#30764,#8876,.T.) ;
#36745=EDGE_CURVE('',#30764,#30765,#8877,.T.) ;
#36746=EDGE_CURVE('',#30765,#30762,#8878,.T.) ;
#36747=EDGE_CURVE('',#30766,#30767,#8879,.T.) ;
#36748=EDGE_CURVE('',#30767,#30768,#8880,.T.) ;
#36749=EDGE_CURVE('',#30768,#30769,#8881,.T.) ;
#36750=EDGE_CURVE('',#30769,#30766,#8882,.T.) ;
#36751=EDGE_CURVE('',#30770,#30771,#8883,.T.) ;
#36752=EDGE_CURVE('',#30771,#30772,#8884,.T.) ;
#36753=EDGE_CURVE('',#30772,#30773,#8885,.T.) ;
#36754=EDGE_CURVE('',#30773,#30770,#8886,.T.) ;
#36755=EDGE_CURVE('',#30774,#30775,#8887,.T.) ;
#36756=EDGE_CURVE('',#30775,#30776,#8888,.T.) ;
#36757=EDGE_CURVE('',#30776,#30777,#8889,.T.) ;
#36758=EDGE_CURVE('',#30774,#30777,#8890,.T.) ;
#36759=EDGE_CURVE('',#30644,#30774,#25688,.T.) ;
#36760=EDGE_CURVE('',#30777,#30639,#25689,.T.) ;
#36761=EDGE_CURVE('',#30778,#30779,#8891,.T.) ;
#36762=EDGE_CURVE('',#30779,#30780,#8892,.T.) ;
#36763=EDGE_CURVE('',#30780,#30781,#8893,.T.) ;
#36764=EDGE_CURVE('',#30781,#30778,#8894,.T.) ;
#36765=EDGE_CURVE('',#30782,#30783,#8895,.T.) ;
#36766=EDGE_CURVE('',#30783,#30784,#8896,.T.) ;
#36767=EDGE_CURVE('',#30784,#30785,#8897,.T.) ;
#36768=EDGE_CURVE('',#30785,#30782,#8898,.T.) ;
#36769=EDGE_CURVE('',#30786,#30787,#8899,.T.) ;
#36770=EDGE_CURVE('',#30787,#30788,#8900,.T.) ;
#36771=EDGE_CURVE('',#30788,#30789,#8901,.T.) ;
#36772=EDGE_CURVE('',#30789,#30786,#8902,.T.) ;
#36773=EDGE_CURVE('',#30790,#30791,#8903,.T.) ;
#36774=EDGE_CURVE('',#30791,#30792,#8904,.T.) ;
#36775=EDGE_CURVE('',#30792,#30793,#8905,.T.) ;
#36776=EDGE_CURVE('',#30793,#30790,#8906,.T.) ;
#36777=EDGE_CURVE('',#30543,#30794,#8907,.T.) ;
#36778=EDGE_CURVE('',#30794,#30795,#25690,.T.) ;
#36779=EDGE_CURVE('',#30795,#30544,#8908,.T.) ;
#36780=EDGE_CURVE('',#30796,#30797,#25691,.T.) ;
#36781=EDGE_CURVE('',#30797,#30468,#25692,.T.) ;
#36782=EDGE_CURVE('',#30467,#30796,#25693,.T.) ;
#36783=EDGE_CURVE('',#30523,#30798,#8909,.T.) ;
#36784=EDGE_CURVE('',#30798,#30799,#25694,.T.) ;
#36785=EDGE_CURVE('',#30799,#30524,#8910,.T.) ;
#36786=EDGE_CURVE('',#30712,#30705,#25695,.T.) ;
#36787=EDGE_CURVE('',#30712,#30701,#25696,.T.) ;
#36788=EDGE_CURVE('',#30701,#30705,#25697,.T.) ;
#36789=EDGE_CURVE('',#30704,#30594,#25698,.T.) ;
#36790=EDGE_CURVE('',#30702,#30704,#25699,.T.) ;
#36791=EDGE_CURVE('',#30710,#30700,#25700,.T.) ;
#36792=EDGE_CURVE('',#30702,#30593,#25701,.T.) ;
#36793=EDGE_CURVE('',#30710,#30709,#25702,.T.) ;
#36794=EDGE_CURVE('',#30709,#30700,#25703,.T.) ;
#36795=EDGE_CURVE('',#30690,#30688,#25704,.T.) ;
#36796=EDGE_CURVE('',#30691,#30695,#25705,.T.) ;
#36797=EDGE_CURVE('',#30692,#30690,#25706,.T.) ;
#36798=EDGE_CURVE('',#30585,#30691,#25707,.T.) ;
#36799=EDGE_CURVE('',#30703,#30592,#25708,.T.) ;
#36800=EDGE_CURVE('',#30706,#30703,#25709,.T.) ;
#36801=EDGE_CURVE('',#30711,#30708,#25710,.T.) ;
#36802=EDGE_CURVE('',#30577,#30711,#25711,.T.) ;
#36803=EDGE_CURVE('',#30692,#30688,#25712,.T.) ;
#36804=EDGE_CURVE('',#30586,#30695,#25713,.T.) ;
#36805=EDGE_CURVE('',#30706,#30591,#25714,.T.) ;
#36806=EDGE_CURVE('',#30577,#30708,#25715,.T.) ;
#36807=EDGE_CURVE('',#30693,#30687,#25716,.T.) ;
#36808=EDGE_CURVE('',#30694,#30699,#25717,.T.) ;
#36809=EDGE_CURVE('',#30696,#30693,#25718,.T.) ;
#36810=EDGE_CURVE('',#30587,#30694,#25719,.T.) ;
#36811=EDGE_CURVE('',#30707,#30590,#25720,.T.) ;
#36812=EDGE_CURVE('',#30578,#30707,#25721,.T.) ;
#36813=EDGE_CURVE('',#30696,#30687,#25722,.T.) ;
#36814=EDGE_CURVE('',#30588,#30699,#25723,.T.) ;
#36815=EDGE_CURVE('',#30579,#30590,#25724,.T.) ;
#36816=EDGE_CURVE('',#30689,#30582,#25725,.T.) ;
#36817=EDGE_CURVE('',#30697,#30689,#25726,.T.) ;
#36818=EDGE_CURVE('',#30589,#30698,#25727,.T.) ;
#36819=EDGE_CURVE('',#30580,#30589,#25728,.T.) ;
#36820=EDGE_CURVE('',#30697,#30582,#25729,.T.) ;
#36821=EDGE_CURVE('',#30581,#30698,#25730,.T.) ;
#36822=EDGE_CURVE('',#30645,#30626,#25731,.T.) ;
#36823=EDGE_CURVE('',#30634,#30645,#25732,.T.) ;
#36824=EDGE_CURVE('',#30626,#30634,#25733,.T.) ;
#36825=EDGE_CURVE('',#30652,#30800,#136,.T.) ;
#36826=EDGE_CURVE('',#30800,#30631,#4882,.T.) ;
#36827=EDGE_CURVE('',#30633,#30801,#4883,.T.) ;
#36828=EDGE_CURVE('',#30801,#30619,#137,.T.) ;
#36829=EDGE_CURVE('',#30646,#30625,#25734,.T.) ;
#36830=EDGE_CURVE('',#30641,#30802,#4884,.T.) ;
#36831=EDGE_CURVE('',#30802,#30652,#138,.T.) ;
#36832=EDGE_CURVE('',#30651,#30803,#139,.T.) ;
#36833=EDGE_CURVE('',#30803,#30642,#4885,.T.) ;
#36834=EDGE_CURVE('',#30619,#30804,#140,.T.) ;
#36835=EDGE_CURVE('',#30804,#30636,#4886,.T.) ;
#36836=EDGE_CURVE('',#30635,#30805,#4887,.T.) ;
#36837=EDGE_CURVE('',#30805,#30620,#141,.T.) ;
#36838=EDGE_CURVE('',#30646,#30617,#25735,.T.) ;
#36839=EDGE_CURVE('',#30616,#30625,#25736,.T.) ;
#36840=EDGE_CURVE('',#30806,#30617,#8911,.T.) ;
#36841=EDGE_CURVE('',#30647,#30806,#25737,.T.) ;
#36842=EDGE_CURVE('',#30807,#30806,#25738,.T.) ;
#36843=EDGE_CURVE('',#30647,#30807,#25739,.T.) ;
#36844=EDGE_CURVE('',#30630,#30808,#4888,.T.) ;
#36845=EDGE_CURVE('',#30808,#30651,#142,.T.) ;
#36846=EDGE_CURVE('',#30627,#30650,#25740,.T.) ;
#36847=EDGE_CURVE('',#30620,#30809,#143,.T.) ;
#36848=EDGE_CURVE('',#30809,#30628,#4889,.T.) ;
#36849=EDGE_CURVE('',#30621,#30627,#25741,.T.) ;
#36850=EDGE_CURVE('',#30810,#30624,#25742,.T.) ;
#36851=EDGE_CURVE('',#30616,#30810,#8912,.T.) ;
#36852=EDGE_CURVE('',#30605,#30618,#4890,.T.) ;
#36853=EDGE_CURVE('',#30806,#30603,#25743,.T.) ;
#36854=EDGE_CURVE('',#30807,#30604,#25744,.T.) ;
#36855=EDGE_CURVE('',#30811,#30807,#8913,.T.) ;
#36856=EDGE_CURVE('',#30648,#30811,#25745,.T.) ;
#36857=EDGE_CURVE('',#30621,#30650,#25746,.T.) ;
#36858=EDGE_CURVE('',#30810,#30812,#25747,.T.) ;
#36859=EDGE_CURVE('',#30812,#30624,#25748,.T.) ;
#36860=EDGE_CURVE('',#30611,#30810,#25749,.T.) ;
#36861=EDGE_CURVE('',#30811,#30608,#25750,.T.) ;
#36862=EDGE_CURVE('',#30813,#30811,#25751,.T.) ;
#36863=EDGE_CURVE('',#30648,#30813,#25752,.T.) ;
#36864=EDGE_CURVE('',#30622,#30649,#25753,.T.) ;
#36865=EDGE_CURVE('',#30814,#30623,#25754,.T.) ;
#36866=EDGE_CURVE('',#30812,#30814,#8914,.T.) ;
#36867=EDGE_CURVE('',#30612,#30812,#25755,.T.) ;
#36868=EDGE_CURVE('',#30813,#30607,#25756,.T.) ;
#36869=EDGE_CURVE('',#30613,#30813,#8915,.T.) ;
#36870=EDGE_CURVE('',#30649,#30613,#25757,.T.) ;
#36871=EDGE_CURVE('',#30622,#30615,#25758,.T.) ;
#36872=EDGE_CURVE('',#30814,#30815,#25759,.T.) ;
#36873=EDGE_CURVE('',#30815,#30623,#25760,.T.) ;
#36874=EDGE_CURVE('',#30610,#30814,#25761,.T.) ;
#36875=EDGE_CURVE('',#30614,#30606,#4891,.T.) ;
#36876=EDGE_CURVE('',#30815,#30615,#8916,.T.) ;
#36877=EDGE_CURVE('',#30609,#30815,#25762,.T.) ;
#36878=EDGE_CURVE('',#30663,#30667,#25763,.T.) ;
#36879=EDGE_CURVE('',#30663,#30671,#25764,.T.) ;
#36880=EDGE_CURVE('',#30671,#30667,#25765,.T.) ;
#36881=EDGE_CURVE('',#30666,#30583,#25766,.T.) ;
#36882=EDGE_CURVE('',#30672,#30666,#25767,.T.) ;
#36883=EDGE_CURVE('',#30664,#30670,#25768,.T.) ;
#36884=EDGE_CURVE('',#30495,#30661,#25769,.T.) ;
#36885=EDGE_CURVE('',#30466,#30496,#25770,.T.) ;
#36886=EDGE_CURVE('',#30469,#30495,#25771,.T.) ;
#36887=EDGE_CURVE('',#30672,#30584,#25772,.T.) ;
#36888=EDGE_CURVE('',#30664,#30668,#25773,.T.) ;
#36889=EDGE_CURVE('',#30668,#30670,#25774,.T.) ;
#36890=EDGE_CURVE('',#30469,#30662,#25775,.T.) ;
#36891=EDGE_CURVE('',#30673,#30602,#25776,.T.) ;
#36892=EDGE_CURVE('',#30669,#30673,#25777,.T.) ;
#36893=EDGE_CURVE('',#30665,#30464,#25778,.T.) ;
#36894=EDGE_CURVE('',#30463,#30665,#25779,.T.) ;
#36895=EDGE_CURVE('',#30501,#30465,#25780,.T.) ;
#36896=EDGE_CURVE('',#30502,#30472,#25781,.T.) ;
#36897=EDGE_CURVE('',#30684,#30502,#25782,.T.) ;
#36898=EDGE_CURVE('',#30680,#30683,#25783,.T.) ;
#36899=EDGE_CURVE('',#30669,#30601,#25784,.T.) ;
#36900=EDGE_CURVE('',#30685,#30472,#25785,.T.) ;
#36901=EDGE_CURVE('',#30680,#30674,#25786,.T.) ;
#36902=EDGE_CURVE('',#30674,#30683,#25787,.T.) ;
#36903=EDGE_CURVE('',#30462,#30600,#144,.T.) ;
#36904=EDGE_CURVE('',#30686,#30460,#25788,.T.) ;
#36905=EDGE_CURVE('',#30682,#30679,#25789,.T.) ;
#36906=EDGE_CURVE('',#30458,#30686,#25790,.T.) ;
#36907=EDGE_CURVE('',#30675,#30682,#25791,.T.) ;
#36908=EDGE_CURVE('',#30681,#30677,#25792,.T.) ;
#36909=EDGE_CURVE('',#30595,#30681,#25793,.T.) ;
#36910=EDGE_CURVE('',#30470,#30600,#25794,.T.) ;
#36911=EDGE_CURVE('',#30816,#30459,#25795,.T.) ;
#36912=EDGE_CURVE('',#30675,#30679,#25796,.T.) ;
#36913=EDGE_CURVE('',#30596,#30677,#25797,.T.) ;
#36914=EDGE_CURVE('',#30471,#30599,#25798,.T.) ;
#36915=EDGE_CURVE('',#30676,#30678,#25799,.T.) ;
#36916=EDGE_CURVE('',#30597,#30676,#25800,.T.) ;
#36917=EDGE_CURVE('',#30456,#30599,#145,.T.) ;
#36918=EDGE_CURVE('',#30598,#30678,#25801,.T.) ;
#36919=EDGE_CURVE('',#30475,#30756,#146,.T.) ;
#36920=EDGE_CURVE('',#30759,#30755,#25802,.T.) ;
#36921=EDGE_CURVE('',#30754,#30760,#25803,.T.) ;
#36922=EDGE_CURVE('',#30757,#30640,#147,.T.) ;
#36923=EDGE_CURVE('',#30752,#30777,#25804,.T.) ;
#36924=EDGE_CURVE('',#30764,#30791,#25805,.T.) ;
#36925=EDGE_CURVE('',#30765,#30790,#25806,.T.) ;
#36926=EDGE_CURVE('',#30751,#30478,#148,.T.) ;
#36927=EDGE_CURVE('',#30746,#30758,#25807,.T.) ;
#36928=EDGE_CURVE('',#30776,#30753,#25808,.T.) ;
#36929=EDGE_CURVE('',#30765,#30769,#25809,.T.) ;
#36930=EDGE_CURVE('',#30769,#30790,#25810,.T.) ;
#36931=EDGE_CURVE('',#30761,#30747,#25811,.T.) ;
#36932=EDGE_CURVE('',#30792,#30771,#25812,.T.) ;
#36933=EDGE_CURVE('',#30793,#30770,#25813,.T.) ;
#36934=EDGE_CURVE('',#30766,#30793,#25814,.T.) ;
#36935=EDGE_CURVE('',#30762,#30768,#25815,.T.) ;
#36936=EDGE_CURVE('',#30788,#30763,#25816,.T.) ;
#36937=EDGE_CURVE('',#30789,#30762,#25817,.T.) ;
#36938=EDGE_CURVE('',#30766,#30770,#25818,.T.) ;
#36939=EDGE_CURVE('',#30789,#30768,#25819,.T.) ;
#36940=EDGE_CURVE('',#30767,#30773,#25820,.T.) ;
#36941=EDGE_CURVE('',#30786,#30767,#25821,.T.) ;
#36942=EDGE_CURVE('',#30786,#30773,#25822,.T.) ;
#36943=EDGE_CURVE('',#30772,#30787,#25823,.T.) ;
#36944=EDGE_CURVE('',#30748,#30775,#25824,.T.) ;
#36945=EDGE_CURVE('',#30749,#30774,#25825,.T.) ;
#36946=EDGE_CURVE('',#30643,#30750,#149,.T.) ;
#36947=EDGE_CURVE('',#30741,#30742,#25826,.T.) ;
#36948=EDGE_CURVE('',#30745,#30740,#25827,.T.) ;
#36949=EDGE_CURVE('',#30728,#30779,#25828,.T.) ;
#36950=EDGE_CURVE('',#30729,#30778,#25829,.T.) ;
#36951=EDGE_CURVE('',#30780,#30735,#25830,.T.) ;
#36952=EDGE_CURVE('',#30781,#30734,#25831,.T.) ;
#36953=EDGE_CURVE('',#30778,#30733,#25832,.T.) ;
#36954=EDGE_CURVE('',#30730,#30781,#25833,.T.) ;
#36955=EDGE_CURVE('',#30729,#30733,#25834,.T.) ;
#36956=EDGE_CURVE('',#30743,#30738,#25835,.T.) ;
#36957=EDGE_CURVE('',#30739,#30744,#25836,.T.) ;
#36958=EDGE_CURVE('',#30730,#30734,#25837,.T.) ;
#36959=EDGE_CURVE('',#30726,#30732,#25838,.T.) ;
#36960=EDGE_CURVE('',#30784,#30727,#25839,.T.) ;
#36961=EDGE_CURVE('',#30785,#30726,#25840,.T.) ;
#36962=EDGE_CURVE('',#30736,#30783,#25841,.T.) ;
#36963=EDGE_CURVE('',#30737,#30782,#25842,.T.) ;
#36964=EDGE_CURVE('',#30731,#30737,#25843,.T.) ;
#36965=EDGE_CURVE('',#30785,#30732,#25844,.T.) ;
#36966=EDGE_CURVE('',#30731,#30782,#25845,.T.) ;
#36967=EDGE_CURVE('',#30489,#30488,#25846,.T.) ;
#36968=EDGE_CURVE('',#30715,#30490,#150,.T.) ;
#36969=EDGE_CURVE('',#30716,#30489,#25847,.T.) ;
#36970=EDGE_CURVE('',#30716,#30488,#25848,.T.) ;
#36971=EDGE_CURVE('',#30487,#30484,#25849,.T.) ;
#36972=EDGE_CURVE('',#30713,#30487,#25850,.T.) ;
#36973=EDGE_CURVE('',#30713,#30484,#25851,.T.) ;
#36974=EDGE_CURVE('',#30483,#30714,#151,.T.) ;
#36975=EDGE_CURVE('',#30445,#30724,#4892,.T.) ;
#36976=EDGE_CURVE('',#30572,#30723,#25852,.T.) ;
#36977=EDGE_CURVE('',#30569,#30572,#25853,.T.) ;
#36978=EDGE_CURVE('',#30569,#30723,#25854,.T.) ;
#36979=EDGE_CURVE('',#30570,#30725,#25855,.T.) ;
#36980=EDGE_CURVE('',#30568,#30570,#25856,.T.) ;
#36981=EDGE_CURVE('',#30568,#30725,#25857,.T.) ;
#36982=EDGE_CURVE('',#30449,#30565,#4893,.T.) ;
#36983=EDGE_CURVE('',#30637,#30474,#25858,.T.) ;
#36984=EDGE_CURVE('',#30473,#30638,#25859,.T.) ;
#36985=EDGE_CURVE('',#30799,#30507,#25860,.T.) ;
#36986=EDGE_CURVE('',#30796,#30508,#25861,.T.) ;
#36987=EDGE_CURVE('',#30507,#30797,#25862,.T.) ;
#36988=EDGE_CURVE('',#30508,#30794,#25863,.T.) ;
#36989=EDGE_CURVE('',#30631,#30641,#25864,.T.) ;
#36990=EDGE_CURVE('',#30632,#30474,#25865,.T.) ;
#36991=EDGE_CURVE('',#30632,#30637,#25866,.T.) ;
#36992=EDGE_CURVE('',#30633,#30636,#25867,.T.) ;
#36993=EDGE_CURVE('',#30628,#30635,#25868,.T.) ;
#36994=EDGE_CURVE('',#30629,#30638,#25869,.T.) ;
#36995=EDGE_CURVE('',#30629,#30473,#25870,.T.) ;
#36996=EDGE_CURVE('',#30630,#30642,#25871,.T.) ;
#36997=EDGE_CURVE('',#30482,#30718,#152,.T.) ;
#36998=EDGE_CURVE('',#30714,#30717,#25872,.T.) ;
#36999=EDGE_CURVE('',#30715,#30722,#25873,.T.) ;
#37000=EDGE_CURVE('',#30817,#30721,#153,.T.) ;
#37001=EDGE_CURVE('',#30818,#30817,#154,.T.) ;
#37002=EDGE_CURVE('',#30819,#30818,#155,.T.) ;
#37003=EDGE_CURVE('',#30491,#30819,#156,.T.) ;
#37004=EDGE_CURVE('',#30573,#30492,#4894,.T.) ;
#37005=EDGE_CURVE('',#30574,#30721,#25874,.T.) ;
#37006=EDGE_CURVE('',#30448,#30566,#157,.T.) ;
#37007=EDGE_CURVE('',#30575,#30720,#25875,.T.) ;
#37008=EDGE_CURVE('',#30571,#30576,#4895,.T.) ;
#37009=EDGE_CURVE('',#30719,#30724,#25876,.T.) ;
#37010=EDGE_CURVE('',#30820,#30720,#158,.T.) ;
#37011=EDGE_CURVE('',#30821,#30820,#159,.T.) ;
#37012=EDGE_CURVE('',#30444,#30821,#160,.T.) ;
#37013=EDGE_CURVE('',#30501,#30795,#25877,.T.) ;
#37014=EDGE_CURVE('',#30467,#30795,#25878,.T.) ;
#37015=EDGE_CURVE('',#30796,#30794,#25879,.T.) ;
#37016=EDGE_CURVE('',#30764,#30760,#25880,.T.) ;
#37017=EDGE_CURVE('',#30791,#30754,#25881,.T.) ;
#37018=EDGE_CURVE('',#30761,#30763,#25882,.T.) ;
#37019=EDGE_CURVE('',#30792,#30753,#25883,.T.) ;
#37020=EDGE_CURVE('',#30747,#30788,#25884,.T.) ;
#37021=EDGE_CURVE('',#30771,#30776,#25885,.T.) ;
#37022=EDGE_CURVE('',#30748,#30787,#25886,.T.) ;
#37023=EDGE_CURVE('',#30772,#30775,#25887,.T.) ;
#37024=EDGE_CURVE('',#30728,#30742,#25888,.T.) ;
#37025=EDGE_CURVE('',#30779,#30741,#25889,.T.) ;
#37026=EDGE_CURVE('',#30743,#30727,#25890,.T.) ;
#37027=EDGE_CURVE('',#30780,#30740,#25891,.T.) ;
#37028=EDGE_CURVE('',#30738,#30784,#25892,.T.) ;
#37029=EDGE_CURVE('',#30735,#30745,#25893,.T.) ;
#37030=EDGE_CURVE('',#30739,#30783,#25894,.T.) ;
#37031=EDGE_CURVE('',#30736,#30744,#25895,.T.) ;
#37032=EDGE_CURVE('',#30798,#30496,#25896,.T.) ;
#37033=EDGE_CURVE('',#30798,#30468,#25897,.T.) ;
#37034=EDGE_CURVE('',#30799,#30797,#25898,.T.) ;
#37035=EDGE_CURVE('',#30563,#30567,#4896,.T.) ;
#37036=EDGE_CURVE('',#30564,#30447,#25899,.T.) ;
#37037=EDGE_CURVE('',#30561,#30718,#25900,.T.) ;
#37038=EDGE_CURVE('',#30562,#30481,#4897,.T.) ;
#37039=EDGE_CURVE('',#30822,#30823,#161,.T.) ;
#37040=EDGE_CURVE('',#30823,#30824,#4898,.T.) ;
#37041=EDGE_CURVE('',#30824,#30825,#25901,.T.) ;
#37042=EDGE_CURVE('',#30826,#30825,#4899,.T.) ;
#37043=EDGE_CURVE('',#30822,#30826,#162,.T.) ;
#37044=EDGE_CURVE('',#30827,#30828,#163,.T.) ;
#37045=EDGE_CURVE('',#30828,#30829,#25902,.T.) ;
#37046=EDGE_CURVE('',#30830,#30829,#4900,.T.) ;
#37047=EDGE_CURVE('',#30831,#30830,#25903,.T.) ;
#37048=EDGE_CURVE('',#30827,#30831,#4901,.T.) ;
#37049=EDGE_CURVE('',#30832,#30832,#25904,.T.) ;
#37050=EDGE_CURVE('',#30832,#30833,#25905,.T.) ;
#37051=EDGE_CURVE('',#30833,#30833,#25906,.T.) ;
#37052=EDGE_CURVE('',#30834,#30834,#25907,.T.) ;
#37053=EDGE_CURVE('',#30834,#30835,#25908,.T.) ;
#37054=EDGE_CURVE('',#30835,#30835,#25909,.T.) ;
#37055=EDGE_CURVE('',#30836,#30837,#25910,.T.) ;
#37056=EDGE_CURVE('',#30838,#30836,#8917,.T.) ;
#37057=EDGE_CURVE('',#30838,#30839,#25911,.T.) ;
#37058=EDGE_CURVE('',#30839,#30840,#25912,.T.) ;
#37059=EDGE_CURVE('',#30837,#30840,#8918,.T.) ;
#37060=EDGE_CURVE('',#30841,#30842,#25913,.T.) ;
#37061=EDGE_CURVE('',#30843,#30841,#8919,.T.) ;
#37062=EDGE_CURVE('',#30843,#30844,#25914,.T.) ;
#37063=EDGE_CURVE('',#30842,#30844,#8920,.T.) ;
#37064=EDGE_CURVE('',#30845,#30846,#25915,.T.) ;
#37065=EDGE_CURVE('',#30845,#30847,#25916,.T.) ;
#37066=EDGE_CURVE('',#30848,#30847,#25917,.T.) ;
#37067=EDGE_CURVE('',#30848,#30846,#25918,.T.) ;
#37068=EDGE_CURVE('',#30833,#30834,#8921,.T.) ;
#37069=EDGE_CURVE('',#30846,#30849,#8922,.T.) ;
#37070=EDGE_CURVE('',#30849,#30843,#25919,.T.) ;
#37071=EDGE_CURVE('',#30850,#30841,#164,.T.) ;
#37072=EDGE_CURVE('',#30850,#30851,#25920,.T.) ;
#37073=EDGE_CURVE('',#30837,#30851,#165,.T.) ;
#37074=EDGE_CURVE('',#30840,#30852,#25921,.T.) ;
#37075=EDGE_CURVE('',#30852,#30845,#8923,.T.) ;
#37076=EDGE_CURVE('',#30853,#30854,#8924,.T.) ;
#37077=EDGE_CURVE('',#30854,#30855,#8925,.T.) ;
#37078=EDGE_CURVE('',#30855,#30856,#166,.T.) ;
#37079=EDGE_CURVE('',#30856,#30857,#8926,.T.) ;
#37080=EDGE_CURVE('',#30857,#30858,#4902,.T.) ;
#37081=EDGE_CURVE('',#30858,#30853,#8927,.T.) ;
#37082=EDGE_CURVE('',#30859,#30860,#8928,.T.) ;
#37083=EDGE_CURVE('',#30860,#30861,#8929,.T.) ;
#37084=EDGE_CURVE('',#30861,#30862,#167,.T.) ;
#37085=EDGE_CURVE('',#30862,#30863,#168,.T.) ;
#37086=EDGE_CURVE('',#30863,#30864,#8930,.T.) ;
#37087=EDGE_CURVE('',#30864,#30859,#8931,.T.) ;
#37088=EDGE_CURVE('',#30865,#30866,#8932,.T.) ;
#37089=EDGE_CURVE('',#30866,#30867,#8933,.T.) ;
#37090=EDGE_CURVE('',#30867,#30868,#8934,.T.) ;
#37091=EDGE_CURVE('',#30868,#30865,#8935,.T.) ;
#37092=EDGE_CURVE('',#30869,#30870,#8936,.T.) ;
#37093=EDGE_CURVE('',#30870,#30871,#169,.T.) ;
#37094=EDGE_CURVE('',#30871,#30872,#170,.T.) ;
#37095=EDGE_CURVE('',#30872,#30873,#8937,.T.) ;
#37096=EDGE_CURVE('',#30873,#30874,#8938,.T.) ;
#37097=EDGE_CURVE('',#30874,#30869,#8939,.T.) ;
#37098=EDGE_CURVE('',#30875,#30876,#8940,.T.) ;
#37099=EDGE_CURVE('',#30876,#30877,#8941,.T.) ;
#37100=EDGE_CURVE('',#30877,#30878,#8942,.T.) ;
#37101=EDGE_CURVE('',#30878,#30875,#8943,.T.) ;
#37102=EDGE_CURVE('',#30879,#30880,#8944,.T.) ;
#37103=EDGE_CURVE('',#30879,#30881,#8945,.T.) ;
#37104=EDGE_CURVE('',#30881,#30882,#8946,.T.) ;
#37105=EDGE_CURVE('',#30882,#30880,#8947,.T.) ;
#37106=EDGE_CURVE('',#30883,#30884,#8948,.T.) ;
#37107=EDGE_CURVE('',#30883,#30885,#8949,.T.) ;
#37108=EDGE_CURVE('',#30885,#30886,#8950,.T.) ;
#37109=EDGE_CURVE('',#30886,#30887,#8951,.T.) ;
#37110=EDGE_CURVE('',#30887,#30888,#25922,.T.) ;
#37111=EDGE_CURVE('',#30888,#30884,#8952,.T.) ;
#37112=EDGE_CURVE('',#30889,#30890,#8953,.T.) ;
#37113=EDGE_CURVE('',#30889,#30860,#25923,.T.) ;
#37114=EDGE_CURVE('',#30859,#30866,#25924,.T.) ;
#37115=EDGE_CURVE('',#30865,#30874,#25925,.T.) ;
#37116=EDGE_CURVE('',#30873,#30891,#25926,.T.) ;
#37117=EDGE_CURVE('',#30892,#30891,#8954,.T.) ;
#37118=EDGE_CURVE('',#30892,#30893,#25927,.T.) ;
#37119=EDGE_CURVE('',#30894,#30893,#8955,.T.) ;
#37120=EDGE_CURVE('',#30894,#30895,#25928,.T.) ;
#37121=EDGE_CURVE('',#30895,#30896,#8956,.T.) ;
#37122=EDGE_CURVE('',#30896,#30897,#25929,.T.) ;
#37123=EDGE_CURVE('',#30898,#30897,#8957,.T.) ;
#37124=EDGE_CURVE('',#30898,#30899,#25930,.T.) ;
#37125=EDGE_CURVE('',#30899,#30900,#8958,.T.) ;
#37126=EDGE_CURVE('',#30900,#30901,#25931,.T.) ;
#37127=EDGE_CURVE('',#30902,#30901,#8959,.T.) ;
#37128=EDGE_CURVE('',#30902,#30878,#25932,.T.) ;
#37129=EDGE_CURVE('',#30877,#30903,#25933,.T.) ;
#37130=EDGE_CURVE('',#30903,#30904,#8960,.T.) ;
#37131=EDGE_CURVE('',#30904,#30886,#25934,.T.) ;
#37132=EDGE_CURVE('',#30885,#30905,#25935,.T.) ;
#37133=EDGE_CURVE('',#30906,#30905,#8961,.T.) ;
#37134=EDGE_CURVE('',#30907,#30906,#8962,.T.) ;
#37135=EDGE_CURVE('',#30907,#30908,#25936,.T.) ;
#37136=EDGE_CURVE('',#30909,#30908,#8963,.T.) ;
#37137=EDGE_CURVE('',#30909,#30910,#25937,.T.) ;
#37138=EDGE_CURVE('',#30911,#30910,#8964,.T.) ;
#37139=EDGE_CURVE('',#30911,#30890,#25938,.T.) ;
#37140=EDGE_CURVE('',#30912,#30913,#8965,.T.) ;
#37141=EDGE_CURVE('',#30913,#30914,#25939,.T.) ;
#37142=EDGE_CURVE('',#30914,#30915,#8966,.T.) ;
#37143=EDGE_CURVE('',#30915,#30916,#25940,.T.) ;
#37144=EDGE_CURVE('',#30916,#30917,#8967,.T.) ;
#37145=EDGE_CURVE('',#30917,#30918,#25941,.T.) ;
#37146=EDGE_CURVE('',#30918,#30919,#8968,.T.) ;
#37147=EDGE_CURVE('',#30919,#30920,#25942,.T.) ;
#37148=EDGE_CURVE('',#30920,#30921,#8969,.T.) ;
#37149=EDGE_CURVE('',#30921,#30922,#8970,.T.) ;
#37150=EDGE_CURVE('',#30922,#30883,#25943,.T.) ;
#37151=EDGE_CURVE('',#30884,#30923,#25944,.T.) ;
#37152=EDGE_CURVE('',#30923,#30924,#8971,.T.) ;
#37153=EDGE_CURVE('',#30924,#30879,#25945,.T.) ;
#37154=EDGE_CURVE('',#30880,#30925,#25946,.T.) ;
#37155=EDGE_CURVE('',#30926,#30925,#8972,.T.) ;
#37156=EDGE_CURVE('',#30926,#30927,#25947,.T.) ;
#37157=EDGE_CURVE('',#30928,#30927,#8973,.T.) ;
#37158=EDGE_CURVE('',#30928,#30929,#25948,.T.) ;
#37159=EDGE_CURVE('',#30929,#30930,#8974,.T.) ;
#37160=EDGE_CURVE('',#30930,#30931,#25949,.T.) ;
#37161=EDGE_CURVE('',#30932,#30931,#8975,.T.) ;
#37162=EDGE_CURVE('',#30932,#30933,#25950,.T.) ;
#37163=EDGE_CURVE('',#30934,#30933,#8976,.T.) ;
#37164=EDGE_CURVE('',#30934,#30935,#25951,.T.) ;
#37165=EDGE_CURVE('',#30935,#30936,#8977,.T.) ;
#37166=EDGE_CURVE('',#30936,#30937,#25952,.T.) ;
#37167=EDGE_CURVE('',#30937,#30938,#8978,.T.) ;
#37168=EDGE_CURVE('',#30938,#30939,#25953,.T.) ;
#37169=EDGE_CURVE('',#30939,#30940,#8979,.T.) ;
#37170=EDGE_CURVE('',#30940,#30912,#25954,.T.) ;
#37171=EDGE_CURVE('',#30908,#30919,#8980,.T.) ;
#37172=EDGE_CURVE('',#30918,#30909,#8981,.T.) ;
#37173=EDGE_CURVE('',#30910,#30917,#8982,.T.) ;
#37174=EDGE_CURVE('',#30916,#30911,#8983,.T.) ;
#37175=EDGE_CURVE('',#30941,#30942,#171,.T.) ;
#37176=EDGE_CURVE('',#30942,#30889,#8984,.T.) ;
#37177=EDGE_CURVE('',#30890,#30915,#8985,.T.) ;
#37178=EDGE_CURVE('',#30914,#30943,#8986,.T.) ;
#37179=EDGE_CURVE('',#30943,#30944,#172,.T.) ;
#37180=EDGE_CURVE('',#30944,#30941,#8987,.T.) ;
#37181=EDGE_CURVE('',#30945,#30946,#173,.T.) ;
#37182=EDGE_CURVE('',#30946,#30947,#4903,.T.) ;
#37183=EDGE_CURVE('',#30947,#30913,#8988,.T.) ;
#37184=EDGE_CURVE('',#30912,#30948,#8989,.T.) ;
#37185=EDGE_CURVE('',#30948,#30945,#8990,.T.) ;
#37186=EDGE_CURVE('',#30949,#30950,#8991,.T.) ;
#37187=EDGE_CURVE('',#30950,#30940,#8992,.T.) ;
#37188=EDGE_CURVE('',#30939,#30949,#8993,.T.) ;
#37189=EDGE_CURVE('',#30951,#30822,#174,.T.) ;
#37190=EDGE_CURVE('',#30826,#30952,#8994,.T.) ;
#37191=EDGE_CURVE('',#30952,#30938,#8995,.T.) ;
#37192=EDGE_CURVE('',#30937,#30951,#8996,.T.) ;
#37193=EDGE_CURVE('',#30891,#30953,#8997,.T.) ;
#37194=EDGE_CURVE('',#30953,#30954,#175,.T.) ;
#37195=EDGE_CURVE('',#30954,#30955,#8998,.T.) ;
#37196=EDGE_CURVE('',#30955,#30956,#176,.T.) ;
#37197=EDGE_CURVE('',#30956,#30936,#8999,.T.) ;
#37198=EDGE_CURVE('',#30935,#30957,#9000,.T.) ;
#37199=EDGE_CURVE('',#30957,#30958,#9001,.T.) ;
#37200=EDGE_CURVE('',#30959,#30958,#25955,.T.) ;
#37201=EDGE_CURVE('',#30959,#30960,#9002,.T.) ;
#37202=EDGE_CURVE('',#30961,#30960,#25956,.T.) ;
#37203=EDGE_CURVE('',#30961,#30962,#9003,.T.) ;
#37204=EDGE_CURVE('',#30962,#30892,#9004,.T.) ;
#37205=EDGE_CURVE('',#30963,#30964,#25957,.T.) ;
#37206=EDGE_CURVE('',#30963,#30898,#9005,.T.) ;
#37207=EDGE_CURVE('',#30897,#30965,#9006,.T.) ;
#37208=EDGE_CURVE('',#30966,#30965,#25958,.T.) ;
#37209=EDGE_CURVE('',#30966,#30967,#25959,.T.) ;
#37210=EDGE_CURVE('',#30968,#30967,#25960,.T.) ;
#37211=EDGE_CURVE('',#30968,#30969,#9007,.T.) ;
#37212=EDGE_CURVE('',#30969,#30970,#9008,.T.) ;
#37213=EDGE_CURVE('',#30970,#30971,#9009,.T.) ;
#37214=EDGE_CURVE('',#30972,#30971,#25961,.T.) ;
#37215=EDGE_CURVE('',#30972,#30973,#25962,.T.) ;
#37216=EDGE_CURVE('',#30974,#30973,#25963,.T.) ;
#37217=EDGE_CURVE('',#30974,#30930,#9010,.T.) ;
#37218=EDGE_CURVE('',#30929,#30975,#9011,.T.) ;
#37219=EDGE_CURVE('',#30976,#30975,#25964,.T.) ;
#37220=EDGE_CURVE('',#30976,#30977,#25965,.T.) ;
#37221=EDGE_CURVE('',#30978,#30977,#25966,.T.) ;
#37222=EDGE_CURVE('',#30978,#30979,#9012,.T.) ;
#37223=EDGE_CURVE('',#30979,#30980,#25967,.T.) ;
#37224=EDGE_CURVE('',#30980,#30981,#9013,.T.) ;
#37225=EDGE_CURVE('',#30982,#30981,#25968,.T.) ;
#37226=EDGE_CURVE('',#30982,#30964,#25969,.T.) ;
#37227=EDGE_CURVE('',#30983,#30984,#25970,.T.) ;
#37228=EDGE_CURVE('',#30983,#30985,#9014,.T.) ;
#37229=EDGE_CURVE('',#30906,#30985,#9015,.T.) ;
#37230=EDGE_CURVE('',#30905,#30922,#9016,.T.) ;
#37231=EDGE_CURVE('',#30986,#30921,#9017,.T.) ;
#37232=EDGE_CURVE('',#30986,#30987,#9018,.T.) ;
#37233=EDGE_CURVE('',#30988,#30987,#25971,.T.) ;
#37234=EDGE_CURVE('',#30988,#30984,#9019,.T.) ;
#37235=EDGE_CURVE('',#30989,#30990,#25972,.T.) ;
#37236=EDGE_CURVE('',#30989,#30986,#9020,.T.) ;
#37237=EDGE_CURVE('',#30920,#30907,#9021,.T.) ;
#37238=EDGE_CURVE('',#30985,#30991,#9022,.T.) ;
#37239=EDGE_CURVE('',#30992,#30991,#25973,.T.) ;
#37240=EDGE_CURVE('',#30992,#30990,#9023,.T.) ;
#37241=EDGE_CURVE('',#30993,#30994,#9024,.T.) ;
#37242=EDGE_CURVE('',#30994,#30995,#9025,.T.) ;
#37243=EDGE_CURVE('',#30993,#30995,#25974,.T.) ;
#37244=EDGE_CURVE('',#30996,#30997,#25975,.T.) ;
#37245=EDGE_CURVE('',#30996,#30998,#9026,.T.) ;
#37246=EDGE_CURVE('',#30998,#30997,#9027,.T.) ;
#37247=EDGE_CURVE('',#30999,#31000,#9028,.T.) ;
#37248=EDGE_CURVE('',#31000,#31001,#9029,.T.) ;
#37249=EDGE_CURVE('',#31001,#31002,#9030,.T.) ;
#37250=EDGE_CURVE('',#31002,#31003,#9031,.T.) ;
#37251=EDGE_CURVE('',#31003,#31004,#9032,.T.) ;
#37252=EDGE_CURVE('',#31004,#31005,#9033,.T.) ;
#37253=EDGE_CURVE('',#31005,#31006,#9034,.T.) ;
#37254=EDGE_CURVE('',#31006,#30999,#9035,.T.) ;
#37255=EDGE_CURVE('',#31007,#31008,#9036,.T.) ;
#37256=EDGE_CURVE('',#31008,#31009,#9037,.T.) ;
#37257=EDGE_CURVE('',#31009,#31010,#9038,.T.) ;
#37258=EDGE_CURVE('',#31010,#31007,#9039,.T.) ;
#37259=EDGE_CURVE('',#31011,#31012,#9040,.T.) ;
#37260=EDGE_CURVE('',#31012,#31013,#9041,.T.) ;
#37261=EDGE_CURVE('',#31013,#31014,#9042,.T.) ;
#37262=EDGE_CURVE('',#31014,#31011,#9043,.T.) ;
#37263=EDGE_CURVE('',#31015,#31016,#9044,.T.) ;
#37264=EDGE_CURVE('',#31016,#31017,#9045,.T.) ;
#37265=EDGE_CURVE('',#31017,#31018,#9046,.T.) ;
#37266=EDGE_CURVE('',#31018,#31015,#9047,.T.) ;
#37267=EDGE_CURVE('',#31019,#31020,#177,.T.) ;
#37268=EDGE_CURVE('',#31020,#31021,#9048,.T.) ;
#37269=EDGE_CURVE('',#31021,#31022,#9049,.T.) ;
#37270=EDGE_CURVE('',#31022,#31023,#9050,.T.) ;
#37271=EDGE_CURVE('',#31023,#31024,#178,.T.) ;
#37272=EDGE_CURVE('',#31024,#31019,#9051,.T.) ;
#37273=EDGE_CURVE('',#31025,#31026,#9052,.T.) ;
#37274=EDGE_CURVE('',#31026,#31027,#9053,.T.) ;
#37275=EDGE_CURVE('',#31027,#31028,#9054,.T.) ;
#37276=EDGE_CURVE('',#31028,#31029,#9055,.T.) ;
#37277=EDGE_CURVE('',#31029,#31030,#9056,.T.) ;
#37278=EDGE_CURVE('',#31030,#31031,#9057,.T.) ;
#37279=EDGE_CURVE('',#31031,#31032,#9058,.T.) ;
#37280=EDGE_CURVE('',#31032,#31025,#9059,.T.) ;
#37281=EDGE_CURVE('',#31033,#31034,#9060,.T.) ;
#37282=EDGE_CURVE('',#31033,#31035,#25976,.T.) ;
#37283=EDGE_CURVE('',#31035,#31036,#9061,.T.) ;
#37284=EDGE_CURVE('',#31036,#31037,#25977,.T.) ;
#37285=EDGE_CURVE('',#31037,#31038,#9062,.T.) ;
#37286=EDGE_CURVE('',#31038,#31039,#25978,.T.) ;
#37287=EDGE_CURVE('',#31039,#31040,#9063,.T.) ;
#37288=EDGE_CURVE('',#31040,#31034,#25979,.T.) ;
#37289=EDGE_CURVE('',#31041,#31042,#25980,.T.) ;
#37290=EDGE_CURVE('',#31041,#30902,#9064,.T.) ;
#37291=EDGE_CURVE('',#30901,#31043,#9065,.T.) ;
#37292=EDGE_CURVE('',#31043,#31044,#25981,.T.) ;
#37293=EDGE_CURVE('',#31044,#31045,#9066,.T.) ;
#37294=EDGE_CURVE('',#31045,#31042,#25982,.T.) ;
#37295=EDGE_CURVE('',#30899,#31046,#9067,.T.) ;
#37296=EDGE_CURVE('',#31046,#31047,#9068,.T.) ;
#37297=EDGE_CURVE('',#31047,#30900,#9069,.T.) ;
#37298=EDGE_CURVE('',#31048,#31049,#9070,.T.) ;
#37299=EDGE_CURVE('',#31049,#30842,#9071,.T.) ;
#37300=EDGE_CURVE('',#30844,#31048,#9072,.T.) ;
#37301=EDGE_CURVE('',#31050,#31051,#25983,.T.) ;
#37302=EDGE_CURVE('',#31051,#31052,#9073,.T.) ;
#37303=EDGE_CURVE('',#31052,#31053,#25984,.T.) ;
#37304=EDGE_CURVE('',#31053,#31050,#9074,.T.) ;
#37305=EDGE_CURVE('',#31054,#31055,#25985,.T.) ;
#37306=EDGE_CURVE('',#31055,#31056,#9075,.T.) ;
#37307=EDGE_CURVE('',#31056,#31057,#25986,.T.) ;
#37308=EDGE_CURVE('',#31057,#31054,#9076,.T.) ;
#37309=EDGE_CURVE('',#30836,#31058,#9077,.T.) ;
#37310=EDGE_CURVE('',#31058,#31059,#9078,.T.) ;
#37311=EDGE_CURVE('',#31059,#30838,#9079,.T.) ;
#37312=EDGE_CURVE('',#31060,#31061,#9080,.T.) ;
#37313=EDGE_CURVE('',#31061,#30928,#9081,.T.) ;
#37314=EDGE_CURVE('',#30927,#31060,#9082,.T.) ;
#37315=EDGE_CURVE('',#31062,#31063,#25987,.T.) ;
#37316=EDGE_CURVE('',#31063,#30926,#9083,.T.) ;
#37317=EDGE_CURVE('',#30925,#31064,#9084,.T.) ;
#37318=EDGE_CURVE('',#31065,#31064,#25988,.T.) ;
#37319=EDGE_CURVE('',#31065,#31066,#25989,.T.) ;
#37320=EDGE_CURVE('',#31066,#31062,#9085,.T.) ;
#37321=EDGE_CURVE('',#31067,#31068,#25990,.T.) ;
#37322=EDGE_CURVE('',#31068,#30894,#9086,.T.) ;
#37323=EDGE_CURVE('',#30893,#31069,#9087,.T.) ;
#37324=EDGE_CURVE('',#31069,#31067,#9088,.T.) ;
#37325=EDGE_CURVE('',#31070,#31071,#9089,.T.) ;
#37326=EDGE_CURVE('',#31071,#30896,#9090,.T.) ;
#37327=EDGE_CURVE('',#30895,#31070,#9091,.T.) ;
#37328=EDGE_CURVE('',#31072,#31073,#25991,.T.) ;
#37329=EDGE_CURVE('',#31073,#31074,#9092,.T.) ;
#37330=EDGE_CURVE('',#31074,#31075,#25992,.T.) ;
#37331=EDGE_CURVE('',#31075,#31072,#9093,.T.) ;
#37332=EDGE_CURVE('',#31076,#31077,#9094,.T.) ;
#37333=EDGE_CURVE('',#31077,#31078,#9095,.T.) ;
#37334=EDGE_CURVE('',#31078,#31079,#9096,.T.) ;
#37335=EDGE_CURVE('',#31079,#31076,#9097,.T.) ;
#37336=EDGE_CURVE('',#31080,#31081,#25993,.T.) ;
#37337=EDGE_CURVE('',#31081,#31082,#9098,.T.) ;
#37338=EDGE_CURVE('',#31082,#31083,#25994,.T.) ;
#37339=EDGE_CURVE('',#31083,#31080,#9099,.T.) ;
#37340=EDGE_CURVE('',#30931,#31084,#9100,.T.) ;
#37341=EDGE_CURVE('',#31084,#31085,#9101,.T.) ;
#37342=EDGE_CURVE('',#31085,#30932,#9102,.T.) ;
#37343=EDGE_CURVE('',#31086,#31087,#9103,.T.) ;
#37344=EDGE_CURVE('',#31087,#31088,#9104,.T.) ;
#37345=EDGE_CURVE('',#31088,#31089,#9105,.T.) ;
#37346=EDGE_CURVE('',#31089,#31086,#9106,.T.) ;
#37347=EDGE_CURVE('',#31090,#31091,#9107,.T.) ;
#37348=EDGE_CURVE('',#31091,#30934,#9108,.T.) ;
#37349=EDGE_CURVE('',#30933,#31092,#9109,.T.) ;
#37350=EDGE_CURVE('',#31092,#31090,#25995,.T.) ;
#37351=EDGE_CURVE('',#31093,#31094,#9110,.T.) ;
#37352=EDGE_CURVE('',#31094,#31095,#9111,.T.) ;
#37353=EDGE_CURVE('',#31095,#31096,#9112,.T.) ;
#37354=EDGE_CURVE('',#31096,#31093,#9113,.T.) ;
#37355=EDGE_CURVE('',#31097,#31098,#4904,.T.) ;
#37356=EDGE_CURVE('',#31098,#30827,#9114,.T.) ;
#37357=EDGE_CURVE('',#30831,#31099,#9115,.T.) ;
#37358=EDGE_CURVE('',#31099,#31100,#4905,.T.) ;
#37359=EDGE_CURVE('',#31100,#31101,#9116,.T.) ;
#37360=EDGE_CURVE('',#31101,#31102,#4906,.T.) ;
#37361=EDGE_CURVE('',#31102,#31097,#9117,.T.) ;
#37362=EDGE_CURVE('',#31103,#31104,#9118,.T.) ;
#37363=EDGE_CURVE('',#31104,#30830,#9119,.T.) ;
#37364=EDGE_CURVE('',#30830,#31105,#9120,.T.) ;
#37365=EDGE_CURVE('',#31105,#31103,#9121,.T.) ;
#37366=EDGE_CURVE('',#31106,#31107,#9122,.T.) ;
#37367=EDGE_CURVE('',#31107,#31108,#9123,.T.) ;
#37368=EDGE_CURVE('',#31108,#31109,#9124,.T.) ;
#37369=EDGE_CURVE('',#31109,#31106,#9125,.T.) ;
#37370=EDGE_CURVE('',#31110,#31111,#9126,.T.) ;
#37371=EDGE_CURVE('',#31111,#31112,#9127,.T.) ;
#37372=EDGE_CURVE('',#31112,#31113,#9128,.T.) ;
#37373=EDGE_CURVE('',#31113,#31110,#9129,.T.) ;
#37374=EDGE_CURVE('',#31114,#31115,#9130,.T.) ;
#37375=EDGE_CURVE('',#31115,#31116,#9131,.T.) ;
#37376=EDGE_CURVE('',#31116,#31117,#9132,.T.) ;
#37377=EDGE_CURVE('',#31117,#31114,#9133,.T.) ;
#37378=EDGE_CURVE('',#31034,#31118,#9134,.T.) ;
#37379=EDGE_CURVE('',#31118,#31119,#9135,.T.) ;
#37380=EDGE_CURVE('',#31119,#31033,#9136,.T.) ;
#37381=EDGE_CURVE('',#31037,#31120,#9137,.T.) ;
#37382=EDGE_CURVE('',#31120,#31121,#9138,.T.) ;
#37383=EDGE_CURVE('',#31121,#31038,#9139,.T.) ;
#37384=EDGE_CURVE('',#31039,#31122,#9140,.T.) ;
#37385=EDGE_CURVE('',#31122,#31123,#9141,.T.) ;
#37386=EDGE_CURVE('',#31123,#31040,#9142,.T.) ;
#37387=EDGE_CURVE('',#31035,#31124,#9143,.T.) ;
#37388=EDGE_CURVE('',#31124,#31125,#9144,.T.) ;
#37389=EDGE_CURVE('',#31125,#31036,#9145,.T.) ;
#37390=EDGE_CURVE('',#31126,#31127,#9146,.T.) ;
#37391=EDGE_CURVE('',#31127,#31128,#9147,.T.) ;
#37392=EDGE_CURVE('',#31128,#31129,#9148,.T.) ;
#37393=EDGE_CURVE('',#31129,#31130,#25996,.T.) ;
#37394=EDGE_CURVE('',#31130,#31131,#9149,.T.) ;
#37395=EDGE_CURVE('',#31131,#31126,#25997,.T.) ;
#37396=EDGE_CURVE('',#31132,#31133,#9150,.T.) ;
#37397=EDGE_CURVE('',#31133,#31134,#9151,.T.) ;
#37398=EDGE_CURVE('',#31134,#31135,#9152,.T.) ;
#37399=EDGE_CURVE('',#31135,#31136,#25998,.T.) ;
#37400=EDGE_CURVE('',#31136,#31137,#9153,.T.) ;
#37401=EDGE_CURVE('',#31137,#31132,#25999,.T.) ;
#37402=EDGE_CURVE('',#31138,#31139,#9154,.T.) ;
#37403=EDGE_CURVE('',#31138,#30857,#26000,.T.) ;
#37404=EDGE_CURVE('',#30856,#31139,#26001,.T.) ;
#37405=EDGE_CURVE('',#31139,#31140,#9155,.T.) ;
#37406=EDGE_CURVE('',#31140,#31141,#9156,.T.) ;
#37407=EDGE_CURVE('',#31141,#31138,#9157,.T.) ;
#37408=EDGE_CURVE('',#31142,#31143,#9158,.T.) ;
#37409=EDGE_CURVE('',#31143,#31144,#9159,.T.) ;
#37410=EDGE_CURVE('',#31144,#31145,#9160,.T.) ;
#37411=EDGE_CURVE('',#31145,#31142,#9161,.T.) ;
#37412=EDGE_CURVE('',#31146,#31147,#9162,.T.) ;
#37413=EDGE_CURVE('',#31147,#31148,#9163,.T.) ;
#37414=EDGE_CURVE('',#31148,#31149,#9164,.T.) ;
#37415=EDGE_CURVE('',#31149,#31146,#9165,.T.) ;
#37416=EDGE_CURVE('',#31150,#31151,#9166,.T.) ;
#37417=EDGE_CURVE('',#31151,#31152,#9167,.T.) ;
#37418=EDGE_CURVE('',#31152,#31153,#9168,.T.) ;
#37419=EDGE_CURVE('',#31153,#31150,#9169,.T.) ;
#37420=EDGE_CURVE('',#31154,#31155,#9170,.T.) ;
#37421=EDGE_CURVE('',#31155,#31156,#9171,.T.) ;
#37422=EDGE_CURVE('',#31156,#31157,#9172,.T.) ;
#37423=EDGE_CURVE('',#31154,#31157,#9173,.T.) ;
#37424=EDGE_CURVE('',#31024,#31154,#26002,.T.) ;
#37425=EDGE_CURVE('',#31157,#31019,#26003,.T.) ;
#37426=EDGE_CURVE('',#31158,#31159,#9174,.T.) ;
#37427=EDGE_CURVE('',#31159,#31160,#9175,.T.) ;
#37428=EDGE_CURVE('',#31160,#31161,#9176,.T.) ;
#37429=EDGE_CURVE('',#31161,#31158,#9177,.T.) ;
#37430=EDGE_CURVE('',#31162,#31163,#9178,.T.) ;
#37431=EDGE_CURVE('',#31163,#31164,#9179,.T.) ;
#37432=EDGE_CURVE('',#31164,#31165,#9180,.T.) ;
#37433=EDGE_CURVE('',#31165,#31162,#9181,.T.) ;
#37434=EDGE_CURVE('',#31166,#31167,#9182,.T.) ;
#37435=EDGE_CURVE('',#31167,#31168,#9183,.T.) ;
#37436=EDGE_CURVE('',#31168,#31169,#9184,.T.) ;
#37437=EDGE_CURVE('',#31169,#31166,#9185,.T.) ;
#37438=EDGE_CURVE('',#31170,#31171,#9186,.T.) ;
#37439=EDGE_CURVE('',#31171,#31172,#9187,.T.) ;
#37440=EDGE_CURVE('',#31172,#31173,#9188,.T.) ;
#37441=EDGE_CURVE('',#31173,#31170,#9189,.T.) ;
#37442=EDGE_CURVE('',#30923,#31174,#9190,.T.) ;
#37443=EDGE_CURVE('',#31174,#31175,#26004,.T.) ;
#37444=EDGE_CURVE('',#31175,#30924,#9191,.T.) ;
#37445=EDGE_CURVE('',#31176,#31177,#26005,.T.) ;
#37446=EDGE_CURVE('',#31177,#30848,#26006,.T.) ;
#37447=EDGE_CURVE('',#30847,#31176,#26007,.T.) ;
#37448=EDGE_CURVE('',#30903,#31178,#9192,.T.) ;
#37449=EDGE_CURVE('',#31178,#31179,#26008,.T.) ;
#37450=EDGE_CURVE('',#31179,#30904,#9193,.T.) ;
#37451=EDGE_CURVE('',#31092,#31085,#26009,.T.) ;
#37452=EDGE_CURVE('',#31092,#31081,#26010,.T.) ;
#37453=EDGE_CURVE('',#31081,#31085,#26011,.T.) ;
#37454=EDGE_CURVE('',#31084,#30974,#26012,.T.) ;
#37455=EDGE_CURVE('',#31082,#31084,#26013,.T.) ;
#37456=EDGE_CURVE('',#31090,#31080,#26014,.T.) ;
#37457=EDGE_CURVE('',#31082,#30973,#26015,.T.) ;
#37458=EDGE_CURVE('',#31090,#31089,#26016,.T.) ;
#37459=EDGE_CURVE('',#31089,#31080,#26017,.T.) ;
#37460=EDGE_CURVE('',#31070,#31068,#26018,.T.) ;
#37461=EDGE_CURVE('',#31071,#31075,#26019,.T.) ;
#37462=EDGE_CURVE('',#31072,#31070,#26020,.T.) ;
#37463=EDGE_CURVE('',#30965,#31071,#26021,.T.) ;
#37464=EDGE_CURVE('',#31083,#30972,#26022,.T.) ;
#37465=EDGE_CURVE('',#31086,#31083,#26023,.T.) ;
#37466=EDGE_CURVE('',#31091,#31088,#26024,.T.) ;
#37467=EDGE_CURVE('',#30957,#31091,#26025,.T.) ;
#37468=EDGE_CURVE('',#31072,#31068,#26026,.T.) ;
#37469=EDGE_CURVE('',#30966,#31075,#26027,.T.) ;
#37470=EDGE_CURVE('',#31086,#30971,#26028,.T.) ;
#37471=EDGE_CURVE('',#30957,#31088,#26029,.T.) ;
#37472=EDGE_CURVE('',#31073,#31067,#26030,.T.) ;
#37473=EDGE_CURVE('',#31074,#31079,#26031,.T.) ;
#37474=EDGE_CURVE('',#31076,#31073,#26032,.T.) ;
#37475=EDGE_CURVE('',#30967,#31074,#26033,.T.) ;
#37476=EDGE_CURVE('',#31087,#30970,#26034,.T.) ;
#37477=EDGE_CURVE('',#30958,#31087,#26035,.T.) ;
#37478=EDGE_CURVE('',#31076,#31067,#26036,.T.) ;
#37479=EDGE_CURVE('',#30968,#31079,#26037,.T.) ;
#37480=EDGE_CURVE('',#30959,#30970,#26038,.T.) ;
#37481=EDGE_CURVE('',#31069,#30962,#26039,.T.) ;
#37482=EDGE_CURVE('',#31077,#31069,#26040,.T.) ;
#37483=EDGE_CURVE('',#30969,#31078,#26041,.T.) ;
#37484=EDGE_CURVE('',#30960,#30969,#26042,.T.) ;
#37485=EDGE_CURVE('',#31077,#30962,#26043,.T.) ;
#37486=EDGE_CURVE('',#30961,#31078,#26044,.T.) ;
#37487=EDGE_CURVE('',#31025,#31006,#26045,.T.) ;
#37488=EDGE_CURVE('',#31014,#31025,#26046,.T.) ;
#37489=EDGE_CURVE('',#31006,#31014,#26047,.T.) ;
#37490=EDGE_CURVE('',#31032,#31180,#179,.T.) ;
#37491=EDGE_CURVE('',#31180,#31011,#4907,.T.) ;
#37492=EDGE_CURVE('',#31013,#31181,#4908,.T.) ;
#37493=EDGE_CURVE('',#31181,#30999,#180,.T.) ;
#37494=EDGE_CURVE('',#31026,#31005,#26048,.T.) ;
#37495=EDGE_CURVE('',#31021,#31182,#4909,.T.) ;
#37496=EDGE_CURVE('',#31182,#31032,#181,.T.) ;
#37497=EDGE_CURVE('',#31031,#31183,#182,.T.) ;
#37498=EDGE_CURVE('',#31183,#31022,#4910,.T.) ;
#37499=EDGE_CURVE('',#30999,#31184,#183,.T.) ;
#37500=EDGE_CURVE('',#31184,#31016,#4911,.T.) ;
#37501=EDGE_CURVE('',#31015,#31185,#4912,.T.) ;
#37502=EDGE_CURVE('',#31185,#31000,#184,.T.) ;
#37503=EDGE_CURVE('',#31026,#30997,#26049,.T.) ;
#37504=EDGE_CURVE('',#30996,#31005,#26050,.T.) ;
#37505=EDGE_CURVE('',#31186,#30997,#9194,.T.) ;
#37506=EDGE_CURVE('',#31027,#31186,#26051,.T.) ;
#37507=EDGE_CURVE('',#31187,#31186,#26052,.T.) ;
#37508=EDGE_CURVE('',#31027,#31187,#26053,.T.) ;
#37509=EDGE_CURVE('',#31010,#31188,#4913,.T.) ;
#37510=EDGE_CURVE('',#31188,#31031,#185,.T.) ;
#37511=EDGE_CURVE('',#31007,#31030,#26054,.T.) ;
#37512=EDGE_CURVE('',#31000,#31189,#186,.T.) ;
#37513=EDGE_CURVE('',#31189,#31008,#4914,.T.) ;
#37514=EDGE_CURVE('',#31001,#31007,#26055,.T.) ;
#37515=EDGE_CURVE('',#31190,#31004,#26056,.T.) ;
#37516=EDGE_CURVE('',#30996,#31190,#9195,.T.) ;
#37517=EDGE_CURVE('',#30985,#30998,#4915,.T.) ;
#37518=EDGE_CURVE('',#31186,#30983,#26057,.T.) ;
#37519=EDGE_CURVE('',#31187,#30984,#26058,.T.) ;
#37520=EDGE_CURVE('',#31191,#31187,#9196,.T.) ;
#37521=EDGE_CURVE('',#31028,#31191,#26059,.T.) ;
#37522=EDGE_CURVE('',#31001,#31030,#26060,.T.) ;
#37523=EDGE_CURVE('',#31190,#31192,#26061,.T.) ;
#37524=EDGE_CURVE('',#31192,#31004,#26062,.T.) ;
#37525=EDGE_CURVE('',#30991,#31190,#26063,.T.) ;
#37526=EDGE_CURVE('',#31191,#30988,#26064,.T.) ;
#37527=EDGE_CURVE('',#31193,#31191,#26065,.T.) ;
#37528=EDGE_CURVE('',#31028,#31193,#26066,.T.) ;
#37529=EDGE_CURVE('',#31002,#31029,#26067,.T.) ;
#37530=EDGE_CURVE('',#31194,#31003,#26068,.T.) ;
#37531=EDGE_CURVE('',#31192,#31194,#9197,.T.) ;
#37532=EDGE_CURVE('',#30992,#31192,#26069,.T.) ;
#37533=EDGE_CURVE('',#31193,#30987,#26070,.T.) ;
#37534=EDGE_CURVE('',#30993,#31193,#9198,.T.) ;
#37535=EDGE_CURVE('',#31029,#30993,#26071,.T.) ;
#37536=EDGE_CURVE('',#31002,#30995,#26072,.T.) ;
#37537=EDGE_CURVE('',#31194,#31195,#26073,.T.) ;
#37538=EDGE_CURVE('',#31195,#31003,#26074,.T.) ;
#37539=EDGE_CURVE('',#30990,#31194,#26075,.T.) ;
#37540=EDGE_CURVE('',#30994,#30986,#4916,.T.) ;
#37541=EDGE_CURVE('',#31195,#30995,#9199,.T.) ;
#37542=EDGE_CURVE('',#30989,#31195,#26076,.T.) ;
#37543=EDGE_CURVE('',#31043,#31047,#26077,.T.) ;
#37544=EDGE_CURVE('',#31043,#31051,#26078,.T.) ;
#37545=EDGE_CURVE('',#31051,#31047,#26079,.T.) ;
#37546=EDGE_CURVE('',#31046,#30963,#26080,.T.) ;
#37547=EDGE_CURVE('',#31052,#31046,#26081,.T.) ;
#37548=EDGE_CURVE('',#31044,#31050,#26082,.T.) ;
#37549=EDGE_CURVE('',#30875,#31041,#26083,.T.) ;
#37550=EDGE_CURVE('',#30846,#30876,#26084,.T.) ;
#37551=EDGE_CURVE('',#30849,#30875,#26085,.T.) ;
#37552=EDGE_CURVE('',#31052,#30964,#26086,.T.) ;
#37553=EDGE_CURVE('',#31044,#31048,#26087,.T.) ;
#37554=EDGE_CURVE('',#31048,#31050,#26088,.T.) ;
#37555=EDGE_CURVE('',#30849,#31042,#26089,.T.) ;
#37556=EDGE_CURVE('',#31053,#30982,#26090,.T.) ;
#37557=EDGE_CURVE('',#31049,#31053,#26091,.T.) ;
#37558=EDGE_CURVE('',#31045,#30844,#26092,.T.) ;
#37559=EDGE_CURVE('',#30843,#31045,#26093,.T.) ;
#37560=EDGE_CURVE('',#30881,#30845,#26094,.T.) ;
#37561=EDGE_CURVE('',#30882,#30852,#26095,.T.) ;
#37562=EDGE_CURVE('',#31064,#30882,#26096,.T.) ;
#37563=EDGE_CURVE('',#31060,#31063,#26097,.T.) ;
#37564=EDGE_CURVE('',#31049,#30981,#26098,.T.) ;
#37565=EDGE_CURVE('',#31065,#30852,#26099,.T.) ;
#37566=EDGE_CURVE('',#31060,#31054,#26100,.T.) ;
#37567=EDGE_CURVE('',#31054,#31063,#26101,.T.) ;
#37568=EDGE_CURVE('',#30842,#30980,#187,.T.) ;
#37569=EDGE_CURVE('',#31066,#30840,#26102,.T.) ;
#37570=EDGE_CURVE('',#31062,#31059,#26103,.T.) ;
#37571=EDGE_CURVE('',#30838,#31066,#26104,.T.) ;
#37572=EDGE_CURVE('',#31055,#31062,#26105,.T.) ;
#37573=EDGE_CURVE('',#31061,#31057,#26106,.T.) ;
#37574=EDGE_CURVE('',#30975,#31061,#26107,.T.) ;
#37575=EDGE_CURVE('',#30850,#30980,#26108,.T.) ;
#37576=EDGE_CURVE('',#31196,#30839,#26109,.T.) ;
#37577=EDGE_CURVE('',#31055,#31059,#26110,.T.) ;
#37578=EDGE_CURVE('',#30976,#31057,#26111,.T.) ;
#37579=EDGE_CURVE('',#30851,#30979,#26112,.T.) ;
#37580=EDGE_CURVE('',#31056,#31058,#26113,.T.) ;
#37581=EDGE_CURVE('',#30977,#31056,#26114,.T.) ;
#37582=EDGE_CURVE('',#30836,#30979,#188,.T.) ;
#37583=EDGE_CURVE('',#30978,#31058,#26115,.T.) ;
#37584=EDGE_CURVE('',#30855,#31136,#189,.T.) ;
#37585=EDGE_CURVE('',#31139,#31135,#26116,.T.) ;
#37586=EDGE_CURVE('',#31134,#31140,#26117,.T.) ;
#37587=EDGE_CURVE('',#31137,#31020,#190,.T.) ;
#37588=EDGE_CURVE('',#31132,#31157,#26118,.T.) ;
#37589=EDGE_CURVE('',#31144,#31171,#26119,.T.) ;
#37590=EDGE_CURVE('',#31145,#31170,#26120,.T.) ;
#37591=EDGE_CURVE('',#31131,#30858,#191,.T.) ;
#37592=EDGE_CURVE('',#31126,#31138,#26121,.T.) ;
#37593=EDGE_CURVE('',#31156,#31133,#26122,.T.) ;
#37594=EDGE_CURVE('',#31145,#31149,#26123,.T.) ;
#37595=EDGE_CURVE('',#31149,#31170,#26124,.T.) ;
#37596=EDGE_CURVE('',#31141,#31127,#26125,.T.) ;
#37597=EDGE_CURVE('',#31172,#31151,#26126,.T.) ;
#37598=EDGE_CURVE('',#31173,#31150,#26127,.T.) ;
#37599=EDGE_CURVE('',#31146,#31173,#26128,.T.) ;
#37600=EDGE_CURVE('',#31142,#31148,#26129,.T.) ;
#37601=EDGE_CURVE('',#31168,#31143,#26130,.T.) ;
#37602=EDGE_CURVE('',#31169,#31142,#26131,.T.) ;
#37603=EDGE_CURVE('',#31146,#31150,#26132,.T.) ;
#37604=EDGE_CURVE('',#31169,#31148,#26133,.T.) ;
#37605=EDGE_CURVE('',#31147,#31153,#26134,.T.) ;
#37606=EDGE_CURVE('',#31166,#31147,#26135,.T.) ;
#37607=EDGE_CURVE('',#31166,#31153,#26136,.T.) ;
#37608=EDGE_CURVE('',#31152,#31167,#26137,.T.) ;
#37609=EDGE_CURVE('',#31128,#31155,#26138,.T.) ;
#37610=EDGE_CURVE('',#31129,#31154,#26139,.T.) ;
#37611=EDGE_CURVE('',#31023,#31130,#192,.T.) ;
#37612=EDGE_CURVE('',#31121,#31122,#26140,.T.) ;
#37613=EDGE_CURVE('',#31125,#31120,#26141,.T.) ;
#37614=EDGE_CURVE('',#31108,#31159,#26142,.T.) ;
#37615=EDGE_CURVE('',#31109,#31158,#26143,.T.) ;
#37616=EDGE_CURVE('',#31160,#31115,#26144,.T.) ;
#37617=EDGE_CURVE('',#31161,#31114,#26145,.T.) ;
#37618=EDGE_CURVE('',#31158,#31113,#26146,.T.) ;
#37619=EDGE_CURVE('',#31110,#31161,#26147,.T.) ;
#37620=EDGE_CURVE('',#31109,#31113,#26148,.T.) ;
#37621=EDGE_CURVE('',#31123,#31118,#26149,.T.) ;
#37622=EDGE_CURVE('',#31119,#31124,#26150,.T.) ;
#37623=EDGE_CURVE('',#31110,#31114,#26151,.T.) ;
#37624=EDGE_CURVE('',#31106,#31112,#26152,.T.) ;
#37625=EDGE_CURVE('',#31164,#31107,#26153,.T.) ;
#37626=EDGE_CURVE('',#31165,#31106,#26154,.T.) ;
#37627=EDGE_CURVE('',#31116,#31163,#26155,.T.) ;
#37628=EDGE_CURVE('',#31117,#31162,#26156,.T.) ;
#37629=EDGE_CURVE('',#31111,#31117,#26157,.T.) ;
#37630=EDGE_CURVE('',#31165,#31112,#26158,.T.) ;
#37631=EDGE_CURVE('',#31111,#31162,#26159,.T.) ;
#37632=EDGE_CURVE('',#30869,#30868,#26160,.T.) ;
#37633=EDGE_CURVE('',#31095,#30870,#193,.T.) ;
#37634=EDGE_CURVE('',#31096,#30869,#26161,.T.) ;
#37635=EDGE_CURVE('',#31096,#30868,#26162,.T.) ;
#37636=EDGE_CURVE('',#30867,#30864,#26163,.T.) ;
#37637=EDGE_CURVE('',#31093,#30867,#26164,.T.) ;
#37638=EDGE_CURVE('',#31093,#30864,#26165,.T.) ;
#37639=EDGE_CURVE('',#30863,#31094,#194,.T.) ;
#37640=EDGE_CURVE('',#30825,#31104,#4917,.T.) ;
#37641=EDGE_CURVE('',#30952,#31103,#26166,.T.) ;
#37642=EDGE_CURVE('',#30949,#30952,#26167,.T.) ;
#37643=EDGE_CURVE('',#30949,#31103,#26168,.T.) ;
#37644=EDGE_CURVE('',#30950,#31105,#26169,.T.) ;
#37645=EDGE_CURVE('',#30948,#30950,#26170,.T.) ;
#37646=EDGE_CURVE('',#30948,#31105,#26171,.T.) ;
#37647=EDGE_CURVE('',#30829,#30945,#4918,.T.) ;
#37648=EDGE_CURVE('',#31017,#30854,#26172,.T.) ;
#37649=EDGE_CURVE('',#30853,#31018,#26173,.T.) ;
#37650=EDGE_CURVE('',#31179,#30887,#26174,.T.) ;
#37651=EDGE_CURVE('',#31176,#30888,#26175,.T.) ;
#37652=EDGE_CURVE('',#30887,#31177,#26176,.T.) ;
#37653=EDGE_CURVE('',#30888,#31174,#26177,.T.) ;
#37654=EDGE_CURVE('',#31011,#31021,#26178,.T.) ;
#37655=EDGE_CURVE('',#31012,#30854,#26179,.T.) ;
#37656=EDGE_CURVE('',#31012,#31017,#26180,.T.) ;
#37657=EDGE_CURVE('',#31013,#31016,#26181,.T.) ;
#37658=EDGE_CURVE('',#31008,#31015,#26182,.T.) ;
#37659=EDGE_CURVE('',#31009,#31018,#26183,.T.) ;
#37660=EDGE_CURVE('',#31009,#30853,#26184,.T.) ;
#37661=EDGE_CURVE('',#31010,#31022,#26185,.T.) ;
#37662=EDGE_CURVE('',#30862,#31098,#195,.T.) ;
#37663=EDGE_CURVE('',#31094,#31097,#26186,.T.) ;
#37664=EDGE_CURVE('',#31095,#31102,#26187,.T.) ;
#37665=EDGE_CURVE('',#31197,#31101,#196,.T.) ;
#37666=EDGE_CURVE('',#31198,#31197,#197,.T.) ;
#37667=EDGE_CURVE('',#31199,#31198,#198,.T.) ;
#37668=EDGE_CURVE('',#30871,#31199,#199,.T.) ;
#37669=EDGE_CURVE('',#30953,#30872,#4919,.T.) ;
#37670=EDGE_CURVE('',#30954,#31101,#26188,.T.) ;
#37671=EDGE_CURVE('',#30828,#30946,#200,.T.) ;
#37672=EDGE_CURVE('',#30955,#31100,#26189,.T.) ;
#37673=EDGE_CURVE('',#30951,#30956,#4920,.T.) ;
#37674=EDGE_CURVE('',#31099,#31104,#26190,.T.) ;
#37675=EDGE_CURVE('',#31200,#31100,#201,.T.) ;
#37676=EDGE_CURVE('',#31201,#31200,#202,.T.) ;
#37677=EDGE_CURVE('',#30824,#31201,#203,.T.) ;
#37678=EDGE_CURVE('',#30881,#31175,#26191,.T.) ;
#37679=EDGE_CURVE('',#30847,#31175,#26192,.T.) ;
#37680=EDGE_CURVE('',#31176,#31174,#26193,.T.) ;
#37681=EDGE_CURVE('',#31144,#31140,#26194,.T.) ;
#37682=EDGE_CURVE('',#31171,#31134,#26195,.T.) ;
#37683=EDGE_CURVE('',#31141,#31143,#26196,.T.) ;
#37684=EDGE_CURVE('',#31172,#31133,#26197,.T.) ;
#37685=EDGE_CURVE('',#31127,#31168,#26198,.T.) ;
#37686=EDGE_CURVE('',#31151,#31156,#26199,.T.) ;
#37687=EDGE_CURVE('',#31128,#31167,#26200,.T.) ;
#37688=EDGE_CURVE('',#31152,#31155,#26201,.T.) ;
#37689=EDGE_CURVE('',#31108,#31122,#26202,.T.) ;
#37690=EDGE_CURVE('',#31159,#31121,#26203,.T.) ;
#37691=EDGE_CURVE('',#31123,#31107,#26204,.T.) ;
#37692=EDGE_CURVE('',#31160,#31120,#26205,.T.) ;
#37693=EDGE_CURVE('',#31118,#31164,#26206,.T.) ;
#37694=EDGE_CURVE('',#31115,#31125,#26207,.T.) ;
#37695=EDGE_CURVE('',#31119,#31163,#26208,.T.) ;
#37696=EDGE_CURVE('',#31116,#31124,#26209,.T.) ;
#37697=EDGE_CURVE('',#31178,#30876,#26210,.T.) ;
#37698=EDGE_CURVE('',#31178,#30848,#26211,.T.) ;
#37699=EDGE_CURVE('',#31179,#31177,#26212,.T.) ;
#37700=EDGE_CURVE('',#30943,#30947,#4921,.T.) ;
#37701=EDGE_CURVE('',#30944,#30827,#26213,.T.) ;
#37702=EDGE_CURVE('',#30941,#31098,#26214,.T.) ;
#37703=EDGE_CURVE('',#30942,#30861,#4922,.T.) ;
#37704=EDGE_CURVE('',#31202,#31203,#204,.T.) ;
#37705=EDGE_CURVE('',#31203,#31204,#4923,.T.) ;
#37706=EDGE_CURVE('',#31204,#31205,#26215,.T.) ;
#37707=EDGE_CURVE('',#31206,#31205,#4924,.T.) ;
#37708=EDGE_CURVE('',#31202,#31206,#205,.T.) ;
#37709=EDGE_CURVE('',#31207,#31208,#206,.T.) ;
#37710=EDGE_CURVE('',#31208,#31209,#26216,.T.) ;
#37711=EDGE_CURVE('',#31210,#31209,#4925,.T.) ;
#37712=EDGE_CURVE('',#31211,#31210,#26217,.T.) ;
#37713=EDGE_CURVE('',#31207,#31211,#4926,.T.) ;
#37714=EDGE_CURVE('',#31212,#31212,#26218,.T.) ;
#37715=EDGE_CURVE('',#31212,#31213,#26219,.T.) ;
#37716=EDGE_CURVE('',#31213,#31213,#26220,.T.) ;
#37717=EDGE_CURVE('',#31214,#31214,#26221,.T.) ;
#37718=EDGE_CURVE('',#31214,#31215,#26222,.T.) ;
#37719=EDGE_CURVE('',#31215,#31215,#26223,.T.) ;
#37720=EDGE_CURVE('',#31216,#31217,#26224,.T.) ;
#37721=EDGE_CURVE('',#31218,#31216,#9200,.T.) ;
#37722=EDGE_CURVE('',#31218,#31219,#26225,.T.) ;
#37723=EDGE_CURVE('',#31219,#31220,#26226,.T.) ;
#37724=EDGE_CURVE('',#31217,#31220,#9201,.T.) ;
#37725=EDGE_CURVE('',#31221,#31222,#26227,.T.) ;
#37726=EDGE_CURVE('',#31223,#31221,#9202,.T.) ;
#37727=EDGE_CURVE('',#31223,#31224,#26228,.T.) ;
#37728=EDGE_CURVE('',#31222,#31224,#9203,.T.) ;
#37729=EDGE_CURVE('',#31225,#31226,#26229,.T.) ;
#37730=EDGE_CURVE('',#31225,#31227,#26230,.T.) ;
#37731=EDGE_CURVE('',#31228,#31227,#26231,.T.) ;
#37732=EDGE_CURVE('',#31228,#31226,#26232,.T.) ;
#37733=EDGE_CURVE('',#31213,#31214,#9204,.T.) ;
#37734=EDGE_CURVE('',#31226,#31229,#9205,.T.) ;
#37735=EDGE_CURVE('',#31229,#31223,#26233,.T.) ;
#37736=EDGE_CURVE('',#31230,#31221,#207,.T.) ;
#37737=EDGE_CURVE('',#31230,#31231,#26234,.T.) ;
#37738=EDGE_CURVE('',#31217,#31231,#208,.T.) ;
#37739=EDGE_CURVE('',#31220,#31232,#26235,.T.) ;
#37740=EDGE_CURVE('',#31232,#31225,#9206,.T.) ;
#37741=EDGE_CURVE('',#31233,#31234,#9207,.T.) ;
#37742=EDGE_CURVE('',#31234,#31235,#9208,.T.) ;
#37743=EDGE_CURVE('',#31235,#31236,#209,.T.) ;
#37744=EDGE_CURVE('',#31236,#31237,#9209,.T.) ;
#37745=EDGE_CURVE('',#31237,#31238,#4927,.T.) ;
#37746=EDGE_CURVE('',#31238,#31233,#9210,.T.) ;
#37747=EDGE_CURVE('',#31239,#31240,#9211,.T.) ;
#37748=EDGE_CURVE('',#31240,#31241,#9212,.T.) ;
#37749=EDGE_CURVE('',#31241,#31242,#210,.T.) ;
#37750=EDGE_CURVE('',#31242,#31243,#211,.T.) ;
#37751=EDGE_CURVE('',#31243,#31244,#9213,.T.) ;
#37752=EDGE_CURVE('',#31244,#31239,#9214,.T.) ;
#37753=EDGE_CURVE('',#31245,#31246,#9215,.T.) ;
#37754=EDGE_CURVE('',#31246,#31247,#9216,.T.) ;
#37755=EDGE_CURVE('',#31247,#31248,#9217,.T.) ;
#37756=EDGE_CURVE('',#31248,#31245,#9218,.T.) ;
#37757=EDGE_CURVE('',#31249,#31250,#9219,.T.) ;
#37758=EDGE_CURVE('',#31250,#31251,#212,.T.) ;
#37759=EDGE_CURVE('',#31251,#31252,#213,.T.) ;
#37760=EDGE_CURVE('',#31252,#31253,#9220,.T.) ;
#37761=EDGE_CURVE('',#31253,#31254,#9221,.T.) ;
#37762=EDGE_CURVE('',#31254,#31249,#9222,.T.) ;
#37763=EDGE_CURVE('',#31255,#31256,#9223,.T.) ;
#37764=EDGE_CURVE('',#31256,#31257,#9224,.T.) ;
#37765=EDGE_CURVE('',#31257,#31258,#9225,.T.) ;
#37766=EDGE_CURVE('',#31258,#31255,#9226,.T.) ;
#37767=EDGE_CURVE('',#31259,#31260,#9227,.T.) ;
#37768=EDGE_CURVE('',#31259,#31261,#9228,.T.) ;
#37769=EDGE_CURVE('',#31261,#31262,#9229,.T.) ;
#37770=EDGE_CURVE('',#31262,#31260,#9230,.T.) ;
#37771=EDGE_CURVE('',#31263,#31264,#9231,.T.) ;
#37772=EDGE_CURVE('',#31263,#31265,#9232,.T.) ;
#37773=EDGE_CURVE('',#31265,#31266,#9233,.T.) ;
#37774=EDGE_CURVE('',#31266,#31267,#9234,.T.) ;
#37775=EDGE_CURVE('',#31267,#31268,#26236,.T.) ;
#37776=EDGE_CURVE('',#31268,#31264,#9235,.T.) ;
#37777=EDGE_CURVE('',#31269,#31270,#9236,.T.) ;
#37778=EDGE_CURVE('',#31269,#31240,#26237,.T.) ;
#37779=EDGE_CURVE('',#31239,#31246,#26238,.T.) ;
#37780=EDGE_CURVE('',#31245,#31254,#26239,.T.) ;
#37781=EDGE_CURVE('',#31253,#31271,#26240,.T.) ;
#37782=EDGE_CURVE('',#31272,#31271,#9237,.T.) ;
#37783=EDGE_CURVE('',#31272,#31273,#26241,.T.) ;
#37784=EDGE_CURVE('',#31274,#31273,#9238,.T.) ;
#37785=EDGE_CURVE('',#31274,#31275,#26242,.T.) ;
#37786=EDGE_CURVE('',#31275,#31276,#9239,.T.) ;
#37787=EDGE_CURVE('',#31276,#31277,#26243,.T.) ;
#37788=EDGE_CURVE('',#31278,#31277,#9240,.T.) ;
#37789=EDGE_CURVE('',#31278,#31279,#26244,.T.) ;
#37790=EDGE_CURVE('',#31279,#31280,#9241,.T.) ;
#37791=EDGE_CURVE('',#31280,#31281,#26245,.T.) ;
#37792=EDGE_CURVE('',#31282,#31281,#9242,.T.) ;
#37793=EDGE_CURVE('',#31282,#31258,#26246,.T.) ;
#37794=EDGE_CURVE('',#31257,#31283,#26247,.T.) ;
#37795=EDGE_CURVE('',#31283,#31284,#9243,.T.) ;
#37796=EDGE_CURVE('',#31284,#31266,#26248,.T.) ;
#37797=EDGE_CURVE('',#31265,#31285,#26249,.T.) ;
#37798=EDGE_CURVE('',#31286,#31285,#9244,.T.) ;
#37799=EDGE_CURVE('',#31287,#31286,#9245,.T.) ;
#37800=EDGE_CURVE('',#31287,#31288,#26250,.T.) ;
#37801=EDGE_CURVE('',#31289,#31288,#9246,.T.) ;
#37802=EDGE_CURVE('',#31289,#31290,#26251,.T.) ;
#37803=EDGE_CURVE('',#31291,#31290,#9247,.T.) ;
#37804=EDGE_CURVE('',#31291,#31270,#26252,.T.) ;
#37805=EDGE_CURVE('',#31292,#31293,#9248,.T.) ;
#37806=EDGE_CURVE('',#31293,#31294,#26253,.T.) ;
#37807=EDGE_CURVE('',#31294,#31295,#9249,.T.) ;
#37808=EDGE_CURVE('',#31295,#31296,#26254,.T.) ;
#37809=EDGE_CURVE('',#31296,#31297,#9250,.T.) ;
#37810=EDGE_CURVE('',#31297,#31298,#26255,.T.) ;
#37811=EDGE_CURVE('',#31298,#31299,#9251,.T.) ;
#37812=EDGE_CURVE('',#31299,#31300,#26256,.T.) ;
#37813=EDGE_CURVE('',#31300,#31301,#9252,.T.) ;
#37814=EDGE_CURVE('',#31301,#31302,#9253,.T.) ;
#37815=EDGE_CURVE('',#31302,#31263,#26257,.T.) ;
#37816=EDGE_CURVE('',#31264,#31303,#26258,.T.) ;
#37817=EDGE_CURVE('',#31303,#31304,#9254,.T.) ;
#37818=EDGE_CURVE('',#31304,#31259,#26259,.T.) ;
#37819=EDGE_CURVE('',#31260,#31305,#26260,.T.) ;
#37820=EDGE_CURVE('',#31306,#31305,#9255,.T.) ;
#37821=EDGE_CURVE('',#31306,#31307,#26261,.T.) ;
#37822=EDGE_CURVE('',#31308,#31307,#9256,.T.) ;
#37823=EDGE_CURVE('',#31308,#31309,#26262,.T.) ;
#37824=EDGE_CURVE('',#31309,#31310,#9257,.T.) ;
#37825=EDGE_CURVE('',#31310,#31311,#26263,.T.) ;
#37826=EDGE_CURVE('',#31312,#31311,#9258,.T.) ;
#37827=EDGE_CURVE('',#31312,#31313,#26264,.T.) ;
#37828=EDGE_CURVE('',#31314,#31313,#9259,.T.) ;
#37829=EDGE_CURVE('',#31314,#31315,#26265,.T.) ;
#37830=EDGE_CURVE('',#31315,#31316,#9260,.T.) ;
#37831=EDGE_CURVE('',#31316,#31317,#26266,.T.) ;
#37832=EDGE_CURVE('',#31317,#31318,#9261,.T.) ;
#37833=EDGE_CURVE('',#31318,#31319,#26267,.T.) ;
#37834=EDGE_CURVE('',#31319,#31320,#9262,.T.) ;
#37835=EDGE_CURVE('',#31320,#31292,#26268,.T.) ;
#37836=EDGE_CURVE('',#31288,#31299,#9263,.T.) ;
#37837=EDGE_CURVE('',#31298,#31289,#9264,.T.) ;
#37838=EDGE_CURVE('',#31290,#31297,#9265,.T.) ;
#37839=EDGE_CURVE('',#31296,#31291,#9266,.T.) ;
#37840=EDGE_CURVE('',#31321,#31322,#214,.T.) ;
#37841=EDGE_CURVE('',#31322,#31269,#9267,.T.) ;
#37842=EDGE_CURVE('',#31270,#31295,#9268,.T.) ;
#37843=EDGE_CURVE('',#31294,#31323,#9269,.T.) ;
#37844=EDGE_CURVE('',#31323,#31324,#215,.T.) ;
#37845=EDGE_CURVE('',#31324,#31321,#9270,.T.) ;
#37846=EDGE_CURVE('',#31325,#31326,#216,.T.) ;
#37847=EDGE_CURVE('',#31326,#31327,#4928,.T.) ;
#37848=EDGE_CURVE('',#31327,#31293,#9271,.T.) ;
#37849=EDGE_CURVE('',#31292,#31328,#9272,.T.) ;
#37850=EDGE_CURVE('',#31328,#31325,#9273,.T.) ;
#37851=EDGE_CURVE('',#31329,#31330,#9274,.T.) ;
#37852=EDGE_CURVE('',#31330,#31320,#9275,.T.) ;
#37853=EDGE_CURVE('',#31319,#31329,#9276,.T.) ;
#37854=EDGE_CURVE('',#31331,#31202,#217,.T.) ;
#37855=EDGE_CURVE('',#31206,#31332,#9277,.T.) ;
#37856=EDGE_CURVE('',#31332,#31318,#9278,.T.) ;
#37857=EDGE_CURVE('',#31317,#31331,#9279,.T.) ;
#37858=EDGE_CURVE('',#31271,#31333,#9280,.T.) ;
#37859=EDGE_CURVE('',#31333,#31334,#218,.T.) ;
#37860=EDGE_CURVE('',#31334,#31335,#9281,.T.) ;
#37861=EDGE_CURVE('',#31335,#31336,#219,.T.) ;
#37862=EDGE_CURVE('',#31336,#31316,#9282,.T.) ;
#37863=EDGE_CURVE('',#31315,#31337,#9283,.T.) ;
#37864=EDGE_CURVE('',#31337,#31338,#9284,.T.) ;
#37865=EDGE_CURVE('',#31339,#31338,#26269,.T.) ;
#37866=EDGE_CURVE('',#31339,#31340,#9285,.T.) ;
#37867=EDGE_CURVE('',#31341,#31340,#26270,.T.) ;
#37868=EDGE_CURVE('',#31341,#31342,#9286,.T.) ;
#37869=EDGE_CURVE('',#31342,#31272,#9287,.T.) ;
#37870=EDGE_CURVE('',#31343,#31344,#26271,.T.) ;
#37871=EDGE_CURVE('',#31343,#31278,#9288,.T.) ;
#37872=EDGE_CURVE('',#31277,#31345,#9289,.T.) ;
#37873=EDGE_CURVE('',#31346,#31345,#26272,.T.) ;
#37874=EDGE_CURVE('',#31346,#31347,#26273,.T.) ;
#37875=EDGE_CURVE('',#31348,#31347,#26274,.T.) ;
#37876=EDGE_CURVE('',#31348,#31349,#9290,.T.) ;
#37877=EDGE_CURVE('',#31349,#31350,#9291,.T.) ;
#37878=EDGE_CURVE('',#31350,#31351,#9292,.T.) ;
#37879=EDGE_CURVE('',#31352,#31351,#26275,.T.) ;
#37880=EDGE_CURVE('',#31352,#31353,#26276,.T.) ;
#37881=EDGE_CURVE('',#31354,#31353,#26277,.T.) ;
#37882=EDGE_CURVE('',#31354,#31310,#9293,.T.) ;
#37883=EDGE_CURVE('',#31309,#31355,#9294,.T.) ;
#37884=EDGE_CURVE('',#31356,#31355,#26278,.T.) ;
#37885=EDGE_CURVE('',#31356,#31357,#26279,.T.) ;
#37886=EDGE_CURVE('',#31358,#31357,#26280,.T.) ;
#37887=EDGE_CURVE('',#31358,#31359,#9295,.T.) ;
#37888=EDGE_CURVE('',#31359,#31360,#26281,.T.) ;
#37889=EDGE_CURVE('',#31360,#31361,#9296,.T.) ;
#37890=EDGE_CURVE('',#31362,#31361,#26282,.T.) ;
#37891=EDGE_CURVE('',#31362,#31344,#26283,.T.) ;
#37892=EDGE_CURVE('',#31363,#31364,#26284,.T.) ;
#37893=EDGE_CURVE('',#31363,#31365,#9297,.T.) ;
#37894=EDGE_CURVE('',#31286,#31365,#9298,.T.) ;
#37895=EDGE_CURVE('',#31285,#31302,#9299,.T.) ;
#37896=EDGE_CURVE('',#31366,#31301,#9300,.T.) ;
#37897=EDGE_CURVE('',#31366,#31367,#9301,.T.) ;
#37898=EDGE_CURVE('',#31368,#31367,#26285,.T.) ;
#37899=EDGE_CURVE('',#31368,#31364,#9302,.T.) ;
#37900=EDGE_CURVE('',#31369,#31370,#26286,.T.) ;
#37901=EDGE_CURVE('',#31369,#31366,#9303,.T.) ;
#37902=EDGE_CURVE('',#31300,#31287,#9304,.T.) ;
#37903=EDGE_CURVE('',#31365,#31371,#9305,.T.) ;
#37904=EDGE_CURVE('',#31372,#31371,#26287,.T.) ;
#37905=EDGE_CURVE('',#31372,#31370,#9306,.T.) ;
#37906=EDGE_CURVE('',#31373,#31374,#9307,.T.) ;
#37907=EDGE_CURVE('',#31374,#31375,#9308,.T.) ;
#37908=EDGE_CURVE('',#31373,#31375,#26288,.T.) ;
#37909=EDGE_CURVE('',#31376,#31377,#26289,.T.) ;
#37910=EDGE_CURVE('',#31376,#31378,#9309,.T.) ;
#37911=EDGE_CURVE('',#31378,#31377,#9310,.T.) ;
#37912=EDGE_CURVE('',#31379,#31380,#9311,.T.) ;
#37913=EDGE_CURVE('',#31380,#31381,#9312,.T.) ;
#37914=EDGE_CURVE('',#31381,#31382,#9313,.T.) ;
#37915=EDGE_CURVE('',#31382,#31383,#9314,.T.) ;
#37916=EDGE_CURVE('',#31383,#31384,#9315,.T.) ;
#37917=EDGE_CURVE('',#31384,#31385,#9316,.T.) ;
#37918=EDGE_CURVE('',#31385,#31386,#9317,.T.) ;
#37919=EDGE_CURVE('',#31386,#31379,#9318,.T.) ;
#37920=EDGE_CURVE('',#31387,#31388,#9319,.T.) ;
#37921=EDGE_CURVE('',#31388,#31389,#9320,.T.) ;
#37922=EDGE_CURVE('',#31389,#31390,#9321,.T.) ;
#37923=EDGE_CURVE('',#31390,#31387,#9322,.T.) ;
#37924=EDGE_CURVE('',#31391,#31392,#9323,.T.) ;
#37925=EDGE_CURVE('',#31392,#31393,#9324,.T.) ;
#37926=EDGE_CURVE('',#31393,#31394,#9325,.T.) ;
#37927=EDGE_CURVE('',#31394,#31391,#9326,.T.) ;
#37928=EDGE_CURVE('',#31395,#31396,#9327,.T.) ;
#37929=EDGE_CURVE('',#31396,#31397,#9328,.T.) ;
#37930=EDGE_CURVE('',#31397,#31398,#9329,.T.) ;
#37931=EDGE_CURVE('',#31398,#31395,#9330,.T.) ;
#37932=EDGE_CURVE('',#31399,#31400,#220,.T.) ;
#37933=EDGE_CURVE('',#31400,#31401,#9331,.T.) ;
#37934=EDGE_CURVE('',#31401,#31402,#9332,.T.) ;
#37935=EDGE_CURVE('',#31402,#31403,#9333,.T.) ;
#37936=EDGE_CURVE('',#31403,#31404,#221,.T.) ;
#37937=EDGE_CURVE('',#31404,#31399,#9334,.T.) ;
#37938=EDGE_CURVE('',#31405,#31406,#9335,.T.) ;
#37939=EDGE_CURVE('',#31406,#31407,#9336,.T.) ;
#37940=EDGE_CURVE('',#31407,#31408,#9337,.T.) ;
#37941=EDGE_CURVE('',#31408,#31409,#9338,.T.) ;
#37942=EDGE_CURVE('',#31409,#31410,#9339,.T.) ;
#37943=EDGE_CURVE('',#31410,#31411,#9340,.T.) ;
#37944=EDGE_CURVE('',#31411,#31412,#9341,.T.) ;
#37945=EDGE_CURVE('',#31412,#31405,#9342,.T.) ;
#37946=EDGE_CURVE('',#31413,#31414,#9343,.T.) ;
#37947=EDGE_CURVE('',#31413,#31415,#26290,.T.) ;
#37948=EDGE_CURVE('',#31415,#31416,#9344,.T.) ;
#37949=EDGE_CURVE('',#31416,#31417,#26291,.T.) ;
#37950=EDGE_CURVE('',#31417,#31418,#9345,.T.) ;
#37951=EDGE_CURVE('',#31418,#31419,#26292,.T.) ;
#37952=EDGE_CURVE('',#31419,#31420,#9346,.T.) ;
#37953=EDGE_CURVE('',#31420,#31414,#26293,.T.) ;
#37954=EDGE_CURVE('',#31421,#31422,#26294,.T.) ;
#37955=EDGE_CURVE('',#31421,#31282,#9347,.T.) ;
#37956=EDGE_CURVE('',#31281,#31423,#9348,.T.) ;
#37957=EDGE_CURVE('',#31423,#31424,#26295,.T.) ;
#37958=EDGE_CURVE('',#31424,#31425,#9349,.T.) ;
#37959=EDGE_CURVE('',#31425,#31422,#26296,.T.) ;
#37960=EDGE_CURVE('',#31279,#31426,#9350,.T.) ;
#37961=EDGE_CURVE('',#31426,#31427,#9351,.T.) ;
#37962=EDGE_CURVE('',#31427,#31280,#9352,.T.) ;
#37963=EDGE_CURVE('',#31428,#31429,#9353,.T.) ;
#37964=EDGE_CURVE('',#31429,#31222,#9354,.T.) ;
#37965=EDGE_CURVE('',#31224,#31428,#9355,.T.) ;
#37966=EDGE_CURVE('',#31430,#31431,#26297,.T.) ;
#37967=EDGE_CURVE('',#31431,#31432,#9356,.T.) ;
#37968=EDGE_CURVE('',#31432,#31433,#26298,.T.) ;
#37969=EDGE_CURVE('',#31433,#31430,#9357,.T.) ;
#37970=EDGE_CURVE('',#31434,#31435,#26299,.T.) ;
#37971=EDGE_CURVE('',#31435,#31436,#9358,.T.) ;
#37972=EDGE_CURVE('',#31436,#31437,#26300,.T.) ;
#37973=EDGE_CURVE('',#31437,#31434,#9359,.T.) ;
#37974=EDGE_CURVE('',#31216,#31438,#9360,.T.) ;
#37975=EDGE_CURVE('',#31438,#31439,#9361,.T.) ;
#37976=EDGE_CURVE('',#31439,#31218,#9362,.T.) ;
#37977=EDGE_CURVE('',#31440,#31441,#9363,.T.) ;
#37978=EDGE_CURVE('',#31441,#31308,#9364,.T.) ;
#37979=EDGE_CURVE('',#31307,#31440,#9365,.T.) ;
#37980=EDGE_CURVE('',#31442,#31443,#26301,.T.) ;
#37981=EDGE_CURVE('',#31443,#31306,#9366,.T.) ;
#37982=EDGE_CURVE('',#31305,#31444,#9367,.T.) ;
#37983=EDGE_CURVE('',#31445,#31444,#26302,.T.) ;
#37984=EDGE_CURVE('',#31445,#31446,#26303,.T.) ;
#37985=EDGE_CURVE('',#31446,#31442,#9368,.T.) ;
#37986=EDGE_CURVE('',#31447,#31448,#26304,.T.) ;
#37987=EDGE_CURVE('',#31448,#31274,#9369,.T.) ;
#37988=EDGE_CURVE('',#31273,#31449,#9370,.T.) ;
#37989=EDGE_CURVE('',#31449,#31447,#9371,.T.) ;
#37990=EDGE_CURVE('',#31450,#31451,#9372,.T.) ;
#37991=EDGE_CURVE('',#31451,#31276,#9373,.T.) ;
#37992=EDGE_CURVE('',#31275,#31450,#9374,.T.) ;
#37993=EDGE_CURVE('',#31452,#31453,#26305,.T.) ;
#37994=EDGE_CURVE('',#31453,#31454,#9375,.T.) ;
#37995=EDGE_CURVE('',#31454,#31455,#26306,.T.) ;
#37996=EDGE_CURVE('',#31455,#31452,#9376,.T.) ;
#37997=EDGE_CURVE('',#31456,#31457,#9377,.T.) ;
#37998=EDGE_CURVE('',#31457,#31458,#9378,.T.) ;
#37999=EDGE_CURVE('',#31458,#31459,#9379,.T.) ;
#38000=EDGE_CURVE('',#31459,#31456,#9380,.T.) ;
#38001=EDGE_CURVE('',#31460,#31461,#26307,.T.) ;
#38002=EDGE_CURVE('',#31461,#31462,#9381,.T.) ;
#38003=EDGE_CURVE('',#31462,#31463,#26308,.T.) ;
#38004=EDGE_CURVE('',#31463,#31460,#9382,.T.) ;
#38005=EDGE_CURVE('',#31311,#31464,#9383,.T.) ;
#38006=EDGE_CURVE('',#31464,#31465,#9384,.T.) ;
#38007=EDGE_CURVE('',#31465,#31312,#9385,.T.) ;
#38008=EDGE_CURVE('',#31466,#31467,#9386,.T.) ;
#38009=EDGE_CURVE('',#31467,#31468,#9387,.T.) ;
#38010=EDGE_CURVE('',#31468,#31469,#9388,.T.) ;
#38011=EDGE_CURVE('',#31469,#31466,#9389,.T.) ;
#38012=EDGE_CURVE('',#31470,#31471,#9390,.T.) ;
#38013=EDGE_CURVE('',#31471,#31314,#9391,.T.) ;
#38014=EDGE_CURVE('',#31313,#31472,#9392,.T.) ;
#38015=EDGE_CURVE('',#31472,#31470,#26309,.T.) ;
#38016=EDGE_CURVE('',#31473,#31474,#9393,.T.) ;
#38017=EDGE_CURVE('',#31474,#31475,#9394,.T.) ;
#38018=EDGE_CURVE('',#31475,#31476,#9395,.T.) ;
#38019=EDGE_CURVE('',#31476,#31473,#9396,.T.) ;
#38020=EDGE_CURVE('',#31477,#31478,#4929,.T.) ;
#38021=EDGE_CURVE('',#31478,#31207,#9397,.T.) ;
#38022=EDGE_CURVE('',#31211,#31479,#9398,.T.) ;
#38023=EDGE_CURVE('',#31479,#31480,#4930,.T.) ;
#38024=EDGE_CURVE('',#31480,#31481,#9399,.T.) ;
#38025=EDGE_CURVE('',#31481,#31482,#4931,.T.) ;
#38026=EDGE_CURVE('',#31482,#31477,#9400,.T.) ;
#38027=EDGE_CURVE('',#31483,#31484,#9401,.T.) ;
#38028=EDGE_CURVE('',#31484,#31210,#9402,.T.) ;
#38029=EDGE_CURVE('',#31210,#31485,#9403,.T.) ;
#38030=EDGE_CURVE('',#31485,#31483,#9404,.T.) ;
#38031=EDGE_CURVE('',#31486,#31487,#9405,.T.) ;
#38032=EDGE_CURVE('',#31487,#31488,#9406,.T.) ;
#38033=EDGE_CURVE('',#31488,#31489,#9407,.T.) ;
#38034=EDGE_CURVE('',#31489,#31486,#9408,.T.) ;
#38035=EDGE_CURVE('',#31490,#31491,#9409,.T.) ;
#38036=EDGE_CURVE('',#31491,#31492,#9410,.T.) ;
#38037=EDGE_CURVE('',#31492,#31493,#9411,.T.) ;
#38038=EDGE_CURVE('',#31493,#31490,#9412,.T.) ;
#38039=EDGE_CURVE('',#31494,#31495,#9413,.T.) ;
#38040=EDGE_CURVE('',#31495,#31496,#9414,.T.) ;
#38041=EDGE_CURVE('',#31496,#31497,#9415,.T.) ;
#38042=EDGE_CURVE('',#31497,#31494,#9416,.T.) ;
#38043=EDGE_CURVE('',#31414,#31498,#9417,.T.) ;
#38044=EDGE_CURVE('',#31498,#31499,#9418,.T.) ;
#38045=EDGE_CURVE('',#31499,#31413,#9419,.T.) ;
#38046=EDGE_CURVE('',#31417,#31500,#9420,.T.) ;
#38047=EDGE_CURVE('',#31500,#31501,#9421,.T.) ;
#38048=EDGE_CURVE('',#31501,#31418,#9422,.T.) ;
#38049=EDGE_CURVE('',#31419,#31502,#9423,.T.) ;
#38050=EDGE_CURVE('',#31502,#31503,#9424,.T.) ;
#38051=EDGE_CURVE('',#31503,#31420,#9425,.T.) ;
#38052=EDGE_CURVE('',#31415,#31504,#9426,.T.) ;
#38053=EDGE_CURVE('',#31504,#31505,#9427,.T.) ;
#38054=EDGE_CURVE('',#31505,#31416,#9428,.T.) ;
#38055=EDGE_CURVE('',#31506,#31507,#9429,.T.) ;
#38056=EDGE_CURVE('',#31507,#31508,#9430,.T.) ;
#38057=EDGE_CURVE('',#31508,#31509,#9431,.T.) ;
#38058=EDGE_CURVE('',#31509,#31510,#26310,.T.) ;
#38059=EDGE_CURVE('',#31510,#31511,#9432,.T.) ;
#38060=EDGE_CURVE('',#31511,#31506,#26311,.T.) ;
#38061=EDGE_CURVE('',#31512,#31513,#9433,.T.) ;
#38062=EDGE_CURVE('',#31513,#31514,#9434,.T.) ;
#38063=EDGE_CURVE('',#31514,#31515,#9435,.T.) ;
#38064=EDGE_CURVE('',#31515,#31516,#26312,.T.) ;
#38065=EDGE_CURVE('',#31516,#31517,#9436,.T.) ;
#38066=EDGE_CURVE('',#31517,#31512,#26313,.T.) ;
#38067=EDGE_CURVE('',#31518,#31519,#9437,.T.) ;
#38068=EDGE_CURVE('',#31518,#31237,#26314,.T.) ;
#38069=EDGE_CURVE('',#31236,#31519,#26315,.T.) ;
#38070=EDGE_CURVE('',#31519,#31520,#9438,.T.) ;
#38071=EDGE_CURVE('',#31520,#31521,#9439,.T.) ;
#38072=EDGE_CURVE('',#31521,#31518,#9440,.T.) ;
#38073=EDGE_CURVE('',#31522,#31523,#9441,.T.) ;
#38074=EDGE_CURVE('',#31523,#31524,#9442,.T.) ;
#38075=EDGE_CURVE('',#31524,#31525,#9443,.T.) ;
#38076=EDGE_CURVE('',#31525,#31522,#9444,.T.) ;
#38077=EDGE_CURVE('',#31526,#31527,#9445,.T.) ;
#38078=EDGE_CURVE('',#31527,#31528,#9446,.T.) ;
#38079=EDGE_CURVE('',#31528,#31529,#9447,.T.) ;
#38080=EDGE_CURVE('',#31529,#31526,#9448,.T.) ;
#38081=EDGE_CURVE('',#31530,#31531,#9449,.T.) ;
#38082=EDGE_CURVE('',#31531,#31532,#9450,.T.) ;
#38083=EDGE_CURVE('',#31532,#31533,#9451,.T.) ;
#38084=EDGE_CURVE('',#31533,#31530,#9452,.T.) ;
#38085=EDGE_CURVE('',#31534,#31535,#9453,.T.) ;
#38086=EDGE_CURVE('',#31535,#31536,#9454,.T.) ;
#38087=EDGE_CURVE('',#31536,#31537,#9455,.T.) ;
#38088=EDGE_CURVE('',#31534,#31537,#9456,.T.) ;
#38089=EDGE_CURVE('',#31404,#31534,#26316,.T.) ;
#38090=EDGE_CURVE('',#31537,#31399,#26317,.T.) ;
#38091=EDGE_CURVE('',#31538,#31539,#9457,.T.) ;
#38092=EDGE_CURVE('',#31539,#31540,#9458,.T.) ;
#38093=EDGE_CURVE('',#31540,#31541,#9459,.T.) ;
#38094=EDGE_CURVE('',#31541,#31538,#9460,.T.) ;
#38095=EDGE_CURVE('',#31542,#31543,#9461,.T.) ;
#38096=EDGE_CURVE('',#31543,#31544,#9462,.T.) ;
#38097=EDGE_CURVE('',#31544,#31545,#9463,.T.) ;
#38098=EDGE_CURVE('',#31545,#31542,#9464,.T.) ;
#38099=EDGE_CURVE('',#31546,#31547,#9465,.T.) ;
#38100=EDGE_CURVE('',#31547,#31548,#9466,.T.) ;
#38101=EDGE_CURVE('',#31548,#31549,#9467,.T.) ;
#38102=EDGE_CURVE('',#31549,#31546,#9468,.T.) ;
#38103=EDGE_CURVE('',#31550,#31551,#9469,.T.) ;
#38104=EDGE_CURVE('',#31551,#31552,#9470,.T.) ;
#38105=EDGE_CURVE('',#31552,#31553,#9471,.T.) ;
#38106=EDGE_CURVE('',#31553,#31550,#9472,.T.) ;
#38107=EDGE_CURVE('',#31303,#31554,#9473,.T.) ;
#38108=EDGE_CURVE('',#31554,#31555,#26318,.T.) ;
#38109=EDGE_CURVE('',#31555,#31304,#9474,.T.) ;
#38110=EDGE_CURVE('',#31556,#31557,#26319,.T.) ;
#38111=EDGE_CURVE('',#31557,#31228,#26320,.T.) ;
#38112=EDGE_CURVE('',#31227,#31556,#26321,.T.) ;
#38113=EDGE_CURVE('',#31283,#31558,#9475,.T.) ;
#38114=EDGE_CURVE('',#31558,#31559,#26322,.T.) ;
#38115=EDGE_CURVE('',#31559,#31284,#9476,.T.) ;
#38116=EDGE_CURVE('',#31472,#31465,#26323,.T.) ;
#38117=EDGE_CURVE('',#31472,#31461,#26324,.T.) ;
#38118=EDGE_CURVE('',#31461,#31465,#26325,.T.) ;
#38119=EDGE_CURVE('',#31464,#31354,#26326,.T.) ;
#38120=EDGE_CURVE('',#31462,#31464,#26327,.T.) ;
#38121=EDGE_CURVE('',#31470,#31460,#26328,.T.) ;
#38122=EDGE_CURVE('',#31462,#31353,#26329,.T.) ;
#38123=EDGE_CURVE('',#31470,#31469,#26330,.T.) ;
#38124=EDGE_CURVE('',#31469,#31460,#26331,.T.) ;
#38125=EDGE_CURVE('',#31450,#31448,#26332,.T.) ;
#38126=EDGE_CURVE('',#31451,#31455,#26333,.T.) ;
#38127=EDGE_CURVE('',#31452,#31450,#26334,.T.) ;
#38128=EDGE_CURVE('',#31345,#31451,#26335,.T.) ;
#38129=EDGE_CURVE('',#31463,#31352,#26336,.T.) ;
#38130=EDGE_CURVE('',#31466,#31463,#26337,.T.) ;
#38131=EDGE_CURVE('',#31471,#31468,#26338,.T.) ;
#38132=EDGE_CURVE('',#31337,#31471,#26339,.T.) ;
#38133=EDGE_CURVE('',#31452,#31448,#26340,.T.) ;
#38134=EDGE_CURVE('',#31346,#31455,#26341,.T.) ;
#38135=EDGE_CURVE('',#31466,#31351,#26342,.T.) ;
#38136=EDGE_CURVE('',#31337,#31468,#26343,.T.) ;
#38137=EDGE_CURVE('',#31453,#31447,#26344,.T.) ;
#38138=EDGE_CURVE('',#31454,#31459,#26345,.T.) ;
#38139=EDGE_CURVE('',#31456,#31453,#26346,.T.) ;
#38140=EDGE_CURVE('',#31347,#31454,#26347,.T.) ;
#38141=EDGE_CURVE('',#31467,#31350,#26348,.T.) ;
#38142=EDGE_CURVE('',#31338,#31467,#26349,.T.) ;
#38143=EDGE_CURVE('',#31456,#31447,#26350,.T.) ;
#38144=EDGE_CURVE('',#31348,#31459,#26351,.T.) ;
#38145=EDGE_CURVE('',#31339,#31350,#26352,.T.) ;
#38146=EDGE_CURVE('',#31449,#31342,#26353,.T.) ;
#38147=EDGE_CURVE('',#31457,#31449,#26354,.T.) ;
#38148=EDGE_CURVE('',#31349,#31458,#26355,.T.) ;
#38149=EDGE_CURVE('',#31340,#31349,#26356,.T.) ;
#38150=EDGE_CURVE('',#31457,#31342,#26357,.T.) ;
#38151=EDGE_CURVE('',#31341,#31458,#26358,.T.) ;
#38152=EDGE_CURVE('',#31405,#31386,#26359,.T.) ;
#38153=EDGE_CURVE('',#31394,#31405,#26360,.T.) ;
#38154=EDGE_CURVE('',#31386,#31394,#26361,.T.) ;
#38155=EDGE_CURVE('',#31412,#31560,#222,.T.) ;
#38156=EDGE_CURVE('',#31560,#31391,#4932,.T.) ;
#38157=EDGE_CURVE('',#31393,#31561,#4933,.T.) ;
#38158=EDGE_CURVE('',#31561,#31379,#223,.T.) ;
#38159=EDGE_CURVE('',#31406,#31385,#26362,.T.) ;
#38160=EDGE_CURVE('',#31401,#31562,#4934,.T.) ;
#38161=EDGE_CURVE('',#31562,#31412,#224,.T.) ;
#38162=EDGE_CURVE('',#31411,#31563,#225,.T.) ;
#38163=EDGE_CURVE('',#31563,#31402,#4935,.T.) ;
#38164=EDGE_CURVE('',#31379,#31564,#226,.T.) ;
#38165=EDGE_CURVE('',#31564,#31396,#4936,.T.) ;
#38166=EDGE_CURVE('',#31395,#31565,#4937,.T.) ;
#38167=EDGE_CURVE('',#31565,#31380,#227,.T.) ;
#38168=EDGE_CURVE('',#31406,#31377,#26363,.T.) ;
#38169=EDGE_CURVE('',#31376,#31385,#26364,.T.) ;
#38170=EDGE_CURVE('',#31566,#31377,#9477,.T.) ;
#38171=EDGE_CURVE('',#31407,#31566,#26365,.T.) ;
#38172=EDGE_CURVE('',#31567,#31566,#26366,.T.) ;
#38173=EDGE_CURVE('',#31407,#31567,#26367,.T.) ;
#38174=EDGE_CURVE('',#31390,#31568,#4938,.T.) ;
#38175=EDGE_CURVE('',#31568,#31411,#228,.T.) ;
#38176=EDGE_CURVE('',#31387,#31410,#26368,.T.) ;
#38177=EDGE_CURVE('',#31380,#31569,#229,.T.) ;
#38178=EDGE_CURVE('',#31569,#31388,#4939,.T.) ;
#38179=EDGE_CURVE('',#31381,#31387,#26369,.T.) ;
#38180=EDGE_CURVE('',#31570,#31384,#26370,.T.) ;
#38181=EDGE_CURVE('',#31376,#31570,#9478,.T.) ;
#38182=EDGE_CURVE('',#31365,#31378,#4940,.T.) ;
#38183=EDGE_CURVE('',#31566,#31363,#26371,.T.) ;
#38184=EDGE_CURVE('',#31567,#31364,#26372,.T.) ;
#38185=EDGE_CURVE('',#31571,#31567,#9479,.T.) ;
#38186=EDGE_CURVE('',#31408,#31571,#26373,.T.) ;
#38187=EDGE_CURVE('',#31381,#31410,#26374,.T.) ;
#38188=EDGE_CURVE('',#31570,#31572,#26375,.T.) ;
#38189=EDGE_CURVE('',#31572,#31384,#26376,.T.) ;
#38190=EDGE_CURVE('',#31371,#31570,#26377,.T.) ;
#38191=EDGE_CURVE('',#31571,#31368,#26378,.T.) ;
#38192=EDGE_CURVE('',#31573,#31571,#26379,.T.) ;
#38193=EDGE_CURVE('',#31408,#31573,#26380,.T.) ;
#38194=EDGE_CURVE('',#31382,#31409,#26381,.T.) ;
#38195=EDGE_CURVE('',#31574,#31383,#26382,.T.) ;
#38196=EDGE_CURVE('',#31572,#31574,#9480,.T.) ;
#38197=EDGE_CURVE('',#31372,#31572,#26383,.T.) ;
#38198=EDGE_CURVE('',#31573,#31367,#26384,.T.) ;
#38199=EDGE_CURVE('',#31373,#31573,#9481,.T.) ;
#38200=EDGE_CURVE('',#31409,#31373,#26385,.T.) ;
#38201=EDGE_CURVE('',#31382,#31375,#26386,.T.) ;
#38202=EDGE_CURVE('',#31574,#31575,#26387,.T.) ;
#38203=EDGE_CURVE('',#31575,#31383,#26388,.T.) ;
#38204=EDGE_CURVE('',#31370,#31574,#26389,.T.) ;
#38205=EDGE_CURVE('',#31374,#31366,#4941,.T.) ;
#38206=EDGE_CURVE('',#31575,#31375,#9482,.T.) ;
#38207=EDGE_CURVE('',#31369,#31575,#26390,.T.) ;
#38208=EDGE_CURVE('',#31423,#31427,#26391,.T.) ;
#38209=EDGE_CURVE('',#31423,#31431,#26392,.T.) ;
#38210=EDGE_CURVE('',#31431,#31427,#26393,.T.) ;
#38211=EDGE_CURVE('',#31426,#31343,#26394,.T.) ;
#38212=EDGE_CURVE('',#31432,#31426,#26395,.T.) ;
#38213=EDGE_CURVE('',#31424,#31430,#26396,.T.) ;
#38214=EDGE_CURVE('',#31255,#31421,#26397,.T.) ;
#38215=EDGE_CURVE('',#31226,#31256,#26398,.T.) ;
#38216=EDGE_CURVE('',#31229,#31255,#26399,.T.) ;
#38217=EDGE_CURVE('',#31432,#31344,#26400,.T.) ;
#38218=EDGE_CURVE('',#31424,#31428,#26401,.T.) ;
#38219=EDGE_CURVE('',#31428,#31430,#26402,.T.) ;
#38220=EDGE_CURVE('',#31229,#31422,#26403,.T.) ;
#38221=EDGE_CURVE('',#31433,#31362,#26404,.T.) ;
#38222=EDGE_CURVE('',#31429,#31433,#26405,.T.) ;
#38223=EDGE_CURVE('',#31425,#31224,#26406,.T.) ;
#38224=EDGE_CURVE('',#31223,#31425,#26407,.T.) ;
#38225=EDGE_CURVE('',#31261,#31225,#26408,.T.) ;
#38226=EDGE_CURVE('',#31262,#31232,#26409,.T.) ;
#38227=EDGE_CURVE('',#31444,#31262,#26410,.T.) ;
#38228=EDGE_CURVE('',#31440,#31443,#26411,.T.) ;
#38229=EDGE_CURVE('',#31429,#31361,#26412,.T.) ;
#38230=EDGE_CURVE('',#31445,#31232,#26413,.T.) ;
#38231=EDGE_CURVE('',#31440,#31434,#26414,.T.) ;
#38232=EDGE_CURVE('',#31434,#31443,#26415,.T.) ;
#38233=EDGE_CURVE('',#31222,#31360,#230,.T.) ;
#38234=EDGE_CURVE('',#31446,#31220,#26416,.T.) ;
#38235=EDGE_CURVE('',#31442,#31439,#26417,.T.) ;
#38236=EDGE_CURVE('',#31218,#31446,#26418,.T.) ;
#38237=EDGE_CURVE('',#31435,#31442,#26419,.T.) ;
#38238=EDGE_CURVE('',#31441,#31437,#26420,.T.) ;
#38239=EDGE_CURVE('',#31355,#31441,#26421,.T.) ;
#38240=EDGE_CURVE('',#31230,#31360,#26422,.T.) ;
#38241=EDGE_CURVE('',#31576,#31219,#26423,.T.) ;
#38242=EDGE_CURVE('',#31435,#31439,#26424,.T.) ;
#38243=EDGE_CURVE('',#31356,#31437,#26425,.T.) ;
#38244=EDGE_CURVE('',#31231,#31359,#26426,.T.) ;
#38245=EDGE_CURVE('',#31436,#31438,#26427,.T.) ;
#38246=EDGE_CURVE('',#31357,#31436,#26428,.T.) ;
#38247=EDGE_CURVE('',#31216,#31359,#231,.T.) ;
#38248=EDGE_CURVE('',#31358,#31438,#26429,.T.) ;
#38249=EDGE_CURVE('',#31235,#31516,#232,.T.) ;
#38250=EDGE_CURVE('',#31519,#31515,#26430,.T.) ;
#38251=EDGE_CURVE('',#31514,#31520,#26431,.T.) ;
#38252=EDGE_CURVE('',#31517,#31400,#233,.T.) ;
#38253=EDGE_CURVE('',#31512,#31537,#26432,.T.) ;
#38254=EDGE_CURVE('',#31524,#31551,#26433,.T.) ;
#38255=EDGE_CURVE('',#31525,#31550,#26434,.T.) ;
#38256=EDGE_CURVE('',#31511,#31238,#234,.T.) ;
#38257=EDGE_CURVE('',#31506,#31518,#26435,.T.) ;
#38258=EDGE_CURVE('',#31536,#31513,#26436,.T.) ;
#38259=EDGE_CURVE('',#31525,#31529,#26437,.T.) ;
#38260=EDGE_CURVE('',#31529,#31550,#26438,.T.) ;
#38261=EDGE_CURVE('',#31521,#31507,#26439,.T.) ;
#38262=EDGE_CURVE('',#31552,#31531,#26440,.T.) ;
#38263=EDGE_CURVE('',#31553,#31530,#26441,.T.) ;
#38264=EDGE_CURVE('',#31526,#31553,#26442,.T.) ;
#38265=EDGE_CURVE('',#31522,#31528,#26443,.T.) ;
#38266=EDGE_CURVE('',#31548,#31523,#26444,.T.) ;
#38267=EDGE_CURVE('',#31549,#31522,#26445,.T.) ;
#38268=EDGE_CURVE('',#31526,#31530,#26446,.T.) ;
#38269=EDGE_CURVE('',#31549,#31528,#26447,.T.) ;
#38270=EDGE_CURVE('',#31527,#31533,#26448,.T.) ;
#38271=EDGE_CURVE('',#31546,#31527,#26449,.T.) ;
#38272=EDGE_CURVE('',#31546,#31533,#26450,.T.) ;
#38273=EDGE_CURVE('',#31532,#31547,#26451,.T.) ;
#38274=EDGE_CURVE('',#31508,#31535,#26452,.T.) ;
#38275=EDGE_CURVE('',#31509,#31534,#26453,.T.) ;
#38276=EDGE_CURVE('',#31403,#31510,#235,.T.) ;
#38277=EDGE_CURVE('',#31501,#31502,#26454,.T.) ;
#38278=EDGE_CURVE('',#31505,#31500,#26455,.T.) ;
#38279=EDGE_CURVE('',#31488,#31539,#26456,.T.) ;
#38280=EDGE_CURVE('',#31489,#31538,#26457,.T.) ;
#38281=EDGE_CURVE('',#31540,#31495,#26458,.T.) ;
#38282=EDGE_CURVE('',#31541,#31494,#26459,.T.) ;
#38283=EDGE_CURVE('',#31538,#31493,#26460,.T.) ;
#38284=EDGE_CURVE('',#31490,#31541,#26461,.T.) ;
#38285=EDGE_CURVE('',#31489,#31493,#26462,.T.) ;
#38286=EDGE_CURVE('',#31503,#31498,#26463,.T.) ;
#38287=EDGE_CURVE('',#31499,#31504,#26464,.T.) ;
#38288=EDGE_CURVE('',#31490,#31494,#26465,.T.) ;
#38289=EDGE_CURVE('',#31486,#31492,#26466,.T.) ;
#38290=EDGE_CURVE('',#31544,#31487,#26467,.T.) ;
#38291=EDGE_CURVE('',#31545,#31486,#26468,.T.) ;
#38292=EDGE_CURVE('',#31496,#31543,#26469,.T.) ;
#38293=EDGE_CURVE('',#31497,#31542,#26470,.T.) ;
#38294=EDGE_CURVE('',#31491,#31497,#26471,.T.) ;
#38295=EDGE_CURVE('',#31545,#31492,#26472,.T.) ;
#38296=EDGE_CURVE('',#31491,#31542,#26473,.T.) ;
#38297=EDGE_CURVE('',#31249,#31248,#26474,.T.) ;
#38298=EDGE_CURVE('',#31475,#31250,#236,.T.) ;
#38299=EDGE_CURVE('',#31476,#31249,#26475,.T.) ;
#38300=EDGE_CURVE('',#31476,#31248,#26476,.T.) ;
#38301=EDGE_CURVE('',#31247,#31244,#26477,.T.) ;
#38302=EDGE_CURVE('',#31473,#31247,#26478,.T.) ;
#38303=EDGE_CURVE('',#31473,#31244,#26479,.T.) ;
#38304=EDGE_CURVE('',#31243,#31474,#237,.T.) ;
#38305=EDGE_CURVE('',#31205,#31484,#4942,.T.) ;
#38306=EDGE_CURVE('',#31332,#31483,#26480,.T.) ;
#38307=EDGE_CURVE('',#31329,#31332,#26481,.T.) ;
#38308=EDGE_CURVE('',#31329,#31483,#26482,.T.) ;
#38309=EDGE_CURVE('',#31330,#31485,#26483,.T.) ;
#38310=EDGE_CURVE('',#31328,#31330,#26484,.T.) ;
#38311=EDGE_CURVE('',#31328,#31485,#26485,.T.) ;
#38312=EDGE_CURVE('',#31209,#31325,#4943,.T.) ;
#38313=EDGE_CURVE('',#31397,#31234,#26486,.T.) ;
#38314=EDGE_CURVE('',#31233,#31398,#26487,.T.) ;
#38315=EDGE_CURVE('',#31559,#31267,#26488,.T.) ;
#38316=EDGE_CURVE('',#31556,#31268,#26489,.T.) ;
#38317=EDGE_CURVE('',#31267,#31557,#26490,.T.) ;
#38318=EDGE_CURVE('',#31268,#31554,#26491,.T.) ;
#38319=EDGE_CURVE('',#31391,#31401,#26492,.T.) ;
#38320=EDGE_CURVE('',#31392,#31234,#26493,.T.) ;
#38321=EDGE_CURVE('',#31392,#31397,#26494,.T.) ;
#38322=EDGE_CURVE('',#31393,#31396,#26495,.T.) ;
#38323=EDGE_CURVE('',#31388,#31395,#26496,.T.) ;
#38324=EDGE_CURVE('',#31389,#31398,#26497,.T.) ;
#38325=EDGE_CURVE('',#31389,#31233,#26498,.T.) ;
#38326=EDGE_CURVE('',#31390,#31402,#26499,.T.) ;
#38327=EDGE_CURVE('',#31242,#31478,#238,.T.) ;
#38328=EDGE_CURVE('',#31474,#31477,#26500,.T.) ;
#38329=EDGE_CURVE('',#31475,#31482,#26501,.T.) ;
#38330=EDGE_CURVE('',#31577,#31481,#239,.T.) ;
#38331=EDGE_CURVE('',#31578,#31577,#240,.T.) ;
#38332=EDGE_CURVE('',#31579,#31578,#241,.T.) ;
#38333=EDGE_CURVE('',#31251,#31579,#242,.T.) ;
#38334=EDGE_CURVE('',#31333,#31252,#4944,.T.) ;
#38335=EDGE_CURVE('',#31334,#31481,#26502,.T.) ;
#38336=EDGE_CURVE('',#31208,#31326,#243,.T.) ;
#38337=EDGE_CURVE('',#31335,#31480,#26503,.T.) ;
#38338=EDGE_CURVE('',#31331,#31336,#4945,.T.) ;
#38339=EDGE_CURVE('',#31479,#31484,#26504,.T.) ;
#38340=EDGE_CURVE('',#31580,#31480,#244,.T.) ;
#38341=EDGE_CURVE('',#31581,#31580,#245,.T.) ;
#38342=EDGE_CURVE('',#31204,#31581,#246,.T.) ;
#38343=EDGE_CURVE('',#31261,#31555,#26505,.T.) ;
#38344=EDGE_CURVE('',#31227,#31555,#26506,.T.) ;
#38345=EDGE_CURVE('',#31556,#31554,#26507,.T.) ;
#38346=EDGE_CURVE('',#31524,#31520,#26508,.T.) ;
#38347=EDGE_CURVE('',#31551,#31514,#26509,.T.) ;
#38348=EDGE_CURVE('',#31521,#31523,#26510,.T.) ;
#38349=EDGE_CURVE('',#31552,#31513,#26511,.T.) ;
#38350=EDGE_CURVE('',#31507,#31548,#26512,.T.) ;
#38351=EDGE_CURVE('',#31531,#31536,#26513,.T.) ;
#38352=EDGE_CURVE('',#31508,#31547,#26514,.T.) ;
#38353=EDGE_CURVE('',#31532,#31535,#26515,.T.) ;
#38354=EDGE_CURVE('',#31488,#31502,#26516,.T.) ;
#38355=EDGE_CURVE('',#31539,#31501,#26517,.T.) ;
#38356=EDGE_CURVE('',#31503,#31487,#26518,.T.) ;
#38357=EDGE_CURVE('',#31540,#31500,#26519,.T.) ;
#38358=EDGE_CURVE('',#31498,#31544,#26520,.T.) ;
#38359=EDGE_CURVE('',#31495,#31505,#26521,.T.) ;
#38360=EDGE_CURVE('',#31499,#31543,#26522,.T.) ;
#38361=EDGE_CURVE('',#31496,#31504,#26523,.T.) ;
#38362=EDGE_CURVE('',#31558,#31256,#26524,.T.) ;
#38363=EDGE_CURVE('',#31558,#31228,#26525,.T.) ;
#38364=EDGE_CURVE('',#31559,#31557,#26526,.T.) ;
#38365=EDGE_CURVE('',#31323,#31327,#4946,.T.) ;
#38366=EDGE_CURVE('',#31324,#31207,#26527,.T.) ;
#38367=EDGE_CURVE('',#31321,#31478,#26528,.T.) ;
#38368=EDGE_CURVE('',#31322,#31241,#4947,.T.) ;
#38369=EDGE_CURVE('',#31582,#31583,#247,.T.) ;
#38370=EDGE_CURVE('',#31583,#31584,#4948,.T.) ;
#38371=EDGE_CURVE('',#31584,#31585,#26529,.T.) ;
#38372=EDGE_CURVE('',#31586,#31585,#4949,.T.) ;
#38373=EDGE_CURVE('',#31582,#31586,#248,.T.) ;
#38374=EDGE_CURVE('',#31587,#31588,#249,.T.) ;
#38375=EDGE_CURVE('',#31588,#31589,#26530,.T.) ;
#38376=EDGE_CURVE('',#31590,#31589,#4950,.T.) ;
#38377=EDGE_CURVE('',#31591,#31590,#26531,.T.) ;
#38378=EDGE_CURVE('',#31587,#31591,#4951,.T.) ;
#38379=EDGE_CURVE('',#31592,#31592,#26532,.T.) ;
#38380=EDGE_CURVE('',#31592,#31593,#26533,.T.) ;
#38381=EDGE_CURVE('',#31593,#31593,#26534,.T.) ;
#38382=EDGE_CURVE('',#31594,#31594,#26535,.T.) ;
#38383=EDGE_CURVE('',#31594,#31595,#26536,.T.) ;
#38384=EDGE_CURVE('',#31595,#31595,#26537,.T.) ;
#38385=EDGE_CURVE('',#31596,#31597,#26538,.T.) ;
#38386=EDGE_CURVE('',#31598,#31596,#9483,.T.) ;
#38387=EDGE_CURVE('',#31598,#31599,#26539,.T.) ;
#38388=EDGE_CURVE('',#31599,#31600,#26540,.T.) ;
#38389=EDGE_CURVE('',#31597,#31600,#9484,.T.) ;
#38390=EDGE_CURVE('',#31601,#31602,#26541,.T.) ;
#38391=EDGE_CURVE('',#31603,#31601,#9485,.T.) ;
#38392=EDGE_CURVE('',#31603,#31604,#26542,.T.) ;
#38393=EDGE_CURVE('',#31602,#31604,#9486,.T.) ;
#38394=EDGE_CURVE('',#31605,#31606,#26543,.T.) ;
#38395=EDGE_CURVE('',#31605,#31607,#26544,.T.) ;
#38396=EDGE_CURVE('',#31608,#31607,#26545,.T.) ;
#38397=EDGE_CURVE('',#31608,#31606,#26546,.T.) ;
#38398=EDGE_CURVE('',#31593,#31594,#9487,.T.) ;
#38399=EDGE_CURVE('',#31606,#31609,#9488,.T.) ;
#38400=EDGE_CURVE('',#31609,#31603,#26547,.T.) ;
#38401=EDGE_CURVE('',#31610,#31601,#250,.T.) ;
#38402=EDGE_CURVE('',#31610,#31611,#26548,.T.) ;
#38403=EDGE_CURVE('',#31597,#31611,#251,.T.) ;
#38404=EDGE_CURVE('',#31600,#31612,#26549,.T.) ;
#38405=EDGE_CURVE('',#31612,#31605,#9489,.T.) ;
#38406=EDGE_CURVE('',#31613,#31614,#9490,.T.) ;
#38407=EDGE_CURVE('',#31614,#31615,#9491,.T.) ;
#38408=EDGE_CURVE('',#31615,#31616,#252,.T.) ;
#38409=EDGE_CURVE('',#31616,#31617,#9492,.T.) ;
#38410=EDGE_CURVE('',#31617,#31618,#4952,.T.) ;
#38411=EDGE_CURVE('',#31618,#31613,#9493,.T.) ;
#38412=EDGE_CURVE('',#31619,#31620,#9494,.T.) ;
#38413=EDGE_CURVE('',#31620,#31621,#9495,.T.) ;
#38414=EDGE_CURVE('',#31621,#31622,#253,.T.) ;
#38415=EDGE_CURVE('',#31622,#31623,#254,.T.) ;
#38416=EDGE_CURVE('',#31623,#31624,#9496,.T.) ;
#38417=EDGE_CURVE('',#31624,#31619,#9497,.T.) ;
#38418=EDGE_CURVE('',#31625,#31626,#9498,.T.) ;
#38419=EDGE_CURVE('',#31626,#31627,#9499,.T.) ;
#38420=EDGE_CURVE('',#31627,#31628,#9500,.T.) ;
#38421=EDGE_CURVE('',#31628,#31625,#9501,.T.) ;
#38422=EDGE_CURVE('',#31629,#31630,#9502,.T.) ;
#38423=EDGE_CURVE('',#31630,#31631,#255,.T.) ;
#38424=EDGE_CURVE('',#31631,#31632,#256,.T.) ;
#38425=EDGE_CURVE('',#31632,#31633,#9503,.T.) ;
#38426=EDGE_CURVE('',#31633,#31634,#9504,.T.) ;
#38427=EDGE_CURVE('',#31634,#31629,#9505,.T.) ;
#38428=EDGE_CURVE('',#31635,#31636,#9506,.T.) ;
#38429=EDGE_CURVE('',#31636,#31637,#9507,.T.) ;
#38430=EDGE_CURVE('',#31637,#31638,#9508,.T.) ;
#38431=EDGE_CURVE('',#31638,#31635,#9509,.T.) ;
#38432=EDGE_CURVE('',#31639,#31640,#9510,.T.) ;
#38433=EDGE_CURVE('',#31639,#31641,#9511,.T.) ;
#38434=EDGE_CURVE('',#31641,#31642,#9512,.T.) ;
#38435=EDGE_CURVE('',#31642,#31640,#9513,.T.) ;
#38436=EDGE_CURVE('',#31643,#31644,#9514,.T.) ;
#38437=EDGE_CURVE('',#31643,#31645,#9515,.T.) ;
#38438=EDGE_CURVE('',#31645,#31646,#9516,.T.) ;
#38439=EDGE_CURVE('',#31646,#31647,#9517,.T.) ;
#38440=EDGE_CURVE('',#31647,#31648,#26550,.T.) ;
#38441=EDGE_CURVE('',#31648,#31644,#9518,.T.) ;
#38442=EDGE_CURVE('',#31649,#31650,#9519,.T.) ;
#38443=EDGE_CURVE('',#31649,#31620,#26551,.T.) ;
#38444=EDGE_CURVE('',#31619,#31626,#26552,.T.) ;
#38445=EDGE_CURVE('',#31625,#31634,#26553,.T.) ;
#38446=EDGE_CURVE('',#31633,#31651,#26554,.T.) ;
#38447=EDGE_CURVE('',#31652,#31651,#9520,.T.) ;
#38448=EDGE_CURVE('',#31652,#31653,#26555,.T.) ;
#38449=EDGE_CURVE('',#31654,#31653,#9521,.T.) ;
#38450=EDGE_CURVE('',#31654,#31655,#26556,.T.) ;
#38451=EDGE_CURVE('',#31655,#31656,#9522,.T.) ;
#38452=EDGE_CURVE('',#31656,#31657,#26557,.T.) ;
#38453=EDGE_CURVE('',#31658,#31657,#9523,.T.) ;
#38454=EDGE_CURVE('',#31658,#31659,#26558,.T.) ;
#38455=EDGE_CURVE('',#31659,#31660,#9524,.T.) ;
#38456=EDGE_CURVE('',#31660,#31661,#26559,.T.) ;
#38457=EDGE_CURVE('',#31662,#31661,#9525,.T.) ;
#38458=EDGE_CURVE('',#31662,#31638,#26560,.T.) ;
#38459=EDGE_CURVE('',#31637,#31663,#26561,.T.) ;
#38460=EDGE_CURVE('',#31663,#31664,#9526,.T.) ;
#38461=EDGE_CURVE('',#31664,#31646,#26562,.T.) ;
#38462=EDGE_CURVE('',#31645,#31665,#26563,.T.) ;
#38463=EDGE_CURVE('',#31666,#31665,#9527,.T.) ;
#38464=EDGE_CURVE('',#31667,#31666,#9528,.T.) ;
#38465=EDGE_CURVE('',#31667,#31668,#26564,.T.) ;
#38466=EDGE_CURVE('',#31669,#31668,#9529,.T.) ;
#38467=EDGE_CURVE('',#31669,#31670,#26565,.T.) ;
#38468=EDGE_CURVE('',#31671,#31670,#9530,.T.) ;
#38469=EDGE_CURVE('',#31671,#31650,#26566,.T.) ;
#38470=EDGE_CURVE('',#31672,#31673,#9531,.T.) ;
#38471=EDGE_CURVE('',#31673,#31674,#26567,.T.) ;
#38472=EDGE_CURVE('',#31674,#31675,#9532,.T.) ;
#38473=EDGE_CURVE('',#31675,#31676,#26568,.T.) ;
#38474=EDGE_CURVE('',#31676,#31677,#9533,.T.) ;
#38475=EDGE_CURVE('',#31677,#31678,#26569,.T.) ;
#38476=EDGE_CURVE('',#31678,#31679,#9534,.T.) ;
#38477=EDGE_CURVE('',#31679,#31680,#26570,.T.) ;
#38478=EDGE_CURVE('',#31680,#31681,#9535,.T.) ;
#38479=EDGE_CURVE('',#31681,#31682,#9536,.T.) ;
#38480=EDGE_CURVE('',#31682,#31643,#26571,.T.) ;
#38481=EDGE_CURVE('',#31644,#31683,#26572,.T.) ;
#38482=EDGE_CURVE('',#31683,#31684,#9537,.T.) ;
#38483=EDGE_CURVE('',#31684,#31639,#26573,.T.) ;
#38484=EDGE_CURVE('',#31640,#31685,#26574,.T.) ;
#38485=EDGE_CURVE('',#31686,#31685,#9538,.T.) ;
#38486=EDGE_CURVE('',#31686,#31687,#26575,.T.) ;
#38487=EDGE_CURVE('',#31688,#31687,#9539,.T.) ;
#38488=EDGE_CURVE('',#31688,#31689,#26576,.T.) ;
#38489=EDGE_CURVE('',#31689,#31690,#9540,.T.) ;
#38490=EDGE_CURVE('',#31690,#31691,#26577,.T.) ;
#38491=EDGE_CURVE('',#31692,#31691,#9541,.T.) ;
#38492=EDGE_CURVE('',#31692,#31693,#26578,.T.) ;
#38493=EDGE_CURVE('',#31694,#31693,#9542,.T.) ;
#38494=EDGE_CURVE('',#31694,#31695,#26579,.T.) ;
#38495=EDGE_CURVE('',#31695,#31696,#9543,.T.) ;
#38496=EDGE_CURVE('',#31696,#31697,#26580,.T.) ;
#38497=EDGE_CURVE('',#31697,#31698,#9544,.T.) ;
#38498=EDGE_CURVE('',#31698,#31699,#26581,.T.) ;
#38499=EDGE_CURVE('',#31699,#31700,#9545,.T.) ;
#38500=EDGE_CURVE('',#31700,#31672,#26582,.T.) ;
#38501=EDGE_CURVE('',#31668,#31679,#9546,.T.) ;
#38502=EDGE_CURVE('',#31678,#31669,#9547,.T.) ;
#38503=EDGE_CURVE('',#31670,#31677,#9548,.T.) ;
#38504=EDGE_CURVE('',#31676,#31671,#9549,.T.) ;
#38505=EDGE_CURVE('',#31701,#31702,#257,.T.) ;
#38506=EDGE_CURVE('',#31702,#31649,#9550,.T.) ;
#38507=EDGE_CURVE('',#31650,#31675,#9551,.T.) ;
#38508=EDGE_CURVE('',#31674,#31703,#9552,.T.) ;
#38509=EDGE_CURVE('',#31703,#31704,#258,.T.) ;
#38510=EDGE_CURVE('',#31704,#31701,#9553,.T.) ;
#38511=EDGE_CURVE('',#31705,#31706,#259,.T.) ;
#38512=EDGE_CURVE('',#31706,#31707,#4953,.T.) ;
#38513=EDGE_CURVE('',#31707,#31673,#9554,.T.) ;
#38514=EDGE_CURVE('',#31672,#31708,#9555,.T.) ;
#38515=EDGE_CURVE('',#31708,#31705,#9556,.T.) ;
#38516=EDGE_CURVE('',#31709,#31710,#9557,.T.) ;
#38517=EDGE_CURVE('',#31710,#31700,#9558,.T.) ;
#38518=EDGE_CURVE('',#31699,#31709,#9559,.T.) ;
#38519=EDGE_CURVE('',#31711,#31582,#260,.T.) ;
#38520=EDGE_CURVE('',#31586,#31712,#9560,.T.) ;
#38521=EDGE_CURVE('',#31712,#31698,#9561,.T.) ;
#38522=EDGE_CURVE('',#31697,#31711,#9562,.T.) ;
#38523=EDGE_CURVE('',#31651,#31713,#9563,.T.) ;
#38524=EDGE_CURVE('',#31713,#31714,#261,.T.) ;
#38525=EDGE_CURVE('',#31714,#31715,#9564,.T.) ;
#38526=EDGE_CURVE('',#31715,#31716,#262,.T.) ;
#38527=EDGE_CURVE('',#31716,#31696,#9565,.T.) ;
#38528=EDGE_CURVE('',#31695,#31717,#9566,.T.) ;
#38529=EDGE_CURVE('',#31717,#31718,#9567,.T.) ;
#38530=EDGE_CURVE('',#31719,#31718,#26583,.T.) ;
#38531=EDGE_CURVE('',#31719,#31720,#9568,.T.) ;
#38532=EDGE_CURVE('',#31721,#31720,#26584,.T.) ;
#38533=EDGE_CURVE('',#31721,#31722,#9569,.T.) ;
#38534=EDGE_CURVE('',#31722,#31652,#9570,.T.) ;
#38535=EDGE_CURVE('',#31723,#31724,#26585,.T.) ;
#38536=EDGE_CURVE('',#31723,#31658,#9571,.T.) ;
#38537=EDGE_CURVE('',#31657,#31725,#9572,.T.) ;
#38538=EDGE_CURVE('',#31726,#31725,#26586,.T.) ;
#38539=EDGE_CURVE('',#31726,#31727,#26587,.T.) ;
#38540=EDGE_CURVE('',#31728,#31727,#26588,.T.) ;
#38541=EDGE_CURVE('',#31728,#31729,#9573,.T.) ;
#38542=EDGE_CURVE('',#31729,#31730,#9574,.T.) ;
#38543=EDGE_CURVE('',#31730,#31731,#9575,.T.) ;
#38544=EDGE_CURVE('',#31732,#31731,#26589,.T.) ;
#38545=EDGE_CURVE('',#31732,#31733,#26590,.T.) ;
#38546=EDGE_CURVE('',#31734,#31733,#26591,.T.) ;
#38547=EDGE_CURVE('',#31734,#31690,#9576,.T.) ;
#38548=EDGE_CURVE('',#31689,#31735,#9577,.T.) ;
#38549=EDGE_CURVE('',#31736,#31735,#26592,.T.) ;
#38550=EDGE_CURVE('',#31736,#31737,#26593,.T.) ;
#38551=EDGE_CURVE('',#31738,#31737,#26594,.T.) ;
#38552=EDGE_CURVE('',#31738,#31739,#9578,.T.) ;
#38553=EDGE_CURVE('',#31739,#31740,#26595,.T.) ;
#38554=EDGE_CURVE('',#31740,#31741,#9579,.T.) ;
#38555=EDGE_CURVE('',#31742,#31741,#26596,.T.) ;
#38556=EDGE_CURVE('',#31742,#31724,#26597,.T.) ;
#38557=EDGE_CURVE('',#31743,#31744,#26598,.T.) ;
#38558=EDGE_CURVE('',#31743,#31745,#9580,.T.) ;
#38559=EDGE_CURVE('',#31666,#31745,#9581,.T.) ;
#38560=EDGE_CURVE('',#31665,#31682,#9582,.T.) ;
#38561=EDGE_CURVE('',#31746,#31681,#9583,.T.) ;
#38562=EDGE_CURVE('',#31746,#31747,#9584,.T.) ;
#38563=EDGE_CURVE('',#31748,#31747,#26599,.T.) ;
#38564=EDGE_CURVE('',#31748,#31744,#9585,.T.) ;
#38565=EDGE_CURVE('',#31749,#31750,#26600,.T.) ;
#38566=EDGE_CURVE('',#31749,#31746,#9586,.T.) ;
#38567=EDGE_CURVE('',#31680,#31667,#9587,.T.) ;
#38568=EDGE_CURVE('',#31745,#31751,#9588,.T.) ;
#38569=EDGE_CURVE('',#31752,#31751,#26601,.T.) ;
#38570=EDGE_CURVE('',#31752,#31750,#9589,.T.) ;
#38571=EDGE_CURVE('',#31753,#31754,#9590,.T.) ;
#38572=EDGE_CURVE('',#31754,#31755,#9591,.T.) ;
#38573=EDGE_CURVE('',#31753,#31755,#26602,.T.) ;
#38574=EDGE_CURVE('',#31756,#31757,#26603,.T.) ;
#38575=EDGE_CURVE('',#31756,#31758,#9592,.T.) ;
#38576=EDGE_CURVE('',#31758,#31757,#9593,.T.) ;
#38577=EDGE_CURVE('',#31759,#31760,#9594,.T.) ;
#38578=EDGE_CURVE('',#31760,#31761,#9595,.T.) ;
#38579=EDGE_CURVE('',#31761,#31762,#9596,.T.) ;
#38580=EDGE_CURVE('',#31762,#31763,#9597,.T.) ;
#38581=EDGE_CURVE('',#31763,#31764,#9598,.T.) ;
#38582=EDGE_CURVE('',#31764,#31765,#9599,.T.) ;
#38583=EDGE_CURVE('',#31765,#31766,#9600,.T.) ;
#38584=EDGE_CURVE('',#31766,#31759,#9601,.T.) ;
#38585=EDGE_CURVE('',#31767,#31768,#9602,.T.) ;
#38586=EDGE_CURVE('',#31768,#31769,#9603,.T.) ;
#38587=EDGE_CURVE('',#31769,#31770,#9604,.T.) ;
#38588=EDGE_CURVE('',#31770,#31767,#9605,.T.) ;
#38589=EDGE_CURVE('',#31771,#31772,#9606,.T.) ;
#38590=EDGE_CURVE('',#31772,#31773,#9607,.T.) ;
#38591=EDGE_CURVE('',#31773,#31774,#9608,.T.) ;
#38592=EDGE_CURVE('',#31774,#31771,#9609,.T.) ;
#38593=EDGE_CURVE('',#31775,#31776,#9610,.T.) ;
#38594=EDGE_CURVE('',#31776,#31777,#9611,.T.) ;
#38595=EDGE_CURVE('',#31777,#31778,#9612,.T.) ;
#38596=EDGE_CURVE('',#31778,#31775,#9613,.T.) ;
#38597=EDGE_CURVE('',#31779,#31780,#263,.T.) ;
#38598=EDGE_CURVE('',#31780,#31781,#9614,.T.) ;
#38599=EDGE_CURVE('',#31781,#31782,#9615,.T.) ;
#38600=EDGE_CURVE('',#31782,#31783,#9616,.T.) ;
#38601=EDGE_CURVE('',#31783,#31784,#264,.T.) ;
#38602=EDGE_CURVE('',#31784,#31779,#9617,.T.) ;
#38603=EDGE_CURVE('',#31785,#31786,#9618,.T.) ;
#38604=EDGE_CURVE('',#31786,#31787,#9619,.T.) ;
#38605=EDGE_CURVE('',#31787,#31788,#9620,.T.) ;
#38606=EDGE_CURVE('',#31788,#31789,#9621,.T.) ;
#38607=EDGE_CURVE('',#31789,#31790,#9622,.T.) ;
#38608=EDGE_CURVE('',#31790,#31791,#9623,.T.) ;
#38609=EDGE_CURVE('',#31791,#31792,#9624,.T.) ;
#38610=EDGE_CURVE('',#31792,#31785,#9625,.T.) ;
#38611=EDGE_CURVE('',#31793,#31794,#9626,.T.) ;
#38612=EDGE_CURVE('',#31793,#31795,#26604,.T.) ;
#38613=EDGE_CURVE('',#31795,#31796,#9627,.T.) ;
#38614=EDGE_CURVE('',#31796,#31797,#26605,.T.) ;
#38615=EDGE_CURVE('',#31797,#31798,#9628,.T.) ;
#38616=EDGE_CURVE('',#31798,#31799,#26606,.T.) ;
#38617=EDGE_CURVE('',#31799,#31800,#9629,.T.) ;
#38618=EDGE_CURVE('',#31800,#31794,#26607,.T.) ;
#38619=EDGE_CURVE('',#31801,#31802,#26608,.T.) ;
#38620=EDGE_CURVE('',#31801,#31662,#9630,.T.) ;
#38621=EDGE_CURVE('',#31661,#31803,#9631,.T.) ;
#38622=EDGE_CURVE('',#31803,#31804,#26609,.T.) ;
#38623=EDGE_CURVE('',#31804,#31805,#9632,.T.) ;
#38624=EDGE_CURVE('',#31805,#31802,#26610,.T.) ;
#38625=EDGE_CURVE('',#31659,#31806,#9633,.T.) ;
#38626=EDGE_CURVE('',#31806,#31807,#9634,.T.) ;
#38627=EDGE_CURVE('',#31807,#31660,#9635,.T.) ;
#38628=EDGE_CURVE('',#31808,#31809,#9636,.T.) ;
#38629=EDGE_CURVE('',#31809,#31602,#9637,.T.) ;
#38630=EDGE_CURVE('',#31604,#31808,#9638,.T.) ;
#38631=EDGE_CURVE('',#31810,#31811,#26611,.T.) ;
#38632=EDGE_CURVE('',#31811,#31812,#9639,.T.) ;
#38633=EDGE_CURVE('',#31812,#31813,#26612,.T.) ;
#38634=EDGE_CURVE('',#31813,#31810,#9640,.T.) ;
#38635=EDGE_CURVE('',#31814,#31815,#26613,.T.) ;
#38636=EDGE_CURVE('',#31815,#31816,#9641,.T.) ;
#38637=EDGE_CURVE('',#31816,#31817,#26614,.T.) ;
#38638=EDGE_CURVE('',#31817,#31814,#9642,.T.) ;
#38639=EDGE_CURVE('',#31596,#31818,#9643,.T.) ;
#38640=EDGE_CURVE('',#31818,#31819,#9644,.T.) ;
#38641=EDGE_CURVE('',#31819,#31598,#9645,.T.) ;
#38642=EDGE_CURVE('',#31820,#31821,#9646,.T.) ;
#38643=EDGE_CURVE('',#31821,#31688,#9647,.T.) ;
#38644=EDGE_CURVE('',#31687,#31820,#9648,.T.) ;
#38645=EDGE_CURVE('',#31822,#31823,#26615,.T.) ;
#38646=EDGE_CURVE('',#31823,#31686,#9649,.T.) ;
#38647=EDGE_CURVE('',#31685,#31824,#9650,.T.) ;
#38648=EDGE_CURVE('',#31825,#31824,#26616,.T.) ;
#38649=EDGE_CURVE('',#31825,#31826,#26617,.T.) ;
#38650=EDGE_CURVE('',#31826,#31822,#9651,.T.) ;
#38651=EDGE_CURVE('',#31827,#31828,#26618,.T.) ;
#38652=EDGE_CURVE('',#31828,#31654,#9652,.T.) ;
#38653=EDGE_CURVE('',#31653,#31829,#9653,.T.) ;
#38654=EDGE_CURVE('',#31829,#31827,#9654,.T.) ;
#38655=EDGE_CURVE('',#31830,#31831,#9655,.T.) ;
#38656=EDGE_CURVE('',#31831,#31656,#9656,.T.) ;
#38657=EDGE_CURVE('',#31655,#31830,#9657,.T.) ;
#38658=EDGE_CURVE('',#31832,#31833,#26619,.T.) ;
#38659=EDGE_CURVE('',#31833,#31834,#9658,.T.) ;
#38660=EDGE_CURVE('',#31834,#31835,#26620,.T.) ;
#38661=EDGE_CURVE('',#31835,#31832,#9659,.T.) ;
#38662=EDGE_CURVE('',#31836,#31837,#9660,.T.) ;
#38663=EDGE_CURVE('',#31837,#31838,#9661,.T.) ;
#38664=EDGE_CURVE('',#31838,#31839,#9662,.T.) ;
#38665=EDGE_CURVE('',#31839,#31836,#9663,.T.) ;
#38666=EDGE_CURVE('',#31840,#31841,#26621,.T.) ;
#38667=EDGE_CURVE('',#31841,#31842,#9664,.T.) ;
#38668=EDGE_CURVE('',#31842,#31843,#26622,.T.) ;
#38669=EDGE_CURVE('',#31843,#31840,#9665,.T.) ;
#38670=EDGE_CURVE('',#31691,#31844,#9666,.T.) ;
#38671=EDGE_CURVE('',#31844,#31845,#9667,.T.) ;
#38672=EDGE_CURVE('',#31845,#31692,#9668,.T.) ;
#38673=EDGE_CURVE('',#31846,#31847,#9669,.T.) ;
#38674=EDGE_CURVE('',#31847,#31848,#9670,.T.) ;
#38675=EDGE_CURVE('',#31848,#31849,#9671,.T.) ;
#38676=EDGE_CURVE('',#31849,#31846,#9672,.T.) ;
#38677=EDGE_CURVE('',#31850,#31851,#9673,.T.) ;
#38678=EDGE_CURVE('',#31851,#31694,#9674,.T.) ;
#38679=EDGE_CURVE('',#31693,#31852,#9675,.T.) ;
#38680=EDGE_CURVE('',#31852,#31850,#26623,.T.) ;
#38681=EDGE_CURVE('',#31853,#31854,#9676,.T.) ;
#38682=EDGE_CURVE('',#31854,#31855,#9677,.T.) ;
#38683=EDGE_CURVE('',#31855,#31856,#9678,.T.) ;
#38684=EDGE_CURVE('',#31856,#31853,#9679,.T.) ;
#38685=EDGE_CURVE('',#31857,#31858,#4954,.T.) ;
#38686=EDGE_CURVE('',#31858,#31587,#9680,.T.) ;
#38687=EDGE_CURVE('',#31591,#31859,#9681,.T.) ;
#38688=EDGE_CURVE('',#31859,#31860,#4955,.T.) ;
#38689=EDGE_CURVE('',#31860,#31861,#9682,.T.) ;
#38690=EDGE_CURVE('',#31861,#31862,#4956,.T.) ;
#38691=EDGE_CURVE('',#31862,#31857,#9683,.T.) ;
#38692=EDGE_CURVE('',#31863,#31864,#9684,.T.) ;
#38693=EDGE_CURVE('',#31864,#31590,#9685,.T.) ;
#38694=EDGE_CURVE('',#31590,#31865,#9686,.T.) ;
#38695=EDGE_CURVE('',#31865,#31863,#9687,.T.) ;
#38696=EDGE_CURVE('',#31866,#31867,#9688,.T.) ;
#38697=EDGE_CURVE('',#31867,#31868,#9689,.T.) ;
#38698=EDGE_CURVE('',#31868,#31869,#9690,.T.) ;
#38699=EDGE_CURVE('',#31869,#31866,#9691,.T.) ;
#38700=EDGE_CURVE('',#31870,#31871,#9692,.T.) ;
#38701=EDGE_CURVE('',#31871,#31872,#9693,.T.) ;
#38702=EDGE_CURVE('',#31872,#31873,#9694,.T.) ;
#38703=EDGE_CURVE('',#31873,#31870,#9695,.T.) ;
#38704=EDGE_CURVE('',#31874,#31875,#9696,.T.) ;
#38705=EDGE_CURVE('',#31875,#31876,#9697,.T.) ;
#38706=EDGE_CURVE('',#31876,#31877,#9698,.T.) ;
#38707=EDGE_CURVE('',#31877,#31874,#9699,.T.) ;
#38708=EDGE_CURVE('',#31794,#31878,#9700,.T.) ;
#38709=EDGE_CURVE('',#31878,#31879,#9701,.T.) ;
#38710=EDGE_CURVE('',#31879,#31793,#9702,.T.) ;
#38711=EDGE_CURVE('',#31797,#31880,#9703,.T.) ;
#38712=EDGE_CURVE('',#31880,#31881,#9704,.T.) ;
#38713=EDGE_CURVE('',#31881,#31798,#9705,.T.) ;
#38714=EDGE_CURVE('',#31799,#31882,#9706,.T.) ;
#38715=EDGE_CURVE('',#31882,#31883,#9707,.T.) ;
#38716=EDGE_CURVE('',#31883,#31800,#9708,.T.) ;
#38717=EDGE_CURVE('',#31795,#31884,#9709,.T.) ;
#38718=EDGE_CURVE('',#31884,#31885,#9710,.T.) ;
#38719=EDGE_CURVE('',#31885,#31796,#9711,.T.) ;
#38720=EDGE_CURVE('',#31886,#31887,#9712,.T.) ;
#38721=EDGE_CURVE('',#31887,#31888,#9713,.T.) ;
#38722=EDGE_CURVE('',#31888,#31889,#9714,.T.) ;
#38723=EDGE_CURVE('',#31889,#31890,#26624,.T.) ;
#38724=EDGE_CURVE('',#31890,#31891,#9715,.T.) ;
#38725=EDGE_CURVE('',#31891,#31886,#26625,.T.) ;
#38726=EDGE_CURVE('',#31892,#31893,#9716,.T.) ;
#38727=EDGE_CURVE('',#31893,#31894,#9717,.T.) ;
#38728=EDGE_CURVE('',#31894,#31895,#9718,.T.) ;
#38729=EDGE_CURVE('',#31895,#31896,#26626,.T.) ;
#38730=EDGE_CURVE('',#31896,#31897,#9719,.T.) ;
#38731=EDGE_CURVE('',#31897,#31892,#26627,.T.) ;
#38732=EDGE_CURVE('',#31898,#31899,#9720,.T.) ;
#38733=EDGE_CURVE('',#31898,#31617,#26628,.T.) ;
#38734=EDGE_CURVE('',#31616,#31899,#26629,.T.) ;
#38735=EDGE_CURVE('',#31899,#31900,#9721,.T.) ;
#38736=EDGE_CURVE('',#31900,#31901,#9722,.T.) ;
#38737=EDGE_CURVE('',#31901,#31898,#9723,.T.) ;
#38738=EDGE_CURVE('',#31902,#31903,#9724,.T.) ;
#38739=EDGE_CURVE('',#31903,#31904,#9725,.T.) ;
#38740=EDGE_CURVE('',#31904,#31905,#9726,.T.) ;
#38741=EDGE_CURVE('',#31905,#31902,#9727,.T.) ;
#38742=EDGE_CURVE('',#31906,#31907,#9728,.T.) ;
#38743=EDGE_CURVE('',#31907,#31908,#9729,.T.) ;
#38744=EDGE_CURVE('',#31908,#31909,#9730,.T.) ;
#38745=EDGE_CURVE('',#31909,#31906,#9731,.T.) ;
#38746=EDGE_CURVE('',#31910,#31911,#9732,.T.) ;
#38747=EDGE_CURVE('',#31911,#31912,#9733,.T.) ;
#38748=EDGE_CURVE('',#31912,#31913,#9734,.T.) ;
#38749=EDGE_CURVE('',#31913,#31910,#9735,.T.) ;
#38750=EDGE_CURVE('',#31914,#31915,#9736,.T.) ;
#38751=EDGE_CURVE('',#31915,#31916,#9737,.T.) ;
#38752=EDGE_CURVE('',#31916,#31917,#9738,.T.) ;
#38753=EDGE_CURVE('',#31914,#31917,#9739,.T.) ;
#38754=EDGE_CURVE('',#31784,#31914,#26630,.T.) ;
#38755=EDGE_CURVE('',#31917,#31779,#26631,.T.) ;
#38756=EDGE_CURVE('',#31918,#31919,#9740,.T.) ;
#38757=EDGE_CURVE('',#31919,#31920,#9741,.T.) ;
#38758=EDGE_CURVE('',#31920,#31921,#9742,.T.) ;
#38759=EDGE_CURVE('',#31921,#31918,#9743,.T.) ;
#38760=EDGE_CURVE('',#31922,#31923,#9744,.T.) ;
#38761=EDGE_CURVE('',#31923,#31924,#9745,.T.) ;
#38762=EDGE_CURVE('',#31924,#31925,#9746,.T.) ;
#38763=EDGE_CURVE('',#31925,#31922,#9747,.T.) ;
#38764=EDGE_CURVE('',#31926,#31927,#9748,.T.) ;
#38765=EDGE_CURVE('',#31927,#31928,#9749,.T.) ;
#38766=EDGE_CURVE('',#31928,#31929,#9750,.T.) ;
#38767=EDGE_CURVE('',#31929,#31926,#9751,.T.) ;
#38768=EDGE_CURVE('',#31930,#31931,#9752,.T.) ;
#38769=EDGE_CURVE('',#31931,#31932,#9753,.T.) ;
#38770=EDGE_CURVE('',#31932,#31933,#9754,.T.) ;
#38771=EDGE_CURVE('',#31933,#31930,#9755,.T.) ;
#38772=EDGE_CURVE('',#31683,#31934,#9756,.T.) ;
#38773=EDGE_CURVE('',#31934,#31935,#26632,.T.) ;
#38774=EDGE_CURVE('',#31935,#31684,#9757,.T.) ;
#38775=EDGE_CURVE('',#31936,#31937,#26633,.T.) ;
#38776=EDGE_CURVE('',#31937,#31608,#26634,.T.) ;
#38777=EDGE_CURVE('',#31607,#31936,#26635,.T.) ;
#38778=EDGE_CURVE('',#31663,#31938,#9758,.T.) ;
#38779=EDGE_CURVE('',#31938,#31939,#26636,.T.) ;
#38780=EDGE_CURVE('',#31939,#31664,#9759,.T.) ;
#38781=EDGE_CURVE('',#31852,#31845,#26637,.T.) ;
#38782=EDGE_CURVE('',#31852,#31841,#26638,.T.) ;
#38783=EDGE_CURVE('',#31841,#31845,#26639,.T.) ;
#38784=EDGE_CURVE('',#31844,#31734,#26640,.T.) ;
#38785=EDGE_CURVE('',#31842,#31844,#26641,.T.) ;
#38786=EDGE_CURVE('',#31850,#31840,#26642,.T.) ;
#38787=EDGE_CURVE('',#31842,#31733,#26643,.T.) ;
#38788=EDGE_CURVE('',#31850,#31849,#26644,.T.) ;
#38789=EDGE_CURVE('',#31849,#31840,#26645,.T.) ;
#38790=EDGE_CURVE('',#31830,#31828,#26646,.T.) ;
#38791=EDGE_CURVE('',#31831,#31835,#26647,.T.) ;
#38792=EDGE_CURVE('',#31832,#31830,#26648,.T.) ;
#38793=EDGE_CURVE('',#31725,#31831,#26649,.T.) ;
#38794=EDGE_CURVE('',#31843,#31732,#26650,.T.) ;
#38795=EDGE_CURVE('',#31846,#31843,#26651,.T.) ;
#38796=EDGE_CURVE('',#31851,#31848,#26652,.T.) ;
#38797=EDGE_CURVE('',#31717,#31851,#26653,.T.) ;
#38798=EDGE_CURVE('',#31832,#31828,#26654,.T.) ;
#38799=EDGE_CURVE('',#31726,#31835,#26655,.T.) ;
#38800=EDGE_CURVE('',#31846,#31731,#26656,.T.) ;
#38801=EDGE_CURVE('',#31717,#31848,#26657,.T.) ;
#38802=EDGE_CURVE('',#31833,#31827,#26658,.T.) ;
#38803=EDGE_CURVE('',#31834,#31839,#26659,.T.) ;
#38804=EDGE_CURVE('',#31836,#31833,#26660,.T.) ;
#38805=EDGE_CURVE('',#31727,#31834,#26661,.T.) ;
#38806=EDGE_CURVE('',#31847,#31730,#26662,.T.) ;
#38807=EDGE_CURVE('',#31718,#31847,#26663,.T.) ;
#38808=EDGE_CURVE('',#31836,#31827,#26664,.T.) ;
#38809=EDGE_CURVE('',#31728,#31839,#26665,.T.) ;
#38810=EDGE_CURVE('',#31719,#31730,#26666,.T.) ;
#38811=EDGE_CURVE('',#31829,#31722,#26667,.T.) ;
#38812=EDGE_CURVE('',#31837,#31829,#26668,.T.) ;
#38813=EDGE_CURVE('',#31729,#31838,#26669,.T.) ;
#38814=EDGE_CURVE('',#31720,#31729,#26670,.T.) ;
#38815=EDGE_CURVE('',#31837,#31722,#26671,.T.) ;
#38816=EDGE_CURVE('',#31721,#31838,#26672,.T.) ;
#38817=EDGE_CURVE('',#31785,#31766,#26673,.T.) ;
#38818=EDGE_CURVE('',#31774,#31785,#26674,.T.) ;
#38819=EDGE_CURVE('',#31766,#31774,#26675,.T.) ;
#38820=EDGE_CURVE('',#31792,#31940,#265,.T.) ;
#38821=EDGE_CURVE('',#31940,#31771,#4957,.T.) ;
#38822=EDGE_CURVE('',#31773,#31941,#4958,.T.) ;
#38823=EDGE_CURVE('',#31941,#31759,#266,.T.) ;
#38824=EDGE_CURVE('',#31786,#31765,#26676,.T.) ;
#38825=EDGE_CURVE('',#31781,#31942,#4959,.T.) ;
#38826=EDGE_CURVE('',#31942,#31792,#267,.T.) ;
#38827=EDGE_CURVE('',#31791,#31943,#268,.T.) ;
#38828=EDGE_CURVE('',#31943,#31782,#4960,.T.) ;
#38829=EDGE_CURVE('',#31759,#31944,#269,.T.) ;
#38830=EDGE_CURVE('',#31944,#31776,#4961,.T.) ;
#38831=EDGE_CURVE('',#31775,#31945,#4962,.T.) ;
#38832=EDGE_CURVE('',#31945,#31760,#270,.T.) ;
#38833=EDGE_CURVE('',#31786,#31757,#26677,.T.) ;
#38834=EDGE_CURVE('',#31756,#31765,#26678,.T.) ;
#38835=EDGE_CURVE('',#31946,#31757,#9760,.T.) ;
#38836=EDGE_CURVE('',#31787,#31946,#26679,.T.) ;
#38837=EDGE_CURVE('',#31947,#31946,#26680,.T.) ;
#38838=EDGE_CURVE('',#31787,#31947,#26681,.T.) ;
#38839=EDGE_CURVE('',#31770,#31948,#4963,.T.) ;
#38840=EDGE_CURVE('',#31948,#31791,#271,.T.) ;
#38841=EDGE_CURVE('',#31767,#31790,#26682,.T.) ;
#38842=EDGE_CURVE('',#31760,#31949,#272,.T.) ;
#38843=EDGE_CURVE('',#31949,#31768,#4964,.T.) ;
#38844=EDGE_CURVE('',#31761,#31767,#26683,.T.) ;
#38845=EDGE_CURVE('',#31950,#31764,#26684,.T.) ;
#38846=EDGE_CURVE('',#31756,#31950,#9761,.T.) ;
#38847=EDGE_CURVE('',#31745,#31758,#4965,.T.) ;
#38848=EDGE_CURVE('',#31946,#31743,#26685,.T.) ;
#38849=EDGE_CURVE('',#31947,#31744,#26686,.T.) ;
#38850=EDGE_CURVE('',#31951,#31947,#9762,.T.) ;
#38851=EDGE_CURVE('',#31788,#31951,#26687,.T.) ;
#38852=EDGE_CURVE('',#31761,#31790,#26688,.T.) ;
#38853=EDGE_CURVE('',#31950,#31952,#26689,.T.) ;
#38854=EDGE_CURVE('',#31952,#31764,#26690,.T.) ;
#38855=EDGE_CURVE('',#31751,#31950,#26691,.T.) ;
#38856=EDGE_CURVE('',#31951,#31748,#26692,.T.) ;
#38857=EDGE_CURVE('',#31953,#31951,#26693,.T.) ;
#38858=EDGE_CURVE('',#31788,#31953,#26694,.T.) ;
#38859=EDGE_CURVE('',#31762,#31789,#26695,.T.) ;
#38860=EDGE_CURVE('',#31954,#31763,#26696,.T.) ;
#38861=EDGE_CURVE('',#31952,#31954,#9763,.T.) ;
#38862=EDGE_CURVE('',#31752,#31952,#26697,.T.) ;
#38863=EDGE_CURVE('',#31953,#31747,#26698,.T.) ;
#38864=EDGE_CURVE('',#31753,#31953,#9764,.T.) ;
#38865=EDGE_CURVE('',#31789,#31753,#26699,.T.) ;
#38866=EDGE_CURVE('',#31762,#31755,#26700,.T.) ;
#38867=EDGE_CURVE('',#31954,#31955,#26701,.T.) ;
#38868=EDGE_CURVE('',#31955,#31763,#26702,.T.) ;
#38869=EDGE_CURVE('',#31750,#31954,#26703,.T.) ;
#38870=EDGE_CURVE('',#31754,#31746,#4966,.T.) ;
#38871=EDGE_CURVE('',#31955,#31755,#9765,.T.) ;
#38872=EDGE_CURVE('',#31749,#31955,#26704,.T.) ;
#38873=EDGE_CURVE('',#31803,#31807,#26705,.T.) ;
#38874=EDGE_CURVE('',#31803,#31811,#26706,.T.) ;
#38875=EDGE_CURVE('',#31811,#31807,#26707,.T.) ;
#38876=EDGE_CURVE('',#31806,#31723,#26708,.T.) ;
#38877=EDGE_CURVE('',#31812,#31806,#26709,.T.) ;
#38878=EDGE_CURVE('',#31804,#31810,#26710,.T.) ;
#38879=EDGE_CURVE('',#31635,#31801,#26711,.T.) ;
#38880=EDGE_CURVE('',#31606,#31636,#26712,.T.) ;
#38881=EDGE_CURVE('',#31609,#31635,#26713,.T.) ;
#38882=EDGE_CURVE('',#31812,#31724,#26714,.T.) ;
#38883=EDGE_CURVE('',#31804,#31808,#26715,.T.) ;
#38884=EDGE_CURVE('',#31808,#31810,#26716,.T.) ;
#38885=EDGE_CURVE('',#31609,#31802,#26717,.T.) ;
#38886=EDGE_CURVE('',#31813,#31742,#26718,.T.) ;
#38887=EDGE_CURVE('',#31809,#31813,#26719,.T.) ;
#38888=EDGE_CURVE('',#31805,#31604,#26720,.T.) ;
#38889=EDGE_CURVE('',#31603,#31805,#26721,.T.) ;
#38890=EDGE_CURVE('',#31641,#31605,#26722,.T.) ;
#38891=EDGE_CURVE('',#31642,#31612,#26723,.T.) ;
#38892=EDGE_CURVE('',#31824,#31642,#26724,.T.) ;
#38893=EDGE_CURVE('',#31820,#31823,#26725,.T.) ;
#38894=EDGE_CURVE('',#31809,#31741,#26726,.T.) ;
#38895=EDGE_CURVE('',#31825,#31612,#26727,.T.) ;
#38896=EDGE_CURVE('',#31820,#31814,#26728,.T.) ;
#38897=EDGE_CURVE('',#31814,#31823,#26729,.T.) ;
#38898=EDGE_CURVE('',#31602,#31740,#273,.T.) ;
#38899=EDGE_CURVE('',#31826,#31600,#26730,.T.) ;
#38900=EDGE_CURVE('',#31822,#31819,#26731,.T.) ;
#38901=EDGE_CURVE('',#31598,#31826,#26732,.T.) ;
#38902=EDGE_CURVE('',#31815,#31822,#26733,.T.) ;
#38903=EDGE_CURVE('',#31821,#31817,#26734,.T.) ;
#38904=EDGE_CURVE('',#31735,#31821,#26735,.T.) ;
#38905=EDGE_CURVE('',#31610,#31740,#26736,.T.) ;
#38906=EDGE_CURVE('',#31956,#31599,#26737,.T.) ;
#38907=EDGE_CURVE('',#31815,#31819,#26738,.T.) ;
#38908=EDGE_CURVE('',#31736,#31817,#26739,.T.) ;
#38909=EDGE_CURVE('',#31611,#31739,#26740,.T.) ;
#38910=EDGE_CURVE('',#31816,#31818,#26741,.T.) ;
#38911=EDGE_CURVE('',#31737,#31816,#26742,.T.) ;
#38912=EDGE_CURVE('',#31596,#31739,#274,.T.) ;
#38913=EDGE_CURVE('',#31738,#31818,#26743,.T.) ;
#38914=EDGE_CURVE('',#31615,#31896,#275,.T.) ;
#38915=EDGE_CURVE('',#31899,#31895,#26744,.T.) ;
#38916=EDGE_CURVE('',#31894,#31900,#26745,.T.) ;
#38917=EDGE_CURVE('',#31897,#31780,#276,.T.) ;
#38918=EDGE_CURVE('',#31892,#31917,#26746,.T.) ;
#38919=EDGE_CURVE('',#31904,#31931,#26747,.T.) ;
#38920=EDGE_CURVE('',#31905,#31930,#26748,.T.) ;
#38921=EDGE_CURVE('',#31891,#31618,#277,.T.) ;
#38922=EDGE_CURVE('',#31886,#31898,#26749,.T.) ;
#38923=EDGE_CURVE('',#31916,#31893,#26750,.T.) ;
#38924=EDGE_CURVE('',#31905,#31909,#26751,.T.) ;
#38925=EDGE_CURVE('',#31909,#31930,#26752,.T.) ;
#38926=EDGE_CURVE('',#31901,#31887,#26753,.T.) ;
#38927=EDGE_CURVE('',#31932,#31911,#26754,.T.) ;
#38928=EDGE_CURVE('',#31933,#31910,#26755,.T.) ;
#38929=EDGE_CURVE('',#31906,#31933,#26756,.T.) ;
#38930=EDGE_CURVE('',#31902,#31908,#26757,.T.) ;
#38931=EDGE_CURVE('',#31928,#31903,#26758,.T.) ;
#38932=EDGE_CURVE('',#31929,#31902,#26759,.T.) ;
#38933=EDGE_CURVE('',#31906,#31910,#26760,.T.) ;
#38934=EDGE_CURVE('',#31929,#31908,#26761,.T.) ;
#38935=EDGE_CURVE('',#31907,#31913,#26762,.T.) ;
#38936=EDGE_CURVE('',#31926,#31907,#26763,.T.) ;
#38937=EDGE_CURVE('',#31926,#31913,#26764,.T.) ;
#38938=EDGE_CURVE('',#31912,#31927,#26765,.T.) ;
#38939=EDGE_CURVE('',#31888,#31915,#26766,.T.) ;
#38940=EDGE_CURVE('',#31889,#31914,#26767,.T.) ;
#38941=EDGE_CURVE('',#31783,#31890,#278,.T.) ;
#38942=EDGE_CURVE('',#31881,#31882,#26768,.T.) ;
#38943=EDGE_CURVE('',#31885,#31880,#26769,.T.) ;
#38944=EDGE_CURVE('',#31868,#31919,#26770,.T.) ;
#38945=EDGE_CURVE('',#31869,#31918,#26771,.T.) ;
#38946=EDGE_CURVE('',#31920,#31875,#26772,.T.) ;
#38947=EDGE_CURVE('',#31921,#31874,#26773,.T.) ;
#38948=EDGE_CURVE('',#31918,#31873,#26774,.T.) ;
#38949=EDGE_CURVE('',#31870,#31921,#26775,.T.) ;
#38950=EDGE_CURVE('',#31869,#31873,#26776,.T.) ;
#38951=EDGE_CURVE('',#31883,#31878,#26777,.T.) ;
#38952=EDGE_CURVE('',#31879,#31884,#26778,.T.) ;
#38953=EDGE_CURVE('',#31870,#31874,#26779,.T.) ;
#38954=EDGE_CURVE('',#31866,#31872,#26780,.T.) ;
#38955=EDGE_CURVE('',#31924,#31867,#26781,.T.) ;
#38956=EDGE_CURVE('',#31925,#31866,#26782,.T.) ;
#38957=EDGE_CURVE('',#31876,#31923,#26783,.T.) ;
#38958=EDGE_CURVE('',#31877,#31922,#26784,.T.) ;
#38959=EDGE_CURVE('',#31871,#31877,#26785,.T.) ;
#38960=EDGE_CURVE('',#31925,#31872,#26786,.T.) ;
#38961=EDGE_CURVE('',#31871,#31922,#26787,.T.) ;
#38962=EDGE_CURVE('',#31629,#31628,#26788,.T.) ;
#38963=EDGE_CURVE('',#31855,#31630,#279,.T.) ;
#38964=EDGE_CURVE('',#31856,#31629,#26789,.T.) ;
#38965=EDGE_CURVE('',#31856,#31628,#26790,.T.) ;
#38966=EDGE_CURVE('',#31627,#31624,#26791,.T.) ;
#38967=EDGE_CURVE('',#31853,#31627,#26792,.T.) ;
#38968=EDGE_CURVE('',#31853,#31624,#26793,.T.) ;
#38969=EDGE_CURVE('',#31623,#31854,#280,.T.) ;
#38970=EDGE_CURVE('',#31585,#31864,#4967,.T.) ;
#38971=EDGE_CURVE('',#31712,#31863,#26794,.T.) ;
#38972=EDGE_CURVE('',#31709,#31712,#26795,.T.) ;
#38973=EDGE_CURVE('',#31709,#31863,#26796,.T.) ;
#38974=EDGE_CURVE('',#31710,#31865,#26797,.T.) ;
#38975=EDGE_CURVE('',#31708,#31710,#26798,.T.) ;
#38976=EDGE_CURVE('',#31708,#31865,#26799,.T.) ;
#38977=EDGE_CURVE('',#31589,#31705,#4968,.T.) ;
#38978=EDGE_CURVE('',#31777,#31614,#26800,.T.) ;
#38979=EDGE_CURVE('',#31613,#31778,#26801,.T.) ;
#38980=EDGE_CURVE('',#31939,#31647,#26802,.T.) ;
#38981=EDGE_CURVE('',#31936,#31648,#26803,.T.) ;
#38982=EDGE_CURVE('',#31647,#31937,#26804,.T.) ;
#38983=EDGE_CURVE('',#31648,#31934,#26805,.T.) ;
#38984=EDGE_CURVE('',#31771,#31781,#26806,.T.) ;
#38985=EDGE_CURVE('',#31772,#31614,#26807,.T.) ;
#38986=EDGE_CURVE('',#31772,#31777,#26808,.T.) ;
#38987=EDGE_CURVE('',#31773,#31776,#26809,.T.) ;
#38988=EDGE_CURVE('',#31768,#31775,#26810,.T.) ;
#38989=EDGE_CURVE('',#31769,#31778,#26811,.T.) ;
#38990=EDGE_CURVE('',#31769,#31613,#26812,.T.) ;
#38991=EDGE_CURVE('',#31770,#31782,#26813,.T.) ;
#38992=EDGE_CURVE('',#31622,#31858,#281,.T.) ;
#38993=EDGE_CURVE('',#31854,#31857,#26814,.T.) ;
#38994=EDGE_CURVE('',#31855,#31862,#26815,.T.) ;
#38995=EDGE_CURVE('',#31957,#31861,#282,.T.) ;
#38996=EDGE_CURVE('',#31958,#31957,#283,.T.) ;
#38997=EDGE_CURVE('',#31959,#31958,#284,.T.) ;
#38998=EDGE_CURVE('',#31631,#31959,#285,.T.) ;
#38999=EDGE_CURVE('',#31713,#31632,#4969,.T.) ;
#39000=EDGE_CURVE('',#31714,#31861,#26816,.T.) ;
#39001=EDGE_CURVE('',#31588,#31706,#286,.T.) ;
#39002=EDGE_CURVE('',#31715,#31860,#26817,.T.) ;
#39003=EDGE_CURVE('',#31711,#31716,#4970,.T.) ;
#39004=EDGE_CURVE('',#31859,#31864,#26818,.T.) ;
#39005=EDGE_CURVE('',#31960,#31860,#287,.T.) ;
#39006=EDGE_CURVE('',#31961,#31960,#288,.T.) ;
#39007=EDGE_CURVE('',#31584,#31961,#289,.T.) ;
#39008=EDGE_CURVE('',#31641,#31935,#26819,.T.) ;
#39009=EDGE_CURVE('',#31607,#31935,#26820,.T.) ;
#39010=EDGE_CURVE('',#31936,#31934,#26821,.T.) ;
#39011=EDGE_CURVE('',#31904,#31900,#26822,.T.) ;
#39012=EDGE_CURVE('',#31931,#31894,#26823,.T.) ;
#39013=EDGE_CURVE('',#31901,#31903,#26824,.T.) ;
#39014=EDGE_CURVE('',#31932,#31893,#26825,.T.) ;
#39015=EDGE_CURVE('',#31887,#31928,#26826,.T.) ;
#39016=EDGE_CURVE('',#31911,#31916,#26827,.T.) ;
#39017=EDGE_CURVE('',#31888,#31927,#26828,.T.) ;
#39018=EDGE_CURVE('',#31912,#31915,#26829,.T.) ;
#39019=EDGE_CURVE('',#31868,#31882,#26830,.T.) ;
#39020=EDGE_CURVE('',#31919,#31881,#26831,.T.) ;
#39021=EDGE_CURVE('',#31883,#31867,#26832,.T.) ;
#39022=EDGE_CURVE('',#31920,#31880,#26833,.T.) ;
#39023=EDGE_CURVE('',#31878,#31924,#26834,.T.) ;
#39024=EDGE_CURVE('',#31875,#31885,#26835,.T.) ;
#39025=EDGE_CURVE('',#31879,#31923,#26836,.T.) ;
#39026=EDGE_CURVE('',#31876,#31884,#26837,.T.) ;
#39027=EDGE_CURVE('',#31938,#31636,#26838,.T.) ;
#39028=EDGE_CURVE('',#31938,#31608,#26839,.T.) ;
#39029=EDGE_CURVE('',#31939,#31937,#26840,.T.) ;
#39030=EDGE_CURVE('',#31703,#31707,#4971,.T.) ;
#39031=EDGE_CURVE('',#31704,#31587,#26841,.T.) ;
#39032=EDGE_CURVE('',#31701,#31858,#26842,.T.) ;
#39033=EDGE_CURVE('',#31702,#31621,#4972,.T.) ;
#46100=ORIENTED_EDGE('',*,*,#35709,.T.) ;
#46101=ORIENTED_EDGE('',*,*,#35710,.T.) ;
#46102=ORIENTED_EDGE('',*,*,#35711,.T.) ;
#46103=ORIENTED_EDGE('',*,*,#35712,.F.) ;
#46104=ORIENTED_EDGE('',*,*,#35713,.F.) ;
#46105=ORIENTED_EDGE('',*,*,#35714,.T.) ;
#46106=ORIENTED_EDGE('',*,*,#35715,.T.) ;
#46107=ORIENTED_EDGE('',*,*,#35716,.F.) ;
#46108=ORIENTED_EDGE('',*,*,#35717,.F.) ;
#46109=ORIENTED_EDGE('',*,*,#35718,.F.) ;
#46110=ORIENTED_EDGE('',*,*,#35719,.F.) ;
#46111=ORIENTED_EDGE('',*,*,#35720,.T.) ;
#46112=ORIENTED_EDGE('',*,*,#35721,.F.) ;
#46113=ORIENTED_EDGE('',*,*,#35720,.F.) ;
#46114=ORIENTED_EDGE('',*,*,#35722,.F.) ;
#46115=ORIENTED_EDGE('',*,*,#35723,.T.) ;
#46116=ORIENTED_EDGE('',*,*,#35724,.F.) ;
#46117=ORIENTED_EDGE('',*,*,#35723,.F.) ;
#46118=ORIENTED_EDGE('',*,*,#35725,.F.) ;
#46119=ORIENTED_EDGE('',*,*,#35726,.F.) ;
#46120=ORIENTED_EDGE('',*,*,#35727,.T.) ;
#46121=ORIENTED_EDGE('',*,*,#35728,.T.) ;
#46122=ORIENTED_EDGE('',*,*,#35729,.F.) ;
#46123=ORIENTED_EDGE('',*,*,#35730,.F.) ;
#46124=ORIENTED_EDGE('',*,*,#35731,.F.) ;
#46125=ORIENTED_EDGE('',*,*,#35732,.T.) ;
#46126=ORIENTED_EDGE('',*,*,#35733,.F.) ;
#46127=ORIENTED_EDGE('',*,*,#35734,.F.) ;
#46128=ORIENTED_EDGE('',*,*,#35735,.T.) ;
#46129=ORIENTED_EDGE('',*,*,#35736,.F.) ;
#46130=ORIENTED_EDGE('',*,*,#35737,.T.) ;
#46131=ORIENTED_EDGE('',*,*,#35721,.T.) ;
#46132=ORIENTED_EDGE('',*,*,#35738,.T.) ;
#46133=ORIENTED_EDGE('',*,*,#35722,.T.) ;
#46134=ORIENTED_EDGE('',*,*,#35738,.F.) ;
#46135=ORIENTED_EDGE('',*,*,#35734,.T.) ;
#46136=ORIENTED_EDGE('',*,*,#35739,.T.) ;
#46137=ORIENTED_EDGE('',*,*,#35740,.T.) ;
#46138=ORIENTED_EDGE('',*,*,#35731,.T.) ;
#46139=ORIENTED_EDGE('',*,*,#35741,.F.) ;
#46140=ORIENTED_EDGE('',*,*,#35742,.T.) ;
#46141=ORIENTED_EDGE('',*,*,#35743,.F.) ;
#46142=ORIENTED_EDGE('',*,*,#35729,.T.) ;
#46143=ORIENTED_EDGE('',*,*,#35744,.T.) ;
#46144=ORIENTED_EDGE('',*,*,#35745,.T.) ;
#46145=ORIENTED_EDGE('',*,*,#35746,.T.) ;
#46146=ORIENTED_EDGE('',*,*,#35747,.T.) ;
#46147=ORIENTED_EDGE('',*,*,#35748,.T.) ;
#46148=ORIENTED_EDGE('',*,*,#35749,.T.) ;
#46149=ORIENTED_EDGE('',*,*,#35750,.T.) ;
#46150=ORIENTED_EDGE('',*,*,#35751,.T.) ;
#46151=ORIENTED_EDGE('',*,*,#35752,.T.) ;
#46152=ORIENTED_EDGE('',*,*,#35753,.T.) ;
#46153=ORIENTED_EDGE('',*,*,#35754,.T.) ;
#46154=ORIENTED_EDGE('',*,*,#35755,.T.) ;
#46155=ORIENTED_EDGE('',*,*,#35756,.T.) ;
#46156=ORIENTED_EDGE('',*,*,#35757,.T.) ;
#46157=ORIENTED_EDGE('',*,*,#35758,.T.) ;
#46158=ORIENTED_EDGE('',*,*,#35759,.T.) ;
#46159=ORIENTED_EDGE('',*,*,#35760,.T.) ;
#46160=ORIENTED_EDGE('',*,*,#35761,.T.) ;
#46161=ORIENTED_EDGE('',*,*,#35762,.T.) ;
#46162=ORIENTED_EDGE('',*,*,#35763,.T.) ;
#46163=ORIENTED_EDGE('',*,*,#35764,.T.) ;
#46164=ORIENTED_EDGE('',*,*,#35765,.T.) ;
#46165=ORIENTED_EDGE('',*,*,#35766,.T.) ;
#46166=ORIENTED_EDGE('',*,*,#35767,.T.) ;
#46167=ORIENTED_EDGE('',*,*,#35768,.T.) ;
#46168=ORIENTED_EDGE('',*,*,#35769,.T.) ;
#46169=ORIENTED_EDGE('',*,*,#35770,.T.) ;
#46170=ORIENTED_EDGE('',*,*,#35771,.T.) ;
#46171=ORIENTED_EDGE('',*,*,#35772,.F.) ;
#46172=ORIENTED_EDGE('',*,*,#35773,.T.) ;
#46173=ORIENTED_EDGE('',*,*,#35774,.T.) ;
#46174=ORIENTED_EDGE('',*,*,#35775,.T.) ;
#46175=ORIENTED_EDGE('',*,*,#35776,.F.) ;
#46176=ORIENTED_EDGE('',*,*,#35777,.T.) ;
#46177=ORIENTED_EDGE('',*,*,#35778,.T.) ;
#46178=ORIENTED_EDGE('',*,*,#35779,.T.) ;
#46179=ORIENTED_EDGE('',*,*,#35780,.T.) ;
#46180=ORIENTED_EDGE('',*,*,#35781,.T.) ;
#46181=ORIENTED_EDGE('',*,*,#35782,.F.) ;
#46182=ORIENTED_EDGE('',*,*,#35783,.T.) ;
#46183=ORIENTED_EDGE('',*,*,#35752,.F.) ;
#46184=ORIENTED_EDGE('',*,*,#35784,.T.) ;
#46185=ORIENTED_EDGE('',*,*,#35758,.F.) ;
#46186=ORIENTED_EDGE('',*,*,#35785,.T.) ;
#46187=ORIENTED_EDGE('',*,*,#35766,.F.) ;
#46188=ORIENTED_EDGE('',*,*,#35786,.T.) ;
#46189=ORIENTED_EDGE('',*,*,#35787,.F.) ;
#46190=ORIENTED_EDGE('',*,*,#35788,.T.) ;
#46191=ORIENTED_EDGE('',*,*,#35789,.F.) ;
#46192=ORIENTED_EDGE('',*,*,#35790,.T.) ;
#46193=ORIENTED_EDGE('',*,*,#35791,.T.) ;
#46194=ORIENTED_EDGE('',*,*,#35792,.T.) ;
#46195=ORIENTED_EDGE('',*,*,#35793,.F.) ;
#46196=ORIENTED_EDGE('',*,*,#35794,.T.) ;
#46197=ORIENTED_EDGE('',*,*,#35795,.T.) ;
#46198=ORIENTED_EDGE('',*,*,#35796,.T.) ;
#46199=ORIENTED_EDGE('',*,*,#35797,.F.) ;
#46200=ORIENTED_EDGE('',*,*,#35798,.T.) ;
#46201=ORIENTED_EDGE('',*,*,#35770,.F.) ;
#46202=ORIENTED_EDGE('',*,*,#35799,.T.) ;
#46203=ORIENTED_EDGE('',*,*,#35800,.T.) ;
#46204=ORIENTED_EDGE('',*,*,#35801,.T.) ;
#46205=ORIENTED_EDGE('',*,*,#35778,.F.) ;
#46206=ORIENTED_EDGE('',*,*,#35802,.T.) ;
#46207=ORIENTED_EDGE('',*,*,#35803,.F.) ;
#46208=ORIENTED_EDGE('',*,*,#35804,.F.) ;
#46209=ORIENTED_EDGE('',*,*,#35805,.T.) ;
#46210=ORIENTED_EDGE('',*,*,#35806,.F.) ;
#46211=ORIENTED_EDGE('',*,*,#35807,.T.) ;
#46212=ORIENTED_EDGE('',*,*,#35808,.F.) ;
#46213=ORIENTED_EDGE('',*,*,#35809,.T.) ;
#46214=ORIENTED_EDGE('',*,*,#35810,.T.) ;
#46215=ORIENTED_EDGE('',*,*,#35811,.T.) ;
#46216=ORIENTED_EDGE('',*,*,#35812,.T.) ;
#46217=ORIENTED_EDGE('',*,*,#35813,.T.) ;
#46218=ORIENTED_EDGE('',*,*,#35814,.T.) ;
#46219=ORIENTED_EDGE('',*,*,#35815,.T.) ;
#46220=ORIENTED_EDGE('',*,*,#35816,.T.) ;
#46221=ORIENTED_EDGE('',*,*,#35817,.T.) ;
#46222=ORIENTED_EDGE('',*,*,#35818,.T.) ;
#46223=ORIENTED_EDGE('',*,*,#35819,.T.) ;
#46224=ORIENTED_EDGE('',*,*,#35820,.T.) ;
#46225=ORIENTED_EDGE('',*,*,#35776,.T.) ;
#46226=ORIENTED_EDGE('',*,*,#35821,.T.) ;
#46227=ORIENTED_EDGE('',*,*,#35822,.T.) ;
#46228=ORIENTED_EDGE('',*,*,#35823,.T.) ;
#46229=ORIENTED_EDGE('',*,*,#35772,.T.) ;
#46230=ORIENTED_EDGE('',*,*,#35824,.T.) ;
#46231=ORIENTED_EDGE('',*,*,#35825,.F.) ;
#46232=ORIENTED_EDGE('',*,*,#35826,.T.) ;
#46233=ORIENTED_EDGE('',*,*,#35827,.F.) ;
#46234=ORIENTED_EDGE('',*,*,#35828,.T.) ;
#46235=ORIENTED_EDGE('',*,*,#35829,.T.) ;
#46236=ORIENTED_EDGE('',*,*,#35830,.T.) ;
#46237=ORIENTED_EDGE('',*,*,#35831,.F.) ;
#46238=ORIENTED_EDGE('',*,*,#35832,.T.) ;
#46239=ORIENTED_EDGE('',*,*,#35833,.F.) ;
#46240=ORIENTED_EDGE('',*,*,#35834,.T.) ;
#46241=ORIENTED_EDGE('',*,*,#35835,.T.) ;
#46242=ORIENTED_EDGE('',*,*,#35836,.T.) ;
#46243=ORIENTED_EDGE('',*,*,#35837,.T.) ;
#46244=ORIENTED_EDGE('',*,*,#35838,.T.) ;
#46245=ORIENTED_EDGE('',*,*,#35839,.T.) ;
#46246=ORIENTED_EDGE('',*,*,#35840,.T.) ;
#46247=ORIENTED_EDGE('',*,*,#35806,.T.) ;
#46248=ORIENTED_EDGE('',*,*,#35841,.T.) ;
#46249=ORIENTED_EDGE('',*,*,#35816,.F.) ;
#46250=ORIENTED_EDGE('',*,*,#35842,.T.) ;
#46251=ORIENTED_EDGE('',*,*,#35808,.T.) ;
#46252=ORIENTED_EDGE('',*,*,#35843,.T.) ;
#46253=ORIENTED_EDGE('',*,*,#35814,.F.) ;
#46254=ORIENTED_EDGE('',*,*,#35844,.T.) ;
#46255=ORIENTED_EDGE('',*,*,#35845,.T.) ;
#46256=ORIENTED_EDGE('',*,*,#35846,.T.) ;
#46257=ORIENTED_EDGE('',*,*,#35782,.T.) ;
#46258=ORIENTED_EDGE('',*,*,#35847,.T.) ;
#46259=ORIENTED_EDGE('',*,*,#35812,.F.) ;
#46260=ORIENTED_EDGE('',*,*,#35848,.T.) ;
#46261=ORIENTED_EDGE('',*,*,#35849,.T.) ;
#46262=ORIENTED_EDGE('',*,*,#35850,.T.) ;
#46263=ORIENTED_EDGE('',*,*,#35851,.T.) ;
#46264=ORIENTED_EDGE('',*,*,#35852,.T.) ;
#46265=ORIENTED_EDGE('',*,*,#35853,.T.) ;
#46266=ORIENTED_EDGE('',*,*,#35810,.F.) ;
#46267=ORIENTED_EDGE('',*,*,#35854,.T.) ;
#46268=ORIENTED_EDGE('',*,*,#35855,.T.) ;
#46269=ORIENTED_EDGE('',*,*,#35856,.T.) ;
#46270=ORIENTED_EDGE('',*,*,#35857,.T.) ;
#46271=ORIENTED_EDGE('',*,*,#35839,.F.) ;
#46272=ORIENTED_EDGE('',*,*,#35858,.T.) ;
#46273=ORIENTED_EDGE('',*,*,#35859,.T.) ;
#46274=ORIENTED_EDGE('',*,*,#35713,.T.) ;
#46275=ORIENTED_EDGE('',*,*,#35860,.T.) ;
#46276=ORIENTED_EDGE('',*,*,#35861,.T.) ;
#46277=ORIENTED_EDGE('',*,*,#35837,.F.) ;
#46278=ORIENTED_EDGE('',*,*,#35862,.T.) ;
#46279=ORIENTED_EDGE('',*,*,#35863,.T.) ;
#46280=ORIENTED_EDGE('',*,*,#35864,.T.) ;
#46281=ORIENTED_EDGE('',*,*,#35865,.T.) ;
#46282=ORIENTED_EDGE('',*,*,#35866,.T.) ;
#46283=ORIENTED_EDGE('',*,*,#35867,.T.) ;
#46284=ORIENTED_EDGE('',*,*,#35835,.F.) ;
#46285=ORIENTED_EDGE('',*,*,#35868,.T.) ;
#46286=ORIENTED_EDGE('',*,*,#35869,.T.) ;
#46287=ORIENTED_EDGE('',*,*,#35870,.F.) ;
#46288=ORIENTED_EDGE('',*,*,#35871,.T.) ;
#46289=ORIENTED_EDGE('',*,*,#35872,.F.) ;
#46290=ORIENTED_EDGE('',*,*,#35873,.T.) ;
#46291=ORIENTED_EDGE('',*,*,#35874,.T.) ;
#46292=ORIENTED_EDGE('',*,*,#35787,.T.) ;
#46293=ORIENTED_EDGE('',*,*,#35875,.F.) ;
#46294=ORIENTED_EDGE('',*,*,#35876,.T.) ;
#46295=ORIENTED_EDGE('',*,*,#35793,.T.) ;
#46296=ORIENTED_EDGE('',*,*,#35877,.T.) ;
#46297=ORIENTED_EDGE('',*,*,#35878,.F.) ;
#46298=ORIENTED_EDGE('',*,*,#35879,.T.) ;
#46299=ORIENTED_EDGE('',*,*,#35880,.F.) ;
#46300=ORIENTED_EDGE('',*,*,#35881,.T.) ;
#46301=ORIENTED_EDGE('',*,*,#35882,.T.) ;
#46302=ORIENTED_EDGE('',*,*,#35883,.T.) ;
#46303=ORIENTED_EDGE('',*,*,#35884,.F.) ;
#46304=ORIENTED_EDGE('',*,*,#35885,.T.) ;
#46305=ORIENTED_EDGE('',*,*,#35886,.F.) ;
#46306=ORIENTED_EDGE('',*,*,#35887,.T.) ;
#46307=ORIENTED_EDGE('',*,*,#35829,.F.) ;
#46308=ORIENTED_EDGE('',*,*,#35888,.T.) ;
#46309=ORIENTED_EDGE('',*,*,#35889,.F.) ;
#46310=ORIENTED_EDGE('',*,*,#35890,.T.) ;
#46311=ORIENTED_EDGE('',*,*,#35891,.F.) ;
#46312=ORIENTED_EDGE('',*,*,#35892,.T.) ;
#46313=ORIENTED_EDGE('',*,*,#35893,.T.) ;
#46314=ORIENTED_EDGE('',*,*,#35894,.T.) ;
#46315=ORIENTED_EDGE('',*,*,#35895,.F.) ;
#46316=ORIENTED_EDGE('',*,*,#35896,.T.) ;
#46317=ORIENTED_EDGE('',*,*,#35724,.T.) ;
#46318=ORIENTED_EDGE('',*,*,#35897,.F.) ;
#46319=ORIENTED_EDGE('',*,*,#35898,.T.) ;
#46320=ORIENTED_EDGE('',*,*,#35899,.F.) ;
#46321=ORIENTED_EDGE('',*,*,#35803,.T.) ;
#46322=ORIENTED_EDGE('',*,*,#35900,.T.) ;
#46323=ORIENTED_EDGE('',*,*,#35819,.F.) ;
#46324=ORIENTED_EDGE('',*,*,#35901,.F.) ;
#46325=ORIENTED_EDGE('',*,*,#35902,.T.) ;
#46326=ORIENTED_EDGE('',*,*,#35903,.F.) ;
#46327=ORIENTED_EDGE('',*,*,#35904,.T.) ;
#46328=ORIENTED_EDGE('',*,*,#35905,.F.) ;
#46329=ORIENTED_EDGE('',*,*,#35906,.T.) ;
#46330=ORIENTED_EDGE('',*,*,#35901,.T.) ;
#46331=ORIENTED_EDGE('',*,*,#35818,.F.) ;
#46332=ORIENTED_EDGE('',*,*,#35907,.T.) ;
#46333=ORIENTED_EDGE('',*,*,#35804,.T.) ;
#46334=ORIENTED_EDGE('',*,*,#35899,.T.) ;
#46335=ORIENTED_EDGE('',*,*,#35908,.T.) ;
#46336=ORIENTED_EDGE('',*,*,#35909,.F.) ;
#46337=ORIENTED_EDGE('',*,*,#35910,.T.) ;
#46338=ORIENTED_EDGE('',*,*,#35911,.T.) ;
#46339=ORIENTED_EDGE('',*,*,#35912,.T.) ;
#46340=ORIENTED_EDGE('',*,*,#35913,.F.) ;
#46341=ORIENTED_EDGE('',*,*,#35914,.F.) ;
#46342=ORIENTED_EDGE('',*,*,#35915,.T.) ;
#46343=ORIENTED_EDGE('',*,*,#35916,.T.) ;
#46344=ORIENTED_EDGE('',*,*,#35917,.T.) ;
#46345=ORIENTED_EDGE('',*,*,#35918,.T.) ;
#46346=ORIENTED_EDGE('',*,*,#35919,.T.) ;
#46347=ORIENTED_EDGE('',*,*,#35920,.T.) ;
#46348=ORIENTED_EDGE('',*,*,#35921,.T.) ;
#46349=ORIENTED_EDGE('',*,*,#35922,.T.) ;
#46350=ORIENTED_EDGE('',*,*,#35923,.T.) ;
#46351=ORIENTED_EDGE('',*,*,#35924,.T.) ;
#46352=ORIENTED_EDGE('',*,*,#35925,.T.) ;
#46353=ORIENTED_EDGE('',*,*,#35926,.T.) ;
#46354=ORIENTED_EDGE('',*,*,#35927,.T.) ;
#46355=ORIENTED_EDGE('',*,*,#35928,.T.) ;
#46356=ORIENTED_EDGE('',*,*,#35929,.T.) ;
#46357=ORIENTED_EDGE('',*,*,#35930,.T.) ;
#46358=ORIENTED_EDGE('',*,*,#35931,.T.) ;
#46359=ORIENTED_EDGE('',*,*,#35932,.T.) ;
#46360=ORIENTED_EDGE('',*,*,#35933,.T.) ;
#46361=ORIENTED_EDGE('',*,*,#35934,.T.) ;
#46362=ORIENTED_EDGE('',*,*,#35935,.T.) ;
#46363=ORIENTED_EDGE('',*,*,#35936,.T.) ;
#46364=ORIENTED_EDGE('',*,*,#35937,.T.) ;
#46365=ORIENTED_EDGE('',*,*,#35938,.T.) ;
#46366=ORIENTED_EDGE('',*,*,#35939,.T.) ;
#46367=ORIENTED_EDGE('',*,*,#35940,.T.) ;
#46368=ORIENTED_EDGE('',*,*,#35941,.T.) ;
#46369=ORIENTED_EDGE('',*,*,#35942,.T.) ;
#46370=ORIENTED_EDGE('',*,*,#35943,.T.) ;
#46371=ORIENTED_EDGE('',*,*,#35944,.T.) ;
#46372=ORIENTED_EDGE('',*,*,#35945,.T.) ;
#46373=ORIENTED_EDGE('',*,*,#35946,.T.) ;
#46374=ORIENTED_EDGE('',*,*,#35947,.T.) ;
#46375=ORIENTED_EDGE('',*,*,#35948,.T.) ;
#46376=ORIENTED_EDGE('',*,*,#35949,.T.) ;
#46377=ORIENTED_EDGE('',*,*,#35950,.T.) ;
#46378=ORIENTED_EDGE('',*,*,#35719,.T.) ;
#46379=ORIENTED_EDGE('',*,*,#35951,.F.) ;
#46380=ORIENTED_EDGE('',*,*,#35952,.T.) ;
#46381=ORIENTED_EDGE('',*,*,#35953,.T.) ;
#46382=ORIENTED_EDGE('',*,*,#35954,.T.) ;
#46383=ORIENTED_EDGE('',*,*,#35955,.T.) ;
#46384=ORIENTED_EDGE('',*,*,#35956,.T.) ;
#46385=ORIENTED_EDGE('',*,*,#35957,.T.) ;
#46386=ORIENTED_EDGE('',*,*,#35958,.T.) ;
#46387=ORIENTED_EDGE('',*,*,#35959,.F.) ;
#46388=ORIENTED_EDGE('',*,*,#35960,.T.) ;
#46389=ORIENTED_EDGE('',*,*,#35797,.T.) ;
#46390=ORIENTED_EDGE('',*,*,#35961,.T.) ;
#46391=ORIENTED_EDGE('',*,*,#35962,.T.) ;
#46392=ORIENTED_EDGE('',*,*,#35963,.T.) ;
#46393=ORIENTED_EDGE('',*,*,#35964,.T.) ;
#46394=ORIENTED_EDGE('',*,*,#35795,.F.) ;
#46395=ORIENTED_EDGE('',*,*,#35965,.T.) ;
#46396=ORIENTED_EDGE('',*,*,#35966,.T.) ;
#46397=ORIENTED_EDGE('',*,*,#35967,.T.) ;
#46398=ORIENTED_EDGE('',*,*,#35968,.T.) ;
#46399=ORIENTED_EDGE('',*,*,#35969,.T.) ;
#46400=ORIENTED_EDGE('',*,*,#35733,.T.) ;
#46401=ORIENTED_EDGE('',*,*,#35970,.T.) ;
#46402=ORIENTED_EDGE('',*,*,#35971,.T.) ;
#46403=ORIENTED_EDGE('',*,*,#35972,.T.) ;
#46404=ORIENTED_EDGE('',*,*,#35973,.T.) ;
#46405=ORIENTED_EDGE('',*,*,#35974,.T.) ;
#46406=ORIENTED_EDGE('',*,*,#35975,.T.) ;
#46407=ORIENTED_EDGE('',*,*,#35976,.T.) ;
#46408=ORIENTED_EDGE('',*,*,#35977,.T.) ;
#46409=ORIENTED_EDGE('',*,*,#35978,.T.) ;
#46410=ORIENTED_EDGE('',*,*,#35726,.T.) ;
#46411=ORIENTED_EDGE('',*,*,#35979,.T.) ;
#46412=ORIENTED_EDGE('',*,*,#35980,.T.) ;
#46413=ORIENTED_EDGE('',*,*,#35981,.T.) ;
#46414=ORIENTED_EDGE('',*,*,#35982,.T.) ;
#46415=ORIENTED_EDGE('',*,*,#35983,.T.) ;
#46416=ORIENTED_EDGE('',*,*,#35827,.T.) ;
#46417=ORIENTED_EDGE('',*,*,#35984,.T.) ;
#46418=ORIENTED_EDGE('',*,*,#35985,.T.) ;
#46419=ORIENTED_EDGE('',*,*,#35986,.T.) ;
#46420=ORIENTED_EDGE('',*,*,#35825,.T.) ;
#46421=ORIENTED_EDGE('',*,*,#35987,.T.) ;
#46422=ORIENTED_EDGE('',*,*,#35988,.F.) ;
#46423=ORIENTED_EDGE('',*,*,#35989,.T.) ;
#46424=ORIENTED_EDGE('',*,*,#35990,.T.) ;
#46425=ORIENTED_EDGE('',*,*,#35991,.T.) ;
#46426=ORIENTED_EDGE('',*,*,#35992,.T.) ;
#46427=ORIENTED_EDGE('',*,*,#35789,.T.) ;
#46428=ORIENTED_EDGE('',*,*,#35993,.T.) ;
#46429=ORIENTED_EDGE('',*,*,#35994,.T.) ;
#46430=ORIENTED_EDGE('',*,*,#35995,.T.) ;
#46431=ORIENTED_EDGE('',*,*,#35996,.T.) ;
#46432=ORIENTED_EDGE('',*,*,#35791,.F.) ;
#46433=ORIENTED_EDGE('',*,*,#35997,.T.) ;
#46434=ORIENTED_EDGE('',*,*,#35998,.T.) ;
#46435=ORIENTED_EDGE('',*,*,#35999,.T.) ;
#46436=ORIENTED_EDGE('',*,*,#36000,.T.) ;
#46437=ORIENTED_EDGE('',*,*,#36001,.T.) ;
#46438=ORIENTED_EDGE('',*,*,#36002,.T.) ;
#46439=ORIENTED_EDGE('',*,*,#36003,.T.) ;
#46440=ORIENTED_EDGE('',*,*,#36004,.T.) ;
#46441=ORIENTED_EDGE('',*,*,#36005,.T.) ;
#46442=ORIENTED_EDGE('',*,*,#36006,.T.) ;
#46443=ORIENTED_EDGE('',*,*,#36007,.T.) ;
#46444=ORIENTED_EDGE('',*,*,#36008,.T.) ;
#46445=ORIENTED_EDGE('',*,*,#36009,.T.) ;
#46446=ORIENTED_EDGE('',*,*,#35831,.T.) ;
#46447=ORIENTED_EDGE('',*,*,#36010,.T.) ;
#46448=ORIENTED_EDGE('',*,*,#36011,.T.) ;
#46449=ORIENTED_EDGE('',*,*,#36012,.T.) ;
#46450=ORIENTED_EDGE('',*,*,#36013,.T.) ;
#46451=ORIENTED_EDGE('',*,*,#36014,.T.) ;
#46452=ORIENTED_EDGE('',*,*,#36015,.T.) ;
#46453=ORIENTED_EDGE('',*,*,#36016,.T.) ;
#46454=ORIENTED_EDGE('',*,*,#36017,.T.) ;
#46455=ORIENTED_EDGE('',*,*,#36018,.T.) ;
#46456=ORIENTED_EDGE('',*,*,#35833,.T.) ;
#46457=ORIENTED_EDGE('',*,*,#36019,.T.) ;
#46458=ORIENTED_EDGE('',*,*,#36020,.T.) ;
#46459=ORIENTED_EDGE('',*,*,#36021,.T.) ;
#46460=ORIENTED_EDGE('',*,*,#36022,.T.) ;
#46461=ORIENTED_EDGE('',*,*,#36023,.T.) ;
#46462=ORIENTED_EDGE('',*,*,#36024,.T.) ;
#46463=ORIENTED_EDGE('',*,*,#36025,.T.) ;
#46464=ORIENTED_EDGE('',*,*,#36026,.T.) ;
#46465=ORIENTED_EDGE('',*,*,#35718,.T.) ;
#46466=ORIENTED_EDGE('',*,*,#36027,.T.) ;
#46467=ORIENTED_EDGE('',*,*,#36028,.T.) ;
#46468=ORIENTED_EDGE('',*,*,#36029,.T.) ;
#46469=ORIENTED_EDGE('',*,*,#36030,.T.) ;
#46470=ORIENTED_EDGE('',*,*,#36031,.T.) ;
#46471=ORIENTED_EDGE('',*,*,#36032,.T.) ;
#46472=ORIENTED_EDGE('',*,*,#36033,.T.) ;
#46473=ORIENTED_EDGE('',*,*,#36034,.T.) ;
#46474=ORIENTED_EDGE('',*,*,#36035,.T.) ;
#46475=ORIENTED_EDGE('',*,*,#36036,.T.) ;
#46476=ORIENTED_EDGE('',*,*,#36037,.T.) ;
#46477=ORIENTED_EDGE('',*,*,#36038,.T.) ;
#46478=ORIENTED_EDGE('',*,*,#36039,.T.) ;
#46479=ORIENTED_EDGE('',*,*,#36040,.T.) ;
#46480=ORIENTED_EDGE('',*,*,#36041,.T.) ;
#46481=ORIENTED_EDGE('',*,*,#36042,.T.) ;
#46482=ORIENTED_EDGE('',*,*,#36043,.T.) ;
#46483=ORIENTED_EDGE('',*,*,#36044,.T.) ;
#46484=ORIENTED_EDGE('',*,*,#36045,.T.) ;
#46485=ORIENTED_EDGE('',*,*,#36046,.T.) ;
#46486=ORIENTED_EDGE('',*,*,#36047,.T.) ;
#46487=ORIENTED_EDGE('',*,*,#36048,.T.) ;
#46488=ORIENTED_EDGE('',*,*,#36049,.T.) ;
#46489=ORIENTED_EDGE('',*,*,#36050,.T.) ;
#46490=ORIENTED_EDGE('',*,*,#35951,.T.) ;
#46491=ORIENTED_EDGE('',*,*,#36051,.T.) ;
#46492=ORIENTED_EDGE('',*,*,#36052,.T.) ;
#46493=ORIENTED_EDGE('',*,*,#36053,.T.) ;
#46494=ORIENTED_EDGE('',*,*,#35955,.F.) ;
#46495=ORIENTED_EDGE('',*,*,#36054,.T.) ;
#46496=ORIENTED_EDGE('',*,*,#36055,.T.) ;
#46497=ORIENTED_EDGE('',*,*,#36056,.T.) ;
#46498=ORIENTED_EDGE('',*,*,#35957,.F.) ;
#46499=ORIENTED_EDGE('',*,*,#36057,.T.) ;
#46500=ORIENTED_EDGE('',*,*,#36058,.T.) ;
#46501=ORIENTED_EDGE('',*,*,#36059,.T.) ;
#46502=ORIENTED_EDGE('',*,*,#35953,.F.) ;
#46503=ORIENTED_EDGE('',*,*,#36060,.T.) ;
#46504=ORIENTED_EDGE('',*,*,#36061,.T.) ;
#46505=ORIENTED_EDGE('',*,*,#36062,.T.) ;
#46506=ORIENTED_EDGE('',*,*,#36063,.T.) ;
#46507=ORIENTED_EDGE('',*,*,#36064,.T.) ;
#46508=ORIENTED_EDGE('',*,*,#36065,.T.) ;
#46509=ORIENTED_EDGE('',*,*,#36066,.T.) ;
#46510=ORIENTED_EDGE('',*,*,#36067,.T.) ;
#46511=ORIENTED_EDGE('',*,*,#36068,.T.) ;
#46512=ORIENTED_EDGE('',*,*,#36069,.T.) ;
#46513=ORIENTED_EDGE('',*,*,#36070,.T.) ;
#46514=ORIENTED_EDGE('',*,*,#36071,.T.) ;
#46515=ORIENTED_EDGE('',*,*,#36072,.F.) ;
#46516=ORIENTED_EDGE('',*,*,#36073,.T.) ;
#46517=ORIENTED_EDGE('',*,*,#35749,.F.) ;
#46518=ORIENTED_EDGE('',*,*,#36074,.T.) ;
#46519=ORIENTED_EDGE('',*,*,#36075,.T.) ;
#46520=ORIENTED_EDGE('',*,*,#36076,.T.) ;
#46521=ORIENTED_EDGE('',*,*,#36077,.T.) ;
#46522=ORIENTED_EDGE('',*,*,#36072,.T.) ;
#46523=ORIENTED_EDGE('',*,*,#36078,.T.) ;
#46524=ORIENTED_EDGE('',*,*,#36079,.T.) ;
#46525=ORIENTED_EDGE('',*,*,#36080,.T.) ;
#46526=ORIENTED_EDGE('',*,*,#36081,.T.) ;
#46527=ORIENTED_EDGE('',*,*,#36082,.T.) ;
#46528=ORIENTED_EDGE('',*,*,#36083,.T.) ;
#46529=ORIENTED_EDGE('',*,*,#36084,.T.) ;
#46530=ORIENTED_EDGE('',*,*,#36085,.T.) ;
#46531=ORIENTED_EDGE('',*,*,#36086,.T.) ;
#46532=ORIENTED_EDGE('',*,*,#36087,.T.) ;
#46533=ORIENTED_EDGE('',*,*,#36088,.T.) ;
#46534=ORIENTED_EDGE('',*,*,#36089,.T.) ;
#46535=ORIENTED_EDGE('',*,*,#36090,.T.) ;
#46536=ORIENTED_EDGE('',*,*,#36091,.T.) ;
#46537=ORIENTED_EDGE('',*,*,#36092,.T.) ;
#46538=ORIENTED_EDGE('',*,*,#36093,.F.) ;
#46539=ORIENTED_EDGE('',*,*,#35942,.F.) ;
#46540=ORIENTED_EDGE('',*,*,#36094,.T.) ;
#46541=ORIENTED_EDGE('',*,*,#36093,.T.) ;
#46542=ORIENTED_EDGE('',*,*,#36095,.T.) ;
#46543=ORIENTED_EDGE('',*,*,#36096,.T.) ;
#46544=ORIENTED_EDGE('',*,*,#36097,.T.) ;
#46545=ORIENTED_EDGE('',*,*,#36098,.T.) ;
#46546=ORIENTED_EDGE('',*,*,#36099,.T.) ;
#46547=ORIENTED_EDGE('',*,*,#36100,.T.) ;
#46548=ORIENTED_EDGE('',*,*,#36101,.T.) ;
#46549=ORIENTED_EDGE('',*,*,#36102,.T.) ;
#46550=ORIENTED_EDGE('',*,*,#36103,.T.) ;
#46551=ORIENTED_EDGE('',*,*,#36104,.T.) ;
#46552=ORIENTED_EDGE('',*,*,#36105,.T.) ;
#46553=ORIENTED_EDGE('',*,*,#36106,.T.) ;
#46554=ORIENTED_EDGE('',*,*,#36107,.T.) ;
#46555=ORIENTED_EDGE('',*,*,#36108,.T.) ;
#46556=ORIENTED_EDGE('',*,*,#36109,.T.) ;
#46557=ORIENTED_EDGE('',*,*,#36110,.T.) ;
#46558=ORIENTED_EDGE('',*,*,#36111,.T.) ;
#46559=ORIENTED_EDGE('',*,*,#36112,.T.) ;
#46560=ORIENTED_EDGE('',*,*,#36113,.T.) ;
#46561=ORIENTED_EDGE('',*,*,#36114,.T.) ;
#46562=ORIENTED_EDGE('',*,*,#35822,.F.) ;
#46563=ORIENTED_EDGE('',*,*,#36115,.T.) ;
#46564=ORIENTED_EDGE('',*,*,#36116,.T.) ;
#46565=ORIENTED_EDGE('',*,*,#35736,.T.) ;
#46566=ORIENTED_EDGE('',*,*,#36117,.T.) ;
#46567=ORIENTED_EDGE('',*,*,#35800,.F.) ;
#46568=ORIENTED_EDGE('',*,*,#36118,.T.) ;
#46569=ORIENTED_EDGE('',*,*,#36119,.T.) ;
#46570=ORIENTED_EDGE('',*,*,#36120,.T.) ;
#46571=ORIENTED_EDGE('',*,*,#36121,.F.) ;
#46572=ORIENTED_EDGE('',*,*,#36019,.F.) ;
#46573=ORIENTED_EDGE('',*,*,#35832,.F.) ;
#46574=ORIENTED_EDGE('',*,*,#36012,.F.) ;
#46575=ORIENTED_EDGE('',*,*,#36122,.F.) ;
#46576=ORIENTED_EDGE('',*,*,#36121,.T.) ;
#46577=ORIENTED_EDGE('',*,*,#36123,.F.) ;
#46578=ORIENTED_EDGE('',*,*,#35830,.F.) ;
#46579=ORIENTED_EDGE('',*,*,#35887,.F.) ;
#46580=ORIENTED_EDGE('',*,*,#36124,.F.) ;
#46581=ORIENTED_EDGE('',*,*,#36010,.F.) ;
#46582=ORIENTED_EDGE('',*,*,#36123,.T.) ;
#46583=ORIENTED_EDGE('',*,*,#36011,.F.) ;
#46584=ORIENTED_EDGE('',*,*,#36125,.F.) ;
#46585=ORIENTED_EDGE('',*,*,#36007,.F.) ;
#46586=ORIENTED_EDGE('',*,*,#36122,.T.) ;
#46587=ORIENTED_EDGE('',*,*,#36006,.F.) ;
#46588=ORIENTED_EDGE('',*,*,#36126,.F.) ;
#46589=ORIENTED_EDGE('',*,*,#36020,.F.) ;
#46590=ORIENTED_EDGE('',*,*,#36124,.T.) ;
#46591=ORIENTED_EDGE('',*,*,#35886,.T.) ;
#46592=ORIENTED_EDGE('',*,*,#36127,.F.) ;
#46593=ORIENTED_EDGE('',*,*,#36125,.T.) ;
#46594=ORIENTED_EDGE('',*,*,#36128,.F.) ;
#46595=ORIENTED_EDGE('',*,*,#36126,.T.) ;
#46596=ORIENTED_EDGE('',*,*,#36129,.F.) ;
#46597=ORIENTED_EDGE('',*,*,#35790,.F.) ;
#46598=ORIENTED_EDGE('',*,*,#35992,.F.) ;
#46599=ORIENTED_EDGE('',*,*,#36130,.F.) ;
#46600=ORIENTED_EDGE('',*,*,#35997,.F.) ;
#46601=ORIENTED_EDGE('',*,*,#36131,.F.) ;
#46602=ORIENTED_EDGE('',*,*,#35995,.F.) ;
#46603=ORIENTED_EDGE('',*,*,#36132,.F.) ;
#46604=ORIENTED_EDGE('',*,*,#36001,.F.) ;
#46605=ORIENTED_EDGE('',*,*,#35792,.F.) ;
#46606=ORIENTED_EDGE('',*,*,#35996,.F.) ;
#46607=ORIENTED_EDGE('',*,*,#36133,.F.) ;
#46608=ORIENTED_EDGE('',*,*,#35877,.F.) ;
#46609=ORIENTED_EDGE('',*,*,#36127,.T.) ;
#46610=ORIENTED_EDGE('',*,*,#35885,.F.) ;
#46611=ORIENTED_EDGE('',*,*,#36134,.F.) ;
#46612=ORIENTED_EDGE('',*,*,#36008,.F.) ;
#46613=ORIENTED_EDGE('',*,*,#36129,.T.) ;
#46614=ORIENTED_EDGE('',*,*,#36009,.F.) ;
#46615=ORIENTED_EDGE('',*,*,#36135,.F.) ;
#46616=ORIENTED_EDGE('',*,*,#36016,.F.) ;
#46617=ORIENTED_EDGE('',*,*,#36128,.T.) ;
#46618=ORIENTED_EDGE('',*,*,#36015,.F.) ;
#46619=ORIENTED_EDGE('',*,*,#36136,.F.) ;
#46620=ORIENTED_EDGE('',*,*,#36017,.F.) ;
#46621=ORIENTED_EDGE('',*,*,#35834,.F.) ;
#46622=ORIENTED_EDGE('',*,*,#36018,.F.) ;
#46623=ORIENTED_EDGE('',*,*,#36137,.F.) ;
#46624=ORIENTED_EDGE('',*,*,#35868,.F.) ;
#46625=ORIENTED_EDGE('',*,*,#36132,.T.) ;
#46626=ORIENTED_EDGE('',*,*,#36130,.T.) ;
#46627=ORIENTED_EDGE('',*,*,#36138,.F.) ;
#46628=ORIENTED_EDGE('',*,*,#36133,.T.) ;
#46629=ORIENTED_EDGE('',*,*,#36131,.T.) ;
#46630=ORIENTED_EDGE('',*,*,#36139,.F.) ;
#46631=ORIENTED_EDGE('',*,*,#35878,.T.) ;
#46632=ORIENTED_EDGE('',*,*,#36134,.T.) ;
#46633=ORIENTED_EDGE('',*,*,#35884,.T.) ;
#46634=ORIENTED_EDGE('',*,*,#36140,.F.) ;
#46635=ORIENTED_EDGE('',*,*,#36135,.T.) ;
#46636=ORIENTED_EDGE('',*,*,#36137,.T.) ;
#46637=ORIENTED_EDGE('',*,*,#36136,.T.) ;
#46638=ORIENTED_EDGE('',*,*,#36141,.F.) ;
#46639=ORIENTED_EDGE('',*,*,#36138,.T.) ;
#46640=ORIENTED_EDGE('',*,*,#35991,.F.) ;
#46641=ORIENTED_EDGE('',*,*,#36142,.F.) ;
#46642=ORIENTED_EDGE('',*,*,#35998,.F.) ;
#46643=ORIENTED_EDGE('',*,*,#36143,.F.) ;
#46644=ORIENTED_EDGE('',*,*,#35999,.F.) ;
#46645=ORIENTED_EDGE('',*,*,#36144,.F.) ;
#46646=ORIENTED_EDGE('',*,*,#36005,.F.) ;
#46647=ORIENTED_EDGE('',*,*,#36139,.T.) ;
#46648=ORIENTED_EDGE('',*,*,#36000,.F.) ;
#46649=ORIENTED_EDGE('',*,*,#36145,.F.) ;
#46650=ORIENTED_EDGE('',*,*,#35879,.F.) ;
#46651=ORIENTED_EDGE('',*,*,#36140,.T.) ;
#46652=ORIENTED_EDGE('',*,*,#35883,.F.) ;
#46653=ORIENTED_EDGE('',*,*,#36146,.F.) ;
#46654=ORIENTED_EDGE('',*,*,#36013,.F.) ;
#46655=ORIENTED_EDGE('',*,*,#36141,.T.) ;
#46656=ORIENTED_EDGE('',*,*,#36014,.F.) ;
#46657=ORIENTED_EDGE('',*,*,#36147,.F.) ;
#46658=ORIENTED_EDGE('',*,*,#35869,.F.) ;
#46659=ORIENTED_EDGE('',*,*,#36144,.T.) ;
#46660=ORIENTED_EDGE('',*,*,#36142,.T.) ;
#46661=ORIENTED_EDGE('',*,*,#36148,.F.) ;
#46662=ORIENTED_EDGE('',*,*,#36145,.T.) ;
#46663=ORIENTED_EDGE('',*,*,#36143,.T.) ;
#46664=ORIENTED_EDGE('',*,*,#36149,.F.) ;
#46665=ORIENTED_EDGE('',*,*,#35880,.T.) ;
#46666=ORIENTED_EDGE('',*,*,#36147,.T.) ;
#46667=ORIENTED_EDGE('',*,*,#36146,.T.) ;
#46668=ORIENTED_EDGE('',*,*,#36150,.F.) ;
#46669=ORIENTED_EDGE('',*,*,#35870,.T.) ;
#46670=ORIENTED_EDGE('',*,*,#35788,.F.) ;
#46671=ORIENTED_EDGE('',*,*,#35874,.F.) ;
#46672=ORIENTED_EDGE('',*,*,#36151,.F.) ;
#46673=ORIENTED_EDGE('',*,*,#35993,.F.) ;
#46674=ORIENTED_EDGE('',*,*,#36148,.T.) ;
#46675=ORIENTED_EDGE('',*,*,#35994,.F.) ;
#46676=ORIENTED_EDGE('',*,*,#36152,.F.) ;
#46677=ORIENTED_EDGE('',*,*,#36002,.F.) ;
#46678=ORIENTED_EDGE('',*,*,#36149,.T.) ;
#46679=ORIENTED_EDGE('',*,*,#36004,.F.) ;
#46680=ORIENTED_EDGE('',*,*,#36153,.F.) ;
#46681=ORIENTED_EDGE('',*,*,#35881,.F.) ;
#46682=ORIENTED_EDGE('',*,*,#36150,.T.) ;
#46683=ORIENTED_EDGE('',*,*,#35882,.F.) ;
#46684=ORIENTED_EDGE('',*,*,#36154,.F.) ;
#46685=ORIENTED_EDGE('',*,*,#35871,.F.) ;
#46686=ORIENTED_EDGE('',*,*,#36152,.T.) ;
#46687=ORIENTED_EDGE('',*,*,#36151,.T.) ;
#46688=ORIENTED_EDGE('',*,*,#36155,.F.) ;
#46689=ORIENTED_EDGE('',*,*,#36154,.T.) ;
#46690=ORIENTED_EDGE('',*,*,#36153,.T.) ;
#46691=ORIENTED_EDGE('',*,*,#36156,.F.) ;
#46692=ORIENTED_EDGE('',*,*,#35872,.T.) ;
#46693=ORIENTED_EDGE('',*,*,#36155,.T.) ;
#46694=ORIENTED_EDGE('',*,*,#35873,.F.) ;
#46695=ORIENTED_EDGE('',*,*,#36156,.T.) ;
#46696=ORIENTED_EDGE('',*,*,#36003,.F.) ;
#46697=ORIENTED_EDGE('',*,*,#36157,.F.) ;
#46698=ORIENTED_EDGE('',*,*,#36158,.F.) ;
#46699=ORIENTED_EDGE('',*,*,#36159,.F.) ;
#46700=ORIENTED_EDGE('',*,*,#35950,.F.) ;
#46701=ORIENTED_EDGE('',*,*,#36160,.T.) ;
#46702=ORIENTED_EDGE('',*,*,#36161,.T.) ;
#46703=ORIENTED_EDGE('',*,*,#35932,.F.) ;
#46704=ORIENTED_EDGE('',*,*,#36158,.T.) ;
#46705=ORIENTED_EDGE('',*,*,#35931,.F.) ;
#46706=ORIENTED_EDGE('',*,*,#36162,.T.) ;
#46707=ORIENTED_EDGE('',*,*,#36163,.T.) ;
#46708=ORIENTED_EDGE('',*,*,#35924,.F.) ;
#46709=ORIENTED_EDGE('',*,*,#36159,.T.) ;
#46710=ORIENTED_EDGE('',*,*,#36157,.T.) ;
#46711=ORIENTED_EDGE('',*,*,#35923,.F.) ;
#46712=ORIENTED_EDGE('',*,*,#36164,.F.) ;
#46713=ORIENTED_EDGE('',*,*,#35943,.F.) ;
#46714=ORIENTED_EDGE('',*,*,#35939,.F.) ;
#46715=ORIENTED_EDGE('',*,*,#36165,.T.) ;
#46716=ORIENTED_EDGE('',*,*,#36166,.T.) ;
#46717=ORIENTED_EDGE('',*,*,#35949,.F.) ;
#46718=ORIENTED_EDGE('',*,*,#36167,.T.) ;
#46719=ORIENTED_EDGE('',*,*,#36168,.T.) ;
#46720=ORIENTED_EDGE('',*,*,#35917,.F.) ;
#46721=ORIENTED_EDGE('',*,*,#36169,.T.) ;
#46722=ORIENTED_EDGE('',*,*,#36170,.T.) ;
#46723=ORIENTED_EDGE('',*,*,#35933,.F.) ;
#46724=ORIENTED_EDGE('',*,*,#36171,.T.) ;
#46725=ORIENTED_EDGE('',*,*,#36172,.T.) ;
#46726=ORIENTED_EDGE('',*,*,#36173,.F.) ;
#46727=ORIENTED_EDGE('',*,*,#36164,.T.) ;
#46728=ORIENTED_EDGE('',*,*,#36174,.F.) ;
#46729=ORIENTED_EDGE('',*,*,#35914,.T.) ;
#46730=ORIENTED_EDGE('',*,*,#36175,.F.) ;
#46731=ORIENTED_EDGE('',*,*,#36176,.F.) ;
#46732=ORIENTED_EDGE('',*,*,#35944,.F.) ;
#46733=ORIENTED_EDGE('',*,*,#36173,.T.) ;
#46734=ORIENTED_EDGE('',*,*,#36176,.T.) ;
#46735=ORIENTED_EDGE('',*,*,#36177,.F.) ;
#46736=ORIENTED_EDGE('',*,*,#36178,.F.) ;
#46737=ORIENTED_EDGE('',*,*,#35928,.F.) ;
#46738=ORIENTED_EDGE('',*,*,#36179,.T.) ;
#46739=ORIENTED_EDGE('',*,*,#36180,.T.) ;
#46740=ORIENTED_EDGE('',*,*,#35948,.F.) ;
#46741=ORIENTED_EDGE('',*,*,#36181,.F.) ;
#46742=ORIENTED_EDGE('',*,*,#35918,.F.) ;
#46743=ORIENTED_EDGE('',*,*,#36182,.T.) ;
#46744=ORIENTED_EDGE('',*,*,#36183,.T.) ;
#46745=ORIENTED_EDGE('',*,*,#35925,.F.) ;
#46746=ORIENTED_EDGE('',*,*,#36184,.F.) ;
#46747=ORIENTED_EDGE('',*,*,#36174,.T.) ;
#46748=ORIENTED_EDGE('',*,*,#35922,.F.) ;
#46749=ORIENTED_EDGE('',*,*,#36185,.F.) ;
#46750=ORIENTED_EDGE('',*,*,#36186,.F.) ;
#46751=ORIENTED_EDGE('',*,*,#36187,.F.) ;
#46752=ORIENTED_EDGE('',*,*,#35898,.F.) ;
#46753=ORIENTED_EDGE('',*,*,#36188,.F.) ;
#46754=ORIENTED_EDGE('',*,*,#36175,.T.) ;
#46755=ORIENTED_EDGE('',*,*,#35916,.F.) ;
#46756=ORIENTED_EDGE('',*,*,#36188,.T.) ;
#46757=ORIENTED_EDGE('',*,*,#35897,.T.) ;
#46758=ORIENTED_EDGE('',*,*,#36189,.F.) ;
#46759=ORIENTED_EDGE('',*,*,#36177,.T.) ;
#46760=ORIENTED_EDGE('',*,*,#35945,.F.) ;
#46761=ORIENTED_EDGE('',*,*,#36178,.T.) ;
#46762=ORIENTED_EDGE('',*,*,#36190,.F.) ;
#46763=ORIENTED_EDGE('',*,*,#36191,.F.) ;
#46764=ORIENTED_EDGE('',*,*,#36184,.T.) ;
#46765=ORIENTED_EDGE('',*,*,#36181,.T.) ;
#46766=ORIENTED_EDGE('',*,*,#36192,.F.) ;
#46767=ORIENTED_EDGE('',*,*,#36193,.F.) ;
#46768=ORIENTED_EDGE('',*,*,#36185,.T.) ;
#46769=ORIENTED_EDGE('',*,*,#36194,.F.) ;
#46770=ORIENTED_EDGE('',*,*,#35915,.F.) ;
#46771=ORIENTED_EDGE('',*,*,#36186,.T.) ;
#46772=ORIENTED_EDGE('',*,*,#36195,.F.) ;
#46773=ORIENTED_EDGE('',*,*,#35908,.F.) ;
#46774=ORIENTED_EDGE('',*,*,#36187,.T.) ;
#46775=ORIENTED_EDGE('',*,*,#36196,.F.) ;
#46776=ORIENTED_EDGE('',*,*,#36190,.T.) ;
#46777=ORIENTED_EDGE('',*,*,#36189,.T.) ;
#46778=ORIENTED_EDGE('',*,*,#35904,.F.) ;
#46779=ORIENTED_EDGE('',*,*,#36191,.T.) ;
#46780=ORIENTED_EDGE('',*,*,#36197,.F.) ;
#46781=ORIENTED_EDGE('',*,*,#36198,.F.) ;
#46782=ORIENTED_EDGE('',*,*,#36192,.T.) ;
#46783=ORIENTED_EDGE('',*,*,#35947,.F.) ;
#46784=ORIENTED_EDGE('',*,*,#36199,.F.) ;
#46785=ORIENTED_EDGE('',*,*,#35919,.F.) ;
#46786=ORIENTED_EDGE('',*,*,#36194,.T.) ;
#46787=ORIENTED_EDGE('',*,*,#35921,.F.) ;
#46788=ORIENTED_EDGE('',*,*,#36200,.F.) ;
#46789=ORIENTED_EDGE('',*,*,#36201,.F.) ;
#46790=ORIENTED_EDGE('',*,*,#36195,.T.) ;
#46791=ORIENTED_EDGE('',*,*,#36193,.T.) ;
#46792=ORIENTED_EDGE('',*,*,#36202,.F.) ;
#46793=ORIENTED_EDGE('',*,*,#35909,.T.) ;
#46794=ORIENTED_EDGE('',*,*,#36196,.T.) ;
#46795=ORIENTED_EDGE('',*,*,#35903,.T.) ;
#46796=ORIENTED_EDGE('',*,*,#36203,.F.) ;
#46797=ORIENTED_EDGE('',*,*,#36197,.T.) ;
#46798=ORIENTED_EDGE('',*,*,#36204,.F.) ;
#46799=ORIENTED_EDGE('',*,*,#36205,.F.) ;
#46800=ORIENTED_EDGE('',*,*,#35946,.F.) ;
#46801=ORIENTED_EDGE('',*,*,#36198,.T.) ;
#46802=ORIENTED_EDGE('',*,*,#36205,.T.) ;
#46803=ORIENTED_EDGE('',*,*,#35913,.T.) ;
#46804=ORIENTED_EDGE('',*,*,#36206,.F.) ;
#46805=ORIENTED_EDGE('',*,*,#36199,.T.) ;
#46806=ORIENTED_EDGE('',*,*,#36207,.F.) ;
#46807=ORIENTED_EDGE('',*,*,#36200,.T.) ;
#46808=ORIENTED_EDGE('',*,*,#36208,.F.) ;
#46809=ORIENTED_EDGE('',*,*,#36202,.T.) ;
#46810=ORIENTED_EDGE('',*,*,#36201,.T.) ;
#46811=ORIENTED_EDGE('',*,*,#36209,.F.) ;
#46812=ORIENTED_EDGE('',*,*,#35910,.F.) ;
#46813=ORIENTED_EDGE('',*,*,#36203,.T.) ;
#46814=ORIENTED_EDGE('',*,*,#35902,.F.) ;
#46815=ORIENTED_EDGE('',*,*,#36210,.F.) ;
#46816=ORIENTED_EDGE('',*,*,#35911,.F.) ;
#46817=ORIENTED_EDGE('',*,*,#36204,.T.) ;
#46818=ORIENTED_EDGE('',*,*,#35920,.F.) ;
#46819=ORIENTED_EDGE('',*,*,#36206,.T.) ;
#46820=ORIENTED_EDGE('',*,*,#36211,.F.) ;
#46821=ORIENTED_EDGE('',*,*,#36208,.T.) ;
#46822=ORIENTED_EDGE('',*,*,#36209,.T.) ;
#46823=ORIENTED_EDGE('',*,*,#36207,.T.) ;
#46824=ORIENTED_EDGE('',*,*,#36212,.F.) ;
#46825=ORIENTED_EDGE('',*,*,#35905,.T.) ;
#46826=ORIENTED_EDGE('',*,*,#36210,.T.) ;
#46827=ORIENTED_EDGE('',*,*,#35906,.F.) ;
#46828=ORIENTED_EDGE('',*,*,#36212,.T.) ;
#46829=ORIENTED_EDGE('',*,*,#36211,.T.) ;
#46830=ORIENTED_EDGE('',*,*,#35912,.F.) ;
#46831=ORIENTED_EDGE('',*,*,#36213,.F.) ;
#46832=ORIENTED_EDGE('',*,*,#35961,.F.) ;
#46833=ORIENTED_EDGE('',*,*,#35796,.F.) ;
#46834=ORIENTED_EDGE('',*,*,#35967,.F.) ;
#46835=ORIENTED_EDGE('',*,*,#36214,.F.) ;
#46836=ORIENTED_EDGE('',*,*,#36213,.T.) ;
#46837=ORIENTED_EDGE('',*,*,#36215,.F.) ;
#46838=ORIENTED_EDGE('',*,*,#35794,.F.) ;
#46839=ORIENTED_EDGE('',*,*,#35876,.F.) ;
#46840=ORIENTED_EDGE('',*,*,#36216,.F.) ;
#46841=ORIENTED_EDGE('',*,*,#35965,.F.) ;
#46842=ORIENTED_EDGE('',*,*,#36215,.T.) ;
#46843=ORIENTED_EDGE('',*,*,#35966,.F.) ;
#46844=ORIENTED_EDGE('',*,*,#36217,.F.) ;
#46845=ORIENTED_EDGE('',*,*,#35972,.F.) ;
#46846=ORIENTED_EDGE('',*,*,#36214,.T.) ;
#46847=ORIENTED_EDGE('',*,*,#35971,.F.) ;
#46848=ORIENTED_EDGE('',*,*,#36218,.F.) ;
#46849=ORIENTED_EDGE('',*,*,#35962,.F.) ;
#46850=ORIENTED_EDGE('',*,*,#35798,.F.) ;
#46851=ORIENTED_EDGE('',*,*,#35960,.F.) ;
#46852=ORIENTED_EDGE('',*,*,#36219,.F.) ;
#46853=ORIENTED_EDGE('',*,*,#35771,.F.) ;
#46854=ORIENTED_EDGE('',*,*,#35739,.F.) ;
#46855=ORIENTED_EDGE('',*,*,#36220,.T.) ;
#46856=ORIENTED_EDGE('',*,*,#35768,.F.) ;
#46857=ORIENTED_EDGE('',*,*,#36221,.F.) ;
#46858=ORIENTED_EDGE('',*,*,#36216,.T.) ;
#46859=ORIENTED_EDGE('',*,*,#35875,.T.) ;
#46860=ORIENTED_EDGE('',*,*,#36222,.F.) ;
#46861=ORIENTED_EDGE('',*,*,#36217,.T.) ;
#46862=ORIENTED_EDGE('',*,*,#36223,.F.) ;
#46863=ORIENTED_EDGE('',*,*,#36218,.T.) ;
#46864=ORIENTED_EDGE('',*,*,#36224,.F.) ;
#46865=ORIENTED_EDGE('',*,*,#36219,.T.) ;
#46866=ORIENTED_EDGE('',*,*,#35959,.T.) ;
#46867=ORIENTED_EDGE('',*,*,#36225,.F.) ;
#46868=ORIENTED_EDGE('',*,*,#36221,.T.) ;
#46869=ORIENTED_EDGE('',*,*,#36222,.T.) ;
#46870=ORIENTED_EDGE('',*,*,#35896,.F.) ;
#46871=ORIENTED_EDGE('',*,*,#36226,.F.) ;
#46872=ORIENTED_EDGE('',*,*,#35973,.F.) ;
#46873=ORIENTED_EDGE('',*,*,#36224,.T.) ;
#46874=ORIENTED_EDGE('',*,*,#35974,.F.) ;
#46875=ORIENTED_EDGE('',*,*,#36227,.F.) ;
#46876=ORIENTED_EDGE('',*,*,#35968,.F.) ;
#46877=ORIENTED_EDGE('',*,*,#36223,.T.) ;
#46878=ORIENTED_EDGE('',*,*,#35970,.F.) ;
#46879=ORIENTED_EDGE('',*,*,#36228,.F.) ;
#46880=ORIENTED_EDGE('',*,*,#35963,.F.) ;
#46881=ORIENTED_EDGE('',*,*,#36225,.T.) ;
#46882=ORIENTED_EDGE('',*,*,#35964,.F.) ;
#46883=ORIENTED_EDGE('',*,*,#36229,.F.) ;
#46884=ORIENTED_EDGE('',*,*,#35740,.F.) ;
#46885=ORIENTED_EDGE('',*,*,#35774,.F.) ;
#46886=ORIENTED_EDGE('',*,*,#36230,.T.) ;
#46887=ORIENTED_EDGE('',*,*,#35745,.F.) ;
#46888=ORIENTED_EDGE('',*,*,#36231,.F.) ;
#46889=ORIENTED_EDGE('',*,*,#35824,.F.) ;
#46890=ORIENTED_EDGE('',*,*,#35775,.F.) ;
#46891=ORIENTED_EDGE('',*,*,#36232,.F.) ;
#46892=ORIENTED_EDGE('',*,*,#35987,.F.) ;
#46893=ORIENTED_EDGE('',*,*,#35826,.F.) ;
#46894=ORIENTED_EDGE('',*,*,#35986,.F.) ;
#46895=ORIENTED_EDGE('',*,*,#36233,.F.) ;
#46896=ORIENTED_EDGE('',*,*,#35984,.F.) ;
#46897=ORIENTED_EDGE('',*,*,#36226,.T.) ;
#46898=ORIENTED_EDGE('',*,*,#35895,.T.) ;
#46899=ORIENTED_EDGE('',*,*,#36234,.F.) ;
#46900=ORIENTED_EDGE('',*,*,#36227,.T.) ;
#46901=ORIENTED_EDGE('',*,*,#36229,.T.) ;
#46902=ORIENTED_EDGE('',*,*,#36228,.T.) ;
#46903=ORIENTED_EDGE('',*,*,#35732,.F.) ;
#46904=ORIENTED_EDGE('',*,*,#36232,.T.) ;
#46905=ORIENTED_EDGE('',*,*,#36231,.T.) ;
#46906=ORIENTED_EDGE('',*,*,#36235,.F.) ;
#46907=ORIENTED_EDGE('',*,*,#35988,.T.) ;
#46908=ORIENTED_EDGE('',*,*,#36236,.F.) ;
#46909=ORIENTED_EDGE('',*,*,#36233,.T.) ;
#46910=ORIENTED_EDGE('',*,*,#36237,.F.) ;
#46911=ORIENTED_EDGE('',*,*,#36234,.T.) ;
#46912=ORIENTED_EDGE('',*,*,#35894,.F.) ;
#46913=ORIENTED_EDGE('',*,*,#36238,.F.) ;
#46914=ORIENTED_EDGE('',*,*,#35969,.F.) ;
#46915=ORIENTED_EDGE('',*,*,#36235,.T.) ;
#46916=ORIENTED_EDGE('',*,*,#35744,.F.) ;
#46917=ORIENTED_EDGE('',*,*,#36239,.F.) ;
#46918=ORIENTED_EDGE('',*,*,#35989,.F.) ;
#46919=ORIENTED_EDGE('',*,*,#36240,.F.) ;
#46920=ORIENTED_EDGE('',*,*,#35990,.F.) ;
#46921=ORIENTED_EDGE('',*,*,#36241,.F.) ;
#46922=ORIENTED_EDGE('',*,*,#35981,.F.) ;
#46923=ORIENTED_EDGE('',*,*,#36237,.T.) ;
#46924=ORIENTED_EDGE('',*,*,#35985,.F.) ;
#46925=ORIENTED_EDGE('',*,*,#36242,.F.) ;
#46926=ORIENTED_EDGE('',*,*,#35975,.F.) ;
#46927=ORIENTED_EDGE('',*,*,#36236,.T.) ;
#46928=ORIENTED_EDGE('',*,*,#35978,.F.) ;
#46929=ORIENTED_EDGE('',*,*,#36243,.F.) ;
#46930=ORIENTED_EDGE('',*,*,#35982,.F.) ;
#46931=ORIENTED_EDGE('',*,*,#35828,.F.) ;
#46932=ORIENTED_EDGE('',*,*,#35983,.F.) ;
#46933=ORIENTED_EDGE('',*,*,#36244,.F.) ;
#46934=ORIENTED_EDGE('',*,*,#35888,.F.) ;
#46935=ORIENTED_EDGE('',*,*,#35730,.T.) ;
#46936=ORIENTED_EDGE('',*,*,#36238,.T.) ;
#46937=ORIENTED_EDGE('',*,*,#36245,.F.) ;
#46938=ORIENTED_EDGE('',*,*,#35741,.T.) ;
#46939=ORIENTED_EDGE('',*,*,#36241,.T.) ;
#46940=ORIENTED_EDGE('',*,*,#36239,.T.) ;
#46941=ORIENTED_EDGE('',*,*,#35728,.F.) ;
#46942=ORIENTED_EDGE('',*,*,#36246,.F.) ;
#46943=ORIENTED_EDGE('',*,*,#36246,.T.) ;
#46944=ORIENTED_EDGE('',*,*,#35727,.F.) ;
#46945=ORIENTED_EDGE('',*,*,#36242,.T.) ;
#46946=ORIENTED_EDGE('',*,*,#36240,.T.) ;
#46947=ORIENTED_EDGE('',*,*,#36247,.F.) ;
#46948=ORIENTED_EDGE('',*,*,#36244,.T.) ;
#46949=ORIENTED_EDGE('',*,*,#36243,.T.) ;
#46950=ORIENTED_EDGE('',*,*,#36248,.F.) ;
#46951=ORIENTED_EDGE('',*,*,#35889,.T.) ;
#46952=ORIENTED_EDGE('',*,*,#36245,.T.) ;
#46953=ORIENTED_EDGE('',*,*,#35893,.F.) ;
#46954=ORIENTED_EDGE('',*,*,#36249,.F.) ;
#46955=ORIENTED_EDGE('',*,*,#35742,.F.) ;
#46956=ORIENTED_EDGE('',*,*,#36247,.T.) ;
#46957=ORIENTED_EDGE('',*,*,#35980,.F.) ;
#46958=ORIENTED_EDGE('',*,*,#36250,.F.) ;
#46959=ORIENTED_EDGE('',*,*,#35976,.F.) ;
#46960=ORIENTED_EDGE('',*,*,#36248,.T.) ;
#46961=ORIENTED_EDGE('',*,*,#35977,.F.) ;
#46962=ORIENTED_EDGE('',*,*,#36251,.F.) ;
#46963=ORIENTED_EDGE('',*,*,#35890,.F.) ;
#46964=ORIENTED_EDGE('',*,*,#35743,.T.) ;
#46965=ORIENTED_EDGE('',*,*,#36249,.T.) ;
#46966=ORIENTED_EDGE('',*,*,#36252,.F.) ;
#46967=ORIENTED_EDGE('',*,*,#35725,.T.) ;
#46968=ORIENTED_EDGE('',*,*,#36251,.T.) ;
#46969=ORIENTED_EDGE('',*,*,#36250,.T.) ;
#46970=ORIENTED_EDGE('',*,*,#36253,.F.) ;
#46971=ORIENTED_EDGE('',*,*,#35891,.T.) ;
#46972=ORIENTED_EDGE('',*,*,#36252,.T.) ;
#46973=ORIENTED_EDGE('',*,*,#35892,.F.) ;
#46974=ORIENTED_EDGE('',*,*,#36253,.T.) ;
#46975=ORIENTED_EDGE('',*,*,#35979,.F.) ;
#46976=ORIENTED_EDGE('',*,*,#35748,.F.) ;
#46977=ORIENTED_EDGE('',*,*,#36254,.T.) ;
#46978=ORIENTED_EDGE('',*,*,#36069,.F.) ;
#46979=ORIENTED_EDGE('',*,*,#36255,.F.) ;
#46980=ORIENTED_EDGE('',*,*,#36074,.F.) ;
#46981=ORIENTED_EDGE('',*,*,#36068,.F.) ;
#46982=ORIENTED_EDGE('',*,*,#36256,.T.) ;
#46983=ORIENTED_EDGE('',*,*,#36075,.F.) ;
#46984=ORIENTED_EDGE('',*,*,#36255,.T.) ;
#46985=ORIENTED_EDGE('',*,*,#36071,.F.) ;
#46986=ORIENTED_EDGE('',*,*,#36257,.T.) ;
#46987=ORIENTED_EDGE('',*,*,#35937,.F.) ;
#46988=ORIENTED_EDGE('',*,*,#36095,.F.) ;
#46989=ORIENTED_EDGE('',*,*,#36258,.F.) ;
#46990=ORIENTED_EDGE('',*,*,#36080,.F.) ;
#46991=ORIENTED_EDGE('',*,*,#36259,.T.) ;
#46992=ORIENTED_EDGE('',*,*,#36108,.F.) ;
#46993=ORIENTED_EDGE('',*,*,#36260,.F.) ;
#46994=ORIENTED_EDGE('',*,*,#36065,.F.) ;
#46995=ORIENTED_EDGE('',*,*,#36261,.T.) ;
#46996=ORIENTED_EDGE('',*,*,#35750,.F.) ;
#46997=ORIENTED_EDGE('',*,*,#36073,.F.) ;
#46998=ORIENTED_EDGE('',*,*,#36262,.F.) ;
#46999=ORIENTED_EDGE('',*,*,#36092,.F.) ;
#47000=ORIENTED_EDGE('',*,*,#36263,.T.) ;
#47001=ORIENTED_EDGE('',*,*,#36066,.F.) ;
#47002=ORIENTED_EDGE('',*,*,#36258,.T.) ;
#47003=ORIENTED_EDGE('',*,*,#36264,.F.) ;
#47004=ORIENTED_EDGE('',*,*,#36260,.T.) ;
#47005=ORIENTED_EDGE('',*,*,#36265,.F.) ;
#47006=ORIENTED_EDGE('',*,*,#36077,.F.) ;
#47007=ORIENTED_EDGE('',*,*,#36266,.T.) ;
#47008=ORIENTED_EDGE('',*,*,#36060,.F.) ;
#47009=ORIENTED_EDGE('',*,*,#36262,.T.) ;
#47010=ORIENTED_EDGE('',*,*,#36110,.F.) ;
#47011=ORIENTED_EDGE('',*,*,#36267,.T.) ;
#47012=ORIENTED_EDGE('',*,*,#36086,.F.) ;
#47013=ORIENTED_EDGE('',*,*,#36268,.F.) ;
#47014=ORIENTED_EDGE('',*,*,#36265,.T.) ;
#47015=ORIENTED_EDGE('',*,*,#36111,.F.) ;
#47016=ORIENTED_EDGE('',*,*,#36269,.F.) ;
#47017=ORIENTED_EDGE('',*,*,#36085,.F.) ;
#47018=ORIENTED_EDGE('',*,*,#36264,.T.) ;
#47019=ORIENTED_EDGE('',*,*,#36084,.F.) ;
#47020=ORIENTED_EDGE('',*,*,#36270,.F.) ;
#47021=ORIENTED_EDGE('',*,*,#36081,.F.) ;
#47022=ORIENTED_EDGE('',*,*,#36106,.F.) ;
#47023=ORIENTED_EDGE('',*,*,#36271,.T.) ;
#47024=ORIENTED_EDGE('',*,*,#36078,.F.) ;
#47025=ORIENTED_EDGE('',*,*,#36272,.F.) ;
#47026=ORIENTED_EDGE('',*,*,#36269,.T.) ;
#47027=ORIENTED_EDGE('',*,*,#36268,.T.) ;
#47028=ORIENTED_EDGE('',*,*,#36273,.F.) ;
#47029=ORIENTED_EDGE('',*,*,#36272,.T.) ;
#47030=ORIENTED_EDGE('',*,*,#36270,.T.) ;
#47031=ORIENTED_EDGE('',*,*,#36274,.F.) ;
#47032=ORIENTED_EDGE('',*,*,#36273,.T.) ;
#47033=ORIENTED_EDGE('',*,*,#36089,.F.) ;
#47034=ORIENTED_EDGE('',*,*,#36275,.F.) ;
#47035=ORIENTED_EDGE('',*,*,#36082,.F.) ;
#47036=ORIENTED_EDGE('',*,*,#36274,.T.) ;
#47037=ORIENTED_EDGE('',*,*,#36083,.F.) ;
#47038=ORIENTED_EDGE('',*,*,#36276,.F.) ;
#47039=ORIENTED_EDGE('',*,*,#36107,.F.) ;
#47040=ORIENTED_EDGE('',*,*,#36276,.T.) ;
#47041=ORIENTED_EDGE('',*,*,#36275,.T.) ;
#47042=ORIENTED_EDGE('',*,*,#36277,.F.) ;
#47043=ORIENTED_EDGE('',*,*,#36088,.F.) ;
#47044=ORIENTED_EDGE('',*,*,#36278,.T.) ;
#47045=ORIENTED_EDGE('',*,*,#36104,.F.) ;
#47046=ORIENTED_EDGE('',*,*,#36277,.T.) ;
#47047=ORIENTED_EDGE('',*,*,#36062,.F.) ;
#47048=ORIENTED_EDGE('',*,*,#36279,.T.) ;
#47049=ORIENTED_EDGE('',*,*,#36090,.F.) ;
#47050=ORIENTED_EDGE('',*,*,#36280,.F.) ;
#47051=ORIENTED_EDGE('',*,*,#35941,.F.) ;
#47052=ORIENTED_EDGE('',*,*,#36281,.T.) ;
#47053=ORIENTED_EDGE('',*,*,#36063,.F.) ;
#47054=ORIENTED_EDGE('',*,*,#36280,.T.) ;
#47055=ORIENTED_EDGE('',*,*,#36094,.F.) ;
#47056=ORIENTED_EDGE('',*,*,#36053,.F.) ;
#47057=ORIENTED_EDGE('',*,*,#36282,.T.) ;
#47058=ORIENTED_EDGE('',*,*,#36054,.F.) ;
#47059=ORIENTED_EDGE('',*,*,#35956,.F.) ;
#47060=ORIENTED_EDGE('',*,*,#36059,.F.) ;
#47061=ORIENTED_EDGE('',*,*,#36283,.T.) ;
#47062=ORIENTED_EDGE('',*,*,#36051,.F.) ;
#47063=ORIENTED_EDGE('',*,*,#35954,.F.) ;
#47064=ORIENTED_EDGE('',*,*,#36038,.F.) ;
#47065=ORIENTED_EDGE('',*,*,#36284,.T.) ;
#47066=ORIENTED_EDGE('',*,*,#36096,.F.) ;
#47067=ORIENTED_EDGE('',*,*,#36285,.F.) ;
#47068=ORIENTED_EDGE('',*,*,#36098,.F.) ;
#47069=ORIENTED_EDGE('',*,*,#36286,.T.) ;
#47070=ORIENTED_EDGE('',*,*,#36044,.F.) ;
#47071=ORIENTED_EDGE('',*,*,#36287,.F.) ;
#47072=ORIENTED_EDGE('',*,*,#36288,.F.) ;
#47073=ORIENTED_EDGE('',*,*,#36099,.F.) ;
#47074=ORIENTED_EDGE('',*,*,#36289,.F.) ;
#47075=ORIENTED_EDGE('',*,*,#36043,.F.) ;
#47076=ORIENTED_EDGE('',*,*,#36285,.T.) ;
#47077=ORIENTED_EDGE('',*,*,#36288,.T.) ;
#47078=ORIENTED_EDGE('',*,*,#36290,.F.) ;
#47079=ORIENTED_EDGE('',*,*,#36056,.F.) ;
#47080=ORIENTED_EDGE('',*,*,#36291,.T.) ;
#47081=ORIENTED_EDGE('',*,*,#36048,.F.) ;
#47082=ORIENTED_EDGE('',*,*,#35958,.F.) ;
#47083=ORIENTED_EDGE('',*,*,#36050,.F.) ;
#47084=ORIENTED_EDGE('',*,*,#36292,.T.) ;
#47085=ORIENTED_EDGE('',*,*,#36057,.F.) ;
#47086=ORIENTED_EDGE('',*,*,#35952,.F.) ;
#47087=ORIENTED_EDGE('',*,*,#36289,.T.) ;
#47088=ORIENTED_EDGE('',*,*,#36287,.T.) ;
#47089=ORIENTED_EDGE('',*,*,#36293,.F.) ;
#47090=ORIENTED_EDGE('',*,*,#36290,.T.) ;
#47091=ORIENTED_EDGE('',*,*,#36042,.F.) ;
#47092=ORIENTED_EDGE('',*,*,#36294,.F.) ;
#47093=ORIENTED_EDGE('',*,*,#36039,.F.) ;
#47094=ORIENTED_EDGE('',*,*,#36102,.F.) ;
#47095=ORIENTED_EDGE('',*,*,#36295,.T.) ;
#47096=ORIENTED_EDGE('',*,*,#36036,.F.) ;
#47097=ORIENTED_EDGE('',*,*,#36296,.F.) ;
#47098=ORIENTED_EDGE('',*,*,#36046,.F.) ;
#47099=ORIENTED_EDGE('',*,*,#36297,.T.) ;
#47100=ORIENTED_EDGE('',*,*,#36100,.F.) ;
#47101=ORIENTED_EDGE('',*,*,#36298,.F.) ;
#47102=ORIENTED_EDGE('',*,*,#36293,.T.) ;
#47103=ORIENTED_EDGE('',*,*,#36047,.F.) ;
#47104=ORIENTED_EDGE('',*,*,#36299,.F.) ;
#47105=ORIENTED_EDGE('',*,*,#36040,.F.) ;
#47106=ORIENTED_EDGE('',*,*,#36296,.T.) ;
#47107=ORIENTED_EDGE('',*,*,#36294,.T.) ;
#47108=ORIENTED_EDGE('',*,*,#36300,.F.) ;
#47109=ORIENTED_EDGE('',*,*,#36299,.T.) ;
#47110=ORIENTED_EDGE('',*,*,#36298,.T.) ;
#47111=ORIENTED_EDGE('',*,*,#36301,.F.) ;
#47112=ORIENTED_EDGE('',*,*,#36300,.T.) ;
#47113=ORIENTED_EDGE('',*,*,#36041,.F.) ;
#47114=ORIENTED_EDGE('',*,*,#36301,.T.) ;
#47115=ORIENTED_EDGE('',*,*,#36103,.F.) ;
#47116=ORIENTED_EDGE('',*,*,#35785,.F.) ;
#47117=ORIENTED_EDGE('',*,*,#35761,.F.) ;
#47118=ORIENTED_EDGE('',*,*,#36302,.F.) ;
#47119=ORIENTED_EDGE('',*,*,#35767,.F.) ;
#47120=ORIENTED_EDGE('',*,*,#36023,.F.) ;
#47121=ORIENTED_EDGE('',*,*,#36303,.T.) ;
#47122=ORIENTED_EDGE('',*,*,#35762,.F.) ;
#47123=ORIENTED_EDGE('',*,*,#36304,.F.) ;
#47124=ORIENTED_EDGE('',*,*,#36304,.T.) ;
#47125=ORIENTED_EDGE('',*,*,#36302,.T.) ;
#47126=ORIENTED_EDGE('',*,*,#36305,.F.) ;
#47127=ORIENTED_EDGE('',*,*,#35784,.F.) ;
#47128=ORIENTED_EDGE('',*,*,#35757,.F.) ;
#47129=ORIENTED_EDGE('',*,*,#36306,.F.) ;
#47130=ORIENTED_EDGE('',*,*,#35759,.F.) ;
#47131=ORIENTED_EDGE('',*,*,#36305,.T.) ;
#47132=ORIENTED_EDGE('',*,*,#35760,.F.) ;
#47133=ORIENTED_EDGE('',*,*,#36307,.F.) ;
#47134=ORIENTED_EDGE('',*,*,#36024,.F.) ;
#47135=ORIENTED_EDGE('',*,*,#36307,.T.) ;
#47136=ORIENTED_EDGE('',*,*,#36306,.T.) ;
#47137=ORIENTED_EDGE('',*,*,#36308,.F.) ;
#47138=ORIENTED_EDGE('',*,*,#35756,.F.) ;
#47139=ORIENTED_EDGE('',*,*,#36309,.T.) ;
#47140=ORIENTED_EDGE('',*,*,#36021,.F.) ;
#47141=ORIENTED_EDGE('',*,*,#36308,.T.) ;
#47142=ORIENTED_EDGE('',*,*,#35860,.F.) ;
#47143=ORIENTED_EDGE('',*,*,#35712,.T.) ;
#47144=ORIENTED_EDGE('',*,*,#36310,.T.) ;
#47145=ORIENTED_EDGE('',*,*,#36032,.F.) ;
#47146=ORIENTED_EDGE('',*,*,#36311,.F.) ;
#47147=ORIENTED_EDGE('',*,*,#35838,.F.) ;
#47148=ORIENTED_EDGE('',*,*,#35861,.F.) ;
#47149=ORIENTED_EDGE('',*,*,#36312,.F.) ;
#47150=ORIENTED_EDGE('',*,*,#35858,.F.) ;
#47151=ORIENTED_EDGE('',*,*,#36312,.T.) ;
#47152=ORIENTED_EDGE('',*,*,#36311,.T.) ;
#47153=ORIENTED_EDGE('',*,*,#36313,.F.) ;
#47154=ORIENTED_EDGE('',*,*,#36313,.T.) ;
#47155=ORIENTED_EDGE('',*,*,#36035,.F.) ;
#47156=ORIENTED_EDGE('',*,*,#36314,.F.) ;
#47157=ORIENTED_EDGE('',*,*,#35856,.F.) ;
#47158=ORIENTED_EDGE('',*,*,#35840,.F.) ;
#47159=ORIENTED_EDGE('',*,*,#35857,.F.) ;
#47160=ORIENTED_EDGE('',*,*,#36315,.F.) ;
#47161=ORIENTED_EDGE('',*,*,#35854,.F.) ;
#47162=ORIENTED_EDGE('',*,*,#36315,.T.) ;
#47163=ORIENTED_EDGE('',*,*,#36314,.T.) ;
#47164=ORIENTED_EDGE('',*,*,#36316,.F.) ;
#47165=ORIENTED_EDGE('',*,*,#36034,.F.) ;
#47166=ORIENTED_EDGE('',*,*,#35716,.T.) ;
#47167=ORIENTED_EDGE('',*,*,#36317,.T.) ;
#47168=ORIENTED_EDGE('',*,*,#35855,.F.) ;
#47169=ORIENTED_EDGE('',*,*,#36316,.T.) ;
#47170=ORIENTED_EDGE('',*,*,#35935,.F.) ;
#47171=ORIENTED_EDGE('',*,*,#36318,.T.) ;
#47172=ORIENTED_EDGE('',*,*,#35746,.F.) ;
#47173=ORIENTED_EDGE('',*,*,#36319,.T.) ;
#47174=ORIENTED_EDGE('',*,*,#35805,.F.) ;
#47175=ORIENTED_EDGE('',*,*,#35907,.F.) ;
#47176=ORIENTED_EDGE('',*,*,#35817,.F.) ;
#47177=ORIENTED_EDGE('',*,*,#35841,.F.) ;
#47178=ORIENTED_EDGE('',*,*,#35807,.F.) ;
#47179=ORIENTED_EDGE('',*,*,#35842,.F.) ;
#47180=ORIENTED_EDGE('',*,*,#35815,.F.) ;
#47181=ORIENTED_EDGE('',*,*,#35843,.F.) ;
#47182=ORIENTED_EDGE('',*,*,#35809,.F.) ;
#47183=ORIENTED_EDGE('',*,*,#35844,.F.) ;
#47184=ORIENTED_EDGE('',*,*,#35813,.F.) ;
#47185=ORIENTED_EDGE('',*,*,#35847,.F.) ;
#47186=ORIENTED_EDGE('',*,*,#35802,.F.) ;
#47187=ORIENTED_EDGE('',*,*,#35777,.F.) ;
#47188=ORIENTED_EDGE('',*,*,#35820,.F.) ;
#47189=ORIENTED_EDGE('',*,*,#35900,.F.) ;
#47190=ORIENTED_EDGE('',*,*,#36120,.F.) ;
#47191=ORIENTED_EDGE('',*,*,#36320,.T.) ;
#47192=ORIENTED_EDGE('',*,*,#35779,.F.) ;
#47193=ORIENTED_EDGE('',*,*,#35801,.F.) ;
#47194=ORIENTED_EDGE('',*,*,#36115,.F.) ;
#47195=ORIENTED_EDGE('',*,*,#36321,.T.) ;
#47196=ORIENTED_EDGE('',*,*,#35780,.F.) ;
#47197=ORIENTED_EDGE('',*,*,#36322,.T.) ;
#47198=ORIENTED_EDGE('',*,*,#35781,.F.) ;
#47199=ORIENTED_EDGE('',*,*,#36323,.T.) ;
#47200=ORIENTED_EDGE('',*,*,#36112,.F.) ;
#47201=ORIENTED_EDGE('',*,*,#35821,.F.) ;
#47202=ORIENTED_EDGE('',*,*,#36160,.F.) ;
#47203=ORIENTED_EDGE('',*,*,#36166,.F.) ;
#47204=ORIENTED_EDGE('',*,*,#36165,.F.) ;
#47205=ORIENTED_EDGE('',*,*,#36324,.F.) ;
#47206=ORIENTED_EDGE('',*,*,#36161,.F.) ;
#47207=ORIENTED_EDGE('',*,*,#36254,.F.) ;
#47208=ORIENTED_EDGE('',*,*,#35747,.F.) ;
#47209=ORIENTED_EDGE('',*,*,#36325,.F.) ;
#47210=ORIENTED_EDGE('',*,*,#35929,.F.) ;
#47211=ORIENTED_EDGE('',*,*,#36324,.T.) ;
#47212=ORIENTED_EDGE('',*,*,#35938,.F.) ;
#47213=ORIENTED_EDGE('',*,*,#36257,.F.) ;
#47214=ORIENTED_EDGE('',*,*,#36070,.F.) ;
#47215=ORIENTED_EDGE('',*,*,#36325,.T.) ;
#47216=ORIENTED_EDGE('',*,*,#36318,.F.) ;
#47217=ORIENTED_EDGE('',*,*,#36326,.F.) ;
#47218=ORIENTED_EDGE('',*,*,#36326,.T.) ;
#47219=ORIENTED_EDGE('',*,*,#35934,.F.) ;
#47220=ORIENTED_EDGE('',*,*,#36327,.F.) ;
#47221=ORIENTED_EDGE('',*,*,#35930,.F.) ;
#47222=ORIENTED_EDGE('',*,*,#36169,.F.) ;
#47223=ORIENTED_EDGE('',*,*,#36163,.F.) ;
#47224=ORIENTED_EDGE('',*,*,#36162,.F.) ;
#47225=ORIENTED_EDGE('',*,*,#36327,.T.) ;
#47226=ORIENTED_EDGE('',*,*,#36170,.F.) ;
#47227=ORIENTED_EDGE('',*,*,#36182,.F.) ;
#47228=ORIENTED_EDGE('',*,*,#36172,.F.) ;
#47229=ORIENTED_EDGE('',*,*,#36171,.F.) ;
#47230=ORIENTED_EDGE('',*,*,#36328,.F.) ;
#47231=ORIENTED_EDGE('',*,*,#36183,.F.) ;
#47232=ORIENTED_EDGE('',*,*,#36328,.T.) ;
#47233=ORIENTED_EDGE('',*,*,#35936,.F.) ;
#47234=ORIENTED_EDGE('',*,*,#36329,.F.) ;
#47235=ORIENTED_EDGE('',*,*,#35926,.F.) ;
#47236=ORIENTED_EDGE('',*,*,#36329,.T.) ;
#47237=ORIENTED_EDGE('',*,*,#36319,.F.) ;
#47238=ORIENTED_EDGE('',*,*,#36330,.F.) ;
#47239=ORIENTED_EDGE('',*,*,#36281,.F.) ;
#47240=ORIENTED_EDGE('',*,*,#35940,.F.) ;
#47241=ORIENTED_EDGE('',*,*,#36331,.F.) ;
#47242=ORIENTED_EDGE('',*,*,#35927,.F.) ;
#47243=ORIENTED_EDGE('',*,*,#36330,.T.) ;
#47244=ORIENTED_EDGE('',*,*,#35751,.F.) ;
#47245=ORIENTED_EDGE('',*,*,#36261,.F.) ;
#47246=ORIENTED_EDGE('',*,*,#36064,.F.) ;
#47247=ORIENTED_EDGE('',*,*,#36331,.T.) ;
#47248=ORIENTED_EDGE('',*,*,#36168,.F.) ;
#47249=ORIENTED_EDGE('',*,*,#36167,.F.) ;
#47250=ORIENTED_EDGE('',*,*,#36180,.F.) ;
#47251=ORIENTED_EDGE('',*,*,#36179,.F.) ;
#47252=ORIENTED_EDGE('',*,*,#35755,.F.) ;
#47253=ORIENTED_EDGE('',*,*,#36332,.T.) ;
#47254=ORIENTED_EDGE('',*,*,#36025,.F.) ;
#47255=ORIENTED_EDGE('',*,*,#36333,.F.) ;
#47256=ORIENTED_EDGE('',*,*,#36309,.F.) ;
#47257=ORIENTED_EDGE('',*,*,#36333,.T.) ;
#47258=ORIENTED_EDGE('',*,*,#36031,.F.) ;
#47259=ORIENTED_EDGE('',*,*,#36334,.F.) ;
#47260=ORIENTED_EDGE('',*,*,#36022,.F.) ;
#47261=ORIENTED_EDGE('',*,*,#36334,.T.) ;
#47262=ORIENTED_EDGE('',*,*,#36030,.F.) ;
#47263=ORIENTED_EDGE('',*,*,#36335,.F.) ;
#47264=ORIENTED_EDGE('',*,*,#36336,.F.) ;
#47265=ORIENTED_EDGE('',*,*,#36337,.F.) ;
#47266=ORIENTED_EDGE('',*,*,#36338,.F.) ;
#47267=ORIENTED_EDGE('',*,*,#35763,.F.) ;
#47268=ORIENTED_EDGE('',*,*,#36303,.F.) ;
#47269=ORIENTED_EDGE('',*,*,#35786,.F.) ;
#47270=ORIENTED_EDGE('',*,*,#35765,.F.) ;
#47271=ORIENTED_EDGE('',*,*,#36339,.F.) ;
#47272=ORIENTED_EDGE('',*,*,#35863,.F.) ;
#47273=ORIENTED_EDGE('',*,*,#35764,.F.) ;
#47274=ORIENTED_EDGE('',*,*,#36338,.T.) ;
#47275=ORIENTED_EDGE('',*,*,#36337,.T.) ;
#47276=ORIENTED_EDGE('',*,*,#36336,.T.) ;
#47277=ORIENTED_EDGE('',*,*,#36335,.T.) ;
#47278=ORIENTED_EDGE('',*,*,#36340,.F.) ;
#47279=ORIENTED_EDGE('',*,*,#35864,.F.) ;
#47280=ORIENTED_EDGE('',*,*,#36339,.T.) ;
#47281=ORIENTED_EDGE('',*,*,#35715,.F.) ;
#47282=ORIENTED_EDGE('',*,*,#36341,.T.) ;
#47283=ORIENTED_EDGE('',*,*,#35851,.F.) ;
#47284=ORIENTED_EDGE('',*,*,#36317,.F.) ;
#47285=ORIENTED_EDGE('',*,*,#36340,.T.) ;
#47286=ORIENTED_EDGE('',*,*,#36029,.F.) ;
#47287=ORIENTED_EDGE('',*,*,#36342,.F.) ;
#47288=ORIENTED_EDGE('',*,*,#35865,.F.) ;
#47289=ORIENTED_EDGE('',*,*,#35836,.F.) ;
#47290=ORIENTED_EDGE('',*,*,#35867,.F.) ;
#47291=ORIENTED_EDGE('',*,*,#36343,.F.) ;
#47292=ORIENTED_EDGE('',*,*,#35862,.F.) ;
#47293=ORIENTED_EDGE('',*,*,#35717,.T.) ;
#47294=ORIENTED_EDGE('',*,*,#36033,.F.) ;
#47295=ORIENTED_EDGE('',*,*,#36344,.F.) ;
#47296=ORIENTED_EDGE('',*,*,#36027,.F.) ;
#47297=ORIENTED_EDGE('',*,*,#35866,.F.) ;
#47298=ORIENTED_EDGE('',*,*,#36342,.T.) ;
#47299=ORIENTED_EDGE('',*,*,#36345,.F.) ;
#47300=ORIENTED_EDGE('',*,*,#36346,.F.) ;
#47301=ORIENTED_EDGE('',*,*,#36347,.F.) ;
#47302=ORIENTED_EDGE('',*,*,#35710,.F.) ;
#47303=ORIENTED_EDGE('',*,*,#35709,.F.) ;
#47304=ORIENTED_EDGE('',*,*,#35859,.F.) ;
#47305=ORIENTED_EDGE('',*,*,#36343,.T.) ;
#47306=ORIENTED_EDGE('',*,*,#35711,.F.) ;
#47307=ORIENTED_EDGE('',*,*,#36347,.T.) ;
#47308=ORIENTED_EDGE('',*,*,#36346,.T.) ;
#47309=ORIENTED_EDGE('',*,*,#36345,.T.) ;
#47310=ORIENTED_EDGE('',*,*,#36028,.F.) ;
#47311=ORIENTED_EDGE('',*,*,#36344,.T.) ;
#47312=ORIENTED_EDGE('',*,*,#36310,.F.) ;
#47313=ORIENTED_EDGE('',*,*,#36348,.F.) ;
#47314=ORIENTED_EDGE('',*,*,#35773,.F.) ;
#47315=ORIENTED_EDGE('',*,*,#35823,.F.) ;
#47316=ORIENTED_EDGE('',*,*,#36114,.F.) ;
#47317=ORIENTED_EDGE('',*,*,#36230,.F.) ;
#47318=ORIENTED_EDGE('',*,*,#36348,.T.) ;
#47319=ORIENTED_EDGE('',*,*,#36349,.F.) ;
#47320=ORIENTED_EDGE('',*,*,#35735,.F.) ;
#47321=ORIENTED_EDGE('',*,*,#36349,.T.) ;
#47322=ORIENTED_EDGE('',*,*,#36113,.F.) ;
#47323=ORIENTED_EDGE('',*,*,#36350,.F.) ;
#47324=ORIENTED_EDGE('',*,*,#36117,.F.) ;
#47325=ORIENTED_EDGE('',*,*,#36323,.F.) ;
#47326=ORIENTED_EDGE('',*,*,#36321,.F.) ;
#47327=ORIENTED_EDGE('',*,*,#36350,.T.) ;
#47328=ORIENTED_EDGE('',*,*,#36351,.T.) ;
#47329=ORIENTED_EDGE('',*,*,#36256,.F.) ;
#47330=ORIENTED_EDGE('',*,*,#36352,.F.) ;
#47331=ORIENTED_EDGE('',*,*,#36259,.F.) ;
#47332=ORIENTED_EDGE('',*,*,#36351,.F.) ;
#47333=ORIENTED_EDGE('',*,*,#36079,.F.) ;
#47334=ORIENTED_EDGE('',*,*,#36353,.F.) ;
#47335=ORIENTED_EDGE('',*,*,#36076,.F.) ;
#47336=ORIENTED_EDGE('',*,*,#36352,.T.) ;
#47337=ORIENTED_EDGE('',*,*,#36067,.F.) ;
#47338=ORIENTED_EDGE('',*,*,#36354,.F.) ;
#47339=ORIENTED_EDGE('',*,*,#36109,.F.) ;
#47340=ORIENTED_EDGE('',*,*,#36353,.T.) ;
#47341=ORIENTED_EDGE('',*,*,#36271,.F.) ;
#47342=ORIENTED_EDGE('',*,*,#36355,.F.) ;
#47343=ORIENTED_EDGE('',*,*,#36266,.F.) ;
#47344=ORIENTED_EDGE('',*,*,#36354,.T.) ;
#47345=ORIENTED_EDGE('',*,*,#36263,.F.) ;
#47346=ORIENTED_EDGE('',*,*,#36356,.F.) ;
#47347=ORIENTED_EDGE('',*,*,#36267,.F.) ;
#47348=ORIENTED_EDGE('',*,*,#36355,.T.) ;
#47349=ORIENTED_EDGE('',*,*,#36105,.F.) ;
#47350=ORIENTED_EDGE('',*,*,#36357,.F.) ;
#47351=ORIENTED_EDGE('',*,*,#36061,.F.) ;
#47352=ORIENTED_EDGE('',*,*,#36356,.T.) ;
#47353=ORIENTED_EDGE('',*,*,#36091,.F.) ;
#47354=ORIENTED_EDGE('',*,*,#36358,.F.) ;
#47355=ORIENTED_EDGE('',*,*,#36087,.F.) ;
#47356=ORIENTED_EDGE('',*,*,#36357,.T.) ;
#47357=ORIENTED_EDGE('',*,*,#36278,.F.) ;
#47358=ORIENTED_EDGE('',*,*,#36358,.T.) ;
#47359=ORIENTED_EDGE('',*,*,#36279,.F.) ;
#47360=ORIENTED_EDGE('',*,*,#36359,.T.) ;
#47361=ORIENTED_EDGE('',*,*,#36282,.F.) ;
#47362=ORIENTED_EDGE('',*,*,#36360,.F.) ;
#47363=ORIENTED_EDGE('',*,*,#36284,.F.) ;
#47364=ORIENTED_EDGE('',*,*,#36359,.F.) ;
#47365=ORIENTED_EDGE('',*,*,#36037,.F.) ;
#47366=ORIENTED_EDGE('',*,*,#36361,.F.) ;
#47367=ORIENTED_EDGE('',*,*,#36055,.F.) ;
#47368=ORIENTED_EDGE('',*,*,#36360,.T.) ;
#47369=ORIENTED_EDGE('',*,*,#36052,.F.) ;
#47370=ORIENTED_EDGE('',*,*,#36362,.F.) ;
#47371=ORIENTED_EDGE('',*,*,#36097,.F.) ;
#47372=ORIENTED_EDGE('',*,*,#36361,.T.) ;
#47373=ORIENTED_EDGE('',*,*,#36295,.F.) ;
#47374=ORIENTED_EDGE('',*,*,#36363,.F.) ;
#47375=ORIENTED_EDGE('',*,*,#36291,.F.) ;
#47376=ORIENTED_EDGE('',*,*,#36362,.T.) ;
#47377=ORIENTED_EDGE('',*,*,#36283,.F.) ;
#47378=ORIENTED_EDGE('',*,*,#36364,.F.) ;
#47379=ORIENTED_EDGE('',*,*,#36286,.F.) ;
#47380=ORIENTED_EDGE('',*,*,#36363,.T.) ;
#47381=ORIENTED_EDGE('',*,*,#36101,.F.) ;
#47382=ORIENTED_EDGE('',*,*,#36365,.F.) ;
#47383=ORIENTED_EDGE('',*,*,#36049,.F.) ;
#47384=ORIENTED_EDGE('',*,*,#36364,.T.) ;
#47385=ORIENTED_EDGE('',*,*,#36058,.F.) ;
#47386=ORIENTED_EDGE('',*,*,#36366,.F.) ;
#47387=ORIENTED_EDGE('',*,*,#36045,.F.) ;
#47388=ORIENTED_EDGE('',*,*,#36365,.T.) ;
#47389=ORIENTED_EDGE('',*,*,#36297,.F.) ;
#47390=ORIENTED_EDGE('',*,*,#36366,.T.) ;
#47391=ORIENTED_EDGE('',*,*,#36292,.F.) ;
#47392=ORIENTED_EDGE('',*,*,#35799,.F.) ;
#47393=ORIENTED_EDGE('',*,*,#35769,.F.) ;
#47394=ORIENTED_EDGE('',*,*,#36367,.F.) ;
#47395=ORIENTED_EDGE('',*,*,#36118,.F.) ;
#47396=ORIENTED_EDGE('',*,*,#36367,.T.) ;
#47397=ORIENTED_EDGE('',*,*,#36220,.F.) ;
#47398=ORIENTED_EDGE('',*,*,#35737,.F.) ;
#47399=ORIENTED_EDGE('',*,*,#36368,.F.) ;
#47400=ORIENTED_EDGE('',*,*,#36368,.T.) ;
#47401=ORIENTED_EDGE('',*,*,#36116,.F.) ;
#47402=ORIENTED_EDGE('',*,*,#36369,.F.) ;
#47403=ORIENTED_EDGE('',*,*,#36119,.F.) ;
#47404=ORIENTED_EDGE('',*,*,#36322,.F.) ;
#47405=ORIENTED_EDGE('',*,*,#36320,.F.) ;
#47406=ORIENTED_EDGE('',*,*,#36369,.T.) ;
#47407=ORIENTED_EDGE('',*,*,#35853,.F.) ;
#47408=ORIENTED_EDGE('',*,*,#36370,.F.) ;
#47409=ORIENTED_EDGE('',*,*,#35848,.F.) ;
#47410=ORIENTED_EDGE('',*,*,#35811,.F.) ;
#47411=ORIENTED_EDGE('',*,*,#35852,.F.) ;
#47412=ORIENTED_EDGE('',*,*,#36341,.F.) ;
#47413=ORIENTED_EDGE('',*,*,#35714,.F.) ;
#47414=ORIENTED_EDGE('',*,*,#36371,.F.) ;
#47415=ORIENTED_EDGE('',*,*,#35849,.F.) ;
#47416=ORIENTED_EDGE('',*,*,#36370,.T.) ;
#47417=ORIENTED_EDGE('',*,*,#36371,.T.) ;
#47418=ORIENTED_EDGE('',*,*,#36026,.F.) ;
#47419=ORIENTED_EDGE('',*,*,#36372,.F.) ;
#47420=ORIENTED_EDGE('',*,*,#35850,.F.) ;
#47421=ORIENTED_EDGE('',*,*,#36332,.F.) ;
#47422=ORIENTED_EDGE('',*,*,#35754,.F.) ;
#47423=ORIENTED_EDGE('',*,*,#36373,.F.) ;
#47424=ORIENTED_EDGE('',*,*,#35845,.F.) ;
#47425=ORIENTED_EDGE('',*,*,#36372,.T.) ;
#47426=ORIENTED_EDGE('',*,*,#35783,.F.) ;
#47427=ORIENTED_EDGE('',*,*,#35846,.F.) ;
#47428=ORIENTED_EDGE('',*,*,#36373,.T.) ;
#47429=ORIENTED_EDGE('',*,*,#35753,.F.) ;
#47430=ORIENTED_EDGE('',*,*,#36374,.T.) ;
#47431=ORIENTED_EDGE('',*,*,#36375,.T.) ;
#47432=ORIENTED_EDGE('',*,*,#36376,.T.) ;
#47433=ORIENTED_EDGE('',*,*,#36377,.F.) ;
#47434=ORIENTED_EDGE('',*,*,#36378,.F.) ;
#47435=ORIENTED_EDGE('',*,*,#36379,.T.) ;
#47436=ORIENTED_EDGE('',*,*,#36380,.T.) ;
#47437=ORIENTED_EDGE('',*,*,#36381,.F.) ;
#47438=ORIENTED_EDGE('',*,*,#36382,.F.) ;
#47439=ORIENTED_EDGE('',*,*,#36383,.F.) ;
#47440=ORIENTED_EDGE('',*,*,#36384,.F.) ;
#47441=ORIENTED_EDGE('',*,*,#36385,.T.) ;
#47442=ORIENTED_EDGE('',*,*,#36386,.F.) ;
#47443=ORIENTED_EDGE('',*,*,#36385,.F.) ;
#47444=ORIENTED_EDGE('',*,*,#36387,.F.) ;
#47445=ORIENTED_EDGE('',*,*,#36388,.T.) ;
#47446=ORIENTED_EDGE('',*,*,#36389,.F.) ;
#47447=ORIENTED_EDGE('',*,*,#36388,.F.) ;
#47448=ORIENTED_EDGE('',*,*,#36390,.F.) ;
#47449=ORIENTED_EDGE('',*,*,#36391,.F.) ;
#47450=ORIENTED_EDGE('',*,*,#36392,.T.) ;
#47451=ORIENTED_EDGE('',*,*,#36393,.T.) ;
#47452=ORIENTED_EDGE('',*,*,#36394,.F.) ;
#47453=ORIENTED_EDGE('',*,*,#36395,.F.) ;
#47454=ORIENTED_EDGE('',*,*,#36396,.F.) ;
#47455=ORIENTED_EDGE('',*,*,#36397,.T.) ;
#47456=ORIENTED_EDGE('',*,*,#36398,.F.) ;
#47457=ORIENTED_EDGE('',*,*,#36399,.F.) ;
#47458=ORIENTED_EDGE('',*,*,#36400,.T.) ;
#47459=ORIENTED_EDGE('',*,*,#36401,.F.) ;
#47460=ORIENTED_EDGE('',*,*,#36402,.T.) ;
#47461=ORIENTED_EDGE('',*,*,#36386,.T.) ;
#47462=ORIENTED_EDGE('',*,*,#36403,.T.) ;
#47463=ORIENTED_EDGE('',*,*,#36387,.T.) ;
#47464=ORIENTED_EDGE('',*,*,#36403,.F.) ;
#47465=ORIENTED_EDGE('',*,*,#36399,.T.) ;
#47466=ORIENTED_EDGE('',*,*,#36404,.T.) ;
#47467=ORIENTED_EDGE('',*,*,#36405,.T.) ;
#47468=ORIENTED_EDGE('',*,*,#36396,.T.) ;
#47469=ORIENTED_EDGE('',*,*,#36406,.F.) ;
#47470=ORIENTED_EDGE('',*,*,#36407,.T.) ;
#47471=ORIENTED_EDGE('',*,*,#36408,.F.) ;
#47472=ORIENTED_EDGE('',*,*,#36394,.T.) ;
#47473=ORIENTED_EDGE('',*,*,#36409,.T.) ;
#47474=ORIENTED_EDGE('',*,*,#36410,.T.) ;
#47475=ORIENTED_EDGE('',*,*,#36411,.T.) ;
#47476=ORIENTED_EDGE('',*,*,#36412,.T.) ;
#47477=ORIENTED_EDGE('',*,*,#36413,.T.) ;
#47478=ORIENTED_EDGE('',*,*,#36414,.T.) ;
#47479=ORIENTED_EDGE('',*,*,#36415,.T.) ;
#47480=ORIENTED_EDGE('',*,*,#36416,.T.) ;
#47481=ORIENTED_EDGE('',*,*,#36417,.T.) ;
#47482=ORIENTED_EDGE('',*,*,#36418,.T.) ;
#47483=ORIENTED_EDGE('',*,*,#36419,.T.) ;
#47484=ORIENTED_EDGE('',*,*,#36420,.T.) ;
#47485=ORIENTED_EDGE('',*,*,#36421,.T.) ;
#47486=ORIENTED_EDGE('',*,*,#36422,.T.) ;
#47487=ORIENTED_EDGE('',*,*,#36423,.T.) ;
#47488=ORIENTED_EDGE('',*,*,#36424,.T.) ;
#47489=ORIENTED_EDGE('',*,*,#36425,.T.) ;
#47490=ORIENTED_EDGE('',*,*,#36426,.T.) ;
#47491=ORIENTED_EDGE('',*,*,#36427,.T.) ;
#47492=ORIENTED_EDGE('',*,*,#36428,.T.) ;
#47493=ORIENTED_EDGE('',*,*,#36429,.T.) ;
#47494=ORIENTED_EDGE('',*,*,#36430,.T.) ;
#47495=ORIENTED_EDGE('',*,*,#36431,.T.) ;
#47496=ORIENTED_EDGE('',*,*,#36432,.T.) ;
#47497=ORIENTED_EDGE('',*,*,#36433,.T.) ;
#47498=ORIENTED_EDGE('',*,*,#36434,.T.) ;
#47499=ORIENTED_EDGE('',*,*,#36435,.T.) ;
#47500=ORIENTED_EDGE('',*,*,#36436,.T.) ;
#47501=ORIENTED_EDGE('',*,*,#36437,.F.) ;
#47502=ORIENTED_EDGE('',*,*,#36438,.T.) ;
#47503=ORIENTED_EDGE('',*,*,#36439,.T.) ;
#47504=ORIENTED_EDGE('',*,*,#36440,.T.) ;
#47505=ORIENTED_EDGE('',*,*,#36441,.F.) ;
#47506=ORIENTED_EDGE('',*,*,#36442,.T.) ;
#47507=ORIENTED_EDGE('',*,*,#36443,.T.) ;
#47508=ORIENTED_EDGE('',*,*,#36444,.T.) ;
#47509=ORIENTED_EDGE('',*,*,#36445,.T.) ;
#47510=ORIENTED_EDGE('',*,*,#36446,.T.) ;
#47511=ORIENTED_EDGE('',*,*,#36447,.F.) ;
#47512=ORIENTED_EDGE('',*,*,#36448,.T.) ;
#47513=ORIENTED_EDGE('',*,*,#36417,.F.) ;
#47514=ORIENTED_EDGE('',*,*,#36449,.T.) ;
#47515=ORIENTED_EDGE('',*,*,#36423,.F.) ;
#47516=ORIENTED_EDGE('',*,*,#36450,.T.) ;
#47517=ORIENTED_EDGE('',*,*,#36431,.F.) ;
#47518=ORIENTED_EDGE('',*,*,#36451,.T.) ;
#47519=ORIENTED_EDGE('',*,*,#36452,.F.) ;
#47520=ORIENTED_EDGE('',*,*,#36453,.T.) ;
#47521=ORIENTED_EDGE('',*,*,#36454,.F.) ;
#47522=ORIENTED_EDGE('',*,*,#36455,.T.) ;
#47523=ORIENTED_EDGE('',*,*,#36456,.T.) ;
#47524=ORIENTED_EDGE('',*,*,#36457,.T.) ;
#47525=ORIENTED_EDGE('',*,*,#36458,.F.) ;
#47526=ORIENTED_EDGE('',*,*,#36459,.T.) ;
#47527=ORIENTED_EDGE('',*,*,#36460,.T.) ;
#47528=ORIENTED_EDGE('',*,*,#36461,.T.) ;
#47529=ORIENTED_EDGE('',*,*,#36462,.F.) ;
#47530=ORIENTED_EDGE('',*,*,#36463,.T.) ;
#47531=ORIENTED_EDGE('',*,*,#36435,.F.) ;
#47532=ORIENTED_EDGE('',*,*,#36464,.T.) ;
#47533=ORIENTED_EDGE('',*,*,#36465,.T.) ;
#47534=ORIENTED_EDGE('',*,*,#36466,.T.) ;
#47535=ORIENTED_EDGE('',*,*,#36443,.F.) ;
#47536=ORIENTED_EDGE('',*,*,#36467,.T.) ;
#47537=ORIENTED_EDGE('',*,*,#36468,.F.) ;
#47538=ORIENTED_EDGE('',*,*,#36469,.F.) ;
#47539=ORIENTED_EDGE('',*,*,#36470,.T.) ;
#47540=ORIENTED_EDGE('',*,*,#36471,.F.) ;
#47541=ORIENTED_EDGE('',*,*,#36472,.T.) ;
#47542=ORIENTED_EDGE('',*,*,#36473,.F.) ;
#47543=ORIENTED_EDGE('',*,*,#36474,.T.) ;
#47544=ORIENTED_EDGE('',*,*,#36475,.T.) ;
#47545=ORIENTED_EDGE('',*,*,#36476,.T.) ;
#47546=ORIENTED_EDGE('',*,*,#36477,.T.) ;
#47547=ORIENTED_EDGE('',*,*,#36478,.T.) ;
#47548=ORIENTED_EDGE('',*,*,#36479,.T.) ;
#47549=ORIENTED_EDGE('',*,*,#36480,.T.) ;
#47550=ORIENTED_EDGE('',*,*,#36481,.T.) ;
#47551=ORIENTED_EDGE('',*,*,#36482,.T.) ;
#47552=ORIENTED_EDGE('',*,*,#36483,.T.) ;
#47553=ORIENTED_EDGE('',*,*,#36484,.T.) ;
#47554=ORIENTED_EDGE('',*,*,#36485,.T.) ;
#47555=ORIENTED_EDGE('',*,*,#36441,.T.) ;
#47556=ORIENTED_EDGE('',*,*,#36486,.T.) ;
#47557=ORIENTED_EDGE('',*,*,#36487,.T.) ;
#47558=ORIENTED_EDGE('',*,*,#36488,.T.) ;
#47559=ORIENTED_EDGE('',*,*,#36437,.T.) ;
#47560=ORIENTED_EDGE('',*,*,#36489,.T.) ;
#47561=ORIENTED_EDGE('',*,*,#36490,.F.) ;
#47562=ORIENTED_EDGE('',*,*,#36491,.T.) ;
#47563=ORIENTED_EDGE('',*,*,#36492,.F.) ;
#47564=ORIENTED_EDGE('',*,*,#36493,.T.) ;
#47565=ORIENTED_EDGE('',*,*,#36494,.T.) ;
#47566=ORIENTED_EDGE('',*,*,#36495,.T.) ;
#47567=ORIENTED_EDGE('',*,*,#36496,.F.) ;
#47568=ORIENTED_EDGE('',*,*,#36497,.T.) ;
#47569=ORIENTED_EDGE('',*,*,#36498,.F.) ;
#47570=ORIENTED_EDGE('',*,*,#36499,.T.) ;
#47571=ORIENTED_EDGE('',*,*,#36500,.T.) ;
#47572=ORIENTED_EDGE('',*,*,#36501,.T.) ;
#47573=ORIENTED_EDGE('',*,*,#36502,.T.) ;
#47574=ORIENTED_EDGE('',*,*,#36503,.T.) ;
#47575=ORIENTED_EDGE('',*,*,#36504,.T.) ;
#47576=ORIENTED_EDGE('',*,*,#36505,.T.) ;
#47577=ORIENTED_EDGE('',*,*,#36471,.T.) ;
#47578=ORIENTED_EDGE('',*,*,#36506,.T.) ;
#47579=ORIENTED_EDGE('',*,*,#36481,.F.) ;
#47580=ORIENTED_EDGE('',*,*,#36507,.T.) ;
#47581=ORIENTED_EDGE('',*,*,#36473,.T.) ;
#47582=ORIENTED_EDGE('',*,*,#36508,.T.) ;
#47583=ORIENTED_EDGE('',*,*,#36479,.F.) ;
#47584=ORIENTED_EDGE('',*,*,#36509,.T.) ;
#47585=ORIENTED_EDGE('',*,*,#36510,.T.) ;
#47586=ORIENTED_EDGE('',*,*,#36511,.T.) ;
#47587=ORIENTED_EDGE('',*,*,#36447,.T.) ;
#47588=ORIENTED_EDGE('',*,*,#36512,.T.) ;
#47589=ORIENTED_EDGE('',*,*,#36477,.F.) ;
#47590=ORIENTED_EDGE('',*,*,#36513,.T.) ;
#47591=ORIENTED_EDGE('',*,*,#36514,.T.) ;
#47592=ORIENTED_EDGE('',*,*,#36515,.T.) ;
#47593=ORIENTED_EDGE('',*,*,#36516,.T.) ;
#47594=ORIENTED_EDGE('',*,*,#36517,.T.) ;
#47595=ORIENTED_EDGE('',*,*,#36518,.T.) ;
#47596=ORIENTED_EDGE('',*,*,#36475,.F.) ;
#47597=ORIENTED_EDGE('',*,*,#36519,.T.) ;
#47598=ORIENTED_EDGE('',*,*,#36520,.T.) ;
#47599=ORIENTED_EDGE('',*,*,#36521,.T.) ;
#47600=ORIENTED_EDGE('',*,*,#36522,.T.) ;
#47601=ORIENTED_EDGE('',*,*,#36504,.F.) ;
#47602=ORIENTED_EDGE('',*,*,#36523,.T.) ;
#47603=ORIENTED_EDGE('',*,*,#36524,.T.) ;
#47604=ORIENTED_EDGE('',*,*,#36378,.T.) ;
#47605=ORIENTED_EDGE('',*,*,#36525,.T.) ;
#47606=ORIENTED_EDGE('',*,*,#36526,.T.) ;
#47607=ORIENTED_EDGE('',*,*,#36502,.F.) ;
#47608=ORIENTED_EDGE('',*,*,#36527,.T.) ;
#47609=ORIENTED_EDGE('',*,*,#36528,.T.) ;
#47610=ORIENTED_EDGE('',*,*,#36529,.T.) ;
#47611=ORIENTED_EDGE('',*,*,#36530,.T.) ;
#47612=ORIENTED_EDGE('',*,*,#36531,.T.) ;
#47613=ORIENTED_EDGE('',*,*,#36532,.T.) ;
#47614=ORIENTED_EDGE('',*,*,#36500,.F.) ;
#47615=ORIENTED_EDGE('',*,*,#36533,.T.) ;
#47616=ORIENTED_EDGE('',*,*,#36534,.T.) ;
#47617=ORIENTED_EDGE('',*,*,#36535,.F.) ;
#47618=ORIENTED_EDGE('',*,*,#36536,.T.) ;
#47619=ORIENTED_EDGE('',*,*,#36537,.F.) ;
#47620=ORIENTED_EDGE('',*,*,#36538,.T.) ;
#47621=ORIENTED_EDGE('',*,*,#36539,.T.) ;
#47622=ORIENTED_EDGE('',*,*,#36452,.T.) ;
#47623=ORIENTED_EDGE('',*,*,#36540,.F.) ;
#47624=ORIENTED_EDGE('',*,*,#36541,.T.) ;
#47625=ORIENTED_EDGE('',*,*,#36458,.T.) ;
#47626=ORIENTED_EDGE('',*,*,#36542,.T.) ;
#47627=ORIENTED_EDGE('',*,*,#36543,.F.) ;
#47628=ORIENTED_EDGE('',*,*,#36544,.T.) ;
#47629=ORIENTED_EDGE('',*,*,#36545,.F.) ;
#47630=ORIENTED_EDGE('',*,*,#36546,.T.) ;
#47631=ORIENTED_EDGE('',*,*,#36547,.T.) ;
#47632=ORIENTED_EDGE('',*,*,#36548,.T.) ;
#47633=ORIENTED_EDGE('',*,*,#36549,.F.) ;
#47634=ORIENTED_EDGE('',*,*,#36550,.T.) ;
#47635=ORIENTED_EDGE('',*,*,#36551,.F.) ;
#47636=ORIENTED_EDGE('',*,*,#36552,.T.) ;
#47637=ORIENTED_EDGE('',*,*,#36494,.F.) ;
#47638=ORIENTED_EDGE('',*,*,#36553,.T.) ;
#47639=ORIENTED_EDGE('',*,*,#36554,.F.) ;
#47640=ORIENTED_EDGE('',*,*,#36555,.T.) ;
#47641=ORIENTED_EDGE('',*,*,#36556,.F.) ;
#47642=ORIENTED_EDGE('',*,*,#36557,.T.) ;
#47643=ORIENTED_EDGE('',*,*,#36558,.T.) ;
#47644=ORIENTED_EDGE('',*,*,#36559,.T.) ;
#47645=ORIENTED_EDGE('',*,*,#36560,.F.) ;
#47646=ORIENTED_EDGE('',*,*,#36561,.T.) ;
#47647=ORIENTED_EDGE('',*,*,#36389,.T.) ;
#47648=ORIENTED_EDGE('',*,*,#36562,.F.) ;
#47649=ORIENTED_EDGE('',*,*,#36563,.T.) ;
#47650=ORIENTED_EDGE('',*,*,#36564,.F.) ;
#47651=ORIENTED_EDGE('',*,*,#36468,.T.) ;
#47652=ORIENTED_EDGE('',*,*,#36565,.T.) ;
#47653=ORIENTED_EDGE('',*,*,#36484,.F.) ;
#47654=ORIENTED_EDGE('',*,*,#36566,.F.) ;
#47655=ORIENTED_EDGE('',*,*,#36567,.T.) ;
#47656=ORIENTED_EDGE('',*,*,#36568,.F.) ;
#47657=ORIENTED_EDGE('',*,*,#36569,.T.) ;
#47658=ORIENTED_EDGE('',*,*,#36570,.F.) ;
#47659=ORIENTED_EDGE('',*,*,#36571,.T.) ;
#47660=ORIENTED_EDGE('',*,*,#36566,.T.) ;
#47661=ORIENTED_EDGE('',*,*,#36483,.F.) ;
#47662=ORIENTED_EDGE('',*,*,#36572,.T.) ;
#47663=ORIENTED_EDGE('',*,*,#36469,.T.) ;
#47664=ORIENTED_EDGE('',*,*,#36564,.T.) ;
#47665=ORIENTED_EDGE('',*,*,#36573,.T.) ;
#47666=ORIENTED_EDGE('',*,*,#36574,.F.) ;
#47667=ORIENTED_EDGE('',*,*,#36575,.T.) ;
#47668=ORIENTED_EDGE('',*,*,#36576,.T.) ;
#47669=ORIENTED_EDGE('',*,*,#36577,.T.) ;
#47670=ORIENTED_EDGE('',*,*,#36578,.F.) ;
#47671=ORIENTED_EDGE('',*,*,#36579,.F.) ;
#47672=ORIENTED_EDGE('',*,*,#36580,.T.) ;
#47673=ORIENTED_EDGE('',*,*,#36581,.T.) ;
#47674=ORIENTED_EDGE('',*,*,#36582,.T.) ;
#47675=ORIENTED_EDGE('',*,*,#36583,.T.) ;
#47676=ORIENTED_EDGE('',*,*,#36584,.T.) ;
#47677=ORIENTED_EDGE('',*,*,#36585,.T.) ;
#47678=ORIENTED_EDGE('',*,*,#36586,.T.) ;
#47679=ORIENTED_EDGE('',*,*,#36587,.T.) ;
#47680=ORIENTED_EDGE('',*,*,#36588,.T.) ;
#47681=ORIENTED_EDGE('',*,*,#36589,.T.) ;
#47682=ORIENTED_EDGE('',*,*,#36590,.T.) ;
#47683=ORIENTED_EDGE('',*,*,#36591,.T.) ;
#47684=ORIENTED_EDGE('',*,*,#36592,.T.) ;
#47685=ORIENTED_EDGE('',*,*,#36593,.T.) ;
#47686=ORIENTED_EDGE('',*,*,#36594,.T.) ;
#47687=ORIENTED_EDGE('',*,*,#36595,.T.) ;
#47688=ORIENTED_EDGE('',*,*,#36596,.T.) ;
#47689=ORIENTED_EDGE('',*,*,#36597,.T.) ;
#47690=ORIENTED_EDGE('',*,*,#36598,.T.) ;
#47691=ORIENTED_EDGE('',*,*,#36599,.T.) ;
#47692=ORIENTED_EDGE('',*,*,#36600,.T.) ;
#47693=ORIENTED_EDGE('',*,*,#36601,.T.) ;
#47694=ORIENTED_EDGE('',*,*,#36602,.T.) ;
#47695=ORIENTED_EDGE('',*,*,#36603,.T.) ;
#47696=ORIENTED_EDGE('',*,*,#36604,.T.) ;
#47697=ORIENTED_EDGE('',*,*,#36605,.T.) ;
#47698=ORIENTED_EDGE('',*,*,#36606,.T.) ;
#47699=ORIENTED_EDGE('',*,*,#36607,.T.) ;
#47700=ORIENTED_EDGE('',*,*,#36608,.T.) ;
#47701=ORIENTED_EDGE('',*,*,#36609,.T.) ;
#47702=ORIENTED_EDGE('',*,*,#36610,.T.) ;
#47703=ORIENTED_EDGE('',*,*,#36611,.T.) ;
#47704=ORIENTED_EDGE('',*,*,#36612,.T.) ;
#47705=ORIENTED_EDGE('',*,*,#36613,.T.) ;
#47706=ORIENTED_EDGE('',*,*,#36614,.T.) ;
#47707=ORIENTED_EDGE('',*,*,#36615,.T.) ;
#47708=ORIENTED_EDGE('',*,*,#36384,.T.) ;
#47709=ORIENTED_EDGE('',*,*,#36616,.F.) ;
#47710=ORIENTED_EDGE('',*,*,#36617,.T.) ;
#47711=ORIENTED_EDGE('',*,*,#36618,.T.) ;
#47712=ORIENTED_EDGE('',*,*,#36619,.T.) ;
#47713=ORIENTED_EDGE('',*,*,#36620,.T.) ;
#47714=ORIENTED_EDGE('',*,*,#36621,.T.) ;
#47715=ORIENTED_EDGE('',*,*,#36622,.T.) ;
#47716=ORIENTED_EDGE('',*,*,#36623,.T.) ;
#47717=ORIENTED_EDGE('',*,*,#36624,.F.) ;
#47718=ORIENTED_EDGE('',*,*,#36625,.T.) ;
#47719=ORIENTED_EDGE('',*,*,#36462,.T.) ;
#47720=ORIENTED_EDGE('',*,*,#36626,.T.) ;
#47721=ORIENTED_EDGE('',*,*,#36627,.T.) ;
#47722=ORIENTED_EDGE('',*,*,#36628,.T.) ;
#47723=ORIENTED_EDGE('',*,*,#36629,.T.) ;
#47724=ORIENTED_EDGE('',*,*,#36460,.F.) ;
#47725=ORIENTED_EDGE('',*,*,#36630,.T.) ;
#47726=ORIENTED_EDGE('',*,*,#36631,.T.) ;
#47727=ORIENTED_EDGE('',*,*,#36632,.T.) ;
#47728=ORIENTED_EDGE('',*,*,#36633,.T.) ;
#47729=ORIENTED_EDGE('',*,*,#36634,.T.) ;
#47730=ORIENTED_EDGE('',*,*,#36398,.T.) ;
#47731=ORIENTED_EDGE('',*,*,#36635,.T.) ;
#47732=ORIENTED_EDGE('',*,*,#36636,.T.) ;
#47733=ORIENTED_EDGE('',*,*,#36637,.T.) ;
#47734=ORIENTED_EDGE('',*,*,#36638,.T.) ;
#47735=ORIENTED_EDGE('',*,*,#36639,.T.) ;
#47736=ORIENTED_EDGE('',*,*,#36640,.T.) ;
#47737=ORIENTED_EDGE('',*,*,#36641,.T.) ;
#47738=ORIENTED_EDGE('',*,*,#36642,.T.) ;
#47739=ORIENTED_EDGE('',*,*,#36643,.T.) ;
#47740=ORIENTED_EDGE('',*,*,#36391,.T.) ;
#47741=ORIENTED_EDGE('',*,*,#36644,.T.) ;
#47742=ORIENTED_EDGE('',*,*,#36645,.T.) ;
#47743=ORIENTED_EDGE('',*,*,#36646,.T.) ;
#47744=ORIENTED_EDGE('',*,*,#36647,.T.) ;
#47745=ORIENTED_EDGE('',*,*,#36648,.T.) ;
#47746=ORIENTED_EDGE('',*,*,#36492,.T.) ;
#47747=ORIENTED_EDGE('',*,*,#36649,.T.) ;
#47748=ORIENTED_EDGE('',*,*,#36650,.T.) ;
#47749=ORIENTED_EDGE('',*,*,#36651,.T.) ;
#47750=ORIENTED_EDGE('',*,*,#36490,.T.) ;
#47751=ORIENTED_EDGE('',*,*,#36652,.T.) ;
#47752=ORIENTED_EDGE('',*,*,#36653,.F.) ;
#47753=ORIENTED_EDGE('',*,*,#36654,.T.) ;
#47754=ORIENTED_EDGE('',*,*,#36655,.T.) ;
#47755=ORIENTED_EDGE('',*,*,#36656,.T.) ;
#47756=ORIENTED_EDGE('',*,*,#36657,.T.) ;
#47757=ORIENTED_EDGE('',*,*,#36454,.T.) ;
#47758=ORIENTED_EDGE('',*,*,#36658,.T.) ;
#47759=ORIENTED_EDGE('',*,*,#36659,.T.) ;
#47760=ORIENTED_EDGE('',*,*,#36660,.T.) ;
#47761=ORIENTED_EDGE('',*,*,#36661,.T.) ;
#47762=ORIENTED_EDGE('',*,*,#36456,.F.) ;
#47763=ORIENTED_EDGE('',*,*,#36662,.T.) ;
#47764=ORIENTED_EDGE('',*,*,#36663,.T.) ;
#47765=ORIENTED_EDGE('',*,*,#36664,.T.) ;
#47766=ORIENTED_EDGE('',*,*,#36665,.T.) ;
#47767=ORIENTED_EDGE('',*,*,#36666,.T.) ;
#47768=ORIENTED_EDGE('',*,*,#36667,.T.) ;
#47769=ORIENTED_EDGE('',*,*,#36668,.T.) ;
#47770=ORIENTED_EDGE('',*,*,#36669,.T.) ;
#47771=ORIENTED_EDGE('',*,*,#36670,.T.) ;
#47772=ORIENTED_EDGE('',*,*,#36671,.T.) ;
#47773=ORIENTED_EDGE('',*,*,#36672,.T.) ;
#47774=ORIENTED_EDGE('',*,*,#36673,.T.) ;
#47775=ORIENTED_EDGE('',*,*,#36674,.T.) ;
#47776=ORIENTED_EDGE('',*,*,#36496,.T.) ;
#47777=ORIENTED_EDGE('',*,*,#36675,.T.) ;
#47778=ORIENTED_EDGE('',*,*,#36676,.T.) ;
#47779=ORIENTED_EDGE('',*,*,#36677,.T.) ;
#47780=ORIENTED_EDGE('',*,*,#36678,.T.) ;
#47781=ORIENTED_EDGE('',*,*,#36679,.T.) ;
#47782=ORIENTED_EDGE('',*,*,#36680,.T.) ;
#47783=ORIENTED_EDGE('',*,*,#36681,.T.) ;
#47784=ORIENTED_EDGE('',*,*,#36682,.T.) ;
#47785=ORIENTED_EDGE('',*,*,#36683,.T.) ;
#47786=ORIENTED_EDGE('',*,*,#36498,.T.) ;
#47787=ORIENTED_EDGE('',*,*,#36684,.T.) ;
#47788=ORIENTED_EDGE('',*,*,#36685,.T.) ;
#47789=ORIENTED_EDGE('',*,*,#36686,.T.) ;
#47790=ORIENTED_EDGE('',*,*,#36687,.T.) ;
#47791=ORIENTED_EDGE('',*,*,#36688,.T.) ;
#47792=ORIENTED_EDGE('',*,*,#36689,.T.) ;
#47793=ORIENTED_EDGE('',*,*,#36690,.T.) ;
#47794=ORIENTED_EDGE('',*,*,#36691,.T.) ;
#47795=ORIENTED_EDGE('',*,*,#36383,.T.) ;
#47796=ORIENTED_EDGE('',*,*,#36692,.T.) ;
#47797=ORIENTED_EDGE('',*,*,#36693,.T.) ;
#47798=ORIENTED_EDGE('',*,*,#36694,.T.) ;
#47799=ORIENTED_EDGE('',*,*,#36695,.T.) ;
#47800=ORIENTED_EDGE('',*,*,#36696,.T.) ;
#47801=ORIENTED_EDGE('',*,*,#36697,.T.) ;
#47802=ORIENTED_EDGE('',*,*,#36698,.T.) ;
#47803=ORIENTED_EDGE('',*,*,#36699,.T.) ;
#47804=ORIENTED_EDGE('',*,*,#36700,.T.) ;
#47805=ORIENTED_EDGE('',*,*,#36701,.T.) ;
#47806=ORIENTED_EDGE('',*,*,#36702,.T.) ;
#47807=ORIENTED_EDGE('',*,*,#36703,.T.) ;
#47808=ORIENTED_EDGE('',*,*,#36704,.T.) ;
#47809=ORIENTED_EDGE('',*,*,#36705,.T.) ;
#47810=ORIENTED_EDGE('',*,*,#36706,.T.) ;
#47811=ORIENTED_EDGE('',*,*,#36707,.T.) ;
#47812=ORIENTED_EDGE('',*,*,#36708,.T.) ;
#47813=ORIENTED_EDGE('',*,*,#36709,.T.) ;
#47814=ORIENTED_EDGE('',*,*,#36710,.T.) ;
#47815=ORIENTED_EDGE('',*,*,#36711,.T.) ;
#47816=ORIENTED_EDGE('',*,*,#36712,.T.) ;
#47817=ORIENTED_EDGE('',*,*,#36713,.T.) ;
#47818=ORIENTED_EDGE('',*,*,#36714,.T.) ;
#47819=ORIENTED_EDGE('',*,*,#36715,.T.) ;
#47820=ORIENTED_EDGE('',*,*,#36616,.T.) ;
#47821=ORIENTED_EDGE('',*,*,#36716,.T.) ;
#47822=ORIENTED_EDGE('',*,*,#36717,.T.) ;
#47823=ORIENTED_EDGE('',*,*,#36718,.T.) ;
#47824=ORIENTED_EDGE('',*,*,#36620,.F.) ;
#47825=ORIENTED_EDGE('',*,*,#36719,.T.) ;
#47826=ORIENTED_EDGE('',*,*,#36720,.T.) ;
#47827=ORIENTED_EDGE('',*,*,#36721,.T.) ;
#47828=ORIENTED_EDGE('',*,*,#36622,.F.) ;
#47829=ORIENTED_EDGE('',*,*,#36722,.T.) ;
#47830=ORIENTED_EDGE('',*,*,#36723,.T.) ;
#47831=ORIENTED_EDGE('',*,*,#36724,.T.) ;
#47832=ORIENTED_EDGE('',*,*,#36618,.F.) ;
#47833=ORIENTED_EDGE('',*,*,#36725,.T.) ;
#47834=ORIENTED_EDGE('',*,*,#36726,.T.) ;
#47835=ORIENTED_EDGE('',*,*,#36727,.T.) ;
#47836=ORIENTED_EDGE('',*,*,#36728,.T.) ;
#47837=ORIENTED_EDGE('',*,*,#36729,.T.) ;
#47838=ORIENTED_EDGE('',*,*,#36730,.T.) ;
#47839=ORIENTED_EDGE('',*,*,#36731,.T.) ;
#47840=ORIENTED_EDGE('',*,*,#36732,.T.) ;
#47841=ORIENTED_EDGE('',*,*,#36733,.T.) ;
#47842=ORIENTED_EDGE('',*,*,#36734,.T.) ;
#47843=ORIENTED_EDGE('',*,*,#36735,.T.) ;
#47844=ORIENTED_EDGE('',*,*,#36736,.T.) ;
#47845=ORIENTED_EDGE('',*,*,#36737,.F.) ;
#47846=ORIENTED_EDGE('',*,*,#36738,.T.) ;
#47847=ORIENTED_EDGE('',*,*,#36414,.F.) ;
#47848=ORIENTED_EDGE('',*,*,#36739,.T.) ;
#47849=ORIENTED_EDGE('',*,*,#36740,.T.) ;
#47850=ORIENTED_EDGE('',*,*,#36741,.T.) ;
#47851=ORIENTED_EDGE('',*,*,#36742,.T.) ;
#47852=ORIENTED_EDGE('',*,*,#36737,.T.) ;
#47853=ORIENTED_EDGE('',*,*,#36743,.T.) ;
#47854=ORIENTED_EDGE('',*,*,#36744,.T.) ;
#47855=ORIENTED_EDGE('',*,*,#36745,.T.) ;
#47856=ORIENTED_EDGE('',*,*,#36746,.T.) ;
#47857=ORIENTED_EDGE('',*,*,#36747,.T.) ;
#47858=ORIENTED_EDGE('',*,*,#36748,.T.) ;
#47859=ORIENTED_EDGE('',*,*,#36749,.T.) ;
#47860=ORIENTED_EDGE('',*,*,#36750,.T.) ;
#47861=ORIENTED_EDGE('',*,*,#36751,.T.) ;
#47862=ORIENTED_EDGE('',*,*,#36752,.T.) ;
#47863=ORIENTED_EDGE('',*,*,#36753,.T.) ;
#47864=ORIENTED_EDGE('',*,*,#36754,.T.) ;
#47865=ORIENTED_EDGE('',*,*,#36755,.T.) ;
#47866=ORIENTED_EDGE('',*,*,#36756,.T.) ;
#47867=ORIENTED_EDGE('',*,*,#36757,.T.) ;
#47868=ORIENTED_EDGE('',*,*,#36758,.F.) ;
#47869=ORIENTED_EDGE('',*,*,#36607,.F.) ;
#47870=ORIENTED_EDGE('',*,*,#36759,.T.) ;
#47871=ORIENTED_EDGE('',*,*,#36758,.T.) ;
#47872=ORIENTED_EDGE('',*,*,#36760,.T.) ;
#47873=ORIENTED_EDGE('',*,*,#36761,.T.) ;
#47874=ORIENTED_EDGE('',*,*,#36762,.T.) ;
#47875=ORIENTED_EDGE('',*,*,#36763,.T.) ;
#47876=ORIENTED_EDGE('',*,*,#36764,.T.) ;
#47877=ORIENTED_EDGE('',*,*,#36765,.T.) ;
#47878=ORIENTED_EDGE('',*,*,#36766,.T.) ;
#47879=ORIENTED_EDGE('',*,*,#36767,.T.) ;
#47880=ORIENTED_EDGE('',*,*,#36768,.T.) ;
#47881=ORIENTED_EDGE('',*,*,#36769,.T.) ;
#47882=ORIENTED_EDGE('',*,*,#36770,.T.) ;
#47883=ORIENTED_EDGE('',*,*,#36771,.T.) ;
#47884=ORIENTED_EDGE('',*,*,#36772,.T.) ;
#47885=ORIENTED_EDGE('',*,*,#36773,.T.) ;
#47886=ORIENTED_EDGE('',*,*,#36774,.T.) ;
#47887=ORIENTED_EDGE('',*,*,#36775,.T.) ;
#47888=ORIENTED_EDGE('',*,*,#36776,.T.) ;
#47889=ORIENTED_EDGE('',*,*,#36777,.T.) ;
#47890=ORIENTED_EDGE('',*,*,#36778,.T.) ;
#47891=ORIENTED_EDGE('',*,*,#36779,.T.) ;
#47892=ORIENTED_EDGE('',*,*,#36487,.F.) ;
#47893=ORIENTED_EDGE('',*,*,#36780,.T.) ;
#47894=ORIENTED_EDGE('',*,*,#36781,.T.) ;
#47895=ORIENTED_EDGE('',*,*,#36401,.T.) ;
#47896=ORIENTED_EDGE('',*,*,#36782,.T.) ;
#47897=ORIENTED_EDGE('',*,*,#36465,.F.) ;
#47898=ORIENTED_EDGE('',*,*,#36783,.T.) ;
#47899=ORIENTED_EDGE('',*,*,#36784,.T.) ;
#47900=ORIENTED_EDGE('',*,*,#36785,.T.) ;
#47901=ORIENTED_EDGE('',*,*,#36786,.F.) ;
#47902=ORIENTED_EDGE('',*,*,#36684,.F.) ;
#47903=ORIENTED_EDGE('',*,*,#36497,.F.) ;
#47904=ORIENTED_EDGE('',*,*,#36677,.F.) ;
#47905=ORIENTED_EDGE('',*,*,#36787,.F.) ;
#47906=ORIENTED_EDGE('',*,*,#36786,.T.) ;
#47907=ORIENTED_EDGE('',*,*,#36788,.F.) ;
#47908=ORIENTED_EDGE('',*,*,#36495,.F.) ;
#47909=ORIENTED_EDGE('',*,*,#36552,.F.) ;
#47910=ORIENTED_EDGE('',*,*,#36789,.F.) ;
#47911=ORIENTED_EDGE('',*,*,#36675,.F.) ;
#47912=ORIENTED_EDGE('',*,*,#36788,.T.) ;
#47913=ORIENTED_EDGE('',*,*,#36676,.F.) ;
#47914=ORIENTED_EDGE('',*,*,#36790,.F.) ;
#47915=ORIENTED_EDGE('',*,*,#36672,.F.) ;
#47916=ORIENTED_EDGE('',*,*,#36787,.T.) ;
#47917=ORIENTED_EDGE('',*,*,#36671,.F.) ;
#47918=ORIENTED_EDGE('',*,*,#36791,.F.) ;
#47919=ORIENTED_EDGE('',*,*,#36685,.F.) ;
#47920=ORIENTED_EDGE('',*,*,#36789,.T.) ;
#47921=ORIENTED_EDGE('',*,*,#36551,.T.) ;
#47922=ORIENTED_EDGE('',*,*,#36792,.F.) ;
#47923=ORIENTED_EDGE('',*,*,#36790,.T.) ;
#47924=ORIENTED_EDGE('',*,*,#36793,.F.) ;
#47925=ORIENTED_EDGE('',*,*,#36791,.T.) ;
#47926=ORIENTED_EDGE('',*,*,#36794,.F.) ;
#47927=ORIENTED_EDGE('',*,*,#36455,.F.) ;
#47928=ORIENTED_EDGE('',*,*,#36657,.F.) ;
#47929=ORIENTED_EDGE('',*,*,#36795,.F.) ;
#47930=ORIENTED_EDGE('',*,*,#36662,.F.) ;
#47931=ORIENTED_EDGE('',*,*,#36796,.F.) ;
#47932=ORIENTED_EDGE('',*,*,#36660,.F.) ;
#47933=ORIENTED_EDGE('',*,*,#36797,.F.) ;
#47934=ORIENTED_EDGE('',*,*,#36666,.F.) ;
#47935=ORIENTED_EDGE('',*,*,#36457,.F.) ;
#47936=ORIENTED_EDGE('',*,*,#36661,.F.) ;
#47937=ORIENTED_EDGE('',*,*,#36798,.F.) ;
#47938=ORIENTED_EDGE('',*,*,#36542,.F.) ;
#47939=ORIENTED_EDGE('',*,*,#36792,.T.) ;
#47940=ORIENTED_EDGE('',*,*,#36550,.F.) ;
#47941=ORIENTED_EDGE('',*,*,#36799,.F.) ;
#47942=ORIENTED_EDGE('',*,*,#36673,.F.) ;
#47943=ORIENTED_EDGE('',*,*,#36794,.T.) ;
#47944=ORIENTED_EDGE('',*,*,#36674,.F.) ;
#47945=ORIENTED_EDGE('',*,*,#36800,.F.) ;
#47946=ORIENTED_EDGE('',*,*,#36681,.F.) ;
#47947=ORIENTED_EDGE('',*,*,#36793,.T.) ;
#47948=ORIENTED_EDGE('',*,*,#36680,.F.) ;
#47949=ORIENTED_EDGE('',*,*,#36801,.F.) ;
#47950=ORIENTED_EDGE('',*,*,#36682,.F.) ;
#47951=ORIENTED_EDGE('',*,*,#36499,.F.) ;
#47952=ORIENTED_EDGE('',*,*,#36683,.F.) ;
#47953=ORIENTED_EDGE('',*,*,#36802,.F.) ;
#47954=ORIENTED_EDGE('',*,*,#36533,.F.) ;
#47955=ORIENTED_EDGE('',*,*,#36797,.T.) ;
#47956=ORIENTED_EDGE('',*,*,#36795,.T.) ;
#47957=ORIENTED_EDGE('',*,*,#36803,.F.) ;
#47958=ORIENTED_EDGE('',*,*,#36798,.T.) ;
#47959=ORIENTED_EDGE('',*,*,#36796,.T.) ;
#47960=ORIENTED_EDGE('',*,*,#36804,.F.) ;
#47961=ORIENTED_EDGE('',*,*,#36543,.T.) ;
#47962=ORIENTED_EDGE('',*,*,#36799,.T.) ;
#47963=ORIENTED_EDGE('',*,*,#36549,.T.) ;
#47964=ORIENTED_EDGE('',*,*,#36805,.F.) ;
#47965=ORIENTED_EDGE('',*,*,#36800,.T.) ;
#47966=ORIENTED_EDGE('',*,*,#36802,.T.) ;
#47967=ORIENTED_EDGE('',*,*,#36801,.T.) ;
#47968=ORIENTED_EDGE('',*,*,#36806,.F.) ;
#47969=ORIENTED_EDGE('',*,*,#36803,.T.) ;
#47970=ORIENTED_EDGE('',*,*,#36656,.F.) ;
#47971=ORIENTED_EDGE('',*,*,#36807,.F.) ;
#47972=ORIENTED_EDGE('',*,*,#36663,.F.) ;
#47973=ORIENTED_EDGE('',*,*,#36808,.F.) ;
#47974=ORIENTED_EDGE('',*,*,#36664,.F.) ;
#47975=ORIENTED_EDGE('',*,*,#36809,.F.) ;
#47976=ORIENTED_EDGE('',*,*,#36670,.F.) ;
#47977=ORIENTED_EDGE('',*,*,#36804,.T.) ;
#47978=ORIENTED_EDGE('',*,*,#36665,.F.) ;
#47979=ORIENTED_EDGE('',*,*,#36810,.F.) ;
#47980=ORIENTED_EDGE('',*,*,#36544,.F.) ;
#47981=ORIENTED_EDGE('',*,*,#36805,.T.) ;
#47982=ORIENTED_EDGE('',*,*,#36548,.F.) ;
#47983=ORIENTED_EDGE('',*,*,#36811,.F.) ;
#47984=ORIENTED_EDGE('',*,*,#36678,.F.) ;
#47985=ORIENTED_EDGE('',*,*,#36806,.T.) ;
#47986=ORIENTED_EDGE('',*,*,#36679,.F.) ;
#47987=ORIENTED_EDGE('',*,*,#36812,.F.) ;
#47988=ORIENTED_EDGE('',*,*,#36534,.F.) ;
#47989=ORIENTED_EDGE('',*,*,#36809,.T.) ;
#47990=ORIENTED_EDGE('',*,*,#36807,.T.) ;
#47991=ORIENTED_EDGE('',*,*,#36813,.F.) ;
#47992=ORIENTED_EDGE('',*,*,#36810,.T.) ;
#47993=ORIENTED_EDGE('',*,*,#36808,.T.) ;
#47994=ORIENTED_EDGE('',*,*,#36814,.F.) ;
#47995=ORIENTED_EDGE('',*,*,#36545,.T.) ;
#47996=ORIENTED_EDGE('',*,*,#36812,.T.) ;
#47997=ORIENTED_EDGE('',*,*,#36811,.T.) ;
#47998=ORIENTED_EDGE('',*,*,#36815,.F.) ;
#47999=ORIENTED_EDGE('',*,*,#36535,.T.) ;
#48000=ORIENTED_EDGE('',*,*,#36453,.F.) ;
#48001=ORIENTED_EDGE('',*,*,#36539,.F.) ;
#48002=ORIENTED_EDGE('',*,*,#36816,.F.) ;
#48003=ORIENTED_EDGE('',*,*,#36658,.F.) ;
#48004=ORIENTED_EDGE('',*,*,#36813,.T.) ;
#48005=ORIENTED_EDGE('',*,*,#36659,.F.) ;
#48006=ORIENTED_EDGE('',*,*,#36817,.F.) ;
#48007=ORIENTED_EDGE('',*,*,#36667,.F.) ;
#48008=ORIENTED_EDGE('',*,*,#36814,.T.) ;
#48009=ORIENTED_EDGE('',*,*,#36669,.F.) ;
#48010=ORIENTED_EDGE('',*,*,#36818,.F.) ;
#48011=ORIENTED_EDGE('',*,*,#36546,.F.) ;
#48012=ORIENTED_EDGE('',*,*,#36815,.T.) ;
#48013=ORIENTED_EDGE('',*,*,#36547,.F.) ;
#48014=ORIENTED_EDGE('',*,*,#36819,.F.) ;
#48015=ORIENTED_EDGE('',*,*,#36536,.F.) ;
#48016=ORIENTED_EDGE('',*,*,#36817,.T.) ;
#48017=ORIENTED_EDGE('',*,*,#36816,.T.) ;
#48018=ORIENTED_EDGE('',*,*,#36820,.F.) ;
#48019=ORIENTED_EDGE('',*,*,#36819,.T.) ;
#48020=ORIENTED_EDGE('',*,*,#36818,.T.) ;
#48021=ORIENTED_EDGE('',*,*,#36821,.F.) ;
#48022=ORIENTED_EDGE('',*,*,#36537,.T.) ;
#48023=ORIENTED_EDGE('',*,*,#36820,.T.) ;
#48024=ORIENTED_EDGE('',*,*,#36538,.F.) ;
#48025=ORIENTED_EDGE('',*,*,#36821,.T.) ;
#48026=ORIENTED_EDGE('',*,*,#36668,.F.) ;
#48027=ORIENTED_EDGE('',*,*,#36822,.F.) ;
#48028=ORIENTED_EDGE('',*,*,#36823,.F.) ;
#48029=ORIENTED_EDGE('',*,*,#36824,.F.) ;
#48030=ORIENTED_EDGE('',*,*,#36615,.F.) ;
#48031=ORIENTED_EDGE('',*,*,#36825,.T.) ;
#48032=ORIENTED_EDGE('',*,*,#36826,.T.) ;
#48033=ORIENTED_EDGE('',*,*,#36597,.F.) ;
#48034=ORIENTED_EDGE('',*,*,#36823,.T.) ;
#48035=ORIENTED_EDGE('',*,*,#36596,.F.) ;
#48036=ORIENTED_EDGE('',*,*,#36827,.T.) ;
#48037=ORIENTED_EDGE('',*,*,#36828,.T.) ;
#48038=ORIENTED_EDGE('',*,*,#36589,.F.) ;
#48039=ORIENTED_EDGE('',*,*,#36824,.T.) ;
#48040=ORIENTED_EDGE('',*,*,#36822,.T.) ;
#48041=ORIENTED_EDGE('',*,*,#36588,.F.) ;
#48042=ORIENTED_EDGE('',*,*,#36829,.F.) ;
#48043=ORIENTED_EDGE('',*,*,#36608,.F.) ;
#48044=ORIENTED_EDGE('',*,*,#36604,.F.) ;
#48045=ORIENTED_EDGE('',*,*,#36830,.T.) ;
#48046=ORIENTED_EDGE('',*,*,#36831,.T.) ;
#48047=ORIENTED_EDGE('',*,*,#36614,.F.) ;
#48048=ORIENTED_EDGE('',*,*,#36832,.T.) ;
#48049=ORIENTED_EDGE('',*,*,#36833,.T.) ;
#48050=ORIENTED_EDGE('',*,*,#36582,.F.) ;
#48051=ORIENTED_EDGE('',*,*,#36834,.T.) ;
#48052=ORIENTED_EDGE('',*,*,#36835,.T.) ;
#48053=ORIENTED_EDGE('',*,*,#36598,.F.) ;
#48054=ORIENTED_EDGE('',*,*,#36836,.T.) ;
#48055=ORIENTED_EDGE('',*,*,#36837,.T.) ;
#48056=ORIENTED_EDGE('',*,*,#36838,.F.) ;
#48057=ORIENTED_EDGE('',*,*,#36829,.T.) ;
#48058=ORIENTED_EDGE('',*,*,#36839,.F.) ;
#48059=ORIENTED_EDGE('',*,*,#36579,.T.) ;
#48060=ORIENTED_EDGE('',*,*,#36840,.F.) ;
#48061=ORIENTED_EDGE('',*,*,#36841,.F.) ;
#48062=ORIENTED_EDGE('',*,*,#36609,.F.) ;
#48063=ORIENTED_EDGE('',*,*,#36838,.T.) ;
#48064=ORIENTED_EDGE('',*,*,#36841,.T.) ;
#48065=ORIENTED_EDGE('',*,*,#36842,.F.) ;
#48066=ORIENTED_EDGE('',*,*,#36843,.F.) ;
#48067=ORIENTED_EDGE('',*,*,#36593,.F.) ;
#48068=ORIENTED_EDGE('',*,*,#36844,.T.) ;
#48069=ORIENTED_EDGE('',*,*,#36845,.T.) ;
#48070=ORIENTED_EDGE('',*,*,#36613,.F.) ;
#48071=ORIENTED_EDGE('',*,*,#36846,.F.) ;
#48072=ORIENTED_EDGE('',*,*,#36583,.F.) ;
#48073=ORIENTED_EDGE('',*,*,#36847,.T.) ;
#48074=ORIENTED_EDGE('',*,*,#36848,.T.) ;
#48075=ORIENTED_EDGE('',*,*,#36590,.F.) ;
#48076=ORIENTED_EDGE('',*,*,#36849,.F.) ;
#48077=ORIENTED_EDGE('',*,*,#36839,.T.) ;
#48078=ORIENTED_EDGE('',*,*,#36587,.F.) ;
#48079=ORIENTED_EDGE('',*,*,#36850,.F.) ;
#48080=ORIENTED_EDGE('',*,*,#36851,.F.) ;
#48081=ORIENTED_EDGE('',*,*,#36852,.F.) ;
#48082=ORIENTED_EDGE('',*,*,#36563,.F.) ;
#48083=ORIENTED_EDGE('',*,*,#36853,.F.) ;
#48084=ORIENTED_EDGE('',*,*,#36840,.T.) ;
#48085=ORIENTED_EDGE('',*,*,#36581,.F.) ;
#48086=ORIENTED_EDGE('',*,*,#36853,.T.) ;
#48087=ORIENTED_EDGE('',*,*,#36562,.T.) ;
#48088=ORIENTED_EDGE('',*,*,#36854,.F.) ;
#48089=ORIENTED_EDGE('',*,*,#36842,.T.) ;
#48090=ORIENTED_EDGE('',*,*,#36610,.F.) ;
#48091=ORIENTED_EDGE('',*,*,#36843,.T.) ;
#48092=ORIENTED_EDGE('',*,*,#36855,.F.) ;
#48093=ORIENTED_EDGE('',*,*,#36856,.F.) ;
#48094=ORIENTED_EDGE('',*,*,#36849,.T.) ;
#48095=ORIENTED_EDGE('',*,*,#36846,.T.) ;
#48096=ORIENTED_EDGE('',*,*,#36857,.F.) ;
#48097=ORIENTED_EDGE('',*,*,#36858,.F.) ;
#48098=ORIENTED_EDGE('',*,*,#36850,.T.) ;
#48099=ORIENTED_EDGE('',*,*,#36859,.F.) ;
#48100=ORIENTED_EDGE('',*,*,#36580,.F.) ;
#48101=ORIENTED_EDGE('',*,*,#36851,.T.) ;
#48102=ORIENTED_EDGE('',*,*,#36860,.F.) ;
#48103=ORIENTED_EDGE('',*,*,#36573,.F.) ;
#48104=ORIENTED_EDGE('',*,*,#36852,.T.) ;
#48105=ORIENTED_EDGE('',*,*,#36861,.F.) ;
#48106=ORIENTED_EDGE('',*,*,#36855,.T.) ;
#48107=ORIENTED_EDGE('',*,*,#36854,.T.) ;
#48108=ORIENTED_EDGE('',*,*,#36569,.F.) ;
#48109=ORIENTED_EDGE('',*,*,#36856,.T.) ;
#48110=ORIENTED_EDGE('',*,*,#36862,.F.) ;
#48111=ORIENTED_EDGE('',*,*,#36863,.F.) ;
#48112=ORIENTED_EDGE('',*,*,#36857,.T.) ;
#48113=ORIENTED_EDGE('',*,*,#36612,.F.) ;
#48114=ORIENTED_EDGE('',*,*,#36864,.F.) ;
#48115=ORIENTED_EDGE('',*,*,#36584,.F.) ;
#48116=ORIENTED_EDGE('',*,*,#36859,.T.) ;
#48117=ORIENTED_EDGE('',*,*,#36586,.F.) ;
#48118=ORIENTED_EDGE('',*,*,#36865,.F.) ;
#48119=ORIENTED_EDGE('',*,*,#36866,.F.) ;
#48120=ORIENTED_EDGE('',*,*,#36860,.T.) ;
#48121=ORIENTED_EDGE('',*,*,#36858,.T.) ;
#48122=ORIENTED_EDGE('',*,*,#36867,.F.) ;
#48123=ORIENTED_EDGE('',*,*,#36574,.T.) ;
#48124=ORIENTED_EDGE('',*,*,#36861,.T.) ;
#48125=ORIENTED_EDGE('',*,*,#36568,.T.) ;
#48126=ORIENTED_EDGE('',*,*,#36868,.F.) ;
#48127=ORIENTED_EDGE('',*,*,#36862,.T.) ;
#48128=ORIENTED_EDGE('',*,*,#36869,.F.) ;
#48129=ORIENTED_EDGE('',*,*,#36870,.F.) ;
#48130=ORIENTED_EDGE('',*,*,#36611,.F.) ;
#48131=ORIENTED_EDGE('',*,*,#36863,.T.) ;
#48132=ORIENTED_EDGE('',*,*,#36870,.T.) ;
#48133=ORIENTED_EDGE('',*,*,#36578,.T.) ;
#48134=ORIENTED_EDGE('',*,*,#36871,.F.) ;
#48135=ORIENTED_EDGE('',*,*,#36864,.T.) ;
#48136=ORIENTED_EDGE('',*,*,#36872,.F.) ;
#48137=ORIENTED_EDGE('',*,*,#36865,.T.) ;
#48138=ORIENTED_EDGE('',*,*,#36873,.F.) ;
#48139=ORIENTED_EDGE('',*,*,#36867,.T.) ;
#48140=ORIENTED_EDGE('',*,*,#36866,.T.) ;
#48141=ORIENTED_EDGE('',*,*,#36874,.F.) ;
#48142=ORIENTED_EDGE('',*,*,#36575,.F.) ;
#48143=ORIENTED_EDGE('',*,*,#36868,.T.) ;
#48144=ORIENTED_EDGE('',*,*,#36567,.F.) ;
#48145=ORIENTED_EDGE('',*,*,#36875,.F.) ;
#48146=ORIENTED_EDGE('',*,*,#36576,.F.) ;
#48147=ORIENTED_EDGE('',*,*,#36869,.T.) ;
#48148=ORIENTED_EDGE('',*,*,#36585,.F.) ;
#48149=ORIENTED_EDGE('',*,*,#36871,.T.) ;
#48150=ORIENTED_EDGE('',*,*,#36876,.F.) ;
#48151=ORIENTED_EDGE('',*,*,#36873,.T.) ;
#48152=ORIENTED_EDGE('',*,*,#36874,.T.) ;
#48153=ORIENTED_EDGE('',*,*,#36872,.T.) ;
#48154=ORIENTED_EDGE('',*,*,#36877,.F.) ;
#48155=ORIENTED_EDGE('',*,*,#36570,.T.) ;
#48156=ORIENTED_EDGE('',*,*,#36875,.T.) ;
#48157=ORIENTED_EDGE('',*,*,#36571,.F.) ;
#48158=ORIENTED_EDGE('',*,*,#36877,.T.) ;
#48159=ORIENTED_EDGE('',*,*,#36876,.T.) ;
#48160=ORIENTED_EDGE('',*,*,#36577,.F.) ;
#48161=ORIENTED_EDGE('',*,*,#36878,.F.) ;
#48162=ORIENTED_EDGE('',*,*,#36626,.F.) ;
#48163=ORIENTED_EDGE('',*,*,#36461,.F.) ;
#48164=ORIENTED_EDGE('',*,*,#36632,.F.) ;
#48165=ORIENTED_EDGE('',*,*,#36879,.F.) ;
#48166=ORIENTED_EDGE('',*,*,#36878,.T.) ;
#48167=ORIENTED_EDGE('',*,*,#36880,.F.) ;
#48168=ORIENTED_EDGE('',*,*,#36459,.F.) ;
#48169=ORIENTED_EDGE('',*,*,#36541,.F.) ;
#48170=ORIENTED_EDGE('',*,*,#36881,.F.) ;
#48171=ORIENTED_EDGE('',*,*,#36630,.F.) ;
#48172=ORIENTED_EDGE('',*,*,#36880,.T.) ;
#48173=ORIENTED_EDGE('',*,*,#36631,.F.) ;
#48174=ORIENTED_EDGE('',*,*,#36882,.F.) ;
#48175=ORIENTED_EDGE('',*,*,#36637,.F.) ;
#48176=ORIENTED_EDGE('',*,*,#36879,.T.) ;
#48177=ORIENTED_EDGE('',*,*,#36636,.F.) ;
#48178=ORIENTED_EDGE('',*,*,#36883,.F.) ;
#48179=ORIENTED_EDGE('',*,*,#36627,.F.) ;
#48180=ORIENTED_EDGE('',*,*,#36463,.F.) ;
#48181=ORIENTED_EDGE('',*,*,#36625,.F.) ;
#48182=ORIENTED_EDGE('',*,*,#36884,.F.) ;
#48183=ORIENTED_EDGE('',*,*,#36436,.F.) ;
#48184=ORIENTED_EDGE('',*,*,#36404,.F.) ;
#48185=ORIENTED_EDGE('',*,*,#36885,.T.) ;
#48186=ORIENTED_EDGE('',*,*,#36433,.F.) ;
#48187=ORIENTED_EDGE('',*,*,#36886,.F.) ;
#48188=ORIENTED_EDGE('',*,*,#36881,.T.) ;
#48189=ORIENTED_EDGE('',*,*,#36540,.T.) ;
#48190=ORIENTED_EDGE('',*,*,#36887,.F.) ;
#48191=ORIENTED_EDGE('',*,*,#36882,.T.) ;
#48192=ORIENTED_EDGE('',*,*,#36888,.F.) ;
#48193=ORIENTED_EDGE('',*,*,#36883,.T.) ;
#48194=ORIENTED_EDGE('',*,*,#36889,.F.) ;
#48195=ORIENTED_EDGE('',*,*,#36884,.T.) ;
#48196=ORIENTED_EDGE('',*,*,#36624,.T.) ;
#48197=ORIENTED_EDGE('',*,*,#36890,.F.) ;
#48198=ORIENTED_EDGE('',*,*,#36886,.T.) ;
#48199=ORIENTED_EDGE('',*,*,#36887,.T.) ;
#48200=ORIENTED_EDGE('',*,*,#36561,.F.) ;
#48201=ORIENTED_EDGE('',*,*,#36891,.F.) ;
#48202=ORIENTED_EDGE('',*,*,#36638,.F.) ;
#48203=ORIENTED_EDGE('',*,*,#36889,.T.) ;
#48204=ORIENTED_EDGE('',*,*,#36639,.F.) ;
#48205=ORIENTED_EDGE('',*,*,#36892,.F.) ;
#48206=ORIENTED_EDGE('',*,*,#36633,.F.) ;
#48207=ORIENTED_EDGE('',*,*,#36888,.T.) ;
#48208=ORIENTED_EDGE('',*,*,#36635,.F.) ;
#48209=ORIENTED_EDGE('',*,*,#36893,.F.) ;
#48210=ORIENTED_EDGE('',*,*,#36628,.F.) ;
#48211=ORIENTED_EDGE('',*,*,#36890,.T.) ;
#48212=ORIENTED_EDGE('',*,*,#36629,.F.) ;
#48213=ORIENTED_EDGE('',*,*,#36894,.F.) ;
#48214=ORIENTED_EDGE('',*,*,#36405,.F.) ;
#48215=ORIENTED_EDGE('',*,*,#36439,.F.) ;
#48216=ORIENTED_EDGE('',*,*,#36895,.T.) ;
#48217=ORIENTED_EDGE('',*,*,#36410,.F.) ;
#48218=ORIENTED_EDGE('',*,*,#36896,.F.) ;
#48219=ORIENTED_EDGE('',*,*,#36489,.F.) ;
#48220=ORIENTED_EDGE('',*,*,#36440,.F.) ;
#48221=ORIENTED_EDGE('',*,*,#36897,.F.) ;
#48222=ORIENTED_EDGE('',*,*,#36652,.F.) ;
#48223=ORIENTED_EDGE('',*,*,#36491,.F.) ;
#48224=ORIENTED_EDGE('',*,*,#36651,.F.) ;
#48225=ORIENTED_EDGE('',*,*,#36898,.F.) ;
#48226=ORIENTED_EDGE('',*,*,#36649,.F.) ;
#48227=ORIENTED_EDGE('',*,*,#36891,.T.) ;
#48228=ORIENTED_EDGE('',*,*,#36560,.T.) ;
#48229=ORIENTED_EDGE('',*,*,#36899,.F.) ;
#48230=ORIENTED_EDGE('',*,*,#36892,.T.) ;
#48231=ORIENTED_EDGE('',*,*,#36894,.T.) ;
#48232=ORIENTED_EDGE('',*,*,#36893,.T.) ;
#48233=ORIENTED_EDGE('',*,*,#36397,.F.) ;
#48234=ORIENTED_EDGE('',*,*,#36897,.T.) ;
#48235=ORIENTED_EDGE('',*,*,#36896,.T.) ;
#48236=ORIENTED_EDGE('',*,*,#36900,.F.) ;
#48237=ORIENTED_EDGE('',*,*,#36653,.T.) ;
#48238=ORIENTED_EDGE('',*,*,#36901,.F.) ;
#48239=ORIENTED_EDGE('',*,*,#36898,.T.) ;
#48240=ORIENTED_EDGE('',*,*,#36902,.F.) ;
#48241=ORIENTED_EDGE('',*,*,#36899,.T.) ;
#48242=ORIENTED_EDGE('',*,*,#36559,.F.) ;
#48243=ORIENTED_EDGE('',*,*,#36903,.F.) ;
#48244=ORIENTED_EDGE('',*,*,#36634,.F.) ;
#48245=ORIENTED_EDGE('',*,*,#36900,.T.) ;
#48246=ORIENTED_EDGE('',*,*,#36409,.F.) ;
#48247=ORIENTED_EDGE('',*,*,#36904,.F.) ;
#48248=ORIENTED_EDGE('',*,*,#36654,.F.) ;
#48249=ORIENTED_EDGE('',*,*,#36905,.F.) ;
#48250=ORIENTED_EDGE('',*,*,#36655,.F.) ;
#48251=ORIENTED_EDGE('',*,*,#36906,.F.) ;
#48252=ORIENTED_EDGE('',*,*,#36646,.F.) ;
#48253=ORIENTED_EDGE('',*,*,#36902,.T.) ;
#48254=ORIENTED_EDGE('',*,*,#36650,.F.) ;
#48255=ORIENTED_EDGE('',*,*,#36907,.F.) ;
#48256=ORIENTED_EDGE('',*,*,#36640,.F.) ;
#48257=ORIENTED_EDGE('',*,*,#36901,.T.) ;
#48258=ORIENTED_EDGE('',*,*,#36643,.F.) ;
#48259=ORIENTED_EDGE('',*,*,#36908,.F.) ;
#48260=ORIENTED_EDGE('',*,*,#36647,.F.) ;
#48261=ORIENTED_EDGE('',*,*,#36493,.F.) ;
#48262=ORIENTED_EDGE('',*,*,#36648,.F.) ;
#48263=ORIENTED_EDGE('',*,*,#36909,.F.) ;
#48264=ORIENTED_EDGE('',*,*,#36553,.F.) ;
#48265=ORIENTED_EDGE('',*,*,#36395,.T.) ;
#48266=ORIENTED_EDGE('',*,*,#36903,.T.) ;
#48267=ORIENTED_EDGE('',*,*,#36910,.F.) ;
#48268=ORIENTED_EDGE('',*,*,#36406,.T.) ;
#48269=ORIENTED_EDGE('',*,*,#36906,.T.) ;
#48270=ORIENTED_EDGE('',*,*,#36904,.T.) ;
#48271=ORIENTED_EDGE('',*,*,#36393,.F.) ;
#48272=ORIENTED_EDGE('',*,*,#36911,.F.) ;
#48273=ORIENTED_EDGE('',*,*,#36911,.T.) ;
#48274=ORIENTED_EDGE('',*,*,#36392,.F.) ;
#48275=ORIENTED_EDGE('',*,*,#36907,.T.) ;
#48276=ORIENTED_EDGE('',*,*,#36905,.T.) ;
#48277=ORIENTED_EDGE('',*,*,#36912,.F.) ;
#48278=ORIENTED_EDGE('',*,*,#36909,.T.) ;
#48279=ORIENTED_EDGE('',*,*,#36908,.T.) ;
#48280=ORIENTED_EDGE('',*,*,#36913,.F.) ;
#48281=ORIENTED_EDGE('',*,*,#36554,.T.) ;
#48282=ORIENTED_EDGE('',*,*,#36910,.T.) ;
#48283=ORIENTED_EDGE('',*,*,#36558,.F.) ;
#48284=ORIENTED_EDGE('',*,*,#36914,.F.) ;
#48285=ORIENTED_EDGE('',*,*,#36407,.F.) ;
#48286=ORIENTED_EDGE('',*,*,#36912,.T.) ;
#48287=ORIENTED_EDGE('',*,*,#36645,.F.) ;
#48288=ORIENTED_EDGE('',*,*,#36915,.F.) ;
#48289=ORIENTED_EDGE('',*,*,#36641,.F.) ;
#48290=ORIENTED_EDGE('',*,*,#36913,.T.) ;
#48291=ORIENTED_EDGE('',*,*,#36642,.F.) ;
#48292=ORIENTED_EDGE('',*,*,#36916,.F.) ;
#48293=ORIENTED_EDGE('',*,*,#36555,.F.) ;
#48294=ORIENTED_EDGE('',*,*,#36408,.T.) ;
#48295=ORIENTED_EDGE('',*,*,#36914,.T.) ;
#48296=ORIENTED_EDGE('',*,*,#36917,.F.) ;
#48297=ORIENTED_EDGE('',*,*,#36390,.T.) ;
#48298=ORIENTED_EDGE('',*,*,#36916,.T.) ;
#48299=ORIENTED_EDGE('',*,*,#36915,.T.) ;
#48300=ORIENTED_EDGE('',*,*,#36918,.F.) ;
#48301=ORIENTED_EDGE('',*,*,#36556,.T.) ;
#48302=ORIENTED_EDGE('',*,*,#36917,.T.) ;
#48303=ORIENTED_EDGE('',*,*,#36557,.F.) ;
#48304=ORIENTED_EDGE('',*,*,#36918,.T.) ;
#48305=ORIENTED_EDGE('',*,*,#36644,.F.) ;
#48306=ORIENTED_EDGE('',*,*,#36413,.F.) ;
#48307=ORIENTED_EDGE('',*,*,#36919,.T.) ;
#48308=ORIENTED_EDGE('',*,*,#36734,.F.) ;
#48309=ORIENTED_EDGE('',*,*,#36920,.F.) ;
#48310=ORIENTED_EDGE('',*,*,#36739,.F.) ;
#48311=ORIENTED_EDGE('',*,*,#36733,.F.) ;
#48312=ORIENTED_EDGE('',*,*,#36921,.T.) ;
#48313=ORIENTED_EDGE('',*,*,#36740,.F.) ;
#48314=ORIENTED_EDGE('',*,*,#36920,.T.) ;
#48315=ORIENTED_EDGE('',*,*,#36736,.F.) ;
#48316=ORIENTED_EDGE('',*,*,#36922,.T.) ;
#48317=ORIENTED_EDGE('',*,*,#36602,.F.) ;
#48318=ORIENTED_EDGE('',*,*,#36760,.F.) ;
#48319=ORIENTED_EDGE('',*,*,#36923,.F.) ;
#48320=ORIENTED_EDGE('',*,*,#36745,.F.) ;
#48321=ORIENTED_EDGE('',*,*,#36924,.T.) ;
#48322=ORIENTED_EDGE('',*,*,#36773,.F.) ;
#48323=ORIENTED_EDGE('',*,*,#36925,.F.) ;
#48324=ORIENTED_EDGE('',*,*,#36730,.F.) ;
#48325=ORIENTED_EDGE('',*,*,#36926,.T.) ;
#48326=ORIENTED_EDGE('',*,*,#36415,.F.) ;
#48327=ORIENTED_EDGE('',*,*,#36738,.F.) ;
#48328=ORIENTED_EDGE('',*,*,#36927,.F.) ;
#48329=ORIENTED_EDGE('',*,*,#36757,.F.) ;
#48330=ORIENTED_EDGE('',*,*,#36928,.T.) ;
#48331=ORIENTED_EDGE('',*,*,#36731,.F.) ;
#48332=ORIENTED_EDGE('',*,*,#36923,.T.) ;
#48333=ORIENTED_EDGE('',*,*,#36929,.F.) ;
#48334=ORIENTED_EDGE('',*,*,#36925,.T.) ;
#48335=ORIENTED_EDGE('',*,*,#36930,.F.) ;
#48336=ORIENTED_EDGE('',*,*,#36742,.F.) ;
#48337=ORIENTED_EDGE('',*,*,#36931,.T.) ;
#48338=ORIENTED_EDGE('',*,*,#36725,.F.) ;
#48339=ORIENTED_EDGE('',*,*,#36927,.T.) ;
#48340=ORIENTED_EDGE('',*,*,#36775,.F.) ;
#48341=ORIENTED_EDGE('',*,*,#36932,.T.) ;
#48342=ORIENTED_EDGE('',*,*,#36751,.F.) ;
#48343=ORIENTED_EDGE('',*,*,#36933,.F.) ;
#48344=ORIENTED_EDGE('',*,*,#36930,.T.) ;
#48345=ORIENTED_EDGE('',*,*,#36776,.F.) ;
#48346=ORIENTED_EDGE('',*,*,#36934,.F.) ;
#48347=ORIENTED_EDGE('',*,*,#36750,.F.) ;
#48348=ORIENTED_EDGE('',*,*,#36929,.T.) ;
#48349=ORIENTED_EDGE('',*,*,#36749,.F.) ;
#48350=ORIENTED_EDGE('',*,*,#36935,.F.) ;
#48351=ORIENTED_EDGE('',*,*,#36746,.F.) ;
#48352=ORIENTED_EDGE('',*,*,#36771,.F.) ;
#48353=ORIENTED_EDGE('',*,*,#36936,.T.) ;
#48354=ORIENTED_EDGE('',*,*,#36743,.F.) ;
#48355=ORIENTED_EDGE('',*,*,#36937,.F.) ;
#48356=ORIENTED_EDGE('',*,*,#36934,.T.) ;
#48357=ORIENTED_EDGE('',*,*,#36933,.T.) ;
#48358=ORIENTED_EDGE('',*,*,#36938,.F.) ;
#48359=ORIENTED_EDGE('',*,*,#36937,.T.) ;
#48360=ORIENTED_EDGE('',*,*,#36935,.T.) ;
#48361=ORIENTED_EDGE('',*,*,#36939,.F.) ;
#48362=ORIENTED_EDGE('',*,*,#36938,.T.) ;
#48363=ORIENTED_EDGE('',*,*,#36754,.F.) ;
#48364=ORIENTED_EDGE('',*,*,#36940,.F.) ;
#48365=ORIENTED_EDGE('',*,*,#36747,.F.) ;
#48366=ORIENTED_EDGE('',*,*,#36939,.T.) ;
#48367=ORIENTED_EDGE('',*,*,#36748,.F.) ;
#48368=ORIENTED_EDGE('',*,*,#36941,.F.) ;
#48369=ORIENTED_EDGE('',*,*,#36772,.F.) ;
#48370=ORIENTED_EDGE('',*,*,#36941,.T.) ;
#48371=ORIENTED_EDGE('',*,*,#36940,.T.) ;
#48372=ORIENTED_EDGE('',*,*,#36942,.F.) ;
#48373=ORIENTED_EDGE('',*,*,#36753,.F.) ;
#48374=ORIENTED_EDGE('',*,*,#36943,.T.) ;
#48375=ORIENTED_EDGE('',*,*,#36769,.F.) ;
#48376=ORIENTED_EDGE('',*,*,#36942,.T.) ;
#48377=ORIENTED_EDGE('',*,*,#36727,.F.) ;
#48378=ORIENTED_EDGE('',*,*,#36944,.T.) ;
#48379=ORIENTED_EDGE('',*,*,#36755,.F.) ;
#48380=ORIENTED_EDGE('',*,*,#36945,.F.) ;
#48381=ORIENTED_EDGE('',*,*,#36606,.F.) ;
#48382=ORIENTED_EDGE('',*,*,#36946,.T.) ;
#48383=ORIENTED_EDGE('',*,*,#36728,.F.) ;
#48384=ORIENTED_EDGE('',*,*,#36945,.T.) ;
#48385=ORIENTED_EDGE('',*,*,#36759,.F.) ;
#48386=ORIENTED_EDGE('',*,*,#36718,.F.) ;
#48387=ORIENTED_EDGE('',*,*,#36947,.T.) ;
#48388=ORIENTED_EDGE('',*,*,#36719,.F.) ;
#48389=ORIENTED_EDGE('',*,*,#36621,.F.) ;
#48390=ORIENTED_EDGE('',*,*,#36724,.F.) ;
#48391=ORIENTED_EDGE('',*,*,#36948,.T.) ;
#48392=ORIENTED_EDGE('',*,*,#36716,.F.) ;
#48393=ORIENTED_EDGE('',*,*,#36619,.F.) ;
#48394=ORIENTED_EDGE('',*,*,#36703,.F.) ;
#48395=ORIENTED_EDGE('',*,*,#36949,.T.) ;
#48396=ORIENTED_EDGE('',*,*,#36761,.F.) ;
#48397=ORIENTED_EDGE('',*,*,#36950,.F.) ;
#48398=ORIENTED_EDGE('',*,*,#36763,.F.) ;
#48399=ORIENTED_EDGE('',*,*,#36951,.T.) ;
#48400=ORIENTED_EDGE('',*,*,#36709,.F.) ;
#48401=ORIENTED_EDGE('',*,*,#36952,.F.) ;
#48402=ORIENTED_EDGE('',*,*,#36953,.F.) ;
#48403=ORIENTED_EDGE('',*,*,#36764,.F.) ;
#48404=ORIENTED_EDGE('',*,*,#36954,.F.) ;
#48405=ORIENTED_EDGE('',*,*,#36708,.F.) ;
#48406=ORIENTED_EDGE('',*,*,#36950,.T.) ;
#48407=ORIENTED_EDGE('',*,*,#36953,.T.) ;
#48408=ORIENTED_EDGE('',*,*,#36955,.F.) ;
#48409=ORIENTED_EDGE('',*,*,#36721,.F.) ;
#48410=ORIENTED_EDGE('',*,*,#36956,.T.) ;
#48411=ORIENTED_EDGE('',*,*,#36713,.F.) ;
#48412=ORIENTED_EDGE('',*,*,#36623,.F.) ;
#48413=ORIENTED_EDGE('',*,*,#36715,.F.) ;
#48414=ORIENTED_EDGE('',*,*,#36957,.T.) ;
#48415=ORIENTED_EDGE('',*,*,#36722,.F.) ;
#48416=ORIENTED_EDGE('',*,*,#36617,.F.) ;
#48417=ORIENTED_EDGE('',*,*,#36954,.T.) ;
#48418=ORIENTED_EDGE('',*,*,#36952,.T.) ;
#48419=ORIENTED_EDGE('',*,*,#36958,.F.) ;
#48420=ORIENTED_EDGE('',*,*,#36955,.T.) ;
#48421=ORIENTED_EDGE('',*,*,#36707,.F.) ;
#48422=ORIENTED_EDGE('',*,*,#36959,.F.) ;
#48423=ORIENTED_EDGE('',*,*,#36704,.F.) ;
#48424=ORIENTED_EDGE('',*,*,#36767,.F.) ;
#48425=ORIENTED_EDGE('',*,*,#36960,.T.) ;
#48426=ORIENTED_EDGE('',*,*,#36701,.F.) ;
#48427=ORIENTED_EDGE('',*,*,#36961,.F.) ;
#48428=ORIENTED_EDGE('',*,*,#36711,.F.) ;
#48429=ORIENTED_EDGE('',*,*,#36962,.T.) ;
#48430=ORIENTED_EDGE('',*,*,#36765,.F.) ;
#48431=ORIENTED_EDGE('',*,*,#36963,.F.) ;
#48432=ORIENTED_EDGE('',*,*,#36958,.T.) ;
#48433=ORIENTED_EDGE('',*,*,#36712,.F.) ;
#48434=ORIENTED_EDGE('',*,*,#36964,.F.) ;
#48435=ORIENTED_EDGE('',*,*,#36705,.F.) ;
#48436=ORIENTED_EDGE('',*,*,#36961,.T.) ;
#48437=ORIENTED_EDGE('',*,*,#36959,.T.) ;
#48438=ORIENTED_EDGE('',*,*,#36965,.F.) ;
#48439=ORIENTED_EDGE('',*,*,#36964,.T.) ;
#48440=ORIENTED_EDGE('',*,*,#36963,.T.) ;
#48441=ORIENTED_EDGE('',*,*,#36966,.F.) ;
#48442=ORIENTED_EDGE('',*,*,#36965,.T.) ;
#48443=ORIENTED_EDGE('',*,*,#36706,.F.) ;
#48444=ORIENTED_EDGE('',*,*,#36966,.T.) ;
#48445=ORIENTED_EDGE('',*,*,#36768,.F.) ;
#48446=ORIENTED_EDGE('',*,*,#36450,.F.) ;
#48447=ORIENTED_EDGE('',*,*,#36426,.F.) ;
#48448=ORIENTED_EDGE('',*,*,#36967,.F.) ;
#48449=ORIENTED_EDGE('',*,*,#36432,.F.) ;
#48450=ORIENTED_EDGE('',*,*,#36688,.F.) ;
#48451=ORIENTED_EDGE('',*,*,#36968,.T.) ;
#48452=ORIENTED_EDGE('',*,*,#36427,.F.) ;
#48453=ORIENTED_EDGE('',*,*,#36969,.F.) ;
#48454=ORIENTED_EDGE('',*,*,#36969,.T.) ;
#48455=ORIENTED_EDGE('',*,*,#36967,.T.) ;
#48456=ORIENTED_EDGE('',*,*,#36970,.F.) ;
#48457=ORIENTED_EDGE('',*,*,#36449,.F.) ;
#48458=ORIENTED_EDGE('',*,*,#36422,.F.) ;
#48459=ORIENTED_EDGE('',*,*,#36971,.F.) ;
#48460=ORIENTED_EDGE('',*,*,#36424,.F.) ;
#48461=ORIENTED_EDGE('',*,*,#36970,.T.) ;
#48462=ORIENTED_EDGE('',*,*,#36425,.F.) ;
#48463=ORIENTED_EDGE('',*,*,#36972,.F.) ;
#48464=ORIENTED_EDGE('',*,*,#36689,.F.) ;
#48465=ORIENTED_EDGE('',*,*,#36972,.T.) ;
#48466=ORIENTED_EDGE('',*,*,#36971,.T.) ;
#48467=ORIENTED_EDGE('',*,*,#36973,.F.) ;
#48468=ORIENTED_EDGE('',*,*,#36421,.F.) ;
#48469=ORIENTED_EDGE('',*,*,#36974,.T.) ;
#48470=ORIENTED_EDGE('',*,*,#36686,.F.) ;
#48471=ORIENTED_EDGE('',*,*,#36973,.T.) ;
#48472=ORIENTED_EDGE('',*,*,#36525,.F.) ;
#48473=ORIENTED_EDGE('',*,*,#36377,.T.) ;
#48474=ORIENTED_EDGE('',*,*,#36975,.T.) ;
#48475=ORIENTED_EDGE('',*,*,#36697,.F.) ;
#48476=ORIENTED_EDGE('',*,*,#36976,.F.) ;
#48477=ORIENTED_EDGE('',*,*,#36503,.F.) ;
#48478=ORIENTED_EDGE('',*,*,#36526,.F.) ;
#48479=ORIENTED_EDGE('',*,*,#36977,.F.) ;
#48480=ORIENTED_EDGE('',*,*,#36523,.F.) ;
#48481=ORIENTED_EDGE('',*,*,#36977,.T.) ;
#48482=ORIENTED_EDGE('',*,*,#36976,.T.) ;
#48483=ORIENTED_EDGE('',*,*,#36978,.F.) ;
#48484=ORIENTED_EDGE('',*,*,#36978,.T.) ;
#48485=ORIENTED_EDGE('',*,*,#36700,.F.) ;
#48486=ORIENTED_EDGE('',*,*,#36979,.F.) ;
#48487=ORIENTED_EDGE('',*,*,#36521,.F.) ;
#48488=ORIENTED_EDGE('',*,*,#36505,.F.) ;
#48489=ORIENTED_EDGE('',*,*,#36522,.F.) ;
#48490=ORIENTED_EDGE('',*,*,#36980,.F.) ;
#48491=ORIENTED_EDGE('',*,*,#36519,.F.) ;
#48492=ORIENTED_EDGE('',*,*,#36980,.T.) ;
#48493=ORIENTED_EDGE('',*,*,#36979,.T.) ;
#48494=ORIENTED_EDGE('',*,*,#36981,.F.) ;
#48495=ORIENTED_EDGE('',*,*,#36699,.F.) ;
#48496=ORIENTED_EDGE('',*,*,#36381,.T.) ;
#48497=ORIENTED_EDGE('',*,*,#36982,.T.) ;
#48498=ORIENTED_EDGE('',*,*,#36520,.F.) ;
#48499=ORIENTED_EDGE('',*,*,#36981,.T.) ;
#48500=ORIENTED_EDGE('',*,*,#36600,.F.) ;
#48501=ORIENTED_EDGE('',*,*,#36983,.T.) ;
#48502=ORIENTED_EDGE('',*,*,#36411,.F.) ;
#48503=ORIENTED_EDGE('',*,*,#36984,.T.) ;
#48504=ORIENTED_EDGE('',*,*,#36470,.F.) ;
#48505=ORIENTED_EDGE('',*,*,#36572,.F.) ;
#48506=ORIENTED_EDGE('',*,*,#36482,.F.) ;
#48507=ORIENTED_EDGE('',*,*,#36506,.F.) ;
#48508=ORIENTED_EDGE('',*,*,#36472,.F.) ;
#48509=ORIENTED_EDGE('',*,*,#36507,.F.) ;
#48510=ORIENTED_EDGE('',*,*,#36480,.F.) ;
#48511=ORIENTED_EDGE('',*,*,#36508,.F.) ;
#48512=ORIENTED_EDGE('',*,*,#36474,.F.) ;
#48513=ORIENTED_EDGE('',*,*,#36509,.F.) ;
#48514=ORIENTED_EDGE('',*,*,#36478,.F.) ;
#48515=ORIENTED_EDGE('',*,*,#36512,.F.) ;
#48516=ORIENTED_EDGE('',*,*,#36467,.F.) ;
#48517=ORIENTED_EDGE('',*,*,#36442,.F.) ;
#48518=ORIENTED_EDGE('',*,*,#36485,.F.) ;
#48519=ORIENTED_EDGE('',*,*,#36565,.F.) ;
#48520=ORIENTED_EDGE('',*,*,#36785,.F.) ;
#48521=ORIENTED_EDGE('',*,*,#36985,.T.) ;
#48522=ORIENTED_EDGE('',*,*,#36444,.F.) ;
#48523=ORIENTED_EDGE('',*,*,#36466,.F.) ;
#48524=ORIENTED_EDGE('',*,*,#36780,.F.) ;
#48525=ORIENTED_EDGE('',*,*,#36986,.T.) ;
#48526=ORIENTED_EDGE('',*,*,#36445,.F.) ;
#48527=ORIENTED_EDGE('',*,*,#36987,.T.) ;
#48528=ORIENTED_EDGE('',*,*,#36446,.F.) ;
#48529=ORIENTED_EDGE('',*,*,#36988,.T.) ;
#48530=ORIENTED_EDGE('',*,*,#36777,.F.) ;
#48531=ORIENTED_EDGE('',*,*,#36486,.F.) ;
#48532=ORIENTED_EDGE('',*,*,#36825,.F.) ;
#48533=ORIENTED_EDGE('',*,*,#36831,.F.) ;
#48534=ORIENTED_EDGE('',*,*,#36830,.F.) ;
#48535=ORIENTED_EDGE('',*,*,#36989,.F.) ;
#48536=ORIENTED_EDGE('',*,*,#36826,.F.) ;
#48537=ORIENTED_EDGE('',*,*,#36919,.F.) ;
#48538=ORIENTED_EDGE('',*,*,#36412,.F.) ;
#48539=ORIENTED_EDGE('',*,*,#36990,.F.) ;
#48540=ORIENTED_EDGE('',*,*,#36594,.F.) ;
#48541=ORIENTED_EDGE('',*,*,#36989,.T.) ;
#48542=ORIENTED_EDGE('',*,*,#36603,.F.) ;
#48543=ORIENTED_EDGE('',*,*,#36922,.F.) ;
#48544=ORIENTED_EDGE('',*,*,#36735,.F.) ;
#48545=ORIENTED_EDGE('',*,*,#36990,.T.) ;
#48546=ORIENTED_EDGE('',*,*,#36983,.F.) ;
#48547=ORIENTED_EDGE('',*,*,#36991,.F.) ;
#48548=ORIENTED_EDGE('',*,*,#36991,.T.) ;
#48549=ORIENTED_EDGE('',*,*,#36599,.F.) ;
#48550=ORIENTED_EDGE('',*,*,#36992,.F.) ;
#48551=ORIENTED_EDGE('',*,*,#36595,.F.) ;
#48552=ORIENTED_EDGE('',*,*,#36834,.F.) ;
#48553=ORIENTED_EDGE('',*,*,#36828,.F.) ;
#48554=ORIENTED_EDGE('',*,*,#36827,.F.) ;
#48555=ORIENTED_EDGE('',*,*,#36992,.T.) ;
#48556=ORIENTED_EDGE('',*,*,#36835,.F.) ;
#48557=ORIENTED_EDGE('',*,*,#36847,.F.) ;
#48558=ORIENTED_EDGE('',*,*,#36837,.F.) ;
#48559=ORIENTED_EDGE('',*,*,#36836,.F.) ;
#48560=ORIENTED_EDGE('',*,*,#36993,.F.) ;
#48561=ORIENTED_EDGE('',*,*,#36848,.F.) ;
#48562=ORIENTED_EDGE('',*,*,#36993,.T.) ;
#48563=ORIENTED_EDGE('',*,*,#36601,.F.) ;
#48564=ORIENTED_EDGE('',*,*,#36994,.F.) ;
#48565=ORIENTED_EDGE('',*,*,#36591,.F.) ;
#48566=ORIENTED_EDGE('',*,*,#36994,.T.) ;
#48567=ORIENTED_EDGE('',*,*,#36984,.F.) ;
#48568=ORIENTED_EDGE('',*,*,#36995,.F.) ;
#48569=ORIENTED_EDGE('',*,*,#36946,.F.) ;
#48570=ORIENTED_EDGE('',*,*,#36605,.F.) ;
#48571=ORIENTED_EDGE('',*,*,#36996,.F.) ;
#48572=ORIENTED_EDGE('',*,*,#36592,.F.) ;
#48573=ORIENTED_EDGE('',*,*,#36995,.T.) ;
#48574=ORIENTED_EDGE('',*,*,#36416,.F.) ;
#48575=ORIENTED_EDGE('',*,*,#36926,.F.) ;
#48576=ORIENTED_EDGE('',*,*,#36729,.F.) ;
#48577=ORIENTED_EDGE('',*,*,#36996,.T.) ;
#48578=ORIENTED_EDGE('',*,*,#36833,.F.) ;
#48579=ORIENTED_EDGE('',*,*,#36832,.F.) ;
#48580=ORIENTED_EDGE('',*,*,#36845,.F.) ;
#48581=ORIENTED_EDGE('',*,*,#36844,.F.) ;
#48582=ORIENTED_EDGE('',*,*,#36420,.F.) ;
#48583=ORIENTED_EDGE('',*,*,#36997,.T.) ;
#48584=ORIENTED_EDGE('',*,*,#36690,.F.) ;
#48585=ORIENTED_EDGE('',*,*,#36998,.F.) ;
#48586=ORIENTED_EDGE('',*,*,#36974,.F.) ;
#48587=ORIENTED_EDGE('',*,*,#36998,.T.) ;
#48588=ORIENTED_EDGE('',*,*,#36696,.F.) ;
#48589=ORIENTED_EDGE('',*,*,#36999,.F.) ;
#48590=ORIENTED_EDGE('',*,*,#36687,.F.) ;
#48591=ORIENTED_EDGE('',*,*,#36999,.T.) ;
#48592=ORIENTED_EDGE('',*,*,#36695,.F.) ;
#48593=ORIENTED_EDGE('',*,*,#37000,.F.) ;
#48594=ORIENTED_EDGE('',*,*,#37001,.F.) ;
#48595=ORIENTED_EDGE('',*,*,#37002,.F.) ;
#48596=ORIENTED_EDGE('',*,*,#37003,.F.) ;
#48597=ORIENTED_EDGE('',*,*,#36428,.F.) ;
#48598=ORIENTED_EDGE('',*,*,#36968,.F.) ;
#48599=ORIENTED_EDGE('',*,*,#36451,.F.) ;
#48600=ORIENTED_EDGE('',*,*,#36430,.F.) ;
#48601=ORIENTED_EDGE('',*,*,#37004,.F.) ;
#48602=ORIENTED_EDGE('',*,*,#36528,.F.) ;
#48603=ORIENTED_EDGE('',*,*,#36429,.F.) ;
#48604=ORIENTED_EDGE('',*,*,#37003,.T.) ;
#48605=ORIENTED_EDGE('',*,*,#37002,.T.) ;
#48606=ORIENTED_EDGE('',*,*,#37001,.T.) ;
#48607=ORIENTED_EDGE('',*,*,#37000,.T.) ;
#48608=ORIENTED_EDGE('',*,*,#37005,.F.) ;
#48609=ORIENTED_EDGE('',*,*,#36529,.F.) ;
#48610=ORIENTED_EDGE('',*,*,#37004,.T.) ;
#48611=ORIENTED_EDGE('',*,*,#36380,.F.) ;
#48612=ORIENTED_EDGE('',*,*,#37006,.T.) ;
#48613=ORIENTED_EDGE('',*,*,#36516,.F.) ;
#48614=ORIENTED_EDGE('',*,*,#36982,.F.) ;
#48615=ORIENTED_EDGE('',*,*,#37005,.T.) ;
#48616=ORIENTED_EDGE('',*,*,#36694,.F.) ;
#48617=ORIENTED_EDGE('',*,*,#37007,.F.) ;
#48618=ORIENTED_EDGE('',*,*,#36530,.F.) ;
#48619=ORIENTED_EDGE('',*,*,#36501,.F.) ;
#48620=ORIENTED_EDGE('',*,*,#36532,.F.) ;
#48621=ORIENTED_EDGE('',*,*,#37008,.F.) ;
#48622=ORIENTED_EDGE('',*,*,#36527,.F.) ;
#48623=ORIENTED_EDGE('',*,*,#36382,.T.) ;
#48624=ORIENTED_EDGE('',*,*,#36698,.F.) ;
#48625=ORIENTED_EDGE('',*,*,#37009,.F.) ;
#48626=ORIENTED_EDGE('',*,*,#36692,.F.) ;
#48627=ORIENTED_EDGE('',*,*,#36531,.F.) ;
#48628=ORIENTED_EDGE('',*,*,#37007,.T.) ;
#48629=ORIENTED_EDGE('',*,*,#37010,.F.) ;
#48630=ORIENTED_EDGE('',*,*,#37011,.F.) ;
#48631=ORIENTED_EDGE('',*,*,#37012,.F.) ;
#48632=ORIENTED_EDGE('',*,*,#36375,.F.) ;
#48633=ORIENTED_EDGE('',*,*,#36374,.F.) ;
#48634=ORIENTED_EDGE('',*,*,#36524,.F.) ;
#48635=ORIENTED_EDGE('',*,*,#37008,.T.) ;
#48636=ORIENTED_EDGE('',*,*,#36376,.F.) ;
#48637=ORIENTED_EDGE('',*,*,#37012,.T.) ;
#48638=ORIENTED_EDGE('',*,*,#37011,.T.) ;
#48639=ORIENTED_EDGE('',*,*,#37010,.T.) ;
#48640=ORIENTED_EDGE('',*,*,#36693,.F.) ;
#48641=ORIENTED_EDGE('',*,*,#37009,.T.) ;
#48642=ORIENTED_EDGE('',*,*,#36975,.F.) ;
#48643=ORIENTED_EDGE('',*,*,#37013,.F.) ;
#48644=ORIENTED_EDGE('',*,*,#36438,.F.) ;
#48645=ORIENTED_EDGE('',*,*,#36488,.F.) ;
#48646=ORIENTED_EDGE('',*,*,#36779,.F.) ;
#48647=ORIENTED_EDGE('',*,*,#36895,.F.) ;
#48648=ORIENTED_EDGE('',*,*,#37013,.T.) ;
#48649=ORIENTED_EDGE('',*,*,#37014,.F.) ;
#48650=ORIENTED_EDGE('',*,*,#36400,.F.) ;
#48651=ORIENTED_EDGE('',*,*,#37014,.T.) ;
#48652=ORIENTED_EDGE('',*,*,#36778,.F.) ;
#48653=ORIENTED_EDGE('',*,*,#37015,.F.) ;
#48654=ORIENTED_EDGE('',*,*,#36782,.F.) ;
#48655=ORIENTED_EDGE('',*,*,#36988,.F.) ;
#48656=ORIENTED_EDGE('',*,*,#36986,.F.) ;
#48657=ORIENTED_EDGE('',*,*,#37015,.T.) ;
#48658=ORIENTED_EDGE('',*,*,#37016,.T.) ;
#48659=ORIENTED_EDGE('',*,*,#36921,.F.) ;
#48660=ORIENTED_EDGE('',*,*,#37017,.F.) ;
#48661=ORIENTED_EDGE('',*,*,#36924,.F.) ;
#48662=ORIENTED_EDGE('',*,*,#37016,.F.) ;
#48663=ORIENTED_EDGE('',*,*,#36744,.F.) ;
#48664=ORIENTED_EDGE('',*,*,#37018,.F.) ;
#48665=ORIENTED_EDGE('',*,*,#36741,.F.) ;
#48666=ORIENTED_EDGE('',*,*,#37017,.T.) ;
#48667=ORIENTED_EDGE('',*,*,#36732,.F.) ;
#48668=ORIENTED_EDGE('',*,*,#37019,.F.) ;
#48669=ORIENTED_EDGE('',*,*,#36774,.F.) ;
#48670=ORIENTED_EDGE('',*,*,#37018,.T.) ;
#48671=ORIENTED_EDGE('',*,*,#36936,.F.) ;
#48672=ORIENTED_EDGE('',*,*,#37020,.F.) ;
#48673=ORIENTED_EDGE('',*,*,#36931,.F.) ;
#48674=ORIENTED_EDGE('',*,*,#37019,.T.) ;
#48675=ORIENTED_EDGE('',*,*,#36928,.F.) ;
#48676=ORIENTED_EDGE('',*,*,#37021,.F.) ;
#48677=ORIENTED_EDGE('',*,*,#36932,.F.) ;
#48678=ORIENTED_EDGE('',*,*,#37020,.T.) ;
#48679=ORIENTED_EDGE('',*,*,#36770,.F.) ;
#48680=ORIENTED_EDGE('',*,*,#37022,.F.) ;
#48681=ORIENTED_EDGE('',*,*,#36726,.F.) ;
#48682=ORIENTED_EDGE('',*,*,#37021,.T.) ;
#48683=ORIENTED_EDGE('',*,*,#36756,.F.) ;
#48684=ORIENTED_EDGE('',*,*,#37023,.F.) ;
#48685=ORIENTED_EDGE('',*,*,#36752,.F.) ;
#48686=ORIENTED_EDGE('',*,*,#37022,.T.) ;
#48687=ORIENTED_EDGE('',*,*,#36943,.F.) ;
#48688=ORIENTED_EDGE('',*,*,#37023,.T.) ;
#48689=ORIENTED_EDGE('',*,*,#36944,.F.) ;
#48690=ORIENTED_EDGE('',*,*,#37024,.T.) ;
#48691=ORIENTED_EDGE('',*,*,#36947,.F.) ;
#48692=ORIENTED_EDGE('',*,*,#37025,.F.) ;
#48693=ORIENTED_EDGE('',*,*,#36949,.F.) ;
#48694=ORIENTED_EDGE('',*,*,#37024,.F.) ;
#48695=ORIENTED_EDGE('',*,*,#36702,.F.) ;
#48696=ORIENTED_EDGE('',*,*,#37026,.F.) ;
#48697=ORIENTED_EDGE('',*,*,#36720,.F.) ;
#48698=ORIENTED_EDGE('',*,*,#37025,.T.) ;
#48699=ORIENTED_EDGE('',*,*,#36717,.F.) ;
#48700=ORIENTED_EDGE('',*,*,#37027,.F.) ;
#48701=ORIENTED_EDGE('',*,*,#36762,.F.) ;
#48702=ORIENTED_EDGE('',*,*,#37026,.T.) ;
#48703=ORIENTED_EDGE('',*,*,#36960,.F.) ;
#48704=ORIENTED_EDGE('',*,*,#37028,.F.) ;
#48705=ORIENTED_EDGE('',*,*,#36956,.F.) ;
#48706=ORIENTED_EDGE('',*,*,#37027,.T.) ;
#48707=ORIENTED_EDGE('',*,*,#36948,.F.) ;
#48708=ORIENTED_EDGE('',*,*,#37029,.F.) ;
#48709=ORIENTED_EDGE('',*,*,#36951,.F.) ;
#48710=ORIENTED_EDGE('',*,*,#37028,.T.) ;
#48711=ORIENTED_EDGE('',*,*,#36766,.F.) ;
#48712=ORIENTED_EDGE('',*,*,#37030,.F.) ;
#48713=ORIENTED_EDGE('',*,*,#36714,.F.) ;
#48714=ORIENTED_EDGE('',*,*,#37029,.T.) ;
#48715=ORIENTED_EDGE('',*,*,#36723,.F.) ;
#48716=ORIENTED_EDGE('',*,*,#37031,.F.) ;
#48717=ORIENTED_EDGE('',*,*,#36710,.F.) ;
#48718=ORIENTED_EDGE('',*,*,#37030,.T.) ;
#48719=ORIENTED_EDGE('',*,*,#36962,.F.) ;
#48720=ORIENTED_EDGE('',*,*,#37031,.T.) ;
#48721=ORIENTED_EDGE('',*,*,#36957,.F.) ;
#48722=ORIENTED_EDGE('',*,*,#36464,.F.) ;
#48723=ORIENTED_EDGE('',*,*,#36434,.F.) ;
#48724=ORIENTED_EDGE('',*,*,#37032,.F.) ;
#48725=ORIENTED_EDGE('',*,*,#36783,.F.) ;
#48726=ORIENTED_EDGE('',*,*,#37032,.T.) ;
#48727=ORIENTED_EDGE('',*,*,#36885,.F.) ;
#48728=ORIENTED_EDGE('',*,*,#36402,.F.) ;
#48729=ORIENTED_EDGE('',*,*,#37033,.F.) ;
#48730=ORIENTED_EDGE('',*,*,#37033,.T.) ;
#48731=ORIENTED_EDGE('',*,*,#36781,.F.) ;
#48732=ORIENTED_EDGE('',*,*,#37034,.F.) ;
#48733=ORIENTED_EDGE('',*,*,#36784,.F.) ;
#48734=ORIENTED_EDGE('',*,*,#36987,.F.) ;
#48735=ORIENTED_EDGE('',*,*,#36985,.F.) ;
#48736=ORIENTED_EDGE('',*,*,#37034,.T.) ;
#48737=ORIENTED_EDGE('',*,*,#36518,.F.) ;
#48738=ORIENTED_EDGE('',*,*,#37035,.F.) ;
#48739=ORIENTED_EDGE('',*,*,#36513,.F.) ;
#48740=ORIENTED_EDGE('',*,*,#36476,.F.) ;
#48741=ORIENTED_EDGE('',*,*,#36517,.F.) ;
#48742=ORIENTED_EDGE('',*,*,#37006,.F.) ;
#48743=ORIENTED_EDGE('',*,*,#36379,.F.) ;
#48744=ORIENTED_EDGE('',*,*,#37036,.F.) ;
#48745=ORIENTED_EDGE('',*,*,#36514,.F.) ;
#48746=ORIENTED_EDGE('',*,*,#37035,.T.) ;
#48747=ORIENTED_EDGE('',*,*,#37036,.T.) ;
#48748=ORIENTED_EDGE('',*,*,#36691,.F.) ;
#48749=ORIENTED_EDGE('',*,*,#37037,.F.) ;
#48750=ORIENTED_EDGE('',*,*,#36515,.F.) ;
#48751=ORIENTED_EDGE('',*,*,#36997,.F.) ;
#48752=ORIENTED_EDGE('',*,*,#36419,.F.) ;
#48753=ORIENTED_EDGE('',*,*,#37038,.F.) ;
#48754=ORIENTED_EDGE('',*,*,#36510,.F.) ;
#48755=ORIENTED_EDGE('',*,*,#37037,.T.) ;
#48756=ORIENTED_EDGE('',*,*,#36448,.F.) ;
#48757=ORIENTED_EDGE('',*,*,#36511,.F.) ;
#48758=ORIENTED_EDGE('',*,*,#37038,.T.) ;
#48759=ORIENTED_EDGE('',*,*,#36418,.F.) ;
#48760=ORIENTED_EDGE('',*,*,#37039,.T.) ;
#48761=ORIENTED_EDGE('',*,*,#37040,.T.) ;
#48762=ORIENTED_EDGE('',*,*,#37041,.T.) ;
#48763=ORIENTED_EDGE('',*,*,#37042,.F.) ;
#48764=ORIENTED_EDGE('',*,*,#37043,.F.) ;
#48765=ORIENTED_EDGE('',*,*,#37044,.T.) ;
#48766=ORIENTED_EDGE('',*,*,#37045,.T.) ;
#48767=ORIENTED_EDGE('',*,*,#37046,.F.) ;
#48768=ORIENTED_EDGE('',*,*,#37047,.F.) ;
#48769=ORIENTED_EDGE('',*,*,#37048,.F.) ;
#48770=ORIENTED_EDGE('',*,*,#37049,.F.) ;
#48771=ORIENTED_EDGE('',*,*,#37050,.T.) ;
#48772=ORIENTED_EDGE('',*,*,#37051,.F.) ;
#48773=ORIENTED_EDGE('',*,*,#37050,.F.) ;
#48774=ORIENTED_EDGE('',*,*,#37052,.F.) ;
#48775=ORIENTED_EDGE('',*,*,#37053,.T.) ;
#48776=ORIENTED_EDGE('',*,*,#37054,.F.) ;
#48777=ORIENTED_EDGE('',*,*,#37053,.F.) ;
#48778=ORIENTED_EDGE('',*,*,#37055,.F.) ;
#48779=ORIENTED_EDGE('',*,*,#37056,.F.) ;
#48780=ORIENTED_EDGE('',*,*,#37057,.T.) ;
#48781=ORIENTED_EDGE('',*,*,#37058,.T.) ;
#48782=ORIENTED_EDGE('',*,*,#37059,.F.) ;
#48783=ORIENTED_EDGE('',*,*,#37060,.F.) ;
#48784=ORIENTED_EDGE('',*,*,#37061,.F.) ;
#48785=ORIENTED_EDGE('',*,*,#37062,.T.) ;
#48786=ORIENTED_EDGE('',*,*,#37063,.F.) ;
#48787=ORIENTED_EDGE('',*,*,#37064,.F.) ;
#48788=ORIENTED_EDGE('',*,*,#37065,.T.) ;
#48789=ORIENTED_EDGE('',*,*,#37066,.F.) ;
#48790=ORIENTED_EDGE('',*,*,#37067,.T.) ;
#48791=ORIENTED_EDGE('',*,*,#37051,.T.) ;
#48792=ORIENTED_EDGE('',*,*,#37068,.T.) ;
#48793=ORIENTED_EDGE('',*,*,#37052,.T.) ;
#48794=ORIENTED_EDGE('',*,*,#37068,.F.) ;
#48795=ORIENTED_EDGE('',*,*,#37064,.T.) ;
#48796=ORIENTED_EDGE('',*,*,#37069,.T.) ;
#48797=ORIENTED_EDGE('',*,*,#37070,.T.) ;
#48798=ORIENTED_EDGE('',*,*,#37061,.T.) ;
#48799=ORIENTED_EDGE('',*,*,#37071,.F.) ;
#48800=ORIENTED_EDGE('',*,*,#37072,.T.) ;
#48801=ORIENTED_EDGE('',*,*,#37073,.F.) ;
#48802=ORIENTED_EDGE('',*,*,#37059,.T.) ;
#48803=ORIENTED_EDGE('',*,*,#37074,.T.) ;
#48804=ORIENTED_EDGE('',*,*,#37075,.T.) ;
#48805=ORIENTED_EDGE('',*,*,#37076,.T.) ;
#48806=ORIENTED_EDGE('',*,*,#37077,.T.) ;
#48807=ORIENTED_EDGE('',*,*,#37078,.T.) ;
#48808=ORIENTED_EDGE('',*,*,#37079,.T.) ;
#48809=ORIENTED_EDGE('',*,*,#37080,.T.) ;
#48810=ORIENTED_EDGE('',*,*,#37081,.T.) ;
#48811=ORIENTED_EDGE('',*,*,#37082,.T.) ;
#48812=ORIENTED_EDGE('',*,*,#37083,.T.) ;
#48813=ORIENTED_EDGE('',*,*,#37084,.T.) ;
#48814=ORIENTED_EDGE('',*,*,#37085,.T.) ;
#48815=ORIENTED_EDGE('',*,*,#37086,.T.) ;
#48816=ORIENTED_EDGE('',*,*,#37087,.T.) ;
#48817=ORIENTED_EDGE('',*,*,#37088,.T.) ;
#48818=ORIENTED_EDGE('',*,*,#37089,.T.) ;
#48819=ORIENTED_EDGE('',*,*,#37090,.T.) ;
#48820=ORIENTED_EDGE('',*,*,#37091,.T.) ;
#48821=ORIENTED_EDGE('',*,*,#37092,.T.) ;
#48822=ORIENTED_EDGE('',*,*,#37093,.T.) ;
#48823=ORIENTED_EDGE('',*,*,#37094,.T.) ;
#48824=ORIENTED_EDGE('',*,*,#37095,.T.) ;
#48825=ORIENTED_EDGE('',*,*,#37096,.T.) ;
#48826=ORIENTED_EDGE('',*,*,#37097,.T.) ;
#48827=ORIENTED_EDGE('',*,*,#37098,.T.) ;
#48828=ORIENTED_EDGE('',*,*,#37099,.T.) ;
#48829=ORIENTED_EDGE('',*,*,#37100,.T.) ;
#48830=ORIENTED_EDGE('',*,*,#37101,.T.) ;
#48831=ORIENTED_EDGE('',*,*,#37102,.F.) ;
#48832=ORIENTED_EDGE('',*,*,#37103,.T.) ;
#48833=ORIENTED_EDGE('',*,*,#37104,.T.) ;
#48834=ORIENTED_EDGE('',*,*,#37105,.T.) ;
#48835=ORIENTED_EDGE('',*,*,#37106,.F.) ;
#48836=ORIENTED_EDGE('',*,*,#37107,.T.) ;
#48837=ORIENTED_EDGE('',*,*,#37108,.T.) ;
#48838=ORIENTED_EDGE('',*,*,#37109,.T.) ;
#48839=ORIENTED_EDGE('',*,*,#37110,.T.) ;
#48840=ORIENTED_EDGE('',*,*,#37111,.T.) ;
#48841=ORIENTED_EDGE('',*,*,#37112,.F.) ;
#48842=ORIENTED_EDGE('',*,*,#37113,.T.) ;
#48843=ORIENTED_EDGE('',*,*,#37082,.F.) ;
#48844=ORIENTED_EDGE('',*,*,#37114,.T.) ;
#48845=ORIENTED_EDGE('',*,*,#37088,.F.) ;
#48846=ORIENTED_EDGE('',*,*,#37115,.T.) ;
#48847=ORIENTED_EDGE('',*,*,#37096,.F.) ;
#48848=ORIENTED_EDGE('',*,*,#37116,.T.) ;
#48849=ORIENTED_EDGE('',*,*,#37117,.F.) ;
#48850=ORIENTED_EDGE('',*,*,#37118,.T.) ;
#48851=ORIENTED_EDGE('',*,*,#37119,.F.) ;
#48852=ORIENTED_EDGE('',*,*,#37120,.T.) ;
#48853=ORIENTED_EDGE('',*,*,#37121,.T.) ;
#48854=ORIENTED_EDGE('',*,*,#37122,.T.) ;
#48855=ORIENTED_EDGE('',*,*,#37123,.F.) ;
#48856=ORIENTED_EDGE('',*,*,#37124,.T.) ;
#48857=ORIENTED_EDGE('',*,*,#37125,.T.) ;
#48858=ORIENTED_EDGE('',*,*,#37126,.T.) ;
#48859=ORIENTED_EDGE('',*,*,#37127,.F.) ;
#48860=ORIENTED_EDGE('',*,*,#37128,.T.) ;
#48861=ORIENTED_EDGE('',*,*,#37100,.F.) ;
#48862=ORIENTED_EDGE('',*,*,#37129,.T.) ;
#48863=ORIENTED_EDGE('',*,*,#37130,.T.) ;
#48864=ORIENTED_EDGE('',*,*,#37131,.T.) ;
#48865=ORIENTED_EDGE('',*,*,#37108,.F.) ;
#48866=ORIENTED_EDGE('',*,*,#37132,.T.) ;
#48867=ORIENTED_EDGE('',*,*,#37133,.F.) ;
#48868=ORIENTED_EDGE('',*,*,#37134,.F.) ;
#48869=ORIENTED_EDGE('',*,*,#37135,.T.) ;
#48870=ORIENTED_EDGE('',*,*,#37136,.F.) ;
#48871=ORIENTED_EDGE('',*,*,#37137,.T.) ;
#48872=ORIENTED_EDGE('',*,*,#37138,.F.) ;
#48873=ORIENTED_EDGE('',*,*,#37139,.T.) ;
#48874=ORIENTED_EDGE('',*,*,#37140,.T.) ;
#48875=ORIENTED_EDGE('',*,*,#37141,.T.) ;
#48876=ORIENTED_EDGE('',*,*,#37142,.T.) ;
#48877=ORIENTED_EDGE('',*,*,#37143,.T.) ;
#48878=ORIENTED_EDGE('',*,*,#37144,.T.) ;
#48879=ORIENTED_EDGE('',*,*,#37145,.T.) ;
#48880=ORIENTED_EDGE('',*,*,#37146,.T.) ;
#48881=ORIENTED_EDGE('',*,*,#37147,.T.) ;
#48882=ORIENTED_EDGE('',*,*,#37148,.T.) ;
#48883=ORIENTED_EDGE('',*,*,#37149,.T.) ;
#48884=ORIENTED_EDGE('',*,*,#37150,.T.) ;
#48885=ORIENTED_EDGE('',*,*,#37106,.T.) ;
#48886=ORIENTED_EDGE('',*,*,#37151,.T.) ;
#48887=ORIENTED_EDGE('',*,*,#37152,.T.) ;
#48888=ORIENTED_EDGE('',*,*,#37153,.T.) ;
#48889=ORIENTED_EDGE('',*,*,#37102,.T.) ;
#48890=ORIENTED_EDGE('',*,*,#37154,.T.) ;
#48891=ORIENTED_EDGE('',*,*,#37155,.F.) ;
#48892=ORIENTED_EDGE('',*,*,#37156,.T.) ;
#48893=ORIENTED_EDGE('',*,*,#37157,.F.) ;
#48894=ORIENTED_EDGE('',*,*,#37158,.T.) ;
#48895=ORIENTED_EDGE('',*,*,#37159,.T.) ;
#48896=ORIENTED_EDGE('',*,*,#37160,.T.) ;
#48897=ORIENTED_EDGE('',*,*,#37161,.F.) ;
#48898=ORIENTED_EDGE('',*,*,#37162,.T.) ;
#48899=ORIENTED_EDGE('',*,*,#37163,.F.) ;
#48900=ORIENTED_EDGE('',*,*,#37164,.T.) ;
#48901=ORIENTED_EDGE('',*,*,#37165,.T.) ;
#48902=ORIENTED_EDGE('',*,*,#37166,.T.) ;
#48903=ORIENTED_EDGE('',*,*,#37167,.T.) ;
#48904=ORIENTED_EDGE('',*,*,#37168,.T.) ;
#48905=ORIENTED_EDGE('',*,*,#37169,.T.) ;
#48906=ORIENTED_EDGE('',*,*,#37170,.T.) ;
#48907=ORIENTED_EDGE('',*,*,#37136,.T.) ;
#48908=ORIENTED_EDGE('',*,*,#37171,.T.) ;
#48909=ORIENTED_EDGE('',*,*,#37146,.F.) ;
#48910=ORIENTED_EDGE('',*,*,#37172,.T.) ;
#48911=ORIENTED_EDGE('',*,*,#37138,.T.) ;
#48912=ORIENTED_EDGE('',*,*,#37173,.T.) ;
#48913=ORIENTED_EDGE('',*,*,#37144,.F.) ;
#48914=ORIENTED_EDGE('',*,*,#37174,.T.) ;
#48915=ORIENTED_EDGE('',*,*,#37175,.T.) ;
#48916=ORIENTED_EDGE('',*,*,#37176,.T.) ;
#48917=ORIENTED_EDGE('',*,*,#37112,.T.) ;
#48918=ORIENTED_EDGE('',*,*,#37177,.T.) ;
#48919=ORIENTED_EDGE('',*,*,#37142,.F.) ;
#48920=ORIENTED_EDGE('',*,*,#37178,.T.) ;
#48921=ORIENTED_EDGE('',*,*,#37179,.T.) ;
#48922=ORIENTED_EDGE('',*,*,#37180,.T.) ;
#48923=ORIENTED_EDGE('',*,*,#37181,.T.) ;
#48924=ORIENTED_EDGE('',*,*,#37182,.T.) ;
#48925=ORIENTED_EDGE('',*,*,#37183,.T.) ;
#48926=ORIENTED_EDGE('',*,*,#37140,.F.) ;
#48927=ORIENTED_EDGE('',*,*,#37184,.T.) ;
#48928=ORIENTED_EDGE('',*,*,#37185,.T.) ;
#48929=ORIENTED_EDGE('',*,*,#37186,.T.) ;
#48930=ORIENTED_EDGE('',*,*,#37187,.T.) ;
#48931=ORIENTED_EDGE('',*,*,#37169,.F.) ;
#48932=ORIENTED_EDGE('',*,*,#37188,.T.) ;
#48933=ORIENTED_EDGE('',*,*,#37189,.T.) ;
#48934=ORIENTED_EDGE('',*,*,#37043,.T.) ;
#48935=ORIENTED_EDGE('',*,*,#37190,.T.) ;
#48936=ORIENTED_EDGE('',*,*,#37191,.T.) ;
#48937=ORIENTED_EDGE('',*,*,#37167,.F.) ;
#48938=ORIENTED_EDGE('',*,*,#37192,.T.) ;
#48939=ORIENTED_EDGE('',*,*,#37193,.T.) ;
#48940=ORIENTED_EDGE('',*,*,#37194,.T.) ;
#48941=ORIENTED_EDGE('',*,*,#37195,.T.) ;
#48942=ORIENTED_EDGE('',*,*,#37196,.T.) ;
#48943=ORIENTED_EDGE('',*,*,#37197,.T.) ;
#48944=ORIENTED_EDGE('',*,*,#37165,.F.) ;
#48945=ORIENTED_EDGE('',*,*,#37198,.T.) ;
#48946=ORIENTED_EDGE('',*,*,#37199,.T.) ;
#48947=ORIENTED_EDGE('',*,*,#37200,.F.) ;
#48948=ORIENTED_EDGE('',*,*,#37201,.T.) ;
#48949=ORIENTED_EDGE('',*,*,#37202,.F.) ;
#48950=ORIENTED_EDGE('',*,*,#37203,.T.) ;
#48951=ORIENTED_EDGE('',*,*,#37204,.T.) ;
#48952=ORIENTED_EDGE('',*,*,#37117,.T.) ;
#48953=ORIENTED_EDGE('',*,*,#37205,.F.) ;
#48954=ORIENTED_EDGE('',*,*,#37206,.T.) ;
#48955=ORIENTED_EDGE('',*,*,#37123,.T.) ;
#48956=ORIENTED_EDGE('',*,*,#37207,.T.) ;
#48957=ORIENTED_EDGE('',*,*,#37208,.F.) ;
#48958=ORIENTED_EDGE('',*,*,#37209,.T.) ;
#48959=ORIENTED_EDGE('',*,*,#37210,.F.) ;
#48960=ORIENTED_EDGE('',*,*,#37211,.T.) ;
#48961=ORIENTED_EDGE('',*,*,#37212,.T.) ;
#48962=ORIENTED_EDGE('',*,*,#37213,.T.) ;
#48963=ORIENTED_EDGE('',*,*,#37214,.F.) ;
#48964=ORIENTED_EDGE('',*,*,#37215,.T.) ;
#48965=ORIENTED_EDGE('',*,*,#37216,.F.) ;
#48966=ORIENTED_EDGE('',*,*,#37217,.T.) ;
#48967=ORIENTED_EDGE('',*,*,#37159,.F.) ;
#48968=ORIENTED_EDGE('',*,*,#37218,.T.) ;
#48969=ORIENTED_EDGE('',*,*,#37219,.F.) ;
#48970=ORIENTED_EDGE('',*,*,#37220,.T.) ;
#48971=ORIENTED_EDGE('',*,*,#37221,.F.) ;
#48972=ORIENTED_EDGE('',*,*,#37222,.T.) ;
#48973=ORIENTED_EDGE('',*,*,#37223,.T.) ;
#48974=ORIENTED_EDGE('',*,*,#37224,.T.) ;
#48975=ORIENTED_EDGE('',*,*,#37225,.F.) ;
#48976=ORIENTED_EDGE('',*,*,#37226,.T.) ;
#48977=ORIENTED_EDGE('',*,*,#37054,.T.) ;
#48978=ORIENTED_EDGE('',*,*,#37227,.F.) ;
#48979=ORIENTED_EDGE('',*,*,#37228,.T.) ;
#48980=ORIENTED_EDGE('',*,*,#37229,.F.) ;
#48981=ORIENTED_EDGE('',*,*,#37133,.T.) ;
#48982=ORIENTED_EDGE('',*,*,#37230,.T.) ;
#48983=ORIENTED_EDGE('',*,*,#37149,.F.) ;
#48984=ORIENTED_EDGE('',*,*,#37231,.F.) ;
#48985=ORIENTED_EDGE('',*,*,#37232,.T.) ;
#48986=ORIENTED_EDGE('',*,*,#37233,.F.) ;
#48987=ORIENTED_EDGE('',*,*,#37234,.T.) ;
#48988=ORIENTED_EDGE('',*,*,#37235,.F.) ;
#48989=ORIENTED_EDGE('',*,*,#37236,.T.) ;
#48990=ORIENTED_EDGE('',*,*,#37231,.T.) ;
#48991=ORIENTED_EDGE('',*,*,#37148,.F.) ;
#48992=ORIENTED_EDGE('',*,*,#37237,.T.) ;
#48993=ORIENTED_EDGE('',*,*,#37134,.T.) ;
#48994=ORIENTED_EDGE('',*,*,#37229,.T.) ;
#48995=ORIENTED_EDGE('',*,*,#37238,.T.) ;
#48996=ORIENTED_EDGE('',*,*,#37239,.F.) ;
#48997=ORIENTED_EDGE('',*,*,#37240,.T.) ;
#48998=ORIENTED_EDGE('',*,*,#37241,.T.) ;
#48999=ORIENTED_EDGE('',*,*,#37242,.T.) ;
#49000=ORIENTED_EDGE('',*,*,#37243,.F.) ;
#49001=ORIENTED_EDGE('',*,*,#37244,.F.) ;
#49002=ORIENTED_EDGE('',*,*,#37245,.T.) ;
#49003=ORIENTED_EDGE('',*,*,#37246,.T.) ;
#49004=ORIENTED_EDGE('',*,*,#37247,.T.) ;
#49005=ORIENTED_EDGE('',*,*,#37248,.T.) ;
#49006=ORIENTED_EDGE('',*,*,#37249,.T.) ;
#49007=ORIENTED_EDGE('',*,*,#37250,.T.) ;
#49008=ORIENTED_EDGE('',*,*,#37251,.T.) ;
#49009=ORIENTED_EDGE('',*,*,#37252,.T.) ;
#49010=ORIENTED_EDGE('',*,*,#37253,.T.) ;
#49011=ORIENTED_EDGE('',*,*,#37254,.T.) ;
#49012=ORIENTED_EDGE('',*,*,#37255,.T.) ;
#49013=ORIENTED_EDGE('',*,*,#37256,.T.) ;
#49014=ORIENTED_EDGE('',*,*,#37257,.T.) ;
#49015=ORIENTED_EDGE('',*,*,#37258,.T.) ;
#49016=ORIENTED_EDGE('',*,*,#37259,.T.) ;
#49017=ORIENTED_EDGE('',*,*,#37260,.T.) ;
#49018=ORIENTED_EDGE('',*,*,#37261,.T.) ;
#49019=ORIENTED_EDGE('',*,*,#37262,.T.) ;
#49020=ORIENTED_EDGE('',*,*,#37263,.T.) ;
#49021=ORIENTED_EDGE('',*,*,#37264,.T.) ;
#49022=ORIENTED_EDGE('',*,*,#37265,.T.) ;
#49023=ORIENTED_EDGE('',*,*,#37266,.T.) ;
#49024=ORIENTED_EDGE('',*,*,#37267,.T.) ;
#49025=ORIENTED_EDGE('',*,*,#37268,.T.) ;
#49026=ORIENTED_EDGE('',*,*,#37269,.T.) ;
#49027=ORIENTED_EDGE('',*,*,#37270,.T.) ;
#49028=ORIENTED_EDGE('',*,*,#37271,.T.) ;
#49029=ORIENTED_EDGE('',*,*,#37272,.T.) ;
#49030=ORIENTED_EDGE('',*,*,#37273,.T.) ;
#49031=ORIENTED_EDGE('',*,*,#37274,.T.) ;
#49032=ORIENTED_EDGE('',*,*,#37275,.T.) ;
#49033=ORIENTED_EDGE('',*,*,#37276,.T.) ;
#49034=ORIENTED_EDGE('',*,*,#37277,.T.) ;
#49035=ORIENTED_EDGE('',*,*,#37278,.T.) ;
#49036=ORIENTED_EDGE('',*,*,#37279,.T.) ;
#49037=ORIENTED_EDGE('',*,*,#37280,.T.) ;
#49038=ORIENTED_EDGE('',*,*,#37049,.T.) ;
#49039=ORIENTED_EDGE('',*,*,#37281,.F.) ;
#49040=ORIENTED_EDGE('',*,*,#37282,.T.) ;
#49041=ORIENTED_EDGE('',*,*,#37283,.T.) ;
#49042=ORIENTED_EDGE('',*,*,#37284,.T.) ;
#49043=ORIENTED_EDGE('',*,*,#37285,.T.) ;
#49044=ORIENTED_EDGE('',*,*,#37286,.T.) ;
#49045=ORIENTED_EDGE('',*,*,#37287,.T.) ;
#49046=ORIENTED_EDGE('',*,*,#37288,.T.) ;
#49047=ORIENTED_EDGE('',*,*,#37289,.F.) ;
#49048=ORIENTED_EDGE('',*,*,#37290,.T.) ;
#49049=ORIENTED_EDGE('',*,*,#37127,.T.) ;
#49050=ORIENTED_EDGE('',*,*,#37291,.T.) ;
#49051=ORIENTED_EDGE('',*,*,#37292,.T.) ;
#49052=ORIENTED_EDGE('',*,*,#37293,.T.) ;
#49053=ORIENTED_EDGE('',*,*,#37294,.T.) ;
#49054=ORIENTED_EDGE('',*,*,#37125,.F.) ;
#49055=ORIENTED_EDGE('',*,*,#37295,.T.) ;
#49056=ORIENTED_EDGE('',*,*,#37296,.T.) ;
#49057=ORIENTED_EDGE('',*,*,#37297,.T.) ;
#49058=ORIENTED_EDGE('',*,*,#37298,.T.) ;
#49059=ORIENTED_EDGE('',*,*,#37299,.T.) ;
#49060=ORIENTED_EDGE('',*,*,#37063,.T.) ;
#49061=ORIENTED_EDGE('',*,*,#37300,.T.) ;
#49062=ORIENTED_EDGE('',*,*,#37301,.T.) ;
#49063=ORIENTED_EDGE('',*,*,#37302,.T.) ;
#49064=ORIENTED_EDGE('',*,*,#37303,.T.) ;
#49065=ORIENTED_EDGE('',*,*,#37304,.T.) ;
#49066=ORIENTED_EDGE('',*,*,#37305,.T.) ;
#49067=ORIENTED_EDGE('',*,*,#37306,.T.) ;
#49068=ORIENTED_EDGE('',*,*,#37307,.T.) ;
#49069=ORIENTED_EDGE('',*,*,#37308,.T.) ;
#49070=ORIENTED_EDGE('',*,*,#37056,.T.) ;
#49071=ORIENTED_EDGE('',*,*,#37309,.T.) ;
#49072=ORIENTED_EDGE('',*,*,#37310,.T.) ;
#49073=ORIENTED_EDGE('',*,*,#37311,.T.) ;
#49074=ORIENTED_EDGE('',*,*,#37312,.T.) ;
#49075=ORIENTED_EDGE('',*,*,#37313,.T.) ;
#49076=ORIENTED_EDGE('',*,*,#37157,.T.) ;
#49077=ORIENTED_EDGE('',*,*,#37314,.T.) ;
#49078=ORIENTED_EDGE('',*,*,#37315,.T.) ;
#49079=ORIENTED_EDGE('',*,*,#37316,.T.) ;
#49080=ORIENTED_EDGE('',*,*,#37155,.T.) ;
#49081=ORIENTED_EDGE('',*,*,#37317,.T.) ;
#49082=ORIENTED_EDGE('',*,*,#37318,.F.) ;
#49083=ORIENTED_EDGE('',*,*,#37319,.T.) ;
#49084=ORIENTED_EDGE('',*,*,#37320,.T.) ;
#49085=ORIENTED_EDGE('',*,*,#37321,.T.) ;
#49086=ORIENTED_EDGE('',*,*,#37322,.T.) ;
#49087=ORIENTED_EDGE('',*,*,#37119,.T.) ;
#49088=ORIENTED_EDGE('',*,*,#37323,.T.) ;
#49089=ORIENTED_EDGE('',*,*,#37324,.T.) ;
#49090=ORIENTED_EDGE('',*,*,#37325,.T.) ;
#49091=ORIENTED_EDGE('',*,*,#37326,.T.) ;
#49092=ORIENTED_EDGE('',*,*,#37121,.F.) ;
#49093=ORIENTED_EDGE('',*,*,#37327,.T.) ;
#49094=ORIENTED_EDGE('',*,*,#37328,.T.) ;
#49095=ORIENTED_EDGE('',*,*,#37329,.T.) ;
#49096=ORIENTED_EDGE('',*,*,#37330,.T.) ;
#49097=ORIENTED_EDGE('',*,*,#37331,.T.) ;
#49098=ORIENTED_EDGE('',*,*,#37332,.T.) ;
#49099=ORIENTED_EDGE('',*,*,#37333,.T.) ;
#49100=ORIENTED_EDGE('',*,*,#37334,.T.) ;
#49101=ORIENTED_EDGE('',*,*,#37335,.T.) ;
#49102=ORIENTED_EDGE('',*,*,#37336,.T.) ;
#49103=ORIENTED_EDGE('',*,*,#37337,.T.) ;
#49104=ORIENTED_EDGE('',*,*,#37338,.T.) ;
#49105=ORIENTED_EDGE('',*,*,#37339,.T.) ;
#49106=ORIENTED_EDGE('',*,*,#37161,.T.) ;
#49107=ORIENTED_EDGE('',*,*,#37340,.T.) ;
#49108=ORIENTED_EDGE('',*,*,#37341,.T.) ;
#49109=ORIENTED_EDGE('',*,*,#37342,.T.) ;
#49110=ORIENTED_EDGE('',*,*,#37343,.T.) ;
#49111=ORIENTED_EDGE('',*,*,#37344,.T.) ;
#49112=ORIENTED_EDGE('',*,*,#37345,.T.) ;
#49113=ORIENTED_EDGE('',*,*,#37346,.T.) ;
#49114=ORIENTED_EDGE('',*,*,#37347,.T.) ;
#49115=ORIENTED_EDGE('',*,*,#37348,.T.) ;
#49116=ORIENTED_EDGE('',*,*,#37163,.T.) ;
#49117=ORIENTED_EDGE('',*,*,#37349,.T.) ;
#49118=ORIENTED_EDGE('',*,*,#37350,.T.) ;
#49119=ORIENTED_EDGE('',*,*,#37351,.T.) ;
#49120=ORIENTED_EDGE('',*,*,#37352,.T.) ;
#49121=ORIENTED_EDGE('',*,*,#37353,.T.) ;
#49122=ORIENTED_EDGE('',*,*,#37354,.T.) ;
#49123=ORIENTED_EDGE('',*,*,#37355,.T.) ;
#49124=ORIENTED_EDGE('',*,*,#37356,.T.) ;
#49125=ORIENTED_EDGE('',*,*,#37048,.T.) ;
#49126=ORIENTED_EDGE('',*,*,#37357,.T.) ;
#49127=ORIENTED_EDGE('',*,*,#37358,.T.) ;
#49128=ORIENTED_EDGE('',*,*,#37359,.T.) ;
#49129=ORIENTED_EDGE('',*,*,#37360,.T.) ;
#49130=ORIENTED_EDGE('',*,*,#37361,.T.) ;
#49131=ORIENTED_EDGE('',*,*,#37362,.T.) ;
#49132=ORIENTED_EDGE('',*,*,#37363,.T.) ;
#49133=ORIENTED_EDGE('',*,*,#37364,.T.) ;
#49134=ORIENTED_EDGE('',*,*,#37365,.T.) ;
#49135=ORIENTED_EDGE('',*,*,#37366,.T.) ;
#49136=ORIENTED_EDGE('',*,*,#37367,.T.) ;
#49137=ORIENTED_EDGE('',*,*,#37368,.T.) ;
#49138=ORIENTED_EDGE('',*,*,#37369,.T.) ;
#49139=ORIENTED_EDGE('',*,*,#37370,.T.) ;
#49140=ORIENTED_EDGE('',*,*,#37371,.T.) ;
#49141=ORIENTED_EDGE('',*,*,#37372,.T.) ;
#49142=ORIENTED_EDGE('',*,*,#37373,.T.) ;
#49143=ORIENTED_EDGE('',*,*,#37374,.T.) ;
#49144=ORIENTED_EDGE('',*,*,#37375,.T.) ;
#49145=ORIENTED_EDGE('',*,*,#37376,.T.) ;
#49146=ORIENTED_EDGE('',*,*,#37377,.T.) ;
#49147=ORIENTED_EDGE('',*,*,#37378,.T.) ;
#49148=ORIENTED_EDGE('',*,*,#37379,.T.) ;
#49149=ORIENTED_EDGE('',*,*,#37380,.T.) ;
#49150=ORIENTED_EDGE('',*,*,#37281,.T.) ;
#49151=ORIENTED_EDGE('',*,*,#37381,.T.) ;
#49152=ORIENTED_EDGE('',*,*,#37382,.T.) ;
#49153=ORIENTED_EDGE('',*,*,#37383,.T.) ;
#49154=ORIENTED_EDGE('',*,*,#37285,.F.) ;
#49155=ORIENTED_EDGE('',*,*,#37384,.T.) ;
#49156=ORIENTED_EDGE('',*,*,#37385,.T.) ;
#49157=ORIENTED_EDGE('',*,*,#37386,.T.) ;
#49158=ORIENTED_EDGE('',*,*,#37287,.F.) ;
#49159=ORIENTED_EDGE('',*,*,#37387,.T.) ;
#49160=ORIENTED_EDGE('',*,*,#37388,.T.) ;
#49161=ORIENTED_EDGE('',*,*,#37389,.T.) ;
#49162=ORIENTED_EDGE('',*,*,#37283,.F.) ;
#49163=ORIENTED_EDGE('',*,*,#37390,.T.) ;
#49164=ORIENTED_EDGE('',*,*,#37391,.T.) ;
#49165=ORIENTED_EDGE('',*,*,#37392,.T.) ;
#49166=ORIENTED_EDGE('',*,*,#37393,.T.) ;
#49167=ORIENTED_EDGE('',*,*,#37394,.T.) ;
#49168=ORIENTED_EDGE('',*,*,#37395,.T.) ;
#49169=ORIENTED_EDGE('',*,*,#37396,.T.) ;
#49170=ORIENTED_EDGE('',*,*,#37397,.T.) ;
#49171=ORIENTED_EDGE('',*,*,#37398,.T.) ;
#49172=ORIENTED_EDGE('',*,*,#37399,.T.) ;
#49173=ORIENTED_EDGE('',*,*,#37400,.T.) ;
#49174=ORIENTED_EDGE('',*,*,#37401,.T.) ;
#49175=ORIENTED_EDGE('',*,*,#37402,.F.) ;
#49176=ORIENTED_EDGE('',*,*,#37403,.T.) ;
#49177=ORIENTED_EDGE('',*,*,#37079,.F.) ;
#49178=ORIENTED_EDGE('',*,*,#37404,.T.) ;
#49179=ORIENTED_EDGE('',*,*,#37405,.T.) ;
#49180=ORIENTED_EDGE('',*,*,#37406,.T.) ;
#49181=ORIENTED_EDGE('',*,*,#37407,.T.) ;
#49182=ORIENTED_EDGE('',*,*,#37402,.T.) ;
#49183=ORIENTED_EDGE('',*,*,#37408,.T.) ;
#49184=ORIENTED_EDGE('',*,*,#37409,.T.) ;
#49185=ORIENTED_EDGE('',*,*,#37410,.T.) ;
#49186=ORIENTED_EDGE('',*,*,#37411,.T.) ;
#49187=ORIENTED_EDGE('',*,*,#37412,.T.) ;
#49188=ORIENTED_EDGE('',*,*,#37413,.T.) ;
#49189=ORIENTED_EDGE('',*,*,#37414,.T.) ;
#49190=ORIENTED_EDGE('',*,*,#37415,.T.) ;
#49191=ORIENTED_EDGE('',*,*,#37416,.T.) ;
#49192=ORIENTED_EDGE('',*,*,#37417,.T.) ;
#49193=ORIENTED_EDGE('',*,*,#37418,.T.) ;
#49194=ORIENTED_EDGE('',*,*,#37419,.T.) ;
#49195=ORIENTED_EDGE('',*,*,#37420,.T.) ;
#49196=ORIENTED_EDGE('',*,*,#37421,.T.) ;
#49197=ORIENTED_EDGE('',*,*,#37422,.T.) ;
#49198=ORIENTED_EDGE('',*,*,#37423,.F.) ;
#49199=ORIENTED_EDGE('',*,*,#37272,.F.) ;
#49200=ORIENTED_EDGE('',*,*,#37424,.T.) ;
#49201=ORIENTED_EDGE('',*,*,#37423,.T.) ;
#49202=ORIENTED_EDGE('',*,*,#37425,.T.) ;
#49203=ORIENTED_EDGE('',*,*,#37426,.T.) ;
#49204=ORIENTED_EDGE('',*,*,#37427,.T.) ;
#49205=ORIENTED_EDGE('',*,*,#37428,.T.) ;
#49206=ORIENTED_EDGE('',*,*,#37429,.T.) ;
#49207=ORIENTED_EDGE('',*,*,#37430,.T.) ;
#49208=ORIENTED_EDGE('',*,*,#37431,.T.) ;
#49209=ORIENTED_EDGE('',*,*,#37432,.T.) ;
#49210=ORIENTED_EDGE('',*,*,#37433,.T.) ;
#49211=ORIENTED_EDGE('',*,*,#37434,.T.) ;
#49212=ORIENTED_EDGE('',*,*,#37435,.T.) ;
#49213=ORIENTED_EDGE('',*,*,#37436,.T.) ;
#49214=ORIENTED_EDGE('',*,*,#37437,.T.) ;
#49215=ORIENTED_EDGE('',*,*,#37438,.T.) ;
#49216=ORIENTED_EDGE('',*,*,#37439,.T.) ;
#49217=ORIENTED_EDGE('',*,*,#37440,.T.) ;
#49218=ORIENTED_EDGE('',*,*,#37441,.T.) ;
#49219=ORIENTED_EDGE('',*,*,#37442,.T.) ;
#49220=ORIENTED_EDGE('',*,*,#37443,.T.) ;
#49221=ORIENTED_EDGE('',*,*,#37444,.T.) ;
#49222=ORIENTED_EDGE('',*,*,#37152,.F.) ;
#49223=ORIENTED_EDGE('',*,*,#37445,.T.) ;
#49224=ORIENTED_EDGE('',*,*,#37446,.T.) ;
#49225=ORIENTED_EDGE('',*,*,#37066,.T.) ;
#49226=ORIENTED_EDGE('',*,*,#37447,.T.) ;
#49227=ORIENTED_EDGE('',*,*,#37130,.F.) ;
#49228=ORIENTED_EDGE('',*,*,#37448,.T.) ;
#49229=ORIENTED_EDGE('',*,*,#37449,.T.) ;
#49230=ORIENTED_EDGE('',*,*,#37450,.T.) ;
#49231=ORIENTED_EDGE('',*,*,#37451,.F.) ;
#49232=ORIENTED_EDGE('',*,*,#37349,.F.) ;
#49233=ORIENTED_EDGE('',*,*,#37162,.F.) ;
#49234=ORIENTED_EDGE('',*,*,#37342,.F.) ;
#49235=ORIENTED_EDGE('',*,*,#37452,.F.) ;
#49236=ORIENTED_EDGE('',*,*,#37451,.T.) ;
#49237=ORIENTED_EDGE('',*,*,#37453,.F.) ;
#49238=ORIENTED_EDGE('',*,*,#37160,.F.) ;
#49239=ORIENTED_EDGE('',*,*,#37217,.F.) ;
#49240=ORIENTED_EDGE('',*,*,#37454,.F.) ;
#49241=ORIENTED_EDGE('',*,*,#37340,.F.) ;
#49242=ORIENTED_EDGE('',*,*,#37453,.T.) ;
#49243=ORIENTED_EDGE('',*,*,#37341,.F.) ;
#49244=ORIENTED_EDGE('',*,*,#37455,.F.) ;
#49245=ORIENTED_EDGE('',*,*,#37337,.F.) ;
#49246=ORIENTED_EDGE('',*,*,#37452,.T.) ;
#49247=ORIENTED_EDGE('',*,*,#37336,.F.) ;
#49248=ORIENTED_EDGE('',*,*,#37456,.F.) ;
#49249=ORIENTED_EDGE('',*,*,#37350,.F.) ;
#49250=ORIENTED_EDGE('',*,*,#37454,.T.) ;
#49251=ORIENTED_EDGE('',*,*,#37216,.T.) ;
#49252=ORIENTED_EDGE('',*,*,#37457,.F.) ;
#49253=ORIENTED_EDGE('',*,*,#37455,.T.) ;
#49254=ORIENTED_EDGE('',*,*,#37458,.F.) ;
#49255=ORIENTED_EDGE('',*,*,#37456,.T.) ;
#49256=ORIENTED_EDGE('',*,*,#37459,.F.) ;
#49257=ORIENTED_EDGE('',*,*,#37120,.F.) ;
#49258=ORIENTED_EDGE('',*,*,#37322,.F.) ;
#49259=ORIENTED_EDGE('',*,*,#37460,.F.) ;
#49260=ORIENTED_EDGE('',*,*,#37327,.F.) ;
#49261=ORIENTED_EDGE('',*,*,#37461,.F.) ;
#49262=ORIENTED_EDGE('',*,*,#37325,.F.) ;
#49263=ORIENTED_EDGE('',*,*,#37462,.F.) ;
#49264=ORIENTED_EDGE('',*,*,#37331,.F.) ;
#49265=ORIENTED_EDGE('',*,*,#37122,.F.) ;
#49266=ORIENTED_EDGE('',*,*,#37326,.F.) ;
#49267=ORIENTED_EDGE('',*,*,#37463,.F.) ;
#49268=ORIENTED_EDGE('',*,*,#37207,.F.) ;
#49269=ORIENTED_EDGE('',*,*,#37457,.T.) ;
#49270=ORIENTED_EDGE('',*,*,#37215,.F.) ;
#49271=ORIENTED_EDGE('',*,*,#37464,.F.) ;
#49272=ORIENTED_EDGE('',*,*,#37338,.F.) ;
#49273=ORIENTED_EDGE('',*,*,#37459,.T.) ;
#49274=ORIENTED_EDGE('',*,*,#37339,.F.) ;
#49275=ORIENTED_EDGE('',*,*,#37465,.F.) ;
#49276=ORIENTED_EDGE('',*,*,#37346,.F.) ;
#49277=ORIENTED_EDGE('',*,*,#37458,.T.) ;
#49278=ORIENTED_EDGE('',*,*,#37345,.F.) ;
#49279=ORIENTED_EDGE('',*,*,#37466,.F.) ;
#49280=ORIENTED_EDGE('',*,*,#37347,.F.) ;
#49281=ORIENTED_EDGE('',*,*,#37164,.F.) ;
#49282=ORIENTED_EDGE('',*,*,#37348,.F.) ;
#49283=ORIENTED_EDGE('',*,*,#37467,.F.) ;
#49284=ORIENTED_EDGE('',*,*,#37198,.F.) ;
#49285=ORIENTED_EDGE('',*,*,#37462,.T.) ;
#49286=ORIENTED_EDGE('',*,*,#37460,.T.) ;
#49287=ORIENTED_EDGE('',*,*,#37468,.F.) ;
#49288=ORIENTED_EDGE('',*,*,#37463,.T.) ;
#49289=ORIENTED_EDGE('',*,*,#37461,.T.) ;
#49290=ORIENTED_EDGE('',*,*,#37469,.F.) ;
#49291=ORIENTED_EDGE('',*,*,#37208,.T.) ;
#49292=ORIENTED_EDGE('',*,*,#37464,.T.) ;
#49293=ORIENTED_EDGE('',*,*,#37214,.T.) ;
#49294=ORIENTED_EDGE('',*,*,#37470,.F.) ;
#49295=ORIENTED_EDGE('',*,*,#37465,.T.) ;
#49296=ORIENTED_EDGE('',*,*,#37467,.T.) ;
#49297=ORIENTED_EDGE('',*,*,#37466,.T.) ;
#49298=ORIENTED_EDGE('',*,*,#37471,.F.) ;
#49299=ORIENTED_EDGE('',*,*,#37468,.T.) ;
#49300=ORIENTED_EDGE('',*,*,#37321,.F.) ;
#49301=ORIENTED_EDGE('',*,*,#37472,.F.) ;
#49302=ORIENTED_EDGE('',*,*,#37328,.F.) ;
#49303=ORIENTED_EDGE('',*,*,#37473,.F.) ;
#49304=ORIENTED_EDGE('',*,*,#37329,.F.) ;
#49305=ORIENTED_EDGE('',*,*,#37474,.F.) ;
#49306=ORIENTED_EDGE('',*,*,#37335,.F.) ;
#49307=ORIENTED_EDGE('',*,*,#37469,.T.) ;
#49308=ORIENTED_EDGE('',*,*,#37330,.F.) ;
#49309=ORIENTED_EDGE('',*,*,#37475,.F.) ;
#49310=ORIENTED_EDGE('',*,*,#37209,.F.) ;
#49311=ORIENTED_EDGE('',*,*,#37470,.T.) ;
#49312=ORIENTED_EDGE('',*,*,#37213,.F.) ;
#49313=ORIENTED_EDGE('',*,*,#37476,.F.) ;
#49314=ORIENTED_EDGE('',*,*,#37343,.F.) ;
#49315=ORIENTED_EDGE('',*,*,#37471,.T.) ;
#49316=ORIENTED_EDGE('',*,*,#37344,.F.) ;
#49317=ORIENTED_EDGE('',*,*,#37477,.F.) ;
#49318=ORIENTED_EDGE('',*,*,#37199,.F.) ;
#49319=ORIENTED_EDGE('',*,*,#37474,.T.) ;
#49320=ORIENTED_EDGE('',*,*,#37472,.T.) ;
#49321=ORIENTED_EDGE('',*,*,#37478,.F.) ;
#49322=ORIENTED_EDGE('',*,*,#37475,.T.) ;
#49323=ORIENTED_EDGE('',*,*,#37473,.T.) ;
#49324=ORIENTED_EDGE('',*,*,#37479,.F.) ;
#49325=ORIENTED_EDGE('',*,*,#37210,.T.) ;
#49326=ORIENTED_EDGE('',*,*,#37477,.T.) ;
#49327=ORIENTED_EDGE('',*,*,#37476,.T.) ;
#49328=ORIENTED_EDGE('',*,*,#37480,.F.) ;
#49329=ORIENTED_EDGE('',*,*,#37200,.T.) ;
#49330=ORIENTED_EDGE('',*,*,#37118,.F.) ;
#49331=ORIENTED_EDGE('',*,*,#37204,.F.) ;
#49332=ORIENTED_EDGE('',*,*,#37481,.F.) ;
#49333=ORIENTED_EDGE('',*,*,#37323,.F.) ;
#49334=ORIENTED_EDGE('',*,*,#37478,.T.) ;
#49335=ORIENTED_EDGE('',*,*,#37324,.F.) ;
#49336=ORIENTED_EDGE('',*,*,#37482,.F.) ;
#49337=ORIENTED_EDGE('',*,*,#37332,.F.) ;
#49338=ORIENTED_EDGE('',*,*,#37479,.T.) ;
#49339=ORIENTED_EDGE('',*,*,#37334,.F.) ;
#49340=ORIENTED_EDGE('',*,*,#37483,.F.) ;
#49341=ORIENTED_EDGE('',*,*,#37211,.F.) ;
#49342=ORIENTED_EDGE('',*,*,#37480,.T.) ;
#49343=ORIENTED_EDGE('',*,*,#37212,.F.) ;
#49344=ORIENTED_EDGE('',*,*,#37484,.F.) ;
#49345=ORIENTED_EDGE('',*,*,#37201,.F.) ;
#49346=ORIENTED_EDGE('',*,*,#37482,.T.) ;
#49347=ORIENTED_EDGE('',*,*,#37481,.T.) ;
#49348=ORIENTED_EDGE('',*,*,#37485,.F.) ;
#49349=ORIENTED_EDGE('',*,*,#37484,.T.) ;
#49350=ORIENTED_EDGE('',*,*,#37483,.T.) ;
#49351=ORIENTED_EDGE('',*,*,#37486,.F.) ;
#49352=ORIENTED_EDGE('',*,*,#37202,.T.) ;
#49353=ORIENTED_EDGE('',*,*,#37485,.T.) ;
#49354=ORIENTED_EDGE('',*,*,#37203,.F.) ;
#49355=ORIENTED_EDGE('',*,*,#37486,.T.) ;
#49356=ORIENTED_EDGE('',*,*,#37333,.F.) ;
#49357=ORIENTED_EDGE('',*,*,#37487,.F.) ;
#49358=ORIENTED_EDGE('',*,*,#37488,.F.) ;
#49359=ORIENTED_EDGE('',*,*,#37489,.F.) ;
#49360=ORIENTED_EDGE('',*,*,#37280,.F.) ;
#49361=ORIENTED_EDGE('',*,*,#37490,.T.) ;
#49362=ORIENTED_EDGE('',*,*,#37491,.T.) ;
#49363=ORIENTED_EDGE('',*,*,#37262,.F.) ;
#49364=ORIENTED_EDGE('',*,*,#37488,.T.) ;
#49365=ORIENTED_EDGE('',*,*,#37261,.F.) ;
#49366=ORIENTED_EDGE('',*,*,#37492,.T.) ;
#49367=ORIENTED_EDGE('',*,*,#37493,.T.) ;
#49368=ORIENTED_EDGE('',*,*,#37254,.F.) ;
#49369=ORIENTED_EDGE('',*,*,#37489,.T.) ;
#49370=ORIENTED_EDGE('',*,*,#37487,.T.) ;
#49371=ORIENTED_EDGE('',*,*,#37253,.F.) ;
#49372=ORIENTED_EDGE('',*,*,#37494,.F.) ;
#49373=ORIENTED_EDGE('',*,*,#37273,.F.) ;
#49374=ORIENTED_EDGE('',*,*,#37269,.F.) ;
#49375=ORIENTED_EDGE('',*,*,#37495,.T.) ;
#49376=ORIENTED_EDGE('',*,*,#37496,.T.) ;
#49377=ORIENTED_EDGE('',*,*,#37279,.F.) ;
#49378=ORIENTED_EDGE('',*,*,#37497,.T.) ;
#49379=ORIENTED_EDGE('',*,*,#37498,.T.) ;
#49380=ORIENTED_EDGE('',*,*,#37247,.F.) ;
#49381=ORIENTED_EDGE('',*,*,#37499,.T.) ;
#49382=ORIENTED_EDGE('',*,*,#37500,.T.) ;
#49383=ORIENTED_EDGE('',*,*,#37263,.F.) ;
#49384=ORIENTED_EDGE('',*,*,#37501,.T.) ;
#49385=ORIENTED_EDGE('',*,*,#37502,.T.) ;
#49386=ORIENTED_EDGE('',*,*,#37503,.F.) ;
#49387=ORIENTED_EDGE('',*,*,#37494,.T.) ;
#49388=ORIENTED_EDGE('',*,*,#37504,.F.) ;
#49389=ORIENTED_EDGE('',*,*,#37244,.T.) ;
#49390=ORIENTED_EDGE('',*,*,#37505,.F.) ;
#49391=ORIENTED_EDGE('',*,*,#37506,.F.) ;
#49392=ORIENTED_EDGE('',*,*,#37274,.F.) ;
#49393=ORIENTED_EDGE('',*,*,#37503,.T.) ;
#49394=ORIENTED_EDGE('',*,*,#37506,.T.) ;
#49395=ORIENTED_EDGE('',*,*,#37507,.F.) ;
#49396=ORIENTED_EDGE('',*,*,#37508,.F.) ;
#49397=ORIENTED_EDGE('',*,*,#37258,.F.) ;
#49398=ORIENTED_EDGE('',*,*,#37509,.T.) ;
#49399=ORIENTED_EDGE('',*,*,#37510,.T.) ;
#49400=ORIENTED_EDGE('',*,*,#37278,.F.) ;
#49401=ORIENTED_EDGE('',*,*,#37511,.F.) ;
#49402=ORIENTED_EDGE('',*,*,#37248,.F.) ;
#49403=ORIENTED_EDGE('',*,*,#37512,.T.) ;
#49404=ORIENTED_EDGE('',*,*,#37513,.T.) ;
#49405=ORIENTED_EDGE('',*,*,#37255,.F.) ;
#49406=ORIENTED_EDGE('',*,*,#37514,.F.) ;
#49407=ORIENTED_EDGE('',*,*,#37504,.T.) ;
#49408=ORIENTED_EDGE('',*,*,#37252,.F.) ;
#49409=ORIENTED_EDGE('',*,*,#37515,.F.) ;
#49410=ORIENTED_EDGE('',*,*,#37516,.F.) ;
#49411=ORIENTED_EDGE('',*,*,#37517,.F.) ;
#49412=ORIENTED_EDGE('',*,*,#37228,.F.) ;
#49413=ORIENTED_EDGE('',*,*,#37518,.F.) ;
#49414=ORIENTED_EDGE('',*,*,#37505,.T.) ;
#49415=ORIENTED_EDGE('',*,*,#37246,.F.) ;
#49416=ORIENTED_EDGE('',*,*,#37518,.T.) ;
#49417=ORIENTED_EDGE('',*,*,#37227,.T.) ;
#49418=ORIENTED_EDGE('',*,*,#37519,.F.) ;
#49419=ORIENTED_EDGE('',*,*,#37507,.T.) ;
#49420=ORIENTED_EDGE('',*,*,#37275,.F.) ;
#49421=ORIENTED_EDGE('',*,*,#37508,.T.) ;
#49422=ORIENTED_EDGE('',*,*,#37520,.F.) ;
#49423=ORIENTED_EDGE('',*,*,#37521,.F.) ;
#49424=ORIENTED_EDGE('',*,*,#37514,.T.) ;
#49425=ORIENTED_EDGE('',*,*,#37511,.T.) ;
#49426=ORIENTED_EDGE('',*,*,#37522,.F.) ;
#49427=ORIENTED_EDGE('',*,*,#37523,.F.) ;
#49428=ORIENTED_EDGE('',*,*,#37515,.T.) ;
#49429=ORIENTED_EDGE('',*,*,#37524,.F.) ;
#49430=ORIENTED_EDGE('',*,*,#37245,.F.) ;
#49431=ORIENTED_EDGE('',*,*,#37516,.T.) ;
#49432=ORIENTED_EDGE('',*,*,#37525,.F.) ;
#49433=ORIENTED_EDGE('',*,*,#37238,.F.) ;
#49434=ORIENTED_EDGE('',*,*,#37517,.T.) ;
#49435=ORIENTED_EDGE('',*,*,#37526,.F.) ;
#49436=ORIENTED_EDGE('',*,*,#37520,.T.) ;
#49437=ORIENTED_EDGE('',*,*,#37519,.T.) ;
#49438=ORIENTED_EDGE('',*,*,#37234,.F.) ;
#49439=ORIENTED_EDGE('',*,*,#37521,.T.) ;
#49440=ORIENTED_EDGE('',*,*,#37527,.F.) ;
#49441=ORIENTED_EDGE('',*,*,#37528,.F.) ;
#49442=ORIENTED_EDGE('',*,*,#37522,.T.) ;
#49443=ORIENTED_EDGE('',*,*,#37277,.F.) ;
#49444=ORIENTED_EDGE('',*,*,#37529,.F.) ;
#49445=ORIENTED_EDGE('',*,*,#37249,.F.) ;
#49446=ORIENTED_EDGE('',*,*,#37524,.T.) ;
#49447=ORIENTED_EDGE('',*,*,#37251,.F.) ;
#49448=ORIENTED_EDGE('',*,*,#37530,.F.) ;
#49449=ORIENTED_EDGE('',*,*,#37531,.F.) ;
#49450=ORIENTED_EDGE('',*,*,#37525,.T.) ;
#49451=ORIENTED_EDGE('',*,*,#37523,.T.) ;
#49452=ORIENTED_EDGE('',*,*,#37532,.F.) ;
#49453=ORIENTED_EDGE('',*,*,#37239,.T.) ;
#49454=ORIENTED_EDGE('',*,*,#37526,.T.) ;
#49455=ORIENTED_EDGE('',*,*,#37233,.T.) ;
#49456=ORIENTED_EDGE('',*,*,#37533,.F.) ;
#49457=ORIENTED_EDGE('',*,*,#37527,.T.) ;
#49458=ORIENTED_EDGE('',*,*,#37534,.F.) ;
#49459=ORIENTED_EDGE('',*,*,#37535,.F.) ;
#49460=ORIENTED_EDGE('',*,*,#37276,.F.) ;
#49461=ORIENTED_EDGE('',*,*,#37528,.T.) ;
#49462=ORIENTED_EDGE('',*,*,#37535,.T.) ;
#49463=ORIENTED_EDGE('',*,*,#37243,.T.) ;
#49464=ORIENTED_EDGE('',*,*,#37536,.F.) ;
#49465=ORIENTED_EDGE('',*,*,#37529,.T.) ;
#49466=ORIENTED_EDGE('',*,*,#37537,.F.) ;
#49467=ORIENTED_EDGE('',*,*,#37530,.T.) ;
#49468=ORIENTED_EDGE('',*,*,#37538,.F.) ;
#49469=ORIENTED_EDGE('',*,*,#37532,.T.) ;
#49470=ORIENTED_EDGE('',*,*,#37531,.T.) ;
#49471=ORIENTED_EDGE('',*,*,#37539,.F.) ;
#49472=ORIENTED_EDGE('',*,*,#37240,.F.) ;
#49473=ORIENTED_EDGE('',*,*,#37533,.T.) ;
#49474=ORIENTED_EDGE('',*,*,#37232,.F.) ;
#49475=ORIENTED_EDGE('',*,*,#37540,.F.) ;
#49476=ORIENTED_EDGE('',*,*,#37241,.F.) ;
#49477=ORIENTED_EDGE('',*,*,#37534,.T.) ;
#49478=ORIENTED_EDGE('',*,*,#37250,.F.) ;
#49479=ORIENTED_EDGE('',*,*,#37536,.T.) ;
#49480=ORIENTED_EDGE('',*,*,#37541,.F.) ;
#49481=ORIENTED_EDGE('',*,*,#37538,.T.) ;
#49482=ORIENTED_EDGE('',*,*,#37539,.T.) ;
#49483=ORIENTED_EDGE('',*,*,#37537,.T.) ;
#49484=ORIENTED_EDGE('',*,*,#37542,.F.) ;
#49485=ORIENTED_EDGE('',*,*,#37235,.T.) ;
#49486=ORIENTED_EDGE('',*,*,#37540,.T.) ;
#49487=ORIENTED_EDGE('',*,*,#37236,.F.) ;
#49488=ORIENTED_EDGE('',*,*,#37542,.T.) ;
#49489=ORIENTED_EDGE('',*,*,#37541,.T.) ;
#49490=ORIENTED_EDGE('',*,*,#37242,.F.) ;
#49491=ORIENTED_EDGE('',*,*,#37543,.F.) ;
#49492=ORIENTED_EDGE('',*,*,#37291,.F.) ;
#49493=ORIENTED_EDGE('',*,*,#37126,.F.) ;
#49494=ORIENTED_EDGE('',*,*,#37297,.F.) ;
#49495=ORIENTED_EDGE('',*,*,#37544,.F.) ;
#49496=ORIENTED_EDGE('',*,*,#37543,.T.) ;
#49497=ORIENTED_EDGE('',*,*,#37545,.F.) ;
#49498=ORIENTED_EDGE('',*,*,#37124,.F.) ;
#49499=ORIENTED_EDGE('',*,*,#37206,.F.) ;
#49500=ORIENTED_EDGE('',*,*,#37546,.F.) ;
#49501=ORIENTED_EDGE('',*,*,#37295,.F.) ;
#49502=ORIENTED_EDGE('',*,*,#37545,.T.) ;
#49503=ORIENTED_EDGE('',*,*,#37296,.F.) ;
#49504=ORIENTED_EDGE('',*,*,#37547,.F.) ;
#49505=ORIENTED_EDGE('',*,*,#37302,.F.) ;
#49506=ORIENTED_EDGE('',*,*,#37544,.T.) ;
#49507=ORIENTED_EDGE('',*,*,#37301,.F.) ;
#49508=ORIENTED_EDGE('',*,*,#37548,.F.) ;
#49509=ORIENTED_EDGE('',*,*,#37292,.F.) ;
#49510=ORIENTED_EDGE('',*,*,#37128,.F.) ;
#49511=ORIENTED_EDGE('',*,*,#37290,.F.) ;
#49512=ORIENTED_EDGE('',*,*,#37549,.F.) ;
#49513=ORIENTED_EDGE('',*,*,#37101,.F.) ;
#49514=ORIENTED_EDGE('',*,*,#37069,.F.) ;
#49515=ORIENTED_EDGE('',*,*,#37550,.T.) ;
#49516=ORIENTED_EDGE('',*,*,#37098,.F.) ;
#49517=ORIENTED_EDGE('',*,*,#37551,.F.) ;
#49518=ORIENTED_EDGE('',*,*,#37546,.T.) ;
#49519=ORIENTED_EDGE('',*,*,#37205,.T.) ;
#49520=ORIENTED_EDGE('',*,*,#37552,.F.) ;
#49521=ORIENTED_EDGE('',*,*,#37547,.T.) ;
#49522=ORIENTED_EDGE('',*,*,#37553,.F.) ;
#49523=ORIENTED_EDGE('',*,*,#37548,.T.) ;
#49524=ORIENTED_EDGE('',*,*,#37554,.F.) ;
#49525=ORIENTED_EDGE('',*,*,#37549,.T.) ;
#49526=ORIENTED_EDGE('',*,*,#37289,.T.) ;
#49527=ORIENTED_EDGE('',*,*,#37555,.F.) ;
#49528=ORIENTED_EDGE('',*,*,#37551,.T.) ;
#49529=ORIENTED_EDGE('',*,*,#37552,.T.) ;
#49530=ORIENTED_EDGE('',*,*,#37226,.F.) ;
#49531=ORIENTED_EDGE('',*,*,#37556,.F.) ;
#49532=ORIENTED_EDGE('',*,*,#37303,.F.) ;
#49533=ORIENTED_EDGE('',*,*,#37554,.T.) ;
#49534=ORIENTED_EDGE('',*,*,#37304,.F.) ;
#49535=ORIENTED_EDGE('',*,*,#37557,.F.) ;
#49536=ORIENTED_EDGE('',*,*,#37298,.F.) ;
#49537=ORIENTED_EDGE('',*,*,#37553,.T.) ;
#49538=ORIENTED_EDGE('',*,*,#37300,.F.) ;
#49539=ORIENTED_EDGE('',*,*,#37558,.F.) ;
#49540=ORIENTED_EDGE('',*,*,#37293,.F.) ;
#49541=ORIENTED_EDGE('',*,*,#37555,.T.) ;
#49542=ORIENTED_EDGE('',*,*,#37294,.F.) ;
#49543=ORIENTED_EDGE('',*,*,#37559,.F.) ;
#49544=ORIENTED_EDGE('',*,*,#37070,.F.) ;
#49545=ORIENTED_EDGE('',*,*,#37104,.F.) ;
#49546=ORIENTED_EDGE('',*,*,#37560,.T.) ;
#49547=ORIENTED_EDGE('',*,*,#37075,.F.) ;
#49548=ORIENTED_EDGE('',*,*,#37561,.F.) ;
#49549=ORIENTED_EDGE('',*,*,#37154,.F.) ;
#49550=ORIENTED_EDGE('',*,*,#37105,.F.) ;
#49551=ORIENTED_EDGE('',*,*,#37562,.F.) ;
#49552=ORIENTED_EDGE('',*,*,#37317,.F.) ;
#49553=ORIENTED_EDGE('',*,*,#37156,.F.) ;
#49554=ORIENTED_EDGE('',*,*,#37316,.F.) ;
#49555=ORIENTED_EDGE('',*,*,#37563,.F.) ;
#49556=ORIENTED_EDGE('',*,*,#37314,.F.) ;
#49557=ORIENTED_EDGE('',*,*,#37556,.T.) ;
#49558=ORIENTED_EDGE('',*,*,#37225,.T.) ;
#49559=ORIENTED_EDGE('',*,*,#37564,.F.) ;
#49560=ORIENTED_EDGE('',*,*,#37557,.T.) ;
#49561=ORIENTED_EDGE('',*,*,#37559,.T.) ;
#49562=ORIENTED_EDGE('',*,*,#37558,.T.) ;
#49563=ORIENTED_EDGE('',*,*,#37062,.F.) ;
#49564=ORIENTED_EDGE('',*,*,#37562,.T.) ;
#49565=ORIENTED_EDGE('',*,*,#37561,.T.) ;
#49566=ORIENTED_EDGE('',*,*,#37565,.F.) ;
#49567=ORIENTED_EDGE('',*,*,#37318,.T.) ;
#49568=ORIENTED_EDGE('',*,*,#37566,.F.) ;
#49569=ORIENTED_EDGE('',*,*,#37563,.T.) ;
#49570=ORIENTED_EDGE('',*,*,#37567,.F.) ;
#49571=ORIENTED_EDGE('',*,*,#37564,.T.) ;
#49572=ORIENTED_EDGE('',*,*,#37224,.F.) ;
#49573=ORIENTED_EDGE('',*,*,#37568,.F.) ;
#49574=ORIENTED_EDGE('',*,*,#37299,.F.) ;
#49575=ORIENTED_EDGE('',*,*,#37565,.T.) ;
#49576=ORIENTED_EDGE('',*,*,#37074,.F.) ;
#49577=ORIENTED_EDGE('',*,*,#37569,.F.) ;
#49578=ORIENTED_EDGE('',*,*,#37319,.F.) ;
#49579=ORIENTED_EDGE('',*,*,#37570,.F.) ;
#49580=ORIENTED_EDGE('',*,*,#37320,.F.) ;
#49581=ORIENTED_EDGE('',*,*,#37571,.F.) ;
#49582=ORIENTED_EDGE('',*,*,#37311,.F.) ;
#49583=ORIENTED_EDGE('',*,*,#37567,.T.) ;
#49584=ORIENTED_EDGE('',*,*,#37315,.F.) ;
#49585=ORIENTED_EDGE('',*,*,#37572,.F.) ;
#49586=ORIENTED_EDGE('',*,*,#37305,.F.) ;
#49587=ORIENTED_EDGE('',*,*,#37566,.T.) ;
#49588=ORIENTED_EDGE('',*,*,#37308,.F.) ;
#49589=ORIENTED_EDGE('',*,*,#37573,.F.) ;
#49590=ORIENTED_EDGE('',*,*,#37312,.F.) ;
#49591=ORIENTED_EDGE('',*,*,#37158,.F.) ;
#49592=ORIENTED_EDGE('',*,*,#37313,.F.) ;
#49593=ORIENTED_EDGE('',*,*,#37574,.F.) ;
#49594=ORIENTED_EDGE('',*,*,#37218,.F.) ;
#49595=ORIENTED_EDGE('',*,*,#37060,.T.) ;
#49596=ORIENTED_EDGE('',*,*,#37568,.T.) ;
#49597=ORIENTED_EDGE('',*,*,#37575,.F.) ;
#49598=ORIENTED_EDGE('',*,*,#37071,.T.) ;
#49599=ORIENTED_EDGE('',*,*,#37571,.T.) ;
#49600=ORIENTED_EDGE('',*,*,#37569,.T.) ;
#49601=ORIENTED_EDGE('',*,*,#37058,.F.) ;
#49602=ORIENTED_EDGE('',*,*,#37576,.F.) ;
#49603=ORIENTED_EDGE('',*,*,#37576,.T.) ;
#49604=ORIENTED_EDGE('',*,*,#37057,.F.) ;
#49605=ORIENTED_EDGE('',*,*,#37572,.T.) ;
#49606=ORIENTED_EDGE('',*,*,#37570,.T.) ;
#49607=ORIENTED_EDGE('',*,*,#37577,.F.) ;
#49608=ORIENTED_EDGE('',*,*,#37574,.T.) ;
#49609=ORIENTED_EDGE('',*,*,#37573,.T.) ;
#49610=ORIENTED_EDGE('',*,*,#37578,.F.) ;
#49611=ORIENTED_EDGE('',*,*,#37219,.T.) ;
#49612=ORIENTED_EDGE('',*,*,#37575,.T.) ;
#49613=ORIENTED_EDGE('',*,*,#37223,.F.) ;
#49614=ORIENTED_EDGE('',*,*,#37579,.F.) ;
#49615=ORIENTED_EDGE('',*,*,#37072,.F.) ;
#49616=ORIENTED_EDGE('',*,*,#37577,.T.) ;
#49617=ORIENTED_EDGE('',*,*,#37310,.F.) ;
#49618=ORIENTED_EDGE('',*,*,#37580,.F.) ;
#49619=ORIENTED_EDGE('',*,*,#37306,.F.) ;
#49620=ORIENTED_EDGE('',*,*,#37578,.T.) ;
#49621=ORIENTED_EDGE('',*,*,#37307,.F.) ;
#49622=ORIENTED_EDGE('',*,*,#37581,.F.) ;
#49623=ORIENTED_EDGE('',*,*,#37220,.F.) ;
#49624=ORIENTED_EDGE('',*,*,#37073,.T.) ;
#49625=ORIENTED_EDGE('',*,*,#37579,.T.) ;
#49626=ORIENTED_EDGE('',*,*,#37582,.F.) ;
#49627=ORIENTED_EDGE('',*,*,#37055,.T.) ;
#49628=ORIENTED_EDGE('',*,*,#37581,.T.) ;
#49629=ORIENTED_EDGE('',*,*,#37580,.T.) ;
#49630=ORIENTED_EDGE('',*,*,#37583,.F.) ;
#49631=ORIENTED_EDGE('',*,*,#37221,.T.) ;
#49632=ORIENTED_EDGE('',*,*,#37582,.T.) ;
#49633=ORIENTED_EDGE('',*,*,#37222,.F.) ;
#49634=ORIENTED_EDGE('',*,*,#37583,.T.) ;
#49635=ORIENTED_EDGE('',*,*,#37309,.F.) ;
#49636=ORIENTED_EDGE('',*,*,#37078,.F.) ;
#49637=ORIENTED_EDGE('',*,*,#37584,.T.) ;
#49638=ORIENTED_EDGE('',*,*,#37399,.F.) ;
#49639=ORIENTED_EDGE('',*,*,#37585,.F.) ;
#49640=ORIENTED_EDGE('',*,*,#37404,.F.) ;
#49641=ORIENTED_EDGE('',*,*,#37398,.F.) ;
#49642=ORIENTED_EDGE('',*,*,#37586,.T.) ;
#49643=ORIENTED_EDGE('',*,*,#37405,.F.) ;
#49644=ORIENTED_EDGE('',*,*,#37585,.T.) ;
#49645=ORIENTED_EDGE('',*,*,#37401,.F.) ;
#49646=ORIENTED_EDGE('',*,*,#37587,.T.) ;
#49647=ORIENTED_EDGE('',*,*,#37267,.F.) ;
#49648=ORIENTED_EDGE('',*,*,#37425,.F.) ;
#49649=ORIENTED_EDGE('',*,*,#37588,.F.) ;
#49650=ORIENTED_EDGE('',*,*,#37410,.F.) ;
#49651=ORIENTED_EDGE('',*,*,#37589,.T.) ;
#49652=ORIENTED_EDGE('',*,*,#37438,.F.) ;
#49653=ORIENTED_EDGE('',*,*,#37590,.F.) ;
#49654=ORIENTED_EDGE('',*,*,#37395,.F.) ;
#49655=ORIENTED_EDGE('',*,*,#37591,.T.) ;
#49656=ORIENTED_EDGE('',*,*,#37080,.F.) ;
#49657=ORIENTED_EDGE('',*,*,#37403,.F.) ;
#49658=ORIENTED_EDGE('',*,*,#37592,.F.) ;
#49659=ORIENTED_EDGE('',*,*,#37422,.F.) ;
#49660=ORIENTED_EDGE('',*,*,#37593,.T.) ;
#49661=ORIENTED_EDGE('',*,*,#37396,.F.) ;
#49662=ORIENTED_EDGE('',*,*,#37588,.T.) ;
#49663=ORIENTED_EDGE('',*,*,#37594,.F.) ;
#49664=ORIENTED_EDGE('',*,*,#37590,.T.) ;
#49665=ORIENTED_EDGE('',*,*,#37595,.F.) ;
#49666=ORIENTED_EDGE('',*,*,#37407,.F.) ;
#49667=ORIENTED_EDGE('',*,*,#37596,.T.) ;
#49668=ORIENTED_EDGE('',*,*,#37390,.F.) ;
#49669=ORIENTED_EDGE('',*,*,#37592,.T.) ;
#49670=ORIENTED_EDGE('',*,*,#37440,.F.) ;
#49671=ORIENTED_EDGE('',*,*,#37597,.T.) ;
#49672=ORIENTED_EDGE('',*,*,#37416,.F.) ;
#49673=ORIENTED_EDGE('',*,*,#37598,.F.) ;
#49674=ORIENTED_EDGE('',*,*,#37595,.T.) ;
#49675=ORIENTED_EDGE('',*,*,#37441,.F.) ;
#49676=ORIENTED_EDGE('',*,*,#37599,.F.) ;
#49677=ORIENTED_EDGE('',*,*,#37415,.F.) ;
#49678=ORIENTED_EDGE('',*,*,#37594,.T.) ;
#49679=ORIENTED_EDGE('',*,*,#37414,.F.) ;
#49680=ORIENTED_EDGE('',*,*,#37600,.F.) ;
#49681=ORIENTED_EDGE('',*,*,#37411,.F.) ;
#49682=ORIENTED_EDGE('',*,*,#37436,.F.) ;
#49683=ORIENTED_EDGE('',*,*,#37601,.T.) ;
#49684=ORIENTED_EDGE('',*,*,#37408,.F.) ;
#49685=ORIENTED_EDGE('',*,*,#37602,.F.) ;
#49686=ORIENTED_EDGE('',*,*,#37599,.T.) ;
#49687=ORIENTED_EDGE('',*,*,#37598,.T.) ;
#49688=ORIENTED_EDGE('',*,*,#37603,.F.) ;
#49689=ORIENTED_EDGE('',*,*,#37602,.T.) ;
#49690=ORIENTED_EDGE('',*,*,#37600,.T.) ;
#49691=ORIENTED_EDGE('',*,*,#37604,.F.) ;
#49692=ORIENTED_EDGE('',*,*,#37603,.T.) ;
#49693=ORIENTED_EDGE('',*,*,#37419,.F.) ;
#49694=ORIENTED_EDGE('',*,*,#37605,.F.) ;
#49695=ORIENTED_EDGE('',*,*,#37412,.F.) ;
#49696=ORIENTED_EDGE('',*,*,#37604,.T.) ;
#49697=ORIENTED_EDGE('',*,*,#37413,.F.) ;
#49698=ORIENTED_EDGE('',*,*,#37606,.F.) ;
#49699=ORIENTED_EDGE('',*,*,#37437,.F.) ;
#49700=ORIENTED_EDGE('',*,*,#37606,.T.) ;
#49701=ORIENTED_EDGE('',*,*,#37605,.T.) ;
#49702=ORIENTED_EDGE('',*,*,#37607,.F.) ;
#49703=ORIENTED_EDGE('',*,*,#37418,.F.) ;
#49704=ORIENTED_EDGE('',*,*,#37608,.T.) ;
#49705=ORIENTED_EDGE('',*,*,#37434,.F.) ;
#49706=ORIENTED_EDGE('',*,*,#37607,.T.) ;
#49707=ORIENTED_EDGE('',*,*,#37392,.F.) ;
#49708=ORIENTED_EDGE('',*,*,#37609,.T.) ;
#49709=ORIENTED_EDGE('',*,*,#37420,.F.) ;
#49710=ORIENTED_EDGE('',*,*,#37610,.F.) ;
#49711=ORIENTED_EDGE('',*,*,#37271,.F.) ;
#49712=ORIENTED_EDGE('',*,*,#37611,.T.) ;
#49713=ORIENTED_EDGE('',*,*,#37393,.F.) ;
#49714=ORIENTED_EDGE('',*,*,#37610,.T.) ;
#49715=ORIENTED_EDGE('',*,*,#37424,.F.) ;
#49716=ORIENTED_EDGE('',*,*,#37383,.F.) ;
#49717=ORIENTED_EDGE('',*,*,#37612,.T.) ;
#49718=ORIENTED_EDGE('',*,*,#37384,.F.) ;
#49719=ORIENTED_EDGE('',*,*,#37286,.F.) ;
#49720=ORIENTED_EDGE('',*,*,#37389,.F.) ;
#49721=ORIENTED_EDGE('',*,*,#37613,.T.) ;
#49722=ORIENTED_EDGE('',*,*,#37381,.F.) ;
#49723=ORIENTED_EDGE('',*,*,#37284,.F.) ;
#49724=ORIENTED_EDGE('',*,*,#37368,.F.) ;
#49725=ORIENTED_EDGE('',*,*,#37614,.T.) ;
#49726=ORIENTED_EDGE('',*,*,#37426,.F.) ;
#49727=ORIENTED_EDGE('',*,*,#37615,.F.) ;
#49728=ORIENTED_EDGE('',*,*,#37428,.F.) ;
#49729=ORIENTED_EDGE('',*,*,#37616,.T.) ;
#49730=ORIENTED_EDGE('',*,*,#37374,.F.) ;
#49731=ORIENTED_EDGE('',*,*,#37617,.F.) ;
#49732=ORIENTED_EDGE('',*,*,#37618,.F.) ;
#49733=ORIENTED_EDGE('',*,*,#37429,.F.) ;
#49734=ORIENTED_EDGE('',*,*,#37619,.F.) ;
#49735=ORIENTED_EDGE('',*,*,#37373,.F.) ;
#49736=ORIENTED_EDGE('',*,*,#37615,.T.) ;
#49737=ORIENTED_EDGE('',*,*,#37618,.T.) ;
#49738=ORIENTED_EDGE('',*,*,#37620,.F.) ;
#49739=ORIENTED_EDGE('',*,*,#37386,.F.) ;
#49740=ORIENTED_EDGE('',*,*,#37621,.T.) ;
#49741=ORIENTED_EDGE('',*,*,#37378,.F.) ;
#49742=ORIENTED_EDGE('',*,*,#37288,.F.) ;
#49743=ORIENTED_EDGE('',*,*,#37380,.F.) ;
#49744=ORIENTED_EDGE('',*,*,#37622,.T.) ;
#49745=ORIENTED_EDGE('',*,*,#37387,.F.) ;
#49746=ORIENTED_EDGE('',*,*,#37282,.F.) ;
#49747=ORIENTED_EDGE('',*,*,#37619,.T.) ;
#49748=ORIENTED_EDGE('',*,*,#37617,.T.) ;
#49749=ORIENTED_EDGE('',*,*,#37623,.F.) ;
#49750=ORIENTED_EDGE('',*,*,#37620,.T.) ;
#49751=ORIENTED_EDGE('',*,*,#37372,.F.) ;
#49752=ORIENTED_EDGE('',*,*,#37624,.F.) ;
#49753=ORIENTED_EDGE('',*,*,#37369,.F.) ;
#49754=ORIENTED_EDGE('',*,*,#37432,.F.) ;
#49755=ORIENTED_EDGE('',*,*,#37625,.T.) ;
#49756=ORIENTED_EDGE('',*,*,#37366,.F.) ;
#49757=ORIENTED_EDGE('',*,*,#37626,.F.) ;
#49758=ORIENTED_EDGE('',*,*,#37376,.F.) ;
#49759=ORIENTED_EDGE('',*,*,#37627,.T.) ;
#49760=ORIENTED_EDGE('',*,*,#37430,.F.) ;
#49761=ORIENTED_EDGE('',*,*,#37628,.F.) ;
#49762=ORIENTED_EDGE('',*,*,#37623,.T.) ;
#49763=ORIENTED_EDGE('',*,*,#37377,.F.) ;
#49764=ORIENTED_EDGE('',*,*,#37629,.F.) ;
#49765=ORIENTED_EDGE('',*,*,#37370,.F.) ;
#49766=ORIENTED_EDGE('',*,*,#37626,.T.) ;
#49767=ORIENTED_EDGE('',*,*,#37624,.T.) ;
#49768=ORIENTED_EDGE('',*,*,#37630,.F.) ;
#49769=ORIENTED_EDGE('',*,*,#37629,.T.) ;
#49770=ORIENTED_EDGE('',*,*,#37628,.T.) ;
#49771=ORIENTED_EDGE('',*,*,#37631,.F.) ;
#49772=ORIENTED_EDGE('',*,*,#37630,.T.) ;
#49773=ORIENTED_EDGE('',*,*,#37371,.F.) ;
#49774=ORIENTED_EDGE('',*,*,#37631,.T.) ;
#49775=ORIENTED_EDGE('',*,*,#37433,.F.) ;
#49776=ORIENTED_EDGE('',*,*,#37115,.F.) ;
#49777=ORIENTED_EDGE('',*,*,#37091,.F.) ;
#49778=ORIENTED_EDGE('',*,*,#37632,.F.) ;
#49779=ORIENTED_EDGE('',*,*,#37097,.F.) ;
#49780=ORIENTED_EDGE('',*,*,#37353,.F.) ;
#49781=ORIENTED_EDGE('',*,*,#37633,.T.) ;
#49782=ORIENTED_EDGE('',*,*,#37092,.F.) ;
#49783=ORIENTED_EDGE('',*,*,#37634,.F.) ;
#49784=ORIENTED_EDGE('',*,*,#37634,.T.) ;
#49785=ORIENTED_EDGE('',*,*,#37632,.T.) ;
#49786=ORIENTED_EDGE('',*,*,#37635,.F.) ;
#49787=ORIENTED_EDGE('',*,*,#37114,.F.) ;
#49788=ORIENTED_EDGE('',*,*,#37087,.F.) ;
#49789=ORIENTED_EDGE('',*,*,#37636,.F.) ;
#49790=ORIENTED_EDGE('',*,*,#37089,.F.) ;
#49791=ORIENTED_EDGE('',*,*,#37635,.T.) ;
#49792=ORIENTED_EDGE('',*,*,#37090,.F.) ;
#49793=ORIENTED_EDGE('',*,*,#37637,.F.) ;
#49794=ORIENTED_EDGE('',*,*,#37354,.F.) ;
#49795=ORIENTED_EDGE('',*,*,#37637,.T.) ;
#49796=ORIENTED_EDGE('',*,*,#37636,.T.) ;
#49797=ORIENTED_EDGE('',*,*,#37638,.F.) ;
#49798=ORIENTED_EDGE('',*,*,#37086,.F.) ;
#49799=ORIENTED_EDGE('',*,*,#37639,.T.) ;
#49800=ORIENTED_EDGE('',*,*,#37351,.F.) ;
#49801=ORIENTED_EDGE('',*,*,#37638,.T.) ;
#49802=ORIENTED_EDGE('',*,*,#37190,.F.) ;
#49803=ORIENTED_EDGE('',*,*,#37042,.T.) ;
#49804=ORIENTED_EDGE('',*,*,#37640,.T.) ;
#49805=ORIENTED_EDGE('',*,*,#37362,.F.) ;
#49806=ORIENTED_EDGE('',*,*,#37641,.F.) ;
#49807=ORIENTED_EDGE('',*,*,#37168,.F.) ;
#49808=ORIENTED_EDGE('',*,*,#37191,.F.) ;
#49809=ORIENTED_EDGE('',*,*,#37642,.F.) ;
#49810=ORIENTED_EDGE('',*,*,#37188,.F.) ;
#49811=ORIENTED_EDGE('',*,*,#37642,.T.) ;
#49812=ORIENTED_EDGE('',*,*,#37641,.T.) ;
#49813=ORIENTED_EDGE('',*,*,#37643,.F.) ;
#49814=ORIENTED_EDGE('',*,*,#37643,.T.) ;
#49815=ORIENTED_EDGE('',*,*,#37365,.F.) ;
#49816=ORIENTED_EDGE('',*,*,#37644,.F.) ;
#49817=ORIENTED_EDGE('',*,*,#37186,.F.) ;
#49818=ORIENTED_EDGE('',*,*,#37170,.F.) ;
#49819=ORIENTED_EDGE('',*,*,#37187,.F.) ;
#49820=ORIENTED_EDGE('',*,*,#37645,.F.) ;
#49821=ORIENTED_EDGE('',*,*,#37184,.F.) ;
#49822=ORIENTED_EDGE('',*,*,#37645,.T.) ;
#49823=ORIENTED_EDGE('',*,*,#37644,.T.) ;
#49824=ORIENTED_EDGE('',*,*,#37646,.F.) ;
#49825=ORIENTED_EDGE('',*,*,#37364,.F.) ;
#49826=ORIENTED_EDGE('',*,*,#37046,.T.) ;
#49827=ORIENTED_EDGE('',*,*,#37647,.T.) ;
#49828=ORIENTED_EDGE('',*,*,#37185,.F.) ;
#49829=ORIENTED_EDGE('',*,*,#37646,.T.) ;
#49830=ORIENTED_EDGE('',*,*,#37265,.F.) ;
#49831=ORIENTED_EDGE('',*,*,#37648,.T.) ;
#49832=ORIENTED_EDGE('',*,*,#37076,.F.) ;
#49833=ORIENTED_EDGE('',*,*,#37649,.T.) ;
#49834=ORIENTED_EDGE('',*,*,#37135,.F.) ;
#49835=ORIENTED_EDGE('',*,*,#37237,.F.) ;
#49836=ORIENTED_EDGE('',*,*,#37147,.F.) ;
#49837=ORIENTED_EDGE('',*,*,#37171,.F.) ;
#49838=ORIENTED_EDGE('',*,*,#37137,.F.) ;
#49839=ORIENTED_EDGE('',*,*,#37172,.F.) ;
#49840=ORIENTED_EDGE('',*,*,#37145,.F.) ;
#49841=ORIENTED_EDGE('',*,*,#37173,.F.) ;
#49842=ORIENTED_EDGE('',*,*,#37139,.F.) ;
#49843=ORIENTED_EDGE('',*,*,#37174,.F.) ;
#49844=ORIENTED_EDGE('',*,*,#37143,.F.) ;
#49845=ORIENTED_EDGE('',*,*,#37177,.F.) ;
#49846=ORIENTED_EDGE('',*,*,#37132,.F.) ;
#49847=ORIENTED_EDGE('',*,*,#37107,.F.) ;
#49848=ORIENTED_EDGE('',*,*,#37150,.F.) ;
#49849=ORIENTED_EDGE('',*,*,#37230,.F.) ;
#49850=ORIENTED_EDGE('',*,*,#37450,.F.) ;
#49851=ORIENTED_EDGE('',*,*,#37650,.T.) ;
#49852=ORIENTED_EDGE('',*,*,#37109,.F.) ;
#49853=ORIENTED_EDGE('',*,*,#37131,.F.) ;
#49854=ORIENTED_EDGE('',*,*,#37445,.F.) ;
#49855=ORIENTED_EDGE('',*,*,#37651,.T.) ;
#49856=ORIENTED_EDGE('',*,*,#37110,.F.) ;
#49857=ORIENTED_EDGE('',*,*,#37652,.T.) ;
#49858=ORIENTED_EDGE('',*,*,#37111,.F.) ;
#49859=ORIENTED_EDGE('',*,*,#37653,.T.) ;
#49860=ORIENTED_EDGE('',*,*,#37442,.F.) ;
#49861=ORIENTED_EDGE('',*,*,#37151,.F.) ;
#49862=ORIENTED_EDGE('',*,*,#37490,.F.) ;
#49863=ORIENTED_EDGE('',*,*,#37496,.F.) ;
#49864=ORIENTED_EDGE('',*,*,#37495,.F.) ;
#49865=ORIENTED_EDGE('',*,*,#37654,.F.) ;
#49866=ORIENTED_EDGE('',*,*,#37491,.F.) ;
#49867=ORIENTED_EDGE('',*,*,#37584,.F.) ;
#49868=ORIENTED_EDGE('',*,*,#37077,.F.) ;
#49869=ORIENTED_EDGE('',*,*,#37655,.F.) ;
#49870=ORIENTED_EDGE('',*,*,#37259,.F.) ;
#49871=ORIENTED_EDGE('',*,*,#37654,.T.) ;
#49872=ORIENTED_EDGE('',*,*,#37268,.F.) ;
#49873=ORIENTED_EDGE('',*,*,#37587,.F.) ;
#49874=ORIENTED_EDGE('',*,*,#37400,.F.) ;
#49875=ORIENTED_EDGE('',*,*,#37655,.T.) ;
#49876=ORIENTED_EDGE('',*,*,#37648,.F.) ;
#49877=ORIENTED_EDGE('',*,*,#37656,.F.) ;
#49878=ORIENTED_EDGE('',*,*,#37656,.T.) ;
#49879=ORIENTED_EDGE('',*,*,#37264,.F.) ;
#49880=ORIENTED_EDGE('',*,*,#37657,.F.) ;
#49881=ORIENTED_EDGE('',*,*,#37260,.F.) ;
#49882=ORIENTED_EDGE('',*,*,#37499,.F.) ;
#49883=ORIENTED_EDGE('',*,*,#37493,.F.) ;
#49884=ORIENTED_EDGE('',*,*,#37492,.F.) ;
#49885=ORIENTED_EDGE('',*,*,#37657,.T.) ;
#49886=ORIENTED_EDGE('',*,*,#37500,.F.) ;
#49887=ORIENTED_EDGE('',*,*,#37512,.F.) ;
#49888=ORIENTED_EDGE('',*,*,#37502,.F.) ;
#49889=ORIENTED_EDGE('',*,*,#37501,.F.) ;
#49890=ORIENTED_EDGE('',*,*,#37658,.F.) ;
#49891=ORIENTED_EDGE('',*,*,#37513,.F.) ;
#49892=ORIENTED_EDGE('',*,*,#37658,.T.) ;
#49893=ORIENTED_EDGE('',*,*,#37266,.F.) ;
#49894=ORIENTED_EDGE('',*,*,#37659,.F.) ;
#49895=ORIENTED_EDGE('',*,*,#37256,.F.) ;
#49896=ORIENTED_EDGE('',*,*,#37659,.T.) ;
#49897=ORIENTED_EDGE('',*,*,#37649,.F.) ;
#49898=ORIENTED_EDGE('',*,*,#37660,.F.) ;
#49899=ORIENTED_EDGE('',*,*,#37611,.F.) ;
#49900=ORIENTED_EDGE('',*,*,#37270,.F.) ;
#49901=ORIENTED_EDGE('',*,*,#37661,.F.) ;
#49902=ORIENTED_EDGE('',*,*,#37257,.F.) ;
#49903=ORIENTED_EDGE('',*,*,#37660,.T.) ;
#49904=ORIENTED_EDGE('',*,*,#37081,.F.) ;
#49905=ORIENTED_EDGE('',*,*,#37591,.F.) ;
#49906=ORIENTED_EDGE('',*,*,#37394,.F.) ;
#49907=ORIENTED_EDGE('',*,*,#37661,.T.) ;
#49908=ORIENTED_EDGE('',*,*,#37498,.F.) ;
#49909=ORIENTED_EDGE('',*,*,#37497,.F.) ;
#49910=ORIENTED_EDGE('',*,*,#37510,.F.) ;
#49911=ORIENTED_EDGE('',*,*,#37509,.F.) ;
#49912=ORIENTED_EDGE('',*,*,#37085,.F.) ;
#49913=ORIENTED_EDGE('',*,*,#37662,.T.) ;
#49914=ORIENTED_EDGE('',*,*,#37355,.F.) ;
#49915=ORIENTED_EDGE('',*,*,#37663,.F.) ;
#49916=ORIENTED_EDGE('',*,*,#37639,.F.) ;
#49917=ORIENTED_EDGE('',*,*,#37663,.T.) ;
#49918=ORIENTED_EDGE('',*,*,#37361,.F.) ;
#49919=ORIENTED_EDGE('',*,*,#37664,.F.) ;
#49920=ORIENTED_EDGE('',*,*,#37352,.F.) ;
#49921=ORIENTED_EDGE('',*,*,#37664,.T.) ;
#49922=ORIENTED_EDGE('',*,*,#37360,.F.) ;
#49923=ORIENTED_EDGE('',*,*,#37665,.F.) ;
#49924=ORIENTED_EDGE('',*,*,#37666,.F.) ;
#49925=ORIENTED_EDGE('',*,*,#37667,.F.) ;
#49926=ORIENTED_EDGE('',*,*,#37668,.F.) ;
#49927=ORIENTED_EDGE('',*,*,#37093,.F.) ;
#49928=ORIENTED_EDGE('',*,*,#37633,.F.) ;
#49929=ORIENTED_EDGE('',*,*,#37116,.F.) ;
#49930=ORIENTED_EDGE('',*,*,#37095,.F.) ;
#49931=ORIENTED_EDGE('',*,*,#37669,.F.) ;
#49932=ORIENTED_EDGE('',*,*,#37193,.F.) ;
#49933=ORIENTED_EDGE('',*,*,#37094,.F.) ;
#49934=ORIENTED_EDGE('',*,*,#37668,.T.) ;
#49935=ORIENTED_EDGE('',*,*,#37667,.T.) ;
#49936=ORIENTED_EDGE('',*,*,#37666,.T.) ;
#49937=ORIENTED_EDGE('',*,*,#37665,.T.) ;
#49938=ORIENTED_EDGE('',*,*,#37670,.F.) ;
#49939=ORIENTED_EDGE('',*,*,#37194,.F.) ;
#49940=ORIENTED_EDGE('',*,*,#37669,.T.) ;
#49941=ORIENTED_EDGE('',*,*,#37045,.F.) ;
#49942=ORIENTED_EDGE('',*,*,#37671,.T.) ;
#49943=ORIENTED_EDGE('',*,*,#37181,.F.) ;
#49944=ORIENTED_EDGE('',*,*,#37647,.F.) ;
#49945=ORIENTED_EDGE('',*,*,#37670,.T.) ;
#49946=ORIENTED_EDGE('',*,*,#37359,.F.) ;
#49947=ORIENTED_EDGE('',*,*,#37672,.F.) ;
#49948=ORIENTED_EDGE('',*,*,#37195,.F.) ;
#49949=ORIENTED_EDGE('',*,*,#37166,.F.) ;
#49950=ORIENTED_EDGE('',*,*,#37197,.F.) ;
#49951=ORIENTED_EDGE('',*,*,#37673,.F.) ;
#49952=ORIENTED_EDGE('',*,*,#37192,.F.) ;
#49953=ORIENTED_EDGE('',*,*,#37047,.T.) ;
#49954=ORIENTED_EDGE('',*,*,#37363,.F.) ;
#49955=ORIENTED_EDGE('',*,*,#37674,.F.) ;
#49956=ORIENTED_EDGE('',*,*,#37357,.F.) ;
#49957=ORIENTED_EDGE('',*,*,#37196,.F.) ;
#49958=ORIENTED_EDGE('',*,*,#37672,.T.) ;
#49959=ORIENTED_EDGE('',*,*,#37675,.F.) ;
#49960=ORIENTED_EDGE('',*,*,#37676,.F.) ;
#49961=ORIENTED_EDGE('',*,*,#37677,.F.) ;
#49962=ORIENTED_EDGE('',*,*,#37040,.F.) ;
#49963=ORIENTED_EDGE('',*,*,#37039,.F.) ;
#49964=ORIENTED_EDGE('',*,*,#37189,.F.) ;
#49965=ORIENTED_EDGE('',*,*,#37673,.T.) ;
#49966=ORIENTED_EDGE('',*,*,#37041,.F.) ;
#49967=ORIENTED_EDGE('',*,*,#37677,.T.) ;
#49968=ORIENTED_EDGE('',*,*,#37676,.T.) ;
#49969=ORIENTED_EDGE('',*,*,#37675,.T.) ;
#49970=ORIENTED_EDGE('',*,*,#37358,.F.) ;
#49971=ORIENTED_EDGE('',*,*,#37674,.T.) ;
#49972=ORIENTED_EDGE('',*,*,#37640,.F.) ;
#49973=ORIENTED_EDGE('',*,*,#37678,.F.) ;
#49974=ORIENTED_EDGE('',*,*,#37103,.F.) ;
#49975=ORIENTED_EDGE('',*,*,#37153,.F.) ;
#49976=ORIENTED_EDGE('',*,*,#37444,.F.) ;
#49977=ORIENTED_EDGE('',*,*,#37560,.F.) ;
#49978=ORIENTED_EDGE('',*,*,#37678,.T.) ;
#49979=ORIENTED_EDGE('',*,*,#37679,.F.) ;
#49980=ORIENTED_EDGE('',*,*,#37065,.F.) ;
#49981=ORIENTED_EDGE('',*,*,#37679,.T.) ;
#49982=ORIENTED_EDGE('',*,*,#37443,.F.) ;
#49983=ORIENTED_EDGE('',*,*,#37680,.F.) ;
#49984=ORIENTED_EDGE('',*,*,#37447,.F.) ;
#49985=ORIENTED_EDGE('',*,*,#37653,.F.) ;
#49986=ORIENTED_EDGE('',*,*,#37651,.F.) ;
#49987=ORIENTED_EDGE('',*,*,#37680,.T.) ;
#49988=ORIENTED_EDGE('',*,*,#37681,.T.) ;
#49989=ORIENTED_EDGE('',*,*,#37586,.F.) ;
#49990=ORIENTED_EDGE('',*,*,#37682,.F.) ;
#49991=ORIENTED_EDGE('',*,*,#37589,.F.) ;
#49992=ORIENTED_EDGE('',*,*,#37681,.F.) ;
#49993=ORIENTED_EDGE('',*,*,#37409,.F.) ;
#49994=ORIENTED_EDGE('',*,*,#37683,.F.) ;
#49995=ORIENTED_EDGE('',*,*,#37406,.F.) ;
#49996=ORIENTED_EDGE('',*,*,#37682,.T.) ;
#49997=ORIENTED_EDGE('',*,*,#37397,.F.) ;
#49998=ORIENTED_EDGE('',*,*,#37684,.F.) ;
#49999=ORIENTED_EDGE('',*,*,#37439,.F.) ;
#50000=ORIENTED_EDGE('',*,*,#37683,.T.) ;
#50001=ORIENTED_EDGE('',*,*,#37601,.F.) ;
#50002=ORIENTED_EDGE('',*,*,#37685,.F.) ;
#50003=ORIENTED_EDGE('',*,*,#37596,.F.) ;
#50004=ORIENTED_EDGE('',*,*,#37684,.T.) ;
#50005=ORIENTED_EDGE('',*,*,#37593,.F.) ;
#50006=ORIENTED_EDGE('',*,*,#37686,.F.) ;
#50007=ORIENTED_EDGE('',*,*,#37597,.F.) ;
#50008=ORIENTED_EDGE('',*,*,#37685,.T.) ;
#50009=ORIENTED_EDGE('',*,*,#37435,.F.) ;
#50010=ORIENTED_EDGE('',*,*,#37687,.F.) ;
#50011=ORIENTED_EDGE('',*,*,#37391,.F.) ;
#50012=ORIENTED_EDGE('',*,*,#37686,.T.) ;
#50013=ORIENTED_EDGE('',*,*,#37421,.F.) ;
#50014=ORIENTED_EDGE('',*,*,#37688,.F.) ;
#50015=ORIENTED_EDGE('',*,*,#37417,.F.) ;
#50016=ORIENTED_EDGE('',*,*,#37687,.T.) ;
#50017=ORIENTED_EDGE('',*,*,#37608,.F.) ;
#50018=ORIENTED_EDGE('',*,*,#37688,.T.) ;
#50019=ORIENTED_EDGE('',*,*,#37609,.F.) ;
#50020=ORIENTED_EDGE('',*,*,#37689,.T.) ;
#50021=ORIENTED_EDGE('',*,*,#37612,.F.) ;
#50022=ORIENTED_EDGE('',*,*,#37690,.F.) ;
#50023=ORIENTED_EDGE('',*,*,#37614,.F.) ;
#50024=ORIENTED_EDGE('',*,*,#37689,.F.) ;
#50025=ORIENTED_EDGE('',*,*,#37367,.F.) ;
#50026=ORIENTED_EDGE('',*,*,#37691,.F.) ;
#50027=ORIENTED_EDGE('',*,*,#37385,.F.) ;
#50028=ORIENTED_EDGE('',*,*,#37690,.T.) ;
#50029=ORIENTED_EDGE('',*,*,#37382,.F.) ;
#50030=ORIENTED_EDGE('',*,*,#37692,.F.) ;
#50031=ORIENTED_EDGE('',*,*,#37427,.F.) ;
#50032=ORIENTED_EDGE('',*,*,#37691,.T.) ;
#50033=ORIENTED_EDGE('',*,*,#37625,.F.) ;
#50034=ORIENTED_EDGE('',*,*,#37693,.F.) ;
#50035=ORIENTED_EDGE('',*,*,#37621,.F.) ;
#50036=ORIENTED_EDGE('',*,*,#37692,.T.) ;
#50037=ORIENTED_EDGE('',*,*,#37613,.F.) ;
#50038=ORIENTED_EDGE('',*,*,#37694,.F.) ;
#50039=ORIENTED_EDGE('',*,*,#37616,.F.) ;
#50040=ORIENTED_EDGE('',*,*,#37693,.T.) ;
#50041=ORIENTED_EDGE('',*,*,#37431,.F.) ;
#50042=ORIENTED_EDGE('',*,*,#37695,.F.) ;
#50043=ORIENTED_EDGE('',*,*,#37379,.F.) ;
#50044=ORIENTED_EDGE('',*,*,#37694,.T.) ;
#50045=ORIENTED_EDGE('',*,*,#37388,.F.) ;
#50046=ORIENTED_EDGE('',*,*,#37696,.F.) ;
#50047=ORIENTED_EDGE('',*,*,#37375,.F.) ;
#50048=ORIENTED_EDGE('',*,*,#37695,.T.) ;
#50049=ORIENTED_EDGE('',*,*,#37627,.F.) ;
#50050=ORIENTED_EDGE('',*,*,#37696,.T.) ;
#50051=ORIENTED_EDGE('',*,*,#37622,.F.) ;
#50052=ORIENTED_EDGE('',*,*,#37129,.F.) ;
#50053=ORIENTED_EDGE('',*,*,#37099,.F.) ;
#50054=ORIENTED_EDGE('',*,*,#37697,.F.) ;
#50055=ORIENTED_EDGE('',*,*,#37448,.F.) ;
#50056=ORIENTED_EDGE('',*,*,#37697,.T.) ;
#50057=ORIENTED_EDGE('',*,*,#37550,.F.) ;
#50058=ORIENTED_EDGE('',*,*,#37067,.F.) ;
#50059=ORIENTED_EDGE('',*,*,#37698,.F.) ;
#50060=ORIENTED_EDGE('',*,*,#37698,.T.) ;
#50061=ORIENTED_EDGE('',*,*,#37446,.F.) ;
#50062=ORIENTED_EDGE('',*,*,#37699,.F.) ;
#50063=ORIENTED_EDGE('',*,*,#37449,.F.) ;
#50064=ORIENTED_EDGE('',*,*,#37652,.F.) ;
#50065=ORIENTED_EDGE('',*,*,#37650,.F.) ;
#50066=ORIENTED_EDGE('',*,*,#37699,.T.) ;
#50067=ORIENTED_EDGE('',*,*,#37183,.F.) ;
#50068=ORIENTED_EDGE('',*,*,#37700,.F.) ;
#50069=ORIENTED_EDGE('',*,*,#37178,.F.) ;
#50070=ORIENTED_EDGE('',*,*,#37141,.F.) ;
#50071=ORIENTED_EDGE('',*,*,#37182,.F.) ;
#50072=ORIENTED_EDGE('',*,*,#37671,.F.) ;
#50073=ORIENTED_EDGE('',*,*,#37044,.F.) ;
#50074=ORIENTED_EDGE('',*,*,#37701,.F.) ;
#50075=ORIENTED_EDGE('',*,*,#37179,.F.) ;
#50076=ORIENTED_EDGE('',*,*,#37700,.T.) ;
#50077=ORIENTED_EDGE('',*,*,#37701,.T.) ;
#50078=ORIENTED_EDGE('',*,*,#37356,.F.) ;
#50079=ORIENTED_EDGE('',*,*,#37702,.F.) ;
#50080=ORIENTED_EDGE('',*,*,#37180,.F.) ;
#50081=ORIENTED_EDGE('',*,*,#37662,.F.) ;
#50082=ORIENTED_EDGE('',*,*,#37084,.F.) ;
#50083=ORIENTED_EDGE('',*,*,#37703,.F.) ;
#50084=ORIENTED_EDGE('',*,*,#37175,.F.) ;
#50085=ORIENTED_EDGE('',*,*,#37702,.T.) ;
#50086=ORIENTED_EDGE('',*,*,#37113,.F.) ;
#50087=ORIENTED_EDGE('',*,*,#37176,.F.) ;
#50088=ORIENTED_EDGE('',*,*,#37703,.T.) ;
#50089=ORIENTED_EDGE('',*,*,#37083,.F.) ;
#50090=ORIENTED_EDGE('',*,*,#37704,.T.) ;
#50091=ORIENTED_EDGE('',*,*,#37705,.T.) ;
#50092=ORIENTED_EDGE('',*,*,#37706,.T.) ;
#50093=ORIENTED_EDGE('',*,*,#37707,.F.) ;
#50094=ORIENTED_EDGE('',*,*,#37708,.F.) ;
#50095=ORIENTED_EDGE('',*,*,#37709,.T.) ;
#50096=ORIENTED_EDGE('',*,*,#37710,.T.) ;
#50097=ORIENTED_EDGE('',*,*,#37711,.F.) ;
#50098=ORIENTED_EDGE('',*,*,#37712,.F.) ;
#50099=ORIENTED_EDGE('',*,*,#37713,.F.) ;
#50100=ORIENTED_EDGE('',*,*,#37714,.F.) ;
#50101=ORIENTED_EDGE('',*,*,#37715,.T.) ;
#50102=ORIENTED_EDGE('',*,*,#37716,.F.) ;
#50103=ORIENTED_EDGE('',*,*,#37715,.F.) ;
#50104=ORIENTED_EDGE('',*,*,#37717,.F.) ;
#50105=ORIENTED_EDGE('',*,*,#37718,.T.) ;
#50106=ORIENTED_EDGE('',*,*,#37719,.F.) ;
#50107=ORIENTED_EDGE('',*,*,#37718,.F.) ;
#50108=ORIENTED_EDGE('',*,*,#37720,.F.) ;
#50109=ORIENTED_EDGE('',*,*,#37721,.F.) ;
#50110=ORIENTED_EDGE('',*,*,#37722,.T.) ;
#50111=ORIENTED_EDGE('',*,*,#37723,.T.) ;
#50112=ORIENTED_EDGE('',*,*,#37724,.F.) ;
#50113=ORIENTED_EDGE('',*,*,#37725,.F.) ;
#50114=ORIENTED_EDGE('',*,*,#37726,.F.) ;
#50115=ORIENTED_EDGE('',*,*,#37727,.T.) ;
#50116=ORIENTED_EDGE('',*,*,#37728,.F.) ;
#50117=ORIENTED_EDGE('',*,*,#37729,.F.) ;
#50118=ORIENTED_EDGE('',*,*,#37730,.T.) ;
#50119=ORIENTED_EDGE('',*,*,#37731,.F.) ;
#50120=ORIENTED_EDGE('',*,*,#37732,.T.) ;
#50121=ORIENTED_EDGE('',*,*,#37716,.T.) ;
#50122=ORIENTED_EDGE('',*,*,#37733,.T.) ;
#50123=ORIENTED_EDGE('',*,*,#37717,.T.) ;
#50124=ORIENTED_EDGE('',*,*,#37733,.F.) ;
#50125=ORIENTED_EDGE('',*,*,#37729,.T.) ;
#50126=ORIENTED_EDGE('',*,*,#37734,.T.) ;
#50127=ORIENTED_EDGE('',*,*,#37735,.T.) ;
#50128=ORIENTED_EDGE('',*,*,#37726,.T.) ;
#50129=ORIENTED_EDGE('',*,*,#37736,.F.) ;
#50130=ORIENTED_EDGE('',*,*,#37737,.T.) ;
#50131=ORIENTED_EDGE('',*,*,#37738,.F.) ;
#50132=ORIENTED_EDGE('',*,*,#37724,.T.) ;
#50133=ORIENTED_EDGE('',*,*,#37739,.T.) ;
#50134=ORIENTED_EDGE('',*,*,#37740,.T.) ;
#50135=ORIENTED_EDGE('',*,*,#37741,.T.) ;
#50136=ORIENTED_EDGE('',*,*,#37742,.T.) ;
#50137=ORIENTED_EDGE('',*,*,#37743,.T.) ;
#50138=ORIENTED_EDGE('',*,*,#37744,.T.) ;
#50139=ORIENTED_EDGE('',*,*,#37745,.T.) ;
#50140=ORIENTED_EDGE('',*,*,#37746,.T.) ;
#50141=ORIENTED_EDGE('',*,*,#37747,.T.) ;
#50142=ORIENTED_EDGE('',*,*,#37748,.T.) ;
#50143=ORIENTED_EDGE('',*,*,#37749,.T.) ;
#50144=ORIENTED_EDGE('',*,*,#37750,.T.) ;
#50145=ORIENTED_EDGE('',*,*,#37751,.T.) ;
#50146=ORIENTED_EDGE('',*,*,#37752,.T.) ;
#50147=ORIENTED_EDGE('',*,*,#37753,.T.) ;
#50148=ORIENTED_EDGE('',*,*,#37754,.T.) ;
#50149=ORIENTED_EDGE('',*,*,#37755,.T.) ;
#50150=ORIENTED_EDGE('',*,*,#37756,.T.) ;
#50151=ORIENTED_EDGE('',*,*,#37757,.T.) ;
#50152=ORIENTED_EDGE('',*,*,#37758,.T.) ;
#50153=ORIENTED_EDGE('',*,*,#37759,.T.) ;
#50154=ORIENTED_EDGE('',*,*,#37760,.T.) ;
#50155=ORIENTED_EDGE('',*,*,#37761,.T.) ;
#50156=ORIENTED_EDGE('',*,*,#37762,.T.) ;
#50157=ORIENTED_EDGE('',*,*,#37763,.T.) ;
#50158=ORIENTED_EDGE('',*,*,#37764,.T.) ;
#50159=ORIENTED_EDGE('',*,*,#37765,.T.) ;
#50160=ORIENTED_EDGE('',*,*,#37766,.T.) ;
#50161=ORIENTED_EDGE('',*,*,#37767,.F.) ;
#50162=ORIENTED_EDGE('',*,*,#37768,.T.) ;
#50163=ORIENTED_EDGE('',*,*,#37769,.T.) ;
#50164=ORIENTED_EDGE('',*,*,#37770,.T.) ;
#50165=ORIENTED_EDGE('',*,*,#37771,.F.) ;
#50166=ORIENTED_EDGE('',*,*,#37772,.T.) ;
#50167=ORIENTED_EDGE('',*,*,#37773,.T.) ;
#50168=ORIENTED_EDGE('',*,*,#37774,.T.) ;
#50169=ORIENTED_EDGE('',*,*,#37775,.T.) ;
#50170=ORIENTED_EDGE('',*,*,#37776,.T.) ;
#50171=ORIENTED_EDGE('',*,*,#37777,.F.) ;
#50172=ORIENTED_EDGE('',*,*,#37778,.T.) ;
#50173=ORIENTED_EDGE('',*,*,#37747,.F.) ;
#50174=ORIENTED_EDGE('',*,*,#37779,.T.) ;
#50175=ORIENTED_EDGE('',*,*,#37753,.F.) ;
#50176=ORIENTED_EDGE('',*,*,#37780,.T.) ;
#50177=ORIENTED_EDGE('',*,*,#37761,.F.) ;
#50178=ORIENTED_EDGE('',*,*,#37781,.T.) ;
#50179=ORIENTED_EDGE('',*,*,#37782,.F.) ;
#50180=ORIENTED_EDGE('',*,*,#37783,.T.) ;
#50181=ORIENTED_EDGE('',*,*,#37784,.F.) ;
#50182=ORIENTED_EDGE('',*,*,#37785,.T.) ;
#50183=ORIENTED_EDGE('',*,*,#37786,.T.) ;
#50184=ORIENTED_EDGE('',*,*,#37787,.T.) ;
#50185=ORIENTED_EDGE('',*,*,#37788,.F.) ;
#50186=ORIENTED_EDGE('',*,*,#37789,.T.) ;
#50187=ORIENTED_EDGE('',*,*,#37790,.T.) ;
#50188=ORIENTED_EDGE('',*,*,#37791,.T.) ;
#50189=ORIENTED_EDGE('',*,*,#37792,.F.) ;
#50190=ORIENTED_EDGE('',*,*,#37793,.T.) ;
#50191=ORIENTED_EDGE('',*,*,#37765,.F.) ;
#50192=ORIENTED_EDGE('',*,*,#37794,.T.) ;
#50193=ORIENTED_EDGE('',*,*,#37795,.T.) ;
#50194=ORIENTED_EDGE('',*,*,#37796,.T.) ;
#50195=ORIENTED_EDGE('',*,*,#37773,.F.) ;
#50196=ORIENTED_EDGE('',*,*,#37797,.T.) ;
#50197=ORIENTED_EDGE('',*,*,#37798,.F.) ;
#50198=ORIENTED_EDGE('',*,*,#37799,.F.) ;
#50199=ORIENTED_EDGE('',*,*,#37800,.T.) ;
#50200=ORIENTED_EDGE('',*,*,#37801,.F.) ;
#50201=ORIENTED_EDGE('',*,*,#37802,.T.) ;
#50202=ORIENTED_EDGE('',*,*,#37803,.F.) ;
#50203=ORIENTED_EDGE('',*,*,#37804,.T.) ;
#50204=ORIENTED_EDGE('',*,*,#37805,.T.) ;
#50205=ORIENTED_EDGE('',*,*,#37806,.T.) ;
#50206=ORIENTED_EDGE('',*,*,#37807,.T.) ;
#50207=ORIENTED_EDGE('',*,*,#37808,.T.) ;
#50208=ORIENTED_EDGE('',*,*,#37809,.T.) ;
#50209=ORIENTED_EDGE('',*,*,#37810,.T.) ;
#50210=ORIENTED_EDGE('',*,*,#37811,.T.) ;
#50211=ORIENTED_EDGE('',*,*,#37812,.T.) ;
#50212=ORIENTED_EDGE('',*,*,#37813,.T.) ;
#50213=ORIENTED_EDGE('',*,*,#37814,.T.) ;
#50214=ORIENTED_EDGE('',*,*,#37815,.T.) ;
#50215=ORIENTED_EDGE('',*,*,#37771,.T.) ;
#50216=ORIENTED_EDGE('',*,*,#37816,.T.) ;
#50217=ORIENTED_EDGE('',*,*,#37817,.T.) ;
#50218=ORIENTED_EDGE('',*,*,#37818,.T.) ;
#50219=ORIENTED_EDGE('',*,*,#37767,.T.) ;
#50220=ORIENTED_EDGE('',*,*,#37819,.T.) ;
#50221=ORIENTED_EDGE('',*,*,#37820,.F.) ;
#50222=ORIENTED_EDGE('',*,*,#37821,.T.) ;
#50223=ORIENTED_EDGE('',*,*,#37822,.F.) ;
#50224=ORIENTED_EDGE('',*,*,#37823,.T.) ;
#50225=ORIENTED_EDGE('',*,*,#37824,.T.) ;
#50226=ORIENTED_EDGE('',*,*,#37825,.T.) ;
#50227=ORIENTED_EDGE('',*,*,#37826,.F.) ;
#50228=ORIENTED_EDGE('',*,*,#37827,.T.) ;
#50229=ORIENTED_EDGE('',*,*,#37828,.F.) ;
#50230=ORIENTED_EDGE('',*,*,#37829,.T.) ;
#50231=ORIENTED_EDGE('',*,*,#37830,.T.) ;
#50232=ORIENTED_EDGE('',*,*,#37831,.T.) ;
#50233=ORIENTED_EDGE('',*,*,#37832,.T.) ;
#50234=ORIENTED_EDGE('',*,*,#37833,.T.) ;
#50235=ORIENTED_EDGE('',*,*,#37834,.T.) ;
#50236=ORIENTED_EDGE('',*,*,#37835,.T.) ;
#50237=ORIENTED_EDGE('',*,*,#37801,.T.) ;
#50238=ORIENTED_EDGE('',*,*,#37836,.T.) ;
#50239=ORIENTED_EDGE('',*,*,#37811,.F.) ;
#50240=ORIENTED_EDGE('',*,*,#37837,.T.) ;
#50241=ORIENTED_EDGE('',*,*,#37803,.T.) ;
#50242=ORIENTED_EDGE('',*,*,#37838,.T.) ;
#50243=ORIENTED_EDGE('',*,*,#37809,.F.) ;
#50244=ORIENTED_EDGE('',*,*,#37839,.T.) ;
#50245=ORIENTED_EDGE('',*,*,#37840,.T.) ;
#50246=ORIENTED_EDGE('',*,*,#37841,.T.) ;
#50247=ORIENTED_EDGE('',*,*,#37777,.T.) ;
#50248=ORIENTED_EDGE('',*,*,#37842,.T.) ;
#50249=ORIENTED_EDGE('',*,*,#37807,.F.) ;
#50250=ORIENTED_EDGE('',*,*,#37843,.T.) ;
#50251=ORIENTED_EDGE('',*,*,#37844,.T.) ;
#50252=ORIENTED_EDGE('',*,*,#37845,.T.) ;
#50253=ORIENTED_EDGE('',*,*,#37846,.T.) ;
#50254=ORIENTED_EDGE('',*,*,#37847,.T.) ;
#50255=ORIENTED_EDGE('',*,*,#37848,.T.) ;
#50256=ORIENTED_EDGE('',*,*,#37805,.F.) ;
#50257=ORIENTED_EDGE('',*,*,#37849,.T.) ;
#50258=ORIENTED_EDGE('',*,*,#37850,.T.) ;
#50259=ORIENTED_EDGE('',*,*,#37851,.T.) ;
#50260=ORIENTED_EDGE('',*,*,#37852,.T.) ;
#50261=ORIENTED_EDGE('',*,*,#37834,.F.) ;
#50262=ORIENTED_EDGE('',*,*,#37853,.T.) ;
#50263=ORIENTED_EDGE('',*,*,#37854,.T.) ;
#50264=ORIENTED_EDGE('',*,*,#37708,.T.) ;
#50265=ORIENTED_EDGE('',*,*,#37855,.T.) ;
#50266=ORIENTED_EDGE('',*,*,#37856,.T.) ;
#50267=ORIENTED_EDGE('',*,*,#37832,.F.) ;
#50268=ORIENTED_EDGE('',*,*,#37857,.T.) ;
#50269=ORIENTED_EDGE('',*,*,#37858,.T.) ;
#50270=ORIENTED_EDGE('',*,*,#37859,.T.) ;
#50271=ORIENTED_EDGE('',*,*,#37860,.T.) ;
#50272=ORIENTED_EDGE('',*,*,#37861,.T.) ;
#50273=ORIENTED_EDGE('',*,*,#37862,.T.) ;
#50274=ORIENTED_EDGE('',*,*,#37830,.F.) ;
#50275=ORIENTED_EDGE('',*,*,#37863,.T.) ;
#50276=ORIENTED_EDGE('',*,*,#37864,.T.) ;
#50277=ORIENTED_EDGE('',*,*,#37865,.F.) ;
#50278=ORIENTED_EDGE('',*,*,#37866,.T.) ;
#50279=ORIENTED_EDGE('',*,*,#37867,.F.) ;
#50280=ORIENTED_EDGE('',*,*,#37868,.T.) ;
#50281=ORIENTED_EDGE('',*,*,#37869,.T.) ;
#50282=ORIENTED_EDGE('',*,*,#37782,.T.) ;
#50283=ORIENTED_EDGE('',*,*,#37870,.F.) ;
#50284=ORIENTED_EDGE('',*,*,#37871,.T.) ;
#50285=ORIENTED_EDGE('',*,*,#37788,.T.) ;
#50286=ORIENTED_EDGE('',*,*,#37872,.T.) ;
#50287=ORIENTED_EDGE('',*,*,#37873,.F.) ;
#50288=ORIENTED_EDGE('',*,*,#37874,.T.) ;
#50289=ORIENTED_EDGE('',*,*,#37875,.F.) ;
#50290=ORIENTED_EDGE('',*,*,#37876,.T.) ;
#50291=ORIENTED_EDGE('',*,*,#37877,.T.) ;
#50292=ORIENTED_EDGE('',*,*,#37878,.T.) ;
#50293=ORIENTED_EDGE('',*,*,#37879,.F.) ;
#50294=ORIENTED_EDGE('',*,*,#37880,.T.) ;
#50295=ORIENTED_EDGE('',*,*,#37881,.F.) ;
#50296=ORIENTED_EDGE('',*,*,#37882,.T.) ;
#50297=ORIENTED_EDGE('',*,*,#37824,.F.) ;
#50298=ORIENTED_EDGE('',*,*,#37883,.T.) ;
#50299=ORIENTED_EDGE('',*,*,#37884,.F.) ;
#50300=ORIENTED_EDGE('',*,*,#37885,.T.) ;
#50301=ORIENTED_EDGE('',*,*,#37886,.F.) ;
#50302=ORIENTED_EDGE('',*,*,#37887,.T.) ;
#50303=ORIENTED_EDGE('',*,*,#37888,.T.) ;
#50304=ORIENTED_EDGE('',*,*,#37889,.T.) ;
#50305=ORIENTED_EDGE('',*,*,#37890,.F.) ;
#50306=ORIENTED_EDGE('',*,*,#37891,.T.) ;
#50307=ORIENTED_EDGE('',*,*,#37719,.T.) ;
#50308=ORIENTED_EDGE('',*,*,#37892,.F.) ;
#50309=ORIENTED_EDGE('',*,*,#37893,.T.) ;
#50310=ORIENTED_EDGE('',*,*,#37894,.F.) ;
#50311=ORIENTED_EDGE('',*,*,#37798,.T.) ;
#50312=ORIENTED_EDGE('',*,*,#37895,.T.) ;
#50313=ORIENTED_EDGE('',*,*,#37814,.F.) ;
#50314=ORIENTED_EDGE('',*,*,#37896,.F.) ;
#50315=ORIENTED_EDGE('',*,*,#37897,.T.) ;
#50316=ORIENTED_EDGE('',*,*,#37898,.F.) ;
#50317=ORIENTED_EDGE('',*,*,#37899,.T.) ;
#50318=ORIENTED_EDGE('',*,*,#37900,.F.) ;
#50319=ORIENTED_EDGE('',*,*,#37901,.T.) ;
#50320=ORIENTED_EDGE('',*,*,#37896,.T.) ;
#50321=ORIENTED_EDGE('',*,*,#37813,.F.) ;
#50322=ORIENTED_EDGE('',*,*,#37902,.T.) ;
#50323=ORIENTED_EDGE('',*,*,#37799,.T.) ;
#50324=ORIENTED_EDGE('',*,*,#37894,.T.) ;
#50325=ORIENTED_EDGE('',*,*,#37903,.T.) ;
#50326=ORIENTED_EDGE('',*,*,#37904,.F.) ;
#50327=ORIENTED_EDGE('',*,*,#37905,.T.) ;
#50328=ORIENTED_EDGE('',*,*,#37906,.T.) ;
#50329=ORIENTED_EDGE('',*,*,#37907,.T.) ;
#50330=ORIENTED_EDGE('',*,*,#37908,.F.) ;
#50331=ORIENTED_EDGE('',*,*,#37909,.F.) ;
#50332=ORIENTED_EDGE('',*,*,#37910,.T.) ;
#50333=ORIENTED_EDGE('',*,*,#37911,.T.) ;
#50334=ORIENTED_EDGE('',*,*,#37912,.T.) ;
#50335=ORIENTED_EDGE('',*,*,#37913,.T.) ;
#50336=ORIENTED_EDGE('',*,*,#37914,.T.) ;
#50337=ORIENTED_EDGE('',*,*,#37915,.T.) ;
#50338=ORIENTED_EDGE('',*,*,#37916,.T.) ;
#50339=ORIENTED_EDGE('',*,*,#37917,.T.) ;
#50340=ORIENTED_EDGE('',*,*,#37918,.T.) ;
#50341=ORIENTED_EDGE('',*,*,#37919,.T.) ;
#50342=ORIENTED_EDGE('',*,*,#37920,.T.) ;
#50343=ORIENTED_EDGE('',*,*,#37921,.T.) ;
#50344=ORIENTED_EDGE('',*,*,#37922,.T.) ;
#50345=ORIENTED_EDGE('',*,*,#37923,.T.) ;
#50346=ORIENTED_EDGE('',*,*,#37924,.T.) ;
#50347=ORIENTED_EDGE('',*,*,#37925,.T.) ;
#50348=ORIENTED_EDGE('',*,*,#37926,.T.) ;
#50349=ORIENTED_EDGE('',*,*,#37927,.T.) ;
#50350=ORIENTED_EDGE('',*,*,#37928,.T.) ;
#50351=ORIENTED_EDGE('',*,*,#37929,.T.) ;
#50352=ORIENTED_EDGE('',*,*,#37930,.T.) ;
#50353=ORIENTED_EDGE('',*,*,#37931,.T.) ;
#50354=ORIENTED_EDGE('',*,*,#37932,.T.) ;
#50355=ORIENTED_EDGE('',*,*,#37933,.T.) ;
#50356=ORIENTED_EDGE('',*,*,#37934,.T.) ;
#50357=ORIENTED_EDGE('',*,*,#37935,.T.) ;
#50358=ORIENTED_EDGE('',*,*,#37936,.T.) ;
#50359=ORIENTED_EDGE('',*,*,#37937,.T.) ;
#50360=ORIENTED_EDGE('',*,*,#37938,.T.) ;
#50361=ORIENTED_EDGE('',*,*,#37939,.T.) ;
#50362=ORIENTED_EDGE('',*,*,#37940,.T.) ;
#50363=ORIENTED_EDGE('',*,*,#37941,.T.) ;
#50364=ORIENTED_EDGE('',*,*,#37942,.T.) ;
#50365=ORIENTED_EDGE('',*,*,#37943,.T.) ;
#50366=ORIENTED_EDGE('',*,*,#37944,.T.) ;
#50367=ORIENTED_EDGE('',*,*,#37945,.T.) ;
#50368=ORIENTED_EDGE('',*,*,#37714,.T.) ;
#50369=ORIENTED_EDGE('',*,*,#37946,.F.) ;
#50370=ORIENTED_EDGE('',*,*,#37947,.T.) ;
#50371=ORIENTED_EDGE('',*,*,#37948,.T.) ;
#50372=ORIENTED_EDGE('',*,*,#37949,.T.) ;
#50373=ORIENTED_EDGE('',*,*,#37950,.T.) ;
#50374=ORIENTED_EDGE('',*,*,#37951,.T.) ;
#50375=ORIENTED_EDGE('',*,*,#37952,.T.) ;
#50376=ORIENTED_EDGE('',*,*,#37953,.T.) ;
#50377=ORIENTED_EDGE('',*,*,#37954,.F.) ;
#50378=ORIENTED_EDGE('',*,*,#37955,.T.) ;
#50379=ORIENTED_EDGE('',*,*,#37792,.T.) ;
#50380=ORIENTED_EDGE('',*,*,#37956,.T.) ;
#50381=ORIENTED_EDGE('',*,*,#37957,.T.) ;
#50382=ORIENTED_EDGE('',*,*,#37958,.T.) ;
#50383=ORIENTED_EDGE('',*,*,#37959,.T.) ;
#50384=ORIENTED_EDGE('',*,*,#37790,.F.) ;
#50385=ORIENTED_EDGE('',*,*,#37960,.T.) ;
#50386=ORIENTED_EDGE('',*,*,#37961,.T.) ;
#50387=ORIENTED_EDGE('',*,*,#37962,.T.) ;
#50388=ORIENTED_EDGE('',*,*,#37963,.T.) ;
#50389=ORIENTED_EDGE('',*,*,#37964,.T.) ;
#50390=ORIENTED_EDGE('',*,*,#37728,.T.) ;
#50391=ORIENTED_EDGE('',*,*,#37965,.T.) ;
#50392=ORIENTED_EDGE('',*,*,#37966,.T.) ;
#50393=ORIENTED_EDGE('',*,*,#37967,.T.) ;
#50394=ORIENTED_EDGE('',*,*,#37968,.T.) ;
#50395=ORIENTED_EDGE('',*,*,#37969,.T.) ;
#50396=ORIENTED_EDGE('',*,*,#37970,.T.) ;
#50397=ORIENTED_EDGE('',*,*,#37971,.T.) ;
#50398=ORIENTED_EDGE('',*,*,#37972,.T.) ;
#50399=ORIENTED_EDGE('',*,*,#37973,.T.) ;
#50400=ORIENTED_EDGE('',*,*,#37721,.T.) ;
#50401=ORIENTED_EDGE('',*,*,#37974,.T.) ;
#50402=ORIENTED_EDGE('',*,*,#37975,.T.) ;
#50403=ORIENTED_EDGE('',*,*,#37976,.T.) ;
#50404=ORIENTED_EDGE('',*,*,#37977,.T.) ;
#50405=ORIENTED_EDGE('',*,*,#37978,.T.) ;
#50406=ORIENTED_EDGE('',*,*,#37822,.T.) ;
#50407=ORIENTED_EDGE('',*,*,#37979,.T.) ;
#50408=ORIENTED_EDGE('',*,*,#37980,.T.) ;
#50409=ORIENTED_EDGE('',*,*,#37981,.T.) ;
#50410=ORIENTED_EDGE('',*,*,#37820,.T.) ;
#50411=ORIENTED_EDGE('',*,*,#37982,.T.) ;
#50412=ORIENTED_EDGE('',*,*,#37983,.F.) ;
#50413=ORIENTED_EDGE('',*,*,#37984,.T.) ;
#50414=ORIENTED_EDGE('',*,*,#37985,.T.) ;
#50415=ORIENTED_EDGE('',*,*,#37986,.T.) ;
#50416=ORIENTED_EDGE('',*,*,#37987,.T.) ;
#50417=ORIENTED_EDGE('',*,*,#37784,.T.) ;
#50418=ORIENTED_EDGE('',*,*,#37988,.T.) ;
#50419=ORIENTED_EDGE('',*,*,#37989,.T.) ;
#50420=ORIENTED_EDGE('',*,*,#37990,.T.) ;
#50421=ORIENTED_EDGE('',*,*,#37991,.T.) ;
#50422=ORIENTED_EDGE('',*,*,#37786,.F.) ;
#50423=ORIENTED_EDGE('',*,*,#37992,.T.) ;
#50424=ORIENTED_EDGE('',*,*,#37993,.T.) ;
#50425=ORIENTED_EDGE('',*,*,#37994,.T.) ;
#50426=ORIENTED_EDGE('',*,*,#37995,.T.) ;
#50427=ORIENTED_EDGE('',*,*,#37996,.T.) ;
#50428=ORIENTED_EDGE('',*,*,#37997,.T.) ;
#50429=ORIENTED_EDGE('',*,*,#37998,.T.) ;
#50430=ORIENTED_EDGE('',*,*,#37999,.T.) ;
#50431=ORIENTED_EDGE('',*,*,#38000,.T.) ;
#50432=ORIENTED_EDGE('',*,*,#38001,.T.) ;
#50433=ORIENTED_EDGE('',*,*,#38002,.T.) ;
#50434=ORIENTED_EDGE('',*,*,#38003,.T.) ;
#50435=ORIENTED_EDGE('',*,*,#38004,.T.) ;
#50436=ORIENTED_EDGE('',*,*,#37826,.T.) ;
#50437=ORIENTED_EDGE('',*,*,#38005,.T.) ;
#50438=ORIENTED_EDGE('',*,*,#38006,.T.) ;
#50439=ORIENTED_EDGE('',*,*,#38007,.T.) ;
#50440=ORIENTED_EDGE('',*,*,#38008,.T.) ;
#50441=ORIENTED_EDGE('',*,*,#38009,.T.) ;
#50442=ORIENTED_EDGE('',*,*,#38010,.T.) ;
#50443=ORIENTED_EDGE('',*,*,#38011,.T.) ;
#50444=ORIENTED_EDGE('',*,*,#38012,.T.) ;
#50445=ORIENTED_EDGE('',*,*,#38013,.T.) ;
#50446=ORIENTED_EDGE('',*,*,#37828,.T.) ;
#50447=ORIENTED_EDGE('',*,*,#38014,.T.) ;
#50448=ORIENTED_EDGE('',*,*,#38015,.T.) ;
#50449=ORIENTED_EDGE('',*,*,#38016,.T.) ;
#50450=ORIENTED_EDGE('',*,*,#38017,.T.) ;
#50451=ORIENTED_EDGE('',*,*,#38018,.T.) ;
#50452=ORIENTED_EDGE('',*,*,#38019,.T.) ;
#50453=ORIENTED_EDGE('',*,*,#38020,.T.) ;
#50454=ORIENTED_EDGE('',*,*,#38021,.T.) ;
#50455=ORIENTED_EDGE('',*,*,#37713,.T.) ;
#50456=ORIENTED_EDGE('',*,*,#38022,.T.) ;
#50457=ORIENTED_EDGE('',*,*,#38023,.T.) ;
#50458=ORIENTED_EDGE('',*,*,#38024,.T.) ;
#50459=ORIENTED_EDGE('',*,*,#38025,.T.) ;
#50460=ORIENTED_EDGE('',*,*,#38026,.T.) ;
#50461=ORIENTED_EDGE('',*,*,#38027,.T.) ;
#50462=ORIENTED_EDGE('',*,*,#38028,.T.) ;
#50463=ORIENTED_EDGE('',*,*,#38029,.T.) ;
#50464=ORIENTED_EDGE('',*,*,#38030,.T.) ;
#50465=ORIENTED_EDGE('',*,*,#38031,.T.) ;
#50466=ORIENTED_EDGE('',*,*,#38032,.T.) ;
#50467=ORIENTED_EDGE('',*,*,#38033,.T.) ;
#50468=ORIENTED_EDGE('',*,*,#38034,.T.) ;
#50469=ORIENTED_EDGE('',*,*,#38035,.T.) ;
#50470=ORIENTED_EDGE('',*,*,#38036,.T.) ;
#50471=ORIENTED_EDGE('',*,*,#38037,.T.) ;
#50472=ORIENTED_EDGE('',*,*,#38038,.T.) ;
#50473=ORIENTED_EDGE('',*,*,#38039,.T.) ;
#50474=ORIENTED_EDGE('',*,*,#38040,.T.) ;
#50475=ORIENTED_EDGE('',*,*,#38041,.T.) ;
#50476=ORIENTED_EDGE('',*,*,#38042,.T.) ;
#50477=ORIENTED_EDGE('',*,*,#38043,.T.) ;
#50478=ORIENTED_EDGE('',*,*,#38044,.T.) ;
#50479=ORIENTED_EDGE('',*,*,#38045,.T.) ;
#50480=ORIENTED_EDGE('',*,*,#37946,.T.) ;
#50481=ORIENTED_EDGE('',*,*,#38046,.T.) ;
#50482=ORIENTED_EDGE('',*,*,#38047,.T.) ;
#50483=ORIENTED_EDGE('',*,*,#38048,.T.) ;
#50484=ORIENTED_EDGE('',*,*,#37950,.F.) ;
#50485=ORIENTED_EDGE('',*,*,#38049,.T.) ;
#50486=ORIENTED_EDGE('',*,*,#38050,.T.) ;
#50487=ORIENTED_EDGE('',*,*,#38051,.T.) ;
#50488=ORIENTED_EDGE('',*,*,#37952,.F.) ;
#50489=ORIENTED_EDGE('',*,*,#38052,.T.) ;
#50490=ORIENTED_EDGE('',*,*,#38053,.T.) ;
#50491=ORIENTED_EDGE('',*,*,#38054,.T.) ;
#50492=ORIENTED_EDGE('',*,*,#37948,.F.) ;
#50493=ORIENTED_EDGE('',*,*,#38055,.T.) ;
#50494=ORIENTED_EDGE('',*,*,#38056,.T.) ;
#50495=ORIENTED_EDGE('',*,*,#38057,.T.) ;
#50496=ORIENTED_EDGE('',*,*,#38058,.T.) ;
#50497=ORIENTED_EDGE('',*,*,#38059,.T.) ;
#50498=ORIENTED_EDGE('',*,*,#38060,.T.) ;
#50499=ORIENTED_EDGE('',*,*,#38061,.T.) ;
#50500=ORIENTED_EDGE('',*,*,#38062,.T.) ;
#50501=ORIENTED_EDGE('',*,*,#38063,.T.) ;
#50502=ORIENTED_EDGE('',*,*,#38064,.T.) ;
#50503=ORIENTED_EDGE('',*,*,#38065,.T.) ;
#50504=ORIENTED_EDGE('',*,*,#38066,.T.) ;
#50505=ORIENTED_EDGE('',*,*,#38067,.F.) ;
#50506=ORIENTED_EDGE('',*,*,#38068,.T.) ;
#50507=ORIENTED_EDGE('',*,*,#37744,.F.) ;
#50508=ORIENTED_EDGE('',*,*,#38069,.T.) ;
#50509=ORIENTED_EDGE('',*,*,#38070,.T.) ;
#50510=ORIENTED_EDGE('',*,*,#38071,.T.) ;
#50511=ORIENTED_EDGE('',*,*,#38072,.T.) ;
#50512=ORIENTED_EDGE('',*,*,#38067,.T.) ;
#50513=ORIENTED_EDGE('',*,*,#38073,.T.) ;
#50514=ORIENTED_EDGE('',*,*,#38074,.T.) ;
#50515=ORIENTED_EDGE('',*,*,#38075,.T.) ;
#50516=ORIENTED_EDGE('',*,*,#38076,.T.) ;
#50517=ORIENTED_EDGE('',*,*,#38077,.T.) ;
#50518=ORIENTED_EDGE('',*,*,#38078,.T.) ;
#50519=ORIENTED_EDGE('',*,*,#38079,.T.) ;
#50520=ORIENTED_EDGE('',*,*,#38080,.T.) ;
#50521=ORIENTED_EDGE('',*,*,#38081,.T.) ;
#50522=ORIENTED_EDGE('',*,*,#38082,.T.) ;
#50523=ORIENTED_EDGE('',*,*,#38083,.T.) ;
#50524=ORIENTED_EDGE('',*,*,#38084,.T.) ;
#50525=ORIENTED_EDGE('',*,*,#38085,.T.) ;
#50526=ORIENTED_EDGE('',*,*,#38086,.T.) ;
#50527=ORIENTED_EDGE('',*,*,#38087,.T.) ;
#50528=ORIENTED_EDGE('',*,*,#38088,.F.) ;
#50529=ORIENTED_EDGE('',*,*,#37937,.F.) ;
#50530=ORIENTED_EDGE('',*,*,#38089,.T.) ;
#50531=ORIENTED_EDGE('',*,*,#38088,.T.) ;
#50532=ORIENTED_EDGE('',*,*,#38090,.T.) ;
#50533=ORIENTED_EDGE('',*,*,#38091,.T.) ;
#50534=ORIENTED_EDGE('',*,*,#38092,.T.) ;
#50535=ORIENTED_EDGE('',*,*,#38093,.T.) ;
#50536=ORIENTED_EDGE('',*,*,#38094,.T.) ;
#50537=ORIENTED_EDGE('',*,*,#38095,.T.) ;
#50538=ORIENTED_EDGE('',*,*,#38096,.T.) ;
#50539=ORIENTED_EDGE('',*,*,#38097,.T.) ;
#50540=ORIENTED_EDGE('',*,*,#38098,.T.) ;
#50541=ORIENTED_EDGE('',*,*,#38099,.T.) ;
#50542=ORIENTED_EDGE('',*,*,#38100,.T.) ;
#50543=ORIENTED_EDGE('',*,*,#38101,.T.) ;
#50544=ORIENTED_EDGE('',*,*,#38102,.T.) ;
#50545=ORIENTED_EDGE('',*,*,#38103,.T.) ;
#50546=ORIENTED_EDGE('',*,*,#38104,.T.) ;
#50547=ORIENTED_EDGE('',*,*,#38105,.T.) ;
#50548=ORIENTED_EDGE('',*,*,#38106,.T.) ;
#50549=ORIENTED_EDGE('',*,*,#38107,.T.) ;
#50550=ORIENTED_EDGE('',*,*,#38108,.T.) ;
#50551=ORIENTED_EDGE('',*,*,#38109,.T.) ;
#50552=ORIENTED_EDGE('',*,*,#37817,.F.) ;
#50553=ORIENTED_EDGE('',*,*,#38110,.T.) ;
#50554=ORIENTED_EDGE('',*,*,#38111,.T.) ;
#50555=ORIENTED_EDGE('',*,*,#37731,.T.) ;
#50556=ORIENTED_EDGE('',*,*,#38112,.T.) ;
#50557=ORIENTED_EDGE('',*,*,#37795,.F.) ;
#50558=ORIENTED_EDGE('',*,*,#38113,.T.) ;
#50559=ORIENTED_EDGE('',*,*,#38114,.T.) ;
#50560=ORIENTED_EDGE('',*,*,#38115,.T.) ;
#50561=ORIENTED_EDGE('',*,*,#38116,.F.) ;
#50562=ORIENTED_EDGE('',*,*,#38014,.F.) ;
#50563=ORIENTED_EDGE('',*,*,#37827,.F.) ;
#50564=ORIENTED_EDGE('',*,*,#38007,.F.) ;
#50565=ORIENTED_EDGE('',*,*,#38117,.F.) ;
#50566=ORIENTED_EDGE('',*,*,#38116,.T.) ;
#50567=ORIENTED_EDGE('',*,*,#38118,.F.) ;
#50568=ORIENTED_EDGE('',*,*,#37825,.F.) ;
#50569=ORIENTED_EDGE('',*,*,#37882,.F.) ;
#50570=ORIENTED_EDGE('',*,*,#38119,.F.) ;
#50571=ORIENTED_EDGE('',*,*,#38005,.F.) ;
#50572=ORIENTED_EDGE('',*,*,#38118,.T.) ;
#50573=ORIENTED_EDGE('',*,*,#38006,.F.) ;
#50574=ORIENTED_EDGE('',*,*,#38120,.F.) ;
#50575=ORIENTED_EDGE('',*,*,#38002,.F.) ;
#50576=ORIENTED_EDGE('',*,*,#38117,.T.) ;
#50577=ORIENTED_EDGE('',*,*,#38001,.F.) ;
#50578=ORIENTED_EDGE('',*,*,#38121,.F.) ;
#50579=ORIENTED_EDGE('',*,*,#38015,.F.) ;
#50580=ORIENTED_EDGE('',*,*,#38119,.T.) ;
#50581=ORIENTED_EDGE('',*,*,#37881,.T.) ;
#50582=ORIENTED_EDGE('',*,*,#38122,.F.) ;
#50583=ORIENTED_EDGE('',*,*,#38120,.T.) ;
#50584=ORIENTED_EDGE('',*,*,#38123,.F.) ;
#50585=ORIENTED_EDGE('',*,*,#38121,.T.) ;
#50586=ORIENTED_EDGE('',*,*,#38124,.F.) ;
#50587=ORIENTED_EDGE('',*,*,#37785,.F.) ;
#50588=ORIENTED_EDGE('',*,*,#37987,.F.) ;
#50589=ORIENTED_EDGE('',*,*,#38125,.F.) ;
#50590=ORIENTED_EDGE('',*,*,#37992,.F.) ;
#50591=ORIENTED_EDGE('',*,*,#38126,.F.) ;
#50592=ORIENTED_EDGE('',*,*,#37990,.F.) ;
#50593=ORIENTED_EDGE('',*,*,#38127,.F.) ;
#50594=ORIENTED_EDGE('',*,*,#37996,.F.) ;
#50595=ORIENTED_EDGE('',*,*,#37787,.F.) ;
#50596=ORIENTED_EDGE('',*,*,#37991,.F.) ;
#50597=ORIENTED_EDGE('',*,*,#38128,.F.) ;
#50598=ORIENTED_EDGE('',*,*,#37872,.F.) ;
#50599=ORIENTED_EDGE('',*,*,#38122,.T.) ;
#50600=ORIENTED_EDGE('',*,*,#37880,.F.) ;
#50601=ORIENTED_EDGE('',*,*,#38129,.F.) ;
#50602=ORIENTED_EDGE('',*,*,#38003,.F.) ;
#50603=ORIENTED_EDGE('',*,*,#38124,.T.) ;
#50604=ORIENTED_EDGE('',*,*,#38004,.F.) ;
#50605=ORIENTED_EDGE('',*,*,#38130,.F.) ;
#50606=ORIENTED_EDGE('',*,*,#38011,.F.) ;
#50607=ORIENTED_EDGE('',*,*,#38123,.T.) ;
#50608=ORIENTED_EDGE('',*,*,#38010,.F.) ;
#50609=ORIENTED_EDGE('',*,*,#38131,.F.) ;
#50610=ORIENTED_EDGE('',*,*,#38012,.F.) ;
#50611=ORIENTED_EDGE('',*,*,#37829,.F.) ;
#50612=ORIENTED_EDGE('',*,*,#38013,.F.) ;
#50613=ORIENTED_EDGE('',*,*,#38132,.F.) ;
#50614=ORIENTED_EDGE('',*,*,#37863,.F.) ;
#50615=ORIENTED_EDGE('',*,*,#38127,.T.) ;
#50616=ORIENTED_EDGE('',*,*,#38125,.T.) ;
#50617=ORIENTED_EDGE('',*,*,#38133,.F.) ;
#50618=ORIENTED_EDGE('',*,*,#38128,.T.) ;
#50619=ORIENTED_EDGE('',*,*,#38126,.T.) ;
#50620=ORIENTED_EDGE('',*,*,#38134,.F.) ;
#50621=ORIENTED_EDGE('',*,*,#37873,.T.) ;
#50622=ORIENTED_EDGE('',*,*,#38129,.T.) ;
#50623=ORIENTED_EDGE('',*,*,#37879,.T.) ;
#50624=ORIENTED_EDGE('',*,*,#38135,.F.) ;
#50625=ORIENTED_EDGE('',*,*,#38130,.T.) ;
#50626=ORIENTED_EDGE('',*,*,#38132,.T.) ;
#50627=ORIENTED_EDGE('',*,*,#38131,.T.) ;
#50628=ORIENTED_EDGE('',*,*,#38136,.F.) ;
#50629=ORIENTED_EDGE('',*,*,#38133,.T.) ;
#50630=ORIENTED_EDGE('',*,*,#37986,.F.) ;
#50631=ORIENTED_EDGE('',*,*,#38137,.F.) ;
#50632=ORIENTED_EDGE('',*,*,#37993,.F.) ;
#50633=ORIENTED_EDGE('',*,*,#38138,.F.) ;
#50634=ORIENTED_EDGE('',*,*,#37994,.F.) ;
#50635=ORIENTED_EDGE('',*,*,#38139,.F.) ;
#50636=ORIENTED_EDGE('',*,*,#38000,.F.) ;
#50637=ORIENTED_EDGE('',*,*,#38134,.T.) ;
#50638=ORIENTED_EDGE('',*,*,#37995,.F.) ;
#50639=ORIENTED_EDGE('',*,*,#38140,.F.) ;
#50640=ORIENTED_EDGE('',*,*,#37874,.F.) ;
#50641=ORIENTED_EDGE('',*,*,#38135,.T.) ;
#50642=ORIENTED_EDGE('',*,*,#37878,.F.) ;
#50643=ORIENTED_EDGE('',*,*,#38141,.F.) ;
#50644=ORIENTED_EDGE('',*,*,#38008,.F.) ;
#50645=ORIENTED_EDGE('',*,*,#38136,.T.) ;
#50646=ORIENTED_EDGE('',*,*,#38009,.F.) ;
#50647=ORIENTED_EDGE('',*,*,#38142,.F.) ;
#50648=ORIENTED_EDGE('',*,*,#37864,.F.) ;
#50649=ORIENTED_EDGE('',*,*,#38139,.T.) ;
#50650=ORIENTED_EDGE('',*,*,#38137,.T.) ;
#50651=ORIENTED_EDGE('',*,*,#38143,.F.) ;
#50652=ORIENTED_EDGE('',*,*,#38140,.T.) ;
#50653=ORIENTED_EDGE('',*,*,#38138,.T.) ;
#50654=ORIENTED_EDGE('',*,*,#38144,.F.) ;
#50655=ORIENTED_EDGE('',*,*,#37875,.T.) ;
#50656=ORIENTED_EDGE('',*,*,#38142,.T.) ;
#50657=ORIENTED_EDGE('',*,*,#38141,.T.) ;
#50658=ORIENTED_EDGE('',*,*,#38145,.F.) ;
#50659=ORIENTED_EDGE('',*,*,#37865,.T.) ;
#50660=ORIENTED_EDGE('',*,*,#37783,.F.) ;
#50661=ORIENTED_EDGE('',*,*,#37869,.F.) ;
#50662=ORIENTED_EDGE('',*,*,#38146,.F.) ;
#50663=ORIENTED_EDGE('',*,*,#37988,.F.) ;
#50664=ORIENTED_EDGE('',*,*,#38143,.T.) ;
#50665=ORIENTED_EDGE('',*,*,#37989,.F.) ;
#50666=ORIENTED_EDGE('',*,*,#38147,.F.) ;
#50667=ORIENTED_EDGE('',*,*,#37997,.F.) ;
#50668=ORIENTED_EDGE('',*,*,#38144,.T.) ;
#50669=ORIENTED_EDGE('',*,*,#37999,.F.) ;
#50670=ORIENTED_EDGE('',*,*,#38148,.F.) ;
#50671=ORIENTED_EDGE('',*,*,#37876,.F.) ;
#50672=ORIENTED_EDGE('',*,*,#38145,.T.) ;
#50673=ORIENTED_EDGE('',*,*,#37877,.F.) ;
#50674=ORIENTED_EDGE('',*,*,#38149,.F.) ;
#50675=ORIENTED_EDGE('',*,*,#37866,.F.) ;
#50676=ORIENTED_EDGE('',*,*,#38147,.T.) ;
#50677=ORIENTED_EDGE('',*,*,#38146,.T.) ;
#50678=ORIENTED_EDGE('',*,*,#38150,.F.) ;
#50679=ORIENTED_EDGE('',*,*,#38149,.T.) ;
#50680=ORIENTED_EDGE('',*,*,#38148,.T.) ;
#50681=ORIENTED_EDGE('',*,*,#38151,.F.) ;
#50682=ORIENTED_EDGE('',*,*,#37867,.T.) ;
#50683=ORIENTED_EDGE('',*,*,#38150,.T.) ;
#50684=ORIENTED_EDGE('',*,*,#37868,.F.) ;
#50685=ORIENTED_EDGE('',*,*,#38151,.T.) ;
#50686=ORIENTED_EDGE('',*,*,#37998,.F.) ;
#50687=ORIENTED_EDGE('',*,*,#38152,.F.) ;
#50688=ORIENTED_EDGE('',*,*,#38153,.F.) ;
#50689=ORIENTED_EDGE('',*,*,#38154,.F.) ;
#50690=ORIENTED_EDGE('',*,*,#37945,.F.) ;
#50691=ORIENTED_EDGE('',*,*,#38155,.T.) ;
#50692=ORIENTED_EDGE('',*,*,#38156,.T.) ;
#50693=ORIENTED_EDGE('',*,*,#37927,.F.) ;
#50694=ORIENTED_EDGE('',*,*,#38153,.T.) ;
#50695=ORIENTED_EDGE('',*,*,#37926,.F.) ;
#50696=ORIENTED_EDGE('',*,*,#38157,.T.) ;
#50697=ORIENTED_EDGE('',*,*,#38158,.T.) ;
#50698=ORIENTED_EDGE('',*,*,#37919,.F.) ;
#50699=ORIENTED_EDGE('',*,*,#38154,.T.) ;
#50700=ORIENTED_EDGE('',*,*,#38152,.T.) ;
#50701=ORIENTED_EDGE('',*,*,#37918,.F.) ;
#50702=ORIENTED_EDGE('',*,*,#38159,.F.) ;
#50703=ORIENTED_EDGE('',*,*,#37938,.F.) ;
#50704=ORIENTED_EDGE('',*,*,#37934,.F.) ;
#50705=ORIENTED_EDGE('',*,*,#38160,.T.) ;
#50706=ORIENTED_EDGE('',*,*,#38161,.T.) ;
#50707=ORIENTED_EDGE('',*,*,#37944,.F.) ;
#50708=ORIENTED_EDGE('',*,*,#38162,.T.) ;
#50709=ORIENTED_EDGE('',*,*,#38163,.T.) ;
#50710=ORIENTED_EDGE('',*,*,#37912,.F.) ;
#50711=ORIENTED_EDGE('',*,*,#38164,.T.) ;
#50712=ORIENTED_EDGE('',*,*,#38165,.T.) ;
#50713=ORIENTED_EDGE('',*,*,#37928,.F.) ;
#50714=ORIENTED_EDGE('',*,*,#38166,.T.) ;
#50715=ORIENTED_EDGE('',*,*,#38167,.T.) ;
#50716=ORIENTED_EDGE('',*,*,#38168,.F.) ;
#50717=ORIENTED_EDGE('',*,*,#38159,.T.) ;
#50718=ORIENTED_EDGE('',*,*,#38169,.F.) ;
#50719=ORIENTED_EDGE('',*,*,#37909,.T.) ;
#50720=ORIENTED_EDGE('',*,*,#38170,.F.) ;
#50721=ORIENTED_EDGE('',*,*,#38171,.F.) ;
#50722=ORIENTED_EDGE('',*,*,#37939,.F.) ;
#50723=ORIENTED_EDGE('',*,*,#38168,.T.) ;
#50724=ORIENTED_EDGE('',*,*,#38171,.T.) ;
#50725=ORIENTED_EDGE('',*,*,#38172,.F.) ;
#50726=ORIENTED_EDGE('',*,*,#38173,.F.) ;
#50727=ORIENTED_EDGE('',*,*,#37923,.F.) ;
#50728=ORIENTED_EDGE('',*,*,#38174,.T.) ;
#50729=ORIENTED_EDGE('',*,*,#38175,.T.) ;
#50730=ORIENTED_EDGE('',*,*,#37943,.F.) ;
#50731=ORIENTED_EDGE('',*,*,#38176,.F.) ;
#50732=ORIENTED_EDGE('',*,*,#37913,.F.) ;
#50733=ORIENTED_EDGE('',*,*,#38177,.T.) ;
#50734=ORIENTED_EDGE('',*,*,#38178,.T.) ;
#50735=ORIENTED_EDGE('',*,*,#37920,.F.) ;
#50736=ORIENTED_EDGE('',*,*,#38179,.F.) ;
#50737=ORIENTED_EDGE('',*,*,#38169,.T.) ;
#50738=ORIENTED_EDGE('',*,*,#37917,.F.) ;
#50739=ORIENTED_EDGE('',*,*,#38180,.F.) ;
#50740=ORIENTED_EDGE('',*,*,#38181,.F.) ;
#50741=ORIENTED_EDGE('',*,*,#38182,.F.) ;
#50742=ORIENTED_EDGE('',*,*,#37893,.F.) ;
#50743=ORIENTED_EDGE('',*,*,#38183,.F.) ;
#50744=ORIENTED_EDGE('',*,*,#38170,.T.) ;
#50745=ORIENTED_EDGE('',*,*,#37911,.F.) ;
#50746=ORIENTED_EDGE('',*,*,#38183,.T.) ;
#50747=ORIENTED_EDGE('',*,*,#37892,.T.) ;
#50748=ORIENTED_EDGE('',*,*,#38184,.F.) ;
#50749=ORIENTED_EDGE('',*,*,#38172,.T.) ;
#50750=ORIENTED_EDGE('',*,*,#37940,.F.) ;
#50751=ORIENTED_EDGE('',*,*,#38173,.T.) ;
#50752=ORIENTED_EDGE('',*,*,#38185,.F.) ;
#50753=ORIENTED_EDGE('',*,*,#38186,.F.) ;
#50754=ORIENTED_EDGE('',*,*,#38179,.T.) ;
#50755=ORIENTED_EDGE('',*,*,#38176,.T.) ;
#50756=ORIENTED_EDGE('',*,*,#38187,.F.) ;
#50757=ORIENTED_EDGE('',*,*,#38188,.F.) ;
#50758=ORIENTED_EDGE('',*,*,#38180,.T.) ;
#50759=ORIENTED_EDGE('',*,*,#38189,.F.) ;
#50760=ORIENTED_EDGE('',*,*,#37910,.F.) ;
#50761=ORIENTED_EDGE('',*,*,#38181,.T.) ;
#50762=ORIENTED_EDGE('',*,*,#38190,.F.) ;
#50763=ORIENTED_EDGE('',*,*,#37903,.F.) ;
#50764=ORIENTED_EDGE('',*,*,#38182,.T.) ;
#50765=ORIENTED_EDGE('',*,*,#38191,.F.) ;
#50766=ORIENTED_EDGE('',*,*,#38185,.T.) ;
#50767=ORIENTED_EDGE('',*,*,#38184,.T.) ;
#50768=ORIENTED_EDGE('',*,*,#37899,.F.) ;
#50769=ORIENTED_EDGE('',*,*,#38186,.T.) ;
#50770=ORIENTED_EDGE('',*,*,#38192,.F.) ;
#50771=ORIENTED_EDGE('',*,*,#38193,.F.) ;
#50772=ORIENTED_EDGE('',*,*,#38187,.T.) ;
#50773=ORIENTED_EDGE('',*,*,#37942,.F.) ;
#50774=ORIENTED_EDGE('',*,*,#38194,.F.) ;
#50775=ORIENTED_EDGE('',*,*,#37914,.F.) ;
#50776=ORIENTED_EDGE('',*,*,#38189,.T.) ;
#50777=ORIENTED_EDGE('',*,*,#37916,.F.) ;
#50778=ORIENTED_EDGE('',*,*,#38195,.F.) ;
#50779=ORIENTED_EDGE('',*,*,#38196,.F.) ;
#50780=ORIENTED_EDGE('',*,*,#38190,.T.) ;
#50781=ORIENTED_EDGE('',*,*,#38188,.T.) ;
#50782=ORIENTED_EDGE('',*,*,#38197,.F.) ;
#50783=ORIENTED_EDGE('',*,*,#37904,.T.) ;
#50784=ORIENTED_EDGE('',*,*,#38191,.T.) ;
#50785=ORIENTED_EDGE('',*,*,#37898,.T.) ;
#50786=ORIENTED_EDGE('',*,*,#38198,.F.) ;
#50787=ORIENTED_EDGE('',*,*,#38192,.T.) ;
#50788=ORIENTED_EDGE('',*,*,#38199,.F.) ;
#50789=ORIENTED_EDGE('',*,*,#38200,.F.) ;
#50790=ORIENTED_EDGE('',*,*,#37941,.F.) ;
#50791=ORIENTED_EDGE('',*,*,#38193,.T.) ;
#50792=ORIENTED_EDGE('',*,*,#38200,.T.) ;
#50793=ORIENTED_EDGE('',*,*,#37908,.T.) ;
#50794=ORIENTED_EDGE('',*,*,#38201,.F.) ;
#50795=ORIENTED_EDGE('',*,*,#38194,.T.) ;
#50796=ORIENTED_EDGE('',*,*,#38202,.F.) ;
#50797=ORIENTED_EDGE('',*,*,#38195,.T.) ;
#50798=ORIENTED_EDGE('',*,*,#38203,.F.) ;
#50799=ORIENTED_EDGE('',*,*,#38197,.T.) ;
#50800=ORIENTED_EDGE('',*,*,#38196,.T.) ;
#50801=ORIENTED_EDGE('',*,*,#38204,.F.) ;
#50802=ORIENTED_EDGE('',*,*,#37905,.F.) ;
#50803=ORIENTED_EDGE('',*,*,#38198,.T.) ;
#50804=ORIENTED_EDGE('',*,*,#37897,.F.) ;
#50805=ORIENTED_EDGE('',*,*,#38205,.F.) ;
#50806=ORIENTED_EDGE('',*,*,#37906,.F.) ;
#50807=ORIENTED_EDGE('',*,*,#38199,.T.) ;
#50808=ORIENTED_EDGE('',*,*,#37915,.F.) ;
#50809=ORIENTED_EDGE('',*,*,#38201,.T.) ;
#50810=ORIENTED_EDGE('',*,*,#38206,.F.) ;
#50811=ORIENTED_EDGE('',*,*,#38203,.T.) ;
#50812=ORIENTED_EDGE('',*,*,#38204,.T.) ;
#50813=ORIENTED_EDGE('',*,*,#38202,.T.) ;
#50814=ORIENTED_EDGE('',*,*,#38207,.F.) ;
#50815=ORIENTED_EDGE('',*,*,#37900,.T.) ;
#50816=ORIENTED_EDGE('',*,*,#38205,.T.) ;
#50817=ORIENTED_EDGE('',*,*,#37901,.F.) ;
#50818=ORIENTED_EDGE('',*,*,#38207,.T.) ;
#50819=ORIENTED_EDGE('',*,*,#38206,.T.) ;
#50820=ORIENTED_EDGE('',*,*,#37907,.F.) ;
#50821=ORIENTED_EDGE('',*,*,#38208,.F.) ;
#50822=ORIENTED_EDGE('',*,*,#37956,.F.) ;
#50823=ORIENTED_EDGE('',*,*,#37791,.F.) ;
#50824=ORIENTED_EDGE('',*,*,#37962,.F.) ;
#50825=ORIENTED_EDGE('',*,*,#38209,.F.) ;
#50826=ORIENTED_EDGE('',*,*,#38208,.T.) ;
#50827=ORIENTED_EDGE('',*,*,#38210,.F.) ;
#50828=ORIENTED_EDGE('',*,*,#37789,.F.) ;
#50829=ORIENTED_EDGE('',*,*,#37871,.F.) ;
#50830=ORIENTED_EDGE('',*,*,#38211,.F.) ;
#50831=ORIENTED_EDGE('',*,*,#37960,.F.) ;
#50832=ORIENTED_EDGE('',*,*,#38210,.T.) ;
#50833=ORIENTED_EDGE('',*,*,#37961,.F.) ;
#50834=ORIENTED_EDGE('',*,*,#38212,.F.) ;
#50835=ORIENTED_EDGE('',*,*,#37967,.F.) ;
#50836=ORIENTED_EDGE('',*,*,#38209,.T.) ;
#50837=ORIENTED_EDGE('',*,*,#37966,.F.) ;
#50838=ORIENTED_EDGE('',*,*,#38213,.F.) ;
#50839=ORIENTED_EDGE('',*,*,#37957,.F.) ;
#50840=ORIENTED_EDGE('',*,*,#37793,.F.) ;
#50841=ORIENTED_EDGE('',*,*,#37955,.F.) ;
#50842=ORIENTED_EDGE('',*,*,#38214,.F.) ;
#50843=ORIENTED_EDGE('',*,*,#37766,.F.) ;
#50844=ORIENTED_EDGE('',*,*,#37734,.F.) ;
#50845=ORIENTED_EDGE('',*,*,#38215,.T.) ;
#50846=ORIENTED_EDGE('',*,*,#37763,.F.) ;
#50847=ORIENTED_EDGE('',*,*,#38216,.F.) ;
#50848=ORIENTED_EDGE('',*,*,#38211,.T.) ;
#50849=ORIENTED_EDGE('',*,*,#37870,.T.) ;
#50850=ORIENTED_EDGE('',*,*,#38217,.F.) ;
#50851=ORIENTED_EDGE('',*,*,#38212,.T.) ;
#50852=ORIENTED_EDGE('',*,*,#38218,.F.) ;
#50853=ORIENTED_EDGE('',*,*,#38213,.T.) ;
#50854=ORIENTED_EDGE('',*,*,#38219,.F.) ;
#50855=ORIENTED_EDGE('',*,*,#38214,.T.) ;
#50856=ORIENTED_EDGE('',*,*,#37954,.T.) ;
#50857=ORIENTED_EDGE('',*,*,#38220,.F.) ;
#50858=ORIENTED_EDGE('',*,*,#38216,.T.) ;
#50859=ORIENTED_EDGE('',*,*,#38217,.T.) ;
#50860=ORIENTED_EDGE('',*,*,#37891,.F.) ;
#50861=ORIENTED_EDGE('',*,*,#38221,.F.) ;
#50862=ORIENTED_EDGE('',*,*,#37968,.F.) ;
#50863=ORIENTED_EDGE('',*,*,#38219,.T.) ;
#50864=ORIENTED_EDGE('',*,*,#37969,.F.) ;
#50865=ORIENTED_EDGE('',*,*,#38222,.F.) ;
#50866=ORIENTED_EDGE('',*,*,#37963,.F.) ;
#50867=ORIENTED_EDGE('',*,*,#38218,.T.) ;
#50868=ORIENTED_EDGE('',*,*,#37965,.F.) ;
#50869=ORIENTED_EDGE('',*,*,#38223,.F.) ;
#50870=ORIENTED_EDGE('',*,*,#37958,.F.) ;
#50871=ORIENTED_EDGE('',*,*,#38220,.T.) ;
#50872=ORIENTED_EDGE('',*,*,#37959,.F.) ;
#50873=ORIENTED_EDGE('',*,*,#38224,.F.) ;
#50874=ORIENTED_EDGE('',*,*,#37735,.F.) ;
#50875=ORIENTED_EDGE('',*,*,#37769,.F.) ;
#50876=ORIENTED_EDGE('',*,*,#38225,.T.) ;
#50877=ORIENTED_EDGE('',*,*,#37740,.F.) ;
#50878=ORIENTED_EDGE('',*,*,#38226,.F.) ;
#50879=ORIENTED_EDGE('',*,*,#37819,.F.) ;
#50880=ORIENTED_EDGE('',*,*,#37770,.F.) ;
#50881=ORIENTED_EDGE('',*,*,#38227,.F.) ;
#50882=ORIENTED_EDGE('',*,*,#37982,.F.) ;
#50883=ORIENTED_EDGE('',*,*,#37821,.F.) ;
#50884=ORIENTED_EDGE('',*,*,#37981,.F.) ;
#50885=ORIENTED_EDGE('',*,*,#38228,.F.) ;
#50886=ORIENTED_EDGE('',*,*,#37979,.F.) ;
#50887=ORIENTED_EDGE('',*,*,#38221,.T.) ;
#50888=ORIENTED_EDGE('',*,*,#37890,.T.) ;
#50889=ORIENTED_EDGE('',*,*,#38229,.F.) ;
#50890=ORIENTED_EDGE('',*,*,#38222,.T.) ;
#50891=ORIENTED_EDGE('',*,*,#38224,.T.) ;
#50892=ORIENTED_EDGE('',*,*,#38223,.T.) ;
#50893=ORIENTED_EDGE('',*,*,#37727,.F.) ;
#50894=ORIENTED_EDGE('',*,*,#38227,.T.) ;
#50895=ORIENTED_EDGE('',*,*,#38226,.T.) ;
#50896=ORIENTED_EDGE('',*,*,#38230,.F.) ;
#50897=ORIENTED_EDGE('',*,*,#37983,.T.) ;
#50898=ORIENTED_EDGE('',*,*,#38231,.F.) ;
#50899=ORIENTED_EDGE('',*,*,#38228,.T.) ;
#50900=ORIENTED_EDGE('',*,*,#38232,.F.) ;
#50901=ORIENTED_EDGE('',*,*,#38229,.T.) ;
#50902=ORIENTED_EDGE('',*,*,#37889,.F.) ;
#50903=ORIENTED_EDGE('',*,*,#38233,.F.) ;
#50904=ORIENTED_EDGE('',*,*,#37964,.F.) ;
#50905=ORIENTED_EDGE('',*,*,#38230,.T.) ;
#50906=ORIENTED_EDGE('',*,*,#37739,.F.) ;
#50907=ORIENTED_EDGE('',*,*,#38234,.F.) ;
#50908=ORIENTED_EDGE('',*,*,#37984,.F.) ;
#50909=ORIENTED_EDGE('',*,*,#38235,.F.) ;
#50910=ORIENTED_EDGE('',*,*,#37985,.F.) ;
#50911=ORIENTED_EDGE('',*,*,#38236,.F.) ;
#50912=ORIENTED_EDGE('',*,*,#37976,.F.) ;
#50913=ORIENTED_EDGE('',*,*,#38232,.T.) ;
#50914=ORIENTED_EDGE('',*,*,#37980,.F.) ;
#50915=ORIENTED_EDGE('',*,*,#38237,.F.) ;
#50916=ORIENTED_EDGE('',*,*,#37970,.F.) ;
#50917=ORIENTED_EDGE('',*,*,#38231,.T.) ;
#50918=ORIENTED_EDGE('',*,*,#37973,.F.) ;
#50919=ORIENTED_EDGE('',*,*,#38238,.F.) ;
#50920=ORIENTED_EDGE('',*,*,#37977,.F.) ;
#50921=ORIENTED_EDGE('',*,*,#37823,.F.) ;
#50922=ORIENTED_EDGE('',*,*,#37978,.F.) ;
#50923=ORIENTED_EDGE('',*,*,#38239,.F.) ;
#50924=ORIENTED_EDGE('',*,*,#37883,.F.) ;
#50925=ORIENTED_EDGE('',*,*,#37725,.T.) ;
#50926=ORIENTED_EDGE('',*,*,#38233,.T.) ;
#50927=ORIENTED_EDGE('',*,*,#38240,.F.) ;
#50928=ORIENTED_EDGE('',*,*,#37736,.T.) ;
#50929=ORIENTED_EDGE('',*,*,#38236,.T.) ;
#50930=ORIENTED_EDGE('',*,*,#38234,.T.) ;
#50931=ORIENTED_EDGE('',*,*,#37723,.F.) ;
#50932=ORIENTED_EDGE('',*,*,#38241,.F.) ;
#50933=ORIENTED_EDGE('',*,*,#38241,.T.) ;
#50934=ORIENTED_EDGE('',*,*,#37722,.F.) ;
#50935=ORIENTED_EDGE('',*,*,#38237,.T.) ;
#50936=ORIENTED_EDGE('',*,*,#38235,.T.) ;
#50937=ORIENTED_EDGE('',*,*,#38242,.F.) ;
#50938=ORIENTED_EDGE('',*,*,#38239,.T.) ;
#50939=ORIENTED_EDGE('',*,*,#38238,.T.) ;
#50940=ORIENTED_EDGE('',*,*,#38243,.F.) ;
#50941=ORIENTED_EDGE('',*,*,#37884,.T.) ;
#50942=ORIENTED_EDGE('',*,*,#38240,.T.) ;
#50943=ORIENTED_EDGE('',*,*,#37888,.F.) ;
#50944=ORIENTED_EDGE('',*,*,#38244,.F.) ;
#50945=ORIENTED_EDGE('',*,*,#37737,.F.) ;
#50946=ORIENTED_EDGE('',*,*,#38242,.T.) ;
#50947=ORIENTED_EDGE('',*,*,#37975,.F.) ;
#50948=ORIENTED_EDGE('',*,*,#38245,.F.) ;
#50949=ORIENTED_EDGE('',*,*,#37971,.F.) ;
#50950=ORIENTED_EDGE('',*,*,#38243,.T.) ;
#50951=ORIENTED_EDGE('',*,*,#37972,.F.) ;
#50952=ORIENTED_EDGE('',*,*,#38246,.F.) ;
#50953=ORIENTED_EDGE('',*,*,#37885,.F.) ;
#50954=ORIENTED_EDGE('',*,*,#37738,.T.) ;
#50955=ORIENTED_EDGE('',*,*,#38244,.T.) ;
#50956=ORIENTED_EDGE('',*,*,#38247,.F.) ;
#50957=ORIENTED_EDGE('',*,*,#37720,.T.) ;
#50958=ORIENTED_EDGE('',*,*,#38246,.T.) ;
#50959=ORIENTED_EDGE('',*,*,#38245,.T.) ;
#50960=ORIENTED_EDGE('',*,*,#38248,.F.) ;
#50961=ORIENTED_EDGE('',*,*,#37886,.T.) ;
#50962=ORIENTED_EDGE('',*,*,#38247,.T.) ;
#50963=ORIENTED_EDGE('',*,*,#37887,.F.) ;
#50964=ORIENTED_EDGE('',*,*,#38248,.T.) ;
#50965=ORIENTED_EDGE('',*,*,#37974,.F.) ;
#50966=ORIENTED_EDGE('',*,*,#37743,.F.) ;
#50967=ORIENTED_EDGE('',*,*,#38249,.T.) ;
#50968=ORIENTED_EDGE('',*,*,#38064,.F.) ;
#50969=ORIENTED_EDGE('',*,*,#38250,.F.) ;
#50970=ORIENTED_EDGE('',*,*,#38069,.F.) ;
#50971=ORIENTED_EDGE('',*,*,#38063,.F.) ;
#50972=ORIENTED_EDGE('',*,*,#38251,.T.) ;
#50973=ORIENTED_EDGE('',*,*,#38070,.F.) ;
#50974=ORIENTED_EDGE('',*,*,#38250,.T.) ;
#50975=ORIENTED_EDGE('',*,*,#38066,.F.) ;
#50976=ORIENTED_EDGE('',*,*,#38252,.T.) ;
#50977=ORIENTED_EDGE('',*,*,#37932,.F.) ;
#50978=ORIENTED_EDGE('',*,*,#38090,.F.) ;
#50979=ORIENTED_EDGE('',*,*,#38253,.F.) ;
#50980=ORIENTED_EDGE('',*,*,#38075,.F.) ;
#50981=ORIENTED_EDGE('',*,*,#38254,.T.) ;
#50982=ORIENTED_EDGE('',*,*,#38103,.F.) ;
#50983=ORIENTED_EDGE('',*,*,#38255,.F.) ;
#50984=ORIENTED_EDGE('',*,*,#38060,.F.) ;
#50985=ORIENTED_EDGE('',*,*,#38256,.T.) ;
#50986=ORIENTED_EDGE('',*,*,#37745,.F.) ;
#50987=ORIENTED_EDGE('',*,*,#38068,.F.) ;
#50988=ORIENTED_EDGE('',*,*,#38257,.F.) ;
#50989=ORIENTED_EDGE('',*,*,#38087,.F.) ;
#50990=ORIENTED_EDGE('',*,*,#38258,.T.) ;
#50991=ORIENTED_EDGE('',*,*,#38061,.F.) ;
#50992=ORIENTED_EDGE('',*,*,#38253,.T.) ;
#50993=ORIENTED_EDGE('',*,*,#38259,.F.) ;
#50994=ORIENTED_EDGE('',*,*,#38255,.T.) ;
#50995=ORIENTED_EDGE('',*,*,#38260,.F.) ;
#50996=ORIENTED_EDGE('',*,*,#38072,.F.) ;
#50997=ORIENTED_EDGE('',*,*,#38261,.T.) ;
#50998=ORIENTED_EDGE('',*,*,#38055,.F.) ;
#50999=ORIENTED_EDGE('',*,*,#38257,.T.) ;
#51000=ORIENTED_EDGE('',*,*,#38105,.F.) ;
#51001=ORIENTED_EDGE('',*,*,#38262,.T.) ;
#51002=ORIENTED_EDGE('',*,*,#38081,.F.) ;
#51003=ORIENTED_EDGE('',*,*,#38263,.F.) ;
#51004=ORIENTED_EDGE('',*,*,#38260,.T.) ;
#51005=ORIENTED_EDGE('',*,*,#38106,.F.) ;
#51006=ORIENTED_EDGE('',*,*,#38264,.F.) ;
#51007=ORIENTED_EDGE('',*,*,#38080,.F.) ;
#51008=ORIENTED_EDGE('',*,*,#38259,.T.) ;
#51009=ORIENTED_EDGE('',*,*,#38079,.F.) ;
#51010=ORIENTED_EDGE('',*,*,#38265,.F.) ;
#51011=ORIENTED_EDGE('',*,*,#38076,.F.) ;
#51012=ORIENTED_EDGE('',*,*,#38101,.F.) ;
#51013=ORIENTED_EDGE('',*,*,#38266,.T.) ;
#51014=ORIENTED_EDGE('',*,*,#38073,.F.) ;
#51015=ORIENTED_EDGE('',*,*,#38267,.F.) ;
#51016=ORIENTED_EDGE('',*,*,#38264,.T.) ;
#51017=ORIENTED_EDGE('',*,*,#38263,.T.) ;
#51018=ORIENTED_EDGE('',*,*,#38268,.F.) ;
#51019=ORIENTED_EDGE('',*,*,#38267,.T.) ;
#51020=ORIENTED_EDGE('',*,*,#38265,.T.) ;
#51021=ORIENTED_EDGE('',*,*,#38269,.F.) ;
#51022=ORIENTED_EDGE('',*,*,#38268,.T.) ;
#51023=ORIENTED_EDGE('',*,*,#38084,.F.) ;
#51024=ORIENTED_EDGE('',*,*,#38270,.F.) ;
#51025=ORIENTED_EDGE('',*,*,#38077,.F.) ;
#51026=ORIENTED_EDGE('',*,*,#38269,.T.) ;
#51027=ORIENTED_EDGE('',*,*,#38078,.F.) ;
#51028=ORIENTED_EDGE('',*,*,#38271,.F.) ;
#51029=ORIENTED_EDGE('',*,*,#38102,.F.) ;
#51030=ORIENTED_EDGE('',*,*,#38271,.T.) ;
#51031=ORIENTED_EDGE('',*,*,#38270,.T.) ;
#51032=ORIENTED_EDGE('',*,*,#38272,.F.) ;
#51033=ORIENTED_EDGE('',*,*,#38083,.F.) ;
#51034=ORIENTED_EDGE('',*,*,#38273,.T.) ;
#51035=ORIENTED_EDGE('',*,*,#38099,.F.) ;
#51036=ORIENTED_EDGE('',*,*,#38272,.T.) ;
#51037=ORIENTED_EDGE('',*,*,#38057,.F.) ;
#51038=ORIENTED_EDGE('',*,*,#38274,.T.) ;
#51039=ORIENTED_EDGE('',*,*,#38085,.F.) ;
#51040=ORIENTED_EDGE('',*,*,#38275,.F.) ;
#51041=ORIENTED_EDGE('',*,*,#37936,.F.) ;
#51042=ORIENTED_EDGE('',*,*,#38276,.T.) ;
#51043=ORIENTED_EDGE('',*,*,#38058,.F.) ;
#51044=ORIENTED_EDGE('',*,*,#38275,.T.) ;
#51045=ORIENTED_EDGE('',*,*,#38089,.F.) ;
#51046=ORIENTED_EDGE('',*,*,#38048,.F.) ;
#51047=ORIENTED_EDGE('',*,*,#38277,.T.) ;
#51048=ORIENTED_EDGE('',*,*,#38049,.F.) ;
#51049=ORIENTED_EDGE('',*,*,#37951,.F.) ;
#51050=ORIENTED_EDGE('',*,*,#38054,.F.) ;
#51051=ORIENTED_EDGE('',*,*,#38278,.T.) ;
#51052=ORIENTED_EDGE('',*,*,#38046,.F.) ;
#51053=ORIENTED_EDGE('',*,*,#37949,.F.) ;
#51054=ORIENTED_EDGE('',*,*,#38033,.F.) ;
#51055=ORIENTED_EDGE('',*,*,#38279,.T.) ;
#51056=ORIENTED_EDGE('',*,*,#38091,.F.) ;
#51057=ORIENTED_EDGE('',*,*,#38280,.F.) ;
#51058=ORIENTED_EDGE('',*,*,#38093,.F.) ;
#51059=ORIENTED_EDGE('',*,*,#38281,.T.) ;
#51060=ORIENTED_EDGE('',*,*,#38039,.F.) ;
#51061=ORIENTED_EDGE('',*,*,#38282,.F.) ;
#51062=ORIENTED_EDGE('',*,*,#38283,.F.) ;
#51063=ORIENTED_EDGE('',*,*,#38094,.F.) ;
#51064=ORIENTED_EDGE('',*,*,#38284,.F.) ;
#51065=ORIENTED_EDGE('',*,*,#38038,.F.) ;
#51066=ORIENTED_EDGE('',*,*,#38280,.T.) ;
#51067=ORIENTED_EDGE('',*,*,#38283,.T.) ;
#51068=ORIENTED_EDGE('',*,*,#38285,.F.) ;
#51069=ORIENTED_EDGE('',*,*,#38051,.F.) ;
#51070=ORIENTED_EDGE('',*,*,#38286,.T.) ;
#51071=ORIENTED_EDGE('',*,*,#38043,.F.) ;
#51072=ORIENTED_EDGE('',*,*,#37953,.F.) ;
#51073=ORIENTED_EDGE('',*,*,#38045,.F.) ;
#51074=ORIENTED_EDGE('',*,*,#38287,.T.) ;
#51075=ORIENTED_EDGE('',*,*,#38052,.F.) ;
#51076=ORIENTED_EDGE('',*,*,#37947,.F.) ;
#51077=ORIENTED_EDGE('',*,*,#38284,.T.) ;
#51078=ORIENTED_EDGE('',*,*,#38282,.T.) ;
#51079=ORIENTED_EDGE('',*,*,#38288,.F.) ;
#51080=ORIENTED_EDGE('',*,*,#38285,.T.) ;
#51081=ORIENTED_EDGE('',*,*,#38037,.F.) ;
#51082=ORIENTED_EDGE('',*,*,#38289,.F.) ;
#51083=ORIENTED_EDGE('',*,*,#38034,.F.) ;
#51084=ORIENTED_EDGE('',*,*,#38097,.F.) ;
#51085=ORIENTED_EDGE('',*,*,#38290,.T.) ;
#51086=ORIENTED_EDGE('',*,*,#38031,.F.) ;
#51087=ORIENTED_EDGE('',*,*,#38291,.F.) ;
#51088=ORIENTED_EDGE('',*,*,#38041,.F.) ;
#51089=ORIENTED_EDGE('',*,*,#38292,.T.) ;
#51090=ORIENTED_EDGE('',*,*,#38095,.F.) ;
#51091=ORIENTED_EDGE('',*,*,#38293,.F.) ;
#51092=ORIENTED_EDGE('',*,*,#38288,.T.) ;
#51093=ORIENTED_EDGE('',*,*,#38042,.F.) ;
#51094=ORIENTED_EDGE('',*,*,#38294,.F.) ;
#51095=ORIENTED_EDGE('',*,*,#38035,.F.) ;
#51096=ORIENTED_EDGE('',*,*,#38291,.T.) ;
#51097=ORIENTED_EDGE('',*,*,#38289,.T.) ;
#51098=ORIENTED_EDGE('',*,*,#38295,.F.) ;
#51099=ORIENTED_EDGE('',*,*,#38294,.T.) ;
#51100=ORIENTED_EDGE('',*,*,#38293,.T.) ;
#51101=ORIENTED_EDGE('',*,*,#38296,.F.) ;
#51102=ORIENTED_EDGE('',*,*,#38295,.T.) ;
#51103=ORIENTED_EDGE('',*,*,#38036,.F.) ;
#51104=ORIENTED_EDGE('',*,*,#38296,.T.) ;
#51105=ORIENTED_EDGE('',*,*,#38098,.F.) ;
#51106=ORIENTED_EDGE('',*,*,#37780,.F.) ;
#51107=ORIENTED_EDGE('',*,*,#37756,.F.) ;
#51108=ORIENTED_EDGE('',*,*,#38297,.F.) ;
#51109=ORIENTED_EDGE('',*,*,#37762,.F.) ;
#51110=ORIENTED_EDGE('',*,*,#38018,.F.) ;
#51111=ORIENTED_EDGE('',*,*,#38298,.T.) ;
#51112=ORIENTED_EDGE('',*,*,#37757,.F.) ;
#51113=ORIENTED_EDGE('',*,*,#38299,.F.) ;
#51114=ORIENTED_EDGE('',*,*,#38299,.T.) ;
#51115=ORIENTED_EDGE('',*,*,#38297,.T.) ;
#51116=ORIENTED_EDGE('',*,*,#38300,.F.) ;
#51117=ORIENTED_EDGE('',*,*,#37779,.F.) ;
#51118=ORIENTED_EDGE('',*,*,#37752,.F.) ;
#51119=ORIENTED_EDGE('',*,*,#38301,.F.) ;
#51120=ORIENTED_EDGE('',*,*,#37754,.F.) ;
#51121=ORIENTED_EDGE('',*,*,#38300,.T.) ;
#51122=ORIENTED_EDGE('',*,*,#37755,.F.) ;
#51123=ORIENTED_EDGE('',*,*,#38302,.F.) ;
#51124=ORIENTED_EDGE('',*,*,#38019,.F.) ;
#51125=ORIENTED_EDGE('',*,*,#38302,.T.) ;
#51126=ORIENTED_EDGE('',*,*,#38301,.T.) ;
#51127=ORIENTED_EDGE('',*,*,#38303,.F.) ;
#51128=ORIENTED_EDGE('',*,*,#37751,.F.) ;
#51129=ORIENTED_EDGE('',*,*,#38304,.T.) ;
#51130=ORIENTED_EDGE('',*,*,#38016,.F.) ;
#51131=ORIENTED_EDGE('',*,*,#38303,.T.) ;
#51132=ORIENTED_EDGE('',*,*,#37855,.F.) ;
#51133=ORIENTED_EDGE('',*,*,#37707,.T.) ;
#51134=ORIENTED_EDGE('',*,*,#38305,.T.) ;
#51135=ORIENTED_EDGE('',*,*,#38027,.F.) ;
#51136=ORIENTED_EDGE('',*,*,#38306,.F.) ;
#51137=ORIENTED_EDGE('',*,*,#37833,.F.) ;
#51138=ORIENTED_EDGE('',*,*,#37856,.F.) ;
#51139=ORIENTED_EDGE('',*,*,#38307,.F.) ;
#51140=ORIENTED_EDGE('',*,*,#37853,.F.) ;
#51141=ORIENTED_EDGE('',*,*,#38307,.T.) ;
#51142=ORIENTED_EDGE('',*,*,#38306,.T.) ;
#51143=ORIENTED_EDGE('',*,*,#38308,.F.) ;
#51144=ORIENTED_EDGE('',*,*,#38308,.T.) ;
#51145=ORIENTED_EDGE('',*,*,#38030,.F.) ;
#51146=ORIENTED_EDGE('',*,*,#38309,.F.) ;
#51147=ORIENTED_EDGE('',*,*,#37851,.F.) ;
#51148=ORIENTED_EDGE('',*,*,#37835,.F.) ;
#51149=ORIENTED_EDGE('',*,*,#37852,.F.) ;
#51150=ORIENTED_EDGE('',*,*,#38310,.F.) ;
#51151=ORIENTED_EDGE('',*,*,#37849,.F.) ;
#51152=ORIENTED_EDGE('',*,*,#38310,.T.) ;
#51153=ORIENTED_EDGE('',*,*,#38309,.T.) ;
#51154=ORIENTED_EDGE('',*,*,#38311,.F.) ;
#51155=ORIENTED_EDGE('',*,*,#38029,.F.) ;
#51156=ORIENTED_EDGE('',*,*,#37711,.T.) ;
#51157=ORIENTED_EDGE('',*,*,#38312,.T.) ;
#51158=ORIENTED_EDGE('',*,*,#37850,.F.) ;
#51159=ORIENTED_EDGE('',*,*,#38311,.T.) ;
#51160=ORIENTED_EDGE('',*,*,#37930,.F.) ;
#51161=ORIENTED_EDGE('',*,*,#38313,.T.) ;
#51162=ORIENTED_EDGE('',*,*,#37741,.F.) ;
#51163=ORIENTED_EDGE('',*,*,#38314,.T.) ;
#51164=ORIENTED_EDGE('',*,*,#37800,.F.) ;
#51165=ORIENTED_EDGE('',*,*,#37902,.F.) ;
#51166=ORIENTED_EDGE('',*,*,#37812,.F.) ;
#51167=ORIENTED_EDGE('',*,*,#37836,.F.) ;
#51168=ORIENTED_EDGE('',*,*,#37802,.F.) ;
#51169=ORIENTED_EDGE('',*,*,#37837,.F.) ;
#51170=ORIENTED_EDGE('',*,*,#37810,.F.) ;
#51171=ORIENTED_EDGE('',*,*,#37838,.F.) ;
#51172=ORIENTED_EDGE('',*,*,#37804,.F.) ;
#51173=ORIENTED_EDGE('',*,*,#37839,.F.) ;
#51174=ORIENTED_EDGE('',*,*,#37808,.F.) ;
#51175=ORIENTED_EDGE('',*,*,#37842,.F.) ;
#51176=ORIENTED_EDGE('',*,*,#37797,.F.) ;
#51177=ORIENTED_EDGE('',*,*,#37772,.F.) ;
#51178=ORIENTED_EDGE('',*,*,#37815,.F.) ;
#51179=ORIENTED_EDGE('',*,*,#37895,.F.) ;
#51180=ORIENTED_EDGE('',*,*,#38115,.F.) ;
#51181=ORIENTED_EDGE('',*,*,#38315,.T.) ;
#51182=ORIENTED_EDGE('',*,*,#37774,.F.) ;
#51183=ORIENTED_EDGE('',*,*,#37796,.F.) ;
#51184=ORIENTED_EDGE('',*,*,#38110,.F.) ;
#51185=ORIENTED_EDGE('',*,*,#38316,.T.) ;
#51186=ORIENTED_EDGE('',*,*,#37775,.F.) ;
#51187=ORIENTED_EDGE('',*,*,#38317,.T.) ;
#51188=ORIENTED_EDGE('',*,*,#37776,.F.) ;
#51189=ORIENTED_EDGE('',*,*,#38318,.T.) ;
#51190=ORIENTED_EDGE('',*,*,#38107,.F.) ;
#51191=ORIENTED_EDGE('',*,*,#37816,.F.) ;
#51192=ORIENTED_EDGE('',*,*,#38155,.F.) ;
#51193=ORIENTED_EDGE('',*,*,#38161,.F.) ;
#51194=ORIENTED_EDGE('',*,*,#38160,.F.) ;
#51195=ORIENTED_EDGE('',*,*,#38319,.F.) ;
#51196=ORIENTED_EDGE('',*,*,#38156,.F.) ;
#51197=ORIENTED_EDGE('',*,*,#38249,.F.) ;
#51198=ORIENTED_EDGE('',*,*,#37742,.F.) ;
#51199=ORIENTED_EDGE('',*,*,#38320,.F.) ;
#51200=ORIENTED_EDGE('',*,*,#37924,.F.) ;
#51201=ORIENTED_EDGE('',*,*,#38319,.T.) ;
#51202=ORIENTED_EDGE('',*,*,#37933,.F.) ;
#51203=ORIENTED_EDGE('',*,*,#38252,.F.) ;
#51204=ORIENTED_EDGE('',*,*,#38065,.F.) ;
#51205=ORIENTED_EDGE('',*,*,#38320,.T.) ;
#51206=ORIENTED_EDGE('',*,*,#38313,.F.) ;
#51207=ORIENTED_EDGE('',*,*,#38321,.F.) ;
#51208=ORIENTED_EDGE('',*,*,#38321,.T.) ;
#51209=ORIENTED_EDGE('',*,*,#37929,.F.) ;
#51210=ORIENTED_EDGE('',*,*,#38322,.F.) ;
#51211=ORIENTED_EDGE('',*,*,#37925,.F.) ;
#51212=ORIENTED_EDGE('',*,*,#38164,.F.) ;
#51213=ORIENTED_EDGE('',*,*,#38158,.F.) ;
#51214=ORIENTED_EDGE('',*,*,#38157,.F.) ;
#51215=ORIENTED_EDGE('',*,*,#38322,.T.) ;
#51216=ORIENTED_EDGE('',*,*,#38165,.F.) ;
#51217=ORIENTED_EDGE('',*,*,#38177,.F.) ;
#51218=ORIENTED_EDGE('',*,*,#38167,.F.) ;
#51219=ORIENTED_EDGE('',*,*,#38166,.F.) ;
#51220=ORIENTED_EDGE('',*,*,#38323,.F.) ;
#51221=ORIENTED_EDGE('',*,*,#38178,.F.) ;
#51222=ORIENTED_EDGE('',*,*,#38323,.T.) ;
#51223=ORIENTED_EDGE('',*,*,#37931,.F.) ;
#51224=ORIENTED_EDGE('',*,*,#38324,.F.) ;
#51225=ORIENTED_EDGE('',*,*,#37921,.F.) ;
#51226=ORIENTED_EDGE('',*,*,#38324,.T.) ;
#51227=ORIENTED_EDGE('',*,*,#38314,.F.) ;
#51228=ORIENTED_EDGE('',*,*,#38325,.F.) ;
#51229=ORIENTED_EDGE('',*,*,#38276,.F.) ;
#51230=ORIENTED_EDGE('',*,*,#37935,.F.) ;
#51231=ORIENTED_EDGE('',*,*,#38326,.F.) ;
#51232=ORIENTED_EDGE('',*,*,#37922,.F.) ;
#51233=ORIENTED_EDGE('',*,*,#38325,.T.) ;
#51234=ORIENTED_EDGE('',*,*,#37746,.F.) ;
#51235=ORIENTED_EDGE('',*,*,#38256,.F.) ;
#51236=ORIENTED_EDGE('',*,*,#38059,.F.) ;
#51237=ORIENTED_EDGE('',*,*,#38326,.T.) ;
#51238=ORIENTED_EDGE('',*,*,#38163,.F.) ;
#51239=ORIENTED_EDGE('',*,*,#38162,.F.) ;
#51240=ORIENTED_EDGE('',*,*,#38175,.F.) ;
#51241=ORIENTED_EDGE('',*,*,#38174,.F.) ;
#51242=ORIENTED_EDGE('',*,*,#37750,.F.) ;
#51243=ORIENTED_EDGE('',*,*,#38327,.T.) ;
#51244=ORIENTED_EDGE('',*,*,#38020,.F.) ;
#51245=ORIENTED_EDGE('',*,*,#38328,.F.) ;
#51246=ORIENTED_EDGE('',*,*,#38304,.F.) ;
#51247=ORIENTED_EDGE('',*,*,#38328,.T.) ;
#51248=ORIENTED_EDGE('',*,*,#38026,.F.) ;
#51249=ORIENTED_EDGE('',*,*,#38329,.F.) ;
#51250=ORIENTED_EDGE('',*,*,#38017,.F.) ;
#51251=ORIENTED_EDGE('',*,*,#38329,.T.) ;
#51252=ORIENTED_EDGE('',*,*,#38025,.F.) ;
#51253=ORIENTED_EDGE('',*,*,#38330,.F.) ;
#51254=ORIENTED_EDGE('',*,*,#38331,.F.) ;
#51255=ORIENTED_EDGE('',*,*,#38332,.F.) ;
#51256=ORIENTED_EDGE('',*,*,#38333,.F.) ;
#51257=ORIENTED_EDGE('',*,*,#37758,.F.) ;
#51258=ORIENTED_EDGE('',*,*,#38298,.F.) ;
#51259=ORIENTED_EDGE('',*,*,#37781,.F.) ;
#51260=ORIENTED_EDGE('',*,*,#37760,.F.) ;
#51261=ORIENTED_EDGE('',*,*,#38334,.F.) ;
#51262=ORIENTED_EDGE('',*,*,#37858,.F.) ;
#51263=ORIENTED_EDGE('',*,*,#37759,.F.) ;
#51264=ORIENTED_EDGE('',*,*,#38333,.T.) ;
#51265=ORIENTED_EDGE('',*,*,#38332,.T.) ;
#51266=ORIENTED_EDGE('',*,*,#38331,.T.) ;
#51267=ORIENTED_EDGE('',*,*,#38330,.T.) ;
#51268=ORIENTED_EDGE('',*,*,#38335,.F.) ;
#51269=ORIENTED_EDGE('',*,*,#37859,.F.) ;
#51270=ORIENTED_EDGE('',*,*,#38334,.T.) ;
#51271=ORIENTED_EDGE('',*,*,#37710,.F.) ;
#51272=ORIENTED_EDGE('',*,*,#38336,.T.) ;
#51273=ORIENTED_EDGE('',*,*,#37846,.F.) ;
#51274=ORIENTED_EDGE('',*,*,#38312,.F.) ;
#51275=ORIENTED_EDGE('',*,*,#38335,.T.) ;
#51276=ORIENTED_EDGE('',*,*,#38024,.F.) ;
#51277=ORIENTED_EDGE('',*,*,#38337,.F.) ;
#51278=ORIENTED_EDGE('',*,*,#37860,.F.) ;
#51279=ORIENTED_EDGE('',*,*,#37831,.F.) ;
#51280=ORIENTED_EDGE('',*,*,#37862,.F.) ;
#51281=ORIENTED_EDGE('',*,*,#38338,.F.) ;
#51282=ORIENTED_EDGE('',*,*,#37857,.F.) ;
#51283=ORIENTED_EDGE('',*,*,#37712,.T.) ;
#51284=ORIENTED_EDGE('',*,*,#38028,.F.) ;
#51285=ORIENTED_EDGE('',*,*,#38339,.F.) ;
#51286=ORIENTED_EDGE('',*,*,#38022,.F.) ;
#51287=ORIENTED_EDGE('',*,*,#37861,.F.) ;
#51288=ORIENTED_EDGE('',*,*,#38337,.T.) ;
#51289=ORIENTED_EDGE('',*,*,#38340,.F.) ;
#51290=ORIENTED_EDGE('',*,*,#38341,.F.) ;
#51291=ORIENTED_EDGE('',*,*,#38342,.F.) ;
#51292=ORIENTED_EDGE('',*,*,#37705,.F.) ;
#51293=ORIENTED_EDGE('',*,*,#37704,.F.) ;
#51294=ORIENTED_EDGE('',*,*,#37854,.F.) ;
#51295=ORIENTED_EDGE('',*,*,#38338,.T.) ;
#51296=ORIENTED_EDGE('',*,*,#37706,.F.) ;
#51297=ORIENTED_EDGE('',*,*,#38342,.T.) ;
#51298=ORIENTED_EDGE('',*,*,#38341,.T.) ;
#51299=ORIENTED_EDGE('',*,*,#38340,.T.) ;
#51300=ORIENTED_EDGE('',*,*,#38023,.F.) ;
#51301=ORIENTED_EDGE('',*,*,#38339,.T.) ;
#51302=ORIENTED_EDGE('',*,*,#38305,.F.) ;
#51303=ORIENTED_EDGE('',*,*,#38343,.F.) ;
#51304=ORIENTED_EDGE('',*,*,#37768,.F.) ;
#51305=ORIENTED_EDGE('',*,*,#37818,.F.) ;
#51306=ORIENTED_EDGE('',*,*,#38109,.F.) ;
#51307=ORIENTED_EDGE('',*,*,#38225,.F.) ;
#51308=ORIENTED_EDGE('',*,*,#38343,.T.) ;
#51309=ORIENTED_EDGE('',*,*,#38344,.F.) ;
#51310=ORIENTED_EDGE('',*,*,#37730,.F.) ;
#51311=ORIENTED_EDGE('',*,*,#38344,.T.) ;
#51312=ORIENTED_EDGE('',*,*,#38108,.F.) ;
#51313=ORIENTED_EDGE('',*,*,#38345,.F.) ;
#51314=ORIENTED_EDGE('',*,*,#38112,.F.) ;
#51315=ORIENTED_EDGE('',*,*,#38318,.F.) ;
#51316=ORIENTED_EDGE('',*,*,#38316,.F.) ;
#51317=ORIENTED_EDGE('',*,*,#38345,.T.) ;
#51318=ORIENTED_EDGE('',*,*,#38346,.T.) ;
#51319=ORIENTED_EDGE('',*,*,#38251,.F.) ;
#51320=ORIENTED_EDGE('',*,*,#38347,.F.) ;
#51321=ORIENTED_EDGE('',*,*,#38254,.F.) ;
#51322=ORIENTED_EDGE('',*,*,#38346,.F.) ;
#51323=ORIENTED_EDGE('',*,*,#38074,.F.) ;
#51324=ORIENTED_EDGE('',*,*,#38348,.F.) ;
#51325=ORIENTED_EDGE('',*,*,#38071,.F.) ;
#51326=ORIENTED_EDGE('',*,*,#38347,.T.) ;
#51327=ORIENTED_EDGE('',*,*,#38062,.F.) ;
#51328=ORIENTED_EDGE('',*,*,#38349,.F.) ;
#51329=ORIENTED_EDGE('',*,*,#38104,.F.) ;
#51330=ORIENTED_EDGE('',*,*,#38348,.T.) ;
#51331=ORIENTED_EDGE('',*,*,#38266,.F.) ;
#51332=ORIENTED_EDGE('',*,*,#38350,.F.) ;
#51333=ORIENTED_EDGE('',*,*,#38261,.F.) ;
#51334=ORIENTED_EDGE('',*,*,#38349,.T.) ;
#51335=ORIENTED_EDGE('',*,*,#38258,.F.) ;
#51336=ORIENTED_EDGE('',*,*,#38351,.F.) ;
#51337=ORIENTED_EDGE('',*,*,#38262,.F.) ;
#51338=ORIENTED_EDGE('',*,*,#38350,.T.) ;
#51339=ORIENTED_EDGE('',*,*,#38100,.F.) ;
#51340=ORIENTED_EDGE('',*,*,#38352,.F.) ;
#51341=ORIENTED_EDGE('',*,*,#38056,.F.) ;
#51342=ORIENTED_EDGE('',*,*,#38351,.T.) ;
#51343=ORIENTED_EDGE('',*,*,#38086,.F.) ;
#51344=ORIENTED_EDGE('',*,*,#38353,.F.) ;
#51345=ORIENTED_EDGE('',*,*,#38082,.F.) ;
#51346=ORIENTED_EDGE('',*,*,#38352,.T.) ;
#51347=ORIENTED_EDGE('',*,*,#38273,.F.) ;
#51348=ORIENTED_EDGE('',*,*,#38353,.T.) ;
#51349=ORIENTED_EDGE('',*,*,#38274,.F.) ;
#51350=ORIENTED_EDGE('',*,*,#38354,.T.) ;
#51351=ORIENTED_EDGE('',*,*,#38277,.F.) ;
#51352=ORIENTED_EDGE('',*,*,#38355,.F.) ;
#51353=ORIENTED_EDGE('',*,*,#38279,.F.) ;
#51354=ORIENTED_EDGE('',*,*,#38354,.F.) ;
#51355=ORIENTED_EDGE('',*,*,#38032,.F.) ;
#51356=ORIENTED_EDGE('',*,*,#38356,.F.) ;
#51357=ORIENTED_EDGE('',*,*,#38050,.F.) ;
#51358=ORIENTED_EDGE('',*,*,#38355,.T.) ;
#51359=ORIENTED_EDGE('',*,*,#38047,.F.) ;
#51360=ORIENTED_EDGE('',*,*,#38357,.F.) ;
#51361=ORIENTED_EDGE('',*,*,#38092,.F.) ;
#51362=ORIENTED_EDGE('',*,*,#38356,.T.) ;
#51363=ORIENTED_EDGE('',*,*,#38290,.F.) ;
#51364=ORIENTED_EDGE('',*,*,#38358,.F.) ;
#51365=ORIENTED_EDGE('',*,*,#38286,.F.) ;
#51366=ORIENTED_EDGE('',*,*,#38357,.T.) ;
#51367=ORIENTED_EDGE('',*,*,#38278,.F.) ;
#51368=ORIENTED_EDGE('',*,*,#38359,.F.) ;
#51369=ORIENTED_EDGE('',*,*,#38281,.F.) ;
#51370=ORIENTED_EDGE('',*,*,#38358,.T.) ;
#51371=ORIENTED_EDGE('',*,*,#38096,.F.) ;
#51372=ORIENTED_EDGE('',*,*,#38360,.F.) ;
#51373=ORIENTED_EDGE('',*,*,#38044,.F.) ;
#51374=ORIENTED_EDGE('',*,*,#38359,.T.) ;
#51375=ORIENTED_EDGE('',*,*,#38053,.F.) ;
#51376=ORIENTED_EDGE('',*,*,#38361,.F.) ;
#51377=ORIENTED_EDGE('',*,*,#38040,.F.) ;
#51378=ORIENTED_EDGE('',*,*,#38360,.T.) ;
#51379=ORIENTED_EDGE('',*,*,#38292,.F.) ;
#51380=ORIENTED_EDGE('',*,*,#38361,.T.) ;
#51381=ORIENTED_EDGE('',*,*,#38287,.F.) ;
#51382=ORIENTED_EDGE('',*,*,#37794,.F.) ;
#51383=ORIENTED_EDGE('',*,*,#37764,.F.) ;
#51384=ORIENTED_EDGE('',*,*,#38362,.F.) ;
#51385=ORIENTED_EDGE('',*,*,#38113,.F.) ;
#51386=ORIENTED_EDGE('',*,*,#38362,.T.) ;
#51387=ORIENTED_EDGE('',*,*,#38215,.F.) ;
#51388=ORIENTED_EDGE('',*,*,#37732,.F.) ;
#51389=ORIENTED_EDGE('',*,*,#38363,.F.) ;
#51390=ORIENTED_EDGE('',*,*,#38363,.T.) ;
#51391=ORIENTED_EDGE('',*,*,#38111,.F.) ;
#51392=ORIENTED_EDGE('',*,*,#38364,.F.) ;
#51393=ORIENTED_EDGE('',*,*,#38114,.F.) ;
#51394=ORIENTED_EDGE('',*,*,#38317,.F.) ;
#51395=ORIENTED_EDGE('',*,*,#38315,.F.) ;
#51396=ORIENTED_EDGE('',*,*,#38364,.T.) ;
#51397=ORIENTED_EDGE('',*,*,#37848,.F.) ;
#51398=ORIENTED_EDGE('',*,*,#38365,.F.) ;
#51399=ORIENTED_EDGE('',*,*,#37843,.F.) ;
#51400=ORIENTED_EDGE('',*,*,#37806,.F.) ;
#51401=ORIENTED_EDGE('',*,*,#37847,.F.) ;
#51402=ORIENTED_EDGE('',*,*,#38336,.F.) ;
#51403=ORIENTED_EDGE('',*,*,#37709,.F.) ;
#51404=ORIENTED_EDGE('',*,*,#38366,.F.) ;
#51405=ORIENTED_EDGE('',*,*,#37844,.F.) ;
#51406=ORIENTED_EDGE('',*,*,#38365,.T.) ;
#51407=ORIENTED_EDGE('',*,*,#38366,.T.) ;
#51408=ORIENTED_EDGE('',*,*,#38021,.F.) ;
#51409=ORIENTED_EDGE('',*,*,#38367,.F.) ;
#51410=ORIENTED_EDGE('',*,*,#37845,.F.) ;
#51411=ORIENTED_EDGE('',*,*,#38327,.F.) ;
#51412=ORIENTED_EDGE('',*,*,#37749,.F.) ;
#51413=ORIENTED_EDGE('',*,*,#38368,.F.) ;
#51414=ORIENTED_EDGE('',*,*,#37840,.F.) ;
#51415=ORIENTED_EDGE('',*,*,#38367,.T.) ;
#51416=ORIENTED_EDGE('',*,*,#37778,.F.) ;
#51417=ORIENTED_EDGE('',*,*,#37841,.F.) ;
#51418=ORIENTED_EDGE('',*,*,#38368,.T.) ;
#51419=ORIENTED_EDGE('',*,*,#37748,.F.) ;
#51420=ORIENTED_EDGE('',*,*,#38369,.T.) ;
#51421=ORIENTED_EDGE('',*,*,#38370,.T.) ;
#51422=ORIENTED_EDGE('',*,*,#38371,.T.) ;
#51423=ORIENTED_EDGE('',*,*,#38372,.F.) ;
#51424=ORIENTED_EDGE('',*,*,#38373,.F.) ;
#51425=ORIENTED_EDGE('',*,*,#38374,.T.) ;
#51426=ORIENTED_EDGE('',*,*,#38375,.T.) ;
#51427=ORIENTED_EDGE('',*,*,#38376,.F.) ;
#51428=ORIENTED_EDGE('',*,*,#38377,.F.) ;
#51429=ORIENTED_EDGE('',*,*,#38378,.F.) ;
#51430=ORIENTED_EDGE('',*,*,#38379,.F.) ;
#51431=ORIENTED_EDGE('',*,*,#38380,.T.) ;
#51432=ORIENTED_EDGE('',*,*,#38381,.F.) ;
#51433=ORIENTED_EDGE('',*,*,#38380,.F.) ;
#51434=ORIENTED_EDGE('',*,*,#38382,.F.) ;
#51435=ORIENTED_EDGE('',*,*,#38383,.T.) ;
#51436=ORIENTED_EDGE('',*,*,#38384,.F.) ;
#51437=ORIENTED_EDGE('',*,*,#38383,.F.) ;
#51438=ORIENTED_EDGE('',*,*,#38385,.F.) ;
#51439=ORIENTED_EDGE('',*,*,#38386,.F.) ;
#51440=ORIENTED_EDGE('',*,*,#38387,.T.) ;
#51441=ORIENTED_EDGE('',*,*,#38388,.T.) ;
#51442=ORIENTED_EDGE('',*,*,#38389,.F.) ;
#51443=ORIENTED_EDGE('',*,*,#38390,.F.) ;
#51444=ORIENTED_EDGE('',*,*,#38391,.F.) ;
#51445=ORIENTED_EDGE('',*,*,#38392,.T.) ;
#51446=ORIENTED_EDGE('',*,*,#38393,.F.) ;
#51447=ORIENTED_EDGE('',*,*,#38394,.F.) ;
#51448=ORIENTED_EDGE('',*,*,#38395,.T.) ;
#51449=ORIENTED_EDGE('',*,*,#38396,.F.) ;
#51450=ORIENTED_EDGE('',*,*,#38397,.T.) ;
#51451=ORIENTED_EDGE('',*,*,#38381,.T.) ;
#51452=ORIENTED_EDGE('',*,*,#38398,.T.) ;
#51453=ORIENTED_EDGE('',*,*,#38382,.T.) ;
#51454=ORIENTED_EDGE('',*,*,#38398,.F.) ;
#51455=ORIENTED_EDGE('',*,*,#38394,.T.) ;
#51456=ORIENTED_EDGE('',*,*,#38399,.T.) ;
#51457=ORIENTED_EDGE('',*,*,#38400,.T.) ;
#51458=ORIENTED_EDGE('',*,*,#38391,.T.) ;
#51459=ORIENTED_EDGE('',*,*,#38401,.F.) ;
#51460=ORIENTED_EDGE('',*,*,#38402,.T.) ;
#51461=ORIENTED_EDGE('',*,*,#38403,.F.) ;
#51462=ORIENTED_EDGE('',*,*,#38389,.T.) ;
#51463=ORIENTED_EDGE('',*,*,#38404,.T.) ;
#51464=ORIENTED_EDGE('',*,*,#38405,.T.) ;
#51465=ORIENTED_EDGE('',*,*,#38406,.T.) ;
#51466=ORIENTED_EDGE('',*,*,#38407,.T.) ;
#51467=ORIENTED_EDGE('',*,*,#38408,.T.) ;
#51468=ORIENTED_EDGE('',*,*,#38409,.T.) ;
#51469=ORIENTED_EDGE('',*,*,#38410,.T.) ;
#51470=ORIENTED_EDGE('',*,*,#38411,.T.) ;
#51471=ORIENTED_EDGE('',*,*,#38412,.T.) ;
#51472=ORIENTED_EDGE('',*,*,#38413,.T.) ;
#51473=ORIENTED_EDGE('',*,*,#38414,.T.) ;
#51474=ORIENTED_EDGE('',*,*,#38415,.T.) ;
#51475=ORIENTED_EDGE('',*,*,#38416,.T.) ;
#51476=ORIENTED_EDGE('',*,*,#38417,.T.) ;
#51477=ORIENTED_EDGE('',*,*,#38418,.T.) ;
#51478=ORIENTED_EDGE('',*,*,#38419,.T.) ;
#51479=ORIENTED_EDGE('',*,*,#38420,.T.) ;
#51480=ORIENTED_EDGE('',*,*,#38421,.T.) ;
#51481=ORIENTED_EDGE('',*,*,#38422,.T.) ;
#51482=ORIENTED_EDGE('',*,*,#38423,.T.) ;
#51483=ORIENTED_EDGE('',*,*,#38424,.T.) ;
#51484=ORIENTED_EDGE('',*,*,#38425,.T.) ;
#51485=ORIENTED_EDGE('',*,*,#38426,.T.) ;
#51486=ORIENTED_EDGE('',*,*,#38427,.T.) ;
#51487=ORIENTED_EDGE('',*,*,#38428,.T.) ;
#51488=ORIENTED_EDGE('',*,*,#38429,.T.) ;
#51489=ORIENTED_EDGE('',*,*,#38430,.T.) ;
#51490=ORIENTED_EDGE('',*,*,#38431,.T.) ;
#51491=ORIENTED_EDGE('',*,*,#38432,.F.) ;
#51492=ORIENTED_EDGE('',*,*,#38433,.T.) ;
#51493=ORIENTED_EDGE('',*,*,#38434,.T.) ;
#51494=ORIENTED_EDGE('',*,*,#38435,.T.) ;
#51495=ORIENTED_EDGE('',*,*,#38436,.F.) ;
#51496=ORIENTED_EDGE('',*,*,#38437,.T.) ;
#51497=ORIENTED_EDGE('',*,*,#38438,.T.) ;
#51498=ORIENTED_EDGE('',*,*,#38439,.T.) ;
#51499=ORIENTED_EDGE('',*,*,#38440,.T.) ;
#51500=ORIENTED_EDGE('',*,*,#38441,.T.) ;
#51501=ORIENTED_EDGE('',*,*,#38442,.F.) ;
#51502=ORIENTED_EDGE('',*,*,#38443,.T.) ;
#51503=ORIENTED_EDGE('',*,*,#38412,.F.) ;
#51504=ORIENTED_EDGE('',*,*,#38444,.T.) ;
#51505=ORIENTED_EDGE('',*,*,#38418,.F.) ;
#51506=ORIENTED_EDGE('',*,*,#38445,.T.) ;
#51507=ORIENTED_EDGE('',*,*,#38426,.F.) ;
#51508=ORIENTED_EDGE('',*,*,#38446,.T.) ;
#51509=ORIENTED_EDGE('',*,*,#38447,.F.) ;
#51510=ORIENTED_EDGE('',*,*,#38448,.T.) ;
#51511=ORIENTED_EDGE('',*,*,#38449,.F.) ;
#51512=ORIENTED_EDGE('',*,*,#38450,.T.) ;
#51513=ORIENTED_EDGE('',*,*,#38451,.T.) ;
#51514=ORIENTED_EDGE('',*,*,#38452,.T.) ;
#51515=ORIENTED_EDGE('',*,*,#38453,.F.) ;
#51516=ORIENTED_EDGE('',*,*,#38454,.T.) ;
#51517=ORIENTED_EDGE('',*,*,#38455,.T.) ;
#51518=ORIENTED_EDGE('',*,*,#38456,.T.) ;
#51519=ORIENTED_EDGE('',*,*,#38457,.F.) ;
#51520=ORIENTED_EDGE('',*,*,#38458,.T.) ;
#51521=ORIENTED_EDGE('',*,*,#38430,.F.) ;
#51522=ORIENTED_EDGE('',*,*,#38459,.T.) ;
#51523=ORIENTED_EDGE('',*,*,#38460,.T.) ;
#51524=ORIENTED_EDGE('',*,*,#38461,.T.) ;
#51525=ORIENTED_EDGE('',*,*,#38438,.F.) ;
#51526=ORIENTED_EDGE('',*,*,#38462,.T.) ;
#51527=ORIENTED_EDGE('',*,*,#38463,.F.) ;
#51528=ORIENTED_EDGE('',*,*,#38464,.F.) ;
#51529=ORIENTED_EDGE('',*,*,#38465,.T.) ;
#51530=ORIENTED_EDGE('',*,*,#38466,.F.) ;
#51531=ORIENTED_EDGE('',*,*,#38467,.T.) ;
#51532=ORIENTED_EDGE('',*,*,#38468,.F.) ;
#51533=ORIENTED_EDGE('',*,*,#38469,.T.) ;
#51534=ORIENTED_EDGE('',*,*,#38470,.T.) ;
#51535=ORIENTED_EDGE('',*,*,#38471,.T.) ;
#51536=ORIENTED_EDGE('',*,*,#38472,.T.) ;
#51537=ORIENTED_EDGE('',*,*,#38473,.T.) ;
#51538=ORIENTED_EDGE('',*,*,#38474,.T.) ;
#51539=ORIENTED_EDGE('',*,*,#38475,.T.) ;
#51540=ORIENTED_EDGE('',*,*,#38476,.T.) ;
#51541=ORIENTED_EDGE('',*,*,#38477,.T.) ;
#51542=ORIENTED_EDGE('',*,*,#38478,.T.) ;
#51543=ORIENTED_EDGE('',*,*,#38479,.T.) ;
#51544=ORIENTED_EDGE('',*,*,#38480,.T.) ;
#51545=ORIENTED_EDGE('',*,*,#38436,.T.) ;
#51546=ORIENTED_EDGE('',*,*,#38481,.T.) ;
#51547=ORIENTED_EDGE('',*,*,#38482,.T.) ;
#51548=ORIENTED_EDGE('',*,*,#38483,.T.) ;
#51549=ORIENTED_EDGE('',*,*,#38432,.T.) ;
#51550=ORIENTED_EDGE('',*,*,#38484,.T.) ;
#51551=ORIENTED_EDGE('',*,*,#38485,.F.) ;
#51552=ORIENTED_EDGE('',*,*,#38486,.T.) ;
#51553=ORIENTED_EDGE('',*,*,#38487,.F.) ;
#51554=ORIENTED_EDGE('',*,*,#38488,.T.) ;
#51555=ORIENTED_EDGE('',*,*,#38489,.T.) ;
#51556=ORIENTED_EDGE('',*,*,#38490,.T.) ;
#51557=ORIENTED_EDGE('',*,*,#38491,.F.) ;
#51558=ORIENTED_EDGE('',*,*,#38492,.T.) ;
#51559=ORIENTED_EDGE('',*,*,#38493,.F.) ;
#51560=ORIENTED_EDGE('',*,*,#38494,.T.) ;
#51561=ORIENTED_EDGE('',*,*,#38495,.T.) ;
#51562=ORIENTED_EDGE('',*,*,#38496,.T.) ;
#51563=ORIENTED_EDGE('',*,*,#38497,.T.) ;
#51564=ORIENTED_EDGE('',*,*,#38498,.T.) ;
#51565=ORIENTED_EDGE('',*,*,#38499,.T.) ;
#51566=ORIENTED_EDGE('',*,*,#38500,.T.) ;
#51567=ORIENTED_EDGE('',*,*,#38466,.T.) ;
#51568=ORIENTED_EDGE('',*,*,#38501,.T.) ;
#51569=ORIENTED_EDGE('',*,*,#38476,.F.) ;
#51570=ORIENTED_EDGE('',*,*,#38502,.T.) ;
#51571=ORIENTED_EDGE('',*,*,#38468,.T.) ;
#51572=ORIENTED_EDGE('',*,*,#38503,.T.) ;
#51573=ORIENTED_EDGE('',*,*,#38474,.F.) ;
#51574=ORIENTED_EDGE('',*,*,#38504,.T.) ;
#51575=ORIENTED_EDGE('',*,*,#38505,.T.) ;
#51576=ORIENTED_EDGE('',*,*,#38506,.T.) ;
#51577=ORIENTED_EDGE('',*,*,#38442,.T.) ;
#51578=ORIENTED_EDGE('',*,*,#38507,.T.) ;
#51579=ORIENTED_EDGE('',*,*,#38472,.F.) ;
#51580=ORIENTED_EDGE('',*,*,#38508,.T.) ;
#51581=ORIENTED_EDGE('',*,*,#38509,.T.) ;
#51582=ORIENTED_EDGE('',*,*,#38510,.T.) ;
#51583=ORIENTED_EDGE('',*,*,#38511,.T.) ;
#51584=ORIENTED_EDGE('',*,*,#38512,.T.) ;
#51585=ORIENTED_EDGE('',*,*,#38513,.T.) ;
#51586=ORIENTED_EDGE('',*,*,#38470,.F.) ;
#51587=ORIENTED_EDGE('',*,*,#38514,.T.) ;
#51588=ORIENTED_EDGE('',*,*,#38515,.T.) ;
#51589=ORIENTED_EDGE('',*,*,#38516,.T.) ;
#51590=ORIENTED_EDGE('',*,*,#38517,.T.) ;
#51591=ORIENTED_EDGE('',*,*,#38499,.F.) ;
#51592=ORIENTED_EDGE('',*,*,#38518,.T.) ;
#51593=ORIENTED_EDGE('',*,*,#38519,.T.) ;
#51594=ORIENTED_EDGE('',*,*,#38373,.T.) ;
#51595=ORIENTED_EDGE('',*,*,#38520,.T.) ;
#51596=ORIENTED_EDGE('',*,*,#38521,.T.) ;
#51597=ORIENTED_EDGE('',*,*,#38497,.F.) ;
#51598=ORIENTED_EDGE('',*,*,#38522,.T.) ;
#51599=ORIENTED_EDGE('',*,*,#38523,.T.) ;
#51600=ORIENTED_EDGE('',*,*,#38524,.T.) ;
#51601=ORIENTED_EDGE('',*,*,#38525,.T.) ;
#51602=ORIENTED_EDGE('',*,*,#38526,.T.) ;
#51603=ORIENTED_EDGE('',*,*,#38527,.T.) ;
#51604=ORIENTED_EDGE('',*,*,#38495,.F.) ;
#51605=ORIENTED_EDGE('',*,*,#38528,.T.) ;
#51606=ORIENTED_EDGE('',*,*,#38529,.T.) ;
#51607=ORIENTED_EDGE('',*,*,#38530,.F.) ;
#51608=ORIENTED_EDGE('',*,*,#38531,.T.) ;
#51609=ORIENTED_EDGE('',*,*,#38532,.F.) ;
#51610=ORIENTED_EDGE('',*,*,#38533,.T.) ;
#51611=ORIENTED_EDGE('',*,*,#38534,.T.) ;
#51612=ORIENTED_EDGE('',*,*,#38447,.T.) ;
#51613=ORIENTED_EDGE('',*,*,#38535,.F.) ;
#51614=ORIENTED_EDGE('',*,*,#38536,.T.) ;
#51615=ORIENTED_EDGE('',*,*,#38453,.T.) ;
#51616=ORIENTED_EDGE('',*,*,#38537,.T.) ;
#51617=ORIENTED_EDGE('',*,*,#38538,.F.) ;
#51618=ORIENTED_EDGE('',*,*,#38539,.T.) ;
#51619=ORIENTED_EDGE('',*,*,#38540,.F.) ;
#51620=ORIENTED_EDGE('',*,*,#38541,.T.) ;
#51621=ORIENTED_EDGE('',*,*,#38542,.T.) ;
#51622=ORIENTED_EDGE('',*,*,#38543,.T.) ;
#51623=ORIENTED_EDGE('',*,*,#38544,.F.) ;
#51624=ORIENTED_EDGE('',*,*,#38545,.T.) ;
#51625=ORIENTED_EDGE('',*,*,#38546,.F.) ;
#51626=ORIENTED_EDGE('',*,*,#38547,.T.) ;
#51627=ORIENTED_EDGE('',*,*,#38489,.F.) ;
#51628=ORIENTED_EDGE('',*,*,#38548,.T.) ;
#51629=ORIENTED_EDGE('',*,*,#38549,.F.) ;
#51630=ORIENTED_EDGE('',*,*,#38550,.T.) ;
#51631=ORIENTED_EDGE('',*,*,#38551,.F.) ;
#51632=ORIENTED_EDGE('',*,*,#38552,.T.) ;
#51633=ORIENTED_EDGE('',*,*,#38553,.T.) ;
#51634=ORIENTED_EDGE('',*,*,#38554,.T.) ;
#51635=ORIENTED_EDGE('',*,*,#38555,.F.) ;
#51636=ORIENTED_EDGE('',*,*,#38556,.T.) ;
#51637=ORIENTED_EDGE('',*,*,#38384,.T.) ;
#51638=ORIENTED_EDGE('',*,*,#38557,.F.) ;
#51639=ORIENTED_EDGE('',*,*,#38558,.T.) ;
#51640=ORIENTED_EDGE('',*,*,#38559,.F.) ;
#51641=ORIENTED_EDGE('',*,*,#38463,.T.) ;
#51642=ORIENTED_EDGE('',*,*,#38560,.T.) ;
#51643=ORIENTED_EDGE('',*,*,#38479,.F.) ;
#51644=ORIENTED_EDGE('',*,*,#38561,.F.) ;
#51645=ORIENTED_EDGE('',*,*,#38562,.T.) ;
#51646=ORIENTED_EDGE('',*,*,#38563,.F.) ;
#51647=ORIENTED_EDGE('',*,*,#38564,.T.) ;
#51648=ORIENTED_EDGE('',*,*,#38565,.F.) ;
#51649=ORIENTED_EDGE('',*,*,#38566,.T.) ;
#51650=ORIENTED_EDGE('',*,*,#38561,.T.) ;
#51651=ORIENTED_EDGE('',*,*,#38478,.F.) ;
#51652=ORIENTED_EDGE('',*,*,#38567,.T.) ;
#51653=ORIENTED_EDGE('',*,*,#38464,.T.) ;
#51654=ORIENTED_EDGE('',*,*,#38559,.T.) ;
#51655=ORIENTED_EDGE('',*,*,#38568,.T.) ;
#51656=ORIENTED_EDGE('',*,*,#38569,.F.) ;
#51657=ORIENTED_EDGE('',*,*,#38570,.T.) ;
#51658=ORIENTED_EDGE('',*,*,#38571,.T.) ;
#51659=ORIENTED_EDGE('',*,*,#38572,.T.) ;
#51660=ORIENTED_EDGE('',*,*,#38573,.F.) ;
#51661=ORIENTED_EDGE('',*,*,#38574,.F.) ;
#51662=ORIENTED_EDGE('',*,*,#38575,.T.) ;
#51663=ORIENTED_EDGE('',*,*,#38576,.T.) ;
#51664=ORIENTED_EDGE('',*,*,#38577,.T.) ;
#51665=ORIENTED_EDGE('',*,*,#38578,.T.) ;
#51666=ORIENTED_EDGE('',*,*,#38579,.T.) ;
#51667=ORIENTED_EDGE('',*,*,#38580,.T.) ;
#51668=ORIENTED_EDGE('',*,*,#38581,.T.) ;
#51669=ORIENTED_EDGE('',*,*,#38582,.T.) ;
#51670=ORIENTED_EDGE('',*,*,#38583,.T.) ;
#51671=ORIENTED_EDGE('',*,*,#38584,.T.) ;
#51672=ORIENTED_EDGE('',*,*,#38585,.T.) ;
#51673=ORIENTED_EDGE('',*,*,#38586,.T.) ;
#51674=ORIENTED_EDGE('',*,*,#38587,.T.) ;
#51675=ORIENTED_EDGE('',*,*,#38588,.T.) ;
#51676=ORIENTED_EDGE('',*,*,#38589,.T.) ;
#51677=ORIENTED_EDGE('',*,*,#38590,.T.) ;
#51678=ORIENTED_EDGE('',*,*,#38591,.T.) ;
#51679=ORIENTED_EDGE('',*,*,#38592,.T.) ;
#51680=ORIENTED_EDGE('',*,*,#38593,.T.) ;
#51681=ORIENTED_EDGE('',*,*,#38594,.T.) ;
#51682=ORIENTED_EDGE('',*,*,#38595,.T.) ;
#51683=ORIENTED_EDGE('',*,*,#38596,.T.) ;
#51684=ORIENTED_EDGE('',*,*,#38597,.T.) ;
#51685=ORIENTED_EDGE('',*,*,#38598,.T.) ;
#51686=ORIENTED_EDGE('',*,*,#38599,.T.) ;
#51687=ORIENTED_EDGE('',*,*,#38600,.T.) ;
#51688=ORIENTED_EDGE('',*,*,#38601,.T.) ;
#51689=ORIENTED_EDGE('',*,*,#38602,.T.) ;
#51690=ORIENTED_EDGE('',*,*,#38603,.T.) ;
#51691=ORIENTED_EDGE('',*,*,#38604,.T.) ;
#51692=ORIENTED_EDGE('',*,*,#38605,.T.) ;
#51693=ORIENTED_EDGE('',*,*,#38606,.T.) ;
#51694=ORIENTED_EDGE('',*,*,#38607,.T.) ;
#51695=ORIENTED_EDGE('',*,*,#38608,.T.) ;
#51696=ORIENTED_EDGE('',*,*,#38609,.T.) ;
#51697=ORIENTED_EDGE('',*,*,#38610,.T.) ;
#51698=ORIENTED_EDGE('',*,*,#38379,.T.) ;
#51699=ORIENTED_EDGE('',*,*,#38611,.F.) ;
#51700=ORIENTED_EDGE('',*,*,#38612,.T.) ;
#51701=ORIENTED_EDGE('',*,*,#38613,.T.) ;
#51702=ORIENTED_EDGE('',*,*,#38614,.T.) ;
#51703=ORIENTED_EDGE('',*,*,#38615,.T.) ;
#51704=ORIENTED_EDGE('',*,*,#38616,.T.) ;
#51705=ORIENTED_EDGE('',*,*,#38617,.T.) ;
#51706=ORIENTED_EDGE('',*,*,#38618,.T.) ;
#51707=ORIENTED_EDGE('',*,*,#38619,.F.) ;
#51708=ORIENTED_EDGE('',*,*,#38620,.T.) ;
#51709=ORIENTED_EDGE('',*,*,#38457,.T.) ;
#51710=ORIENTED_EDGE('',*,*,#38621,.T.) ;
#51711=ORIENTED_EDGE('',*,*,#38622,.T.) ;
#51712=ORIENTED_EDGE('',*,*,#38623,.T.) ;
#51713=ORIENTED_EDGE('',*,*,#38624,.T.) ;
#51714=ORIENTED_EDGE('',*,*,#38455,.F.) ;
#51715=ORIENTED_EDGE('',*,*,#38625,.T.) ;
#51716=ORIENTED_EDGE('',*,*,#38626,.T.) ;
#51717=ORIENTED_EDGE('',*,*,#38627,.T.) ;
#51718=ORIENTED_EDGE('',*,*,#38628,.T.) ;
#51719=ORIENTED_EDGE('',*,*,#38629,.T.) ;
#51720=ORIENTED_EDGE('',*,*,#38393,.T.) ;
#51721=ORIENTED_EDGE('',*,*,#38630,.T.) ;
#51722=ORIENTED_EDGE('',*,*,#38631,.T.) ;
#51723=ORIENTED_EDGE('',*,*,#38632,.T.) ;
#51724=ORIENTED_EDGE('',*,*,#38633,.T.) ;
#51725=ORIENTED_EDGE('',*,*,#38634,.T.) ;
#51726=ORIENTED_EDGE('',*,*,#38635,.T.) ;
#51727=ORIENTED_EDGE('',*,*,#38636,.T.) ;
#51728=ORIENTED_EDGE('',*,*,#38637,.T.) ;
#51729=ORIENTED_EDGE('',*,*,#38638,.T.) ;
#51730=ORIENTED_EDGE('',*,*,#38386,.T.) ;
#51731=ORIENTED_EDGE('',*,*,#38639,.T.) ;
#51732=ORIENTED_EDGE('',*,*,#38640,.T.) ;
#51733=ORIENTED_EDGE('',*,*,#38641,.T.) ;
#51734=ORIENTED_EDGE('',*,*,#38642,.T.) ;
#51735=ORIENTED_EDGE('',*,*,#38643,.T.) ;
#51736=ORIENTED_EDGE('',*,*,#38487,.T.) ;
#51737=ORIENTED_EDGE('',*,*,#38644,.T.) ;
#51738=ORIENTED_EDGE('',*,*,#38645,.T.) ;
#51739=ORIENTED_EDGE('',*,*,#38646,.T.) ;
#51740=ORIENTED_EDGE('',*,*,#38485,.T.) ;
#51741=ORIENTED_EDGE('',*,*,#38647,.T.) ;
#51742=ORIENTED_EDGE('',*,*,#38648,.F.) ;
#51743=ORIENTED_EDGE('',*,*,#38649,.T.) ;
#51744=ORIENTED_EDGE('',*,*,#38650,.T.) ;
#51745=ORIENTED_EDGE('',*,*,#38651,.T.) ;
#51746=ORIENTED_EDGE('',*,*,#38652,.T.) ;
#51747=ORIENTED_EDGE('',*,*,#38449,.T.) ;
#51748=ORIENTED_EDGE('',*,*,#38653,.T.) ;
#51749=ORIENTED_EDGE('',*,*,#38654,.T.) ;
#51750=ORIENTED_EDGE('',*,*,#38655,.T.) ;
#51751=ORIENTED_EDGE('',*,*,#38656,.T.) ;
#51752=ORIENTED_EDGE('',*,*,#38451,.F.) ;
#51753=ORIENTED_EDGE('',*,*,#38657,.T.) ;
#51754=ORIENTED_EDGE('',*,*,#38658,.T.) ;
#51755=ORIENTED_EDGE('',*,*,#38659,.T.) ;
#51756=ORIENTED_EDGE('',*,*,#38660,.T.) ;
#51757=ORIENTED_EDGE('',*,*,#38661,.T.) ;
#51758=ORIENTED_EDGE('',*,*,#38662,.T.) ;
#51759=ORIENTED_EDGE('',*,*,#38663,.T.) ;
#51760=ORIENTED_EDGE('',*,*,#38664,.T.) ;
#51761=ORIENTED_EDGE('',*,*,#38665,.T.) ;
#51762=ORIENTED_EDGE('',*,*,#38666,.T.) ;
#51763=ORIENTED_EDGE('',*,*,#38667,.T.) ;
#51764=ORIENTED_EDGE('',*,*,#38668,.T.) ;
#51765=ORIENTED_EDGE('',*,*,#38669,.T.) ;
#51766=ORIENTED_EDGE('',*,*,#38491,.T.) ;
#51767=ORIENTED_EDGE('',*,*,#38670,.T.) ;
#51768=ORIENTED_EDGE('',*,*,#38671,.T.) ;
#51769=ORIENTED_EDGE('',*,*,#38672,.T.) ;
#51770=ORIENTED_EDGE('',*,*,#38673,.T.) ;
#51771=ORIENTED_EDGE('',*,*,#38674,.T.) ;
#51772=ORIENTED_EDGE('',*,*,#38675,.T.) ;
#51773=ORIENTED_EDGE('',*,*,#38676,.T.) ;
#51774=ORIENTED_EDGE('',*,*,#38677,.T.) ;
#51775=ORIENTED_EDGE('',*,*,#38678,.T.) ;
#51776=ORIENTED_EDGE('',*,*,#38493,.T.) ;
#51777=ORIENTED_EDGE('',*,*,#38679,.T.) ;
#51778=ORIENTED_EDGE('',*,*,#38680,.T.) ;
#51779=ORIENTED_EDGE('',*,*,#38681,.T.) ;
#51780=ORIENTED_EDGE('',*,*,#38682,.T.) ;
#51781=ORIENTED_EDGE('',*,*,#38683,.T.) ;
#51782=ORIENTED_EDGE('',*,*,#38684,.T.) ;
#51783=ORIENTED_EDGE('',*,*,#38685,.T.) ;
#51784=ORIENTED_EDGE('',*,*,#38686,.T.) ;
#51785=ORIENTED_EDGE('',*,*,#38378,.T.) ;
#51786=ORIENTED_EDGE('',*,*,#38687,.T.) ;
#51787=ORIENTED_EDGE('',*,*,#38688,.T.) ;
#51788=ORIENTED_EDGE('',*,*,#38689,.T.) ;
#51789=ORIENTED_EDGE('',*,*,#38690,.T.) ;
#51790=ORIENTED_EDGE('',*,*,#38691,.T.) ;
#51791=ORIENTED_EDGE('',*,*,#38692,.T.) ;
#51792=ORIENTED_EDGE('',*,*,#38693,.T.) ;
#51793=ORIENTED_EDGE('',*,*,#38694,.T.) ;
#51794=ORIENTED_EDGE('',*,*,#38695,.T.) ;
#51795=ORIENTED_EDGE('',*,*,#38696,.T.) ;
#51796=ORIENTED_EDGE('',*,*,#38697,.T.) ;
#51797=ORIENTED_EDGE('',*,*,#38698,.T.) ;
#51798=ORIENTED_EDGE('',*,*,#38699,.T.) ;
#51799=ORIENTED_EDGE('',*,*,#38700,.T.) ;
#51800=ORIENTED_EDGE('',*,*,#38701,.T.) ;
#51801=ORIENTED_EDGE('',*,*,#38702,.T.) ;
#51802=ORIENTED_EDGE('',*,*,#38703,.T.) ;
#51803=ORIENTED_EDGE('',*,*,#38704,.T.) ;
#51804=ORIENTED_EDGE('',*,*,#38705,.T.) ;
#51805=ORIENTED_EDGE('',*,*,#38706,.T.) ;
#51806=ORIENTED_EDGE('',*,*,#38707,.T.) ;
#51807=ORIENTED_EDGE('',*,*,#38708,.T.) ;
#51808=ORIENTED_EDGE('',*,*,#38709,.T.) ;
#51809=ORIENTED_EDGE('',*,*,#38710,.T.) ;
#51810=ORIENTED_EDGE('',*,*,#38611,.T.) ;
#51811=ORIENTED_EDGE('',*,*,#38711,.T.) ;
#51812=ORIENTED_EDGE('',*,*,#38712,.T.) ;
#51813=ORIENTED_EDGE('',*,*,#38713,.T.) ;
#51814=ORIENTED_EDGE('',*,*,#38615,.F.) ;
#51815=ORIENTED_EDGE('',*,*,#38714,.T.) ;
#51816=ORIENTED_EDGE('',*,*,#38715,.T.) ;
#51817=ORIENTED_EDGE('',*,*,#38716,.T.) ;
#51818=ORIENTED_EDGE('',*,*,#38617,.F.) ;
#51819=ORIENTED_EDGE('',*,*,#38717,.T.) ;
#51820=ORIENTED_EDGE('',*,*,#38718,.T.) ;
#51821=ORIENTED_EDGE('',*,*,#38719,.T.) ;
#51822=ORIENTED_EDGE('',*,*,#38613,.F.) ;
#51823=ORIENTED_EDGE('',*,*,#38720,.T.) ;
#51824=ORIENTED_EDGE('',*,*,#38721,.T.) ;
#51825=ORIENTED_EDGE('',*,*,#38722,.T.) ;
#51826=ORIENTED_EDGE('',*,*,#38723,.T.) ;
#51827=ORIENTED_EDGE('',*,*,#38724,.T.) ;
#51828=ORIENTED_EDGE('',*,*,#38725,.T.) ;
#51829=ORIENTED_EDGE('',*,*,#38726,.T.) ;
#51830=ORIENTED_EDGE('',*,*,#38727,.T.) ;
#51831=ORIENTED_EDGE('',*,*,#38728,.T.) ;
#51832=ORIENTED_EDGE('',*,*,#38729,.T.) ;
#51833=ORIENTED_EDGE('',*,*,#38730,.T.) ;
#51834=ORIENTED_EDGE('',*,*,#38731,.T.) ;
#51835=ORIENTED_EDGE('',*,*,#38732,.F.) ;
#51836=ORIENTED_EDGE('',*,*,#38733,.T.) ;
#51837=ORIENTED_EDGE('',*,*,#38409,.F.) ;
#51838=ORIENTED_EDGE('',*,*,#38734,.T.) ;
#51839=ORIENTED_EDGE('',*,*,#38735,.T.) ;
#51840=ORIENTED_EDGE('',*,*,#38736,.T.) ;
#51841=ORIENTED_EDGE('',*,*,#38737,.T.) ;
#51842=ORIENTED_EDGE('',*,*,#38732,.T.) ;
#51843=ORIENTED_EDGE('',*,*,#38738,.T.) ;
#51844=ORIENTED_EDGE('',*,*,#38739,.T.) ;
#51845=ORIENTED_EDGE('',*,*,#38740,.T.) ;
#51846=ORIENTED_EDGE('',*,*,#38741,.T.) ;
#51847=ORIENTED_EDGE('',*,*,#38742,.T.) ;
#51848=ORIENTED_EDGE('',*,*,#38743,.T.) ;
#51849=ORIENTED_EDGE('',*,*,#38744,.T.) ;
#51850=ORIENTED_EDGE('',*,*,#38745,.T.) ;
#51851=ORIENTED_EDGE('',*,*,#38746,.T.) ;
#51852=ORIENTED_EDGE('',*,*,#38747,.T.) ;
#51853=ORIENTED_EDGE('',*,*,#38748,.T.) ;
#51854=ORIENTED_EDGE('',*,*,#38749,.T.) ;
#51855=ORIENTED_EDGE('',*,*,#38750,.T.) ;
#51856=ORIENTED_EDGE('',*,*,#38751,.T.) ;
#51857=ORIENTED_EDGE('',*,*,#38752,.T.) ;
#51858=ORIENTED_EDGE('',*,*,#38753,.F.) ;
#51859=ORIENTED_EDGE('',*,*,#38602,.F.) ;
#51860=ORIENTED_EDGE('',*,*,#38754,.T.) ;
#51861=ORIENTED_EDGE('',*,*,#38753,.T.) ;
#51862=ORIENTED_EDGE('',*,*,#38755,.T.) ;
#51863=ORIENTED_EDGE('',*,*,#38756,.T.) ;
#51864=ORIENTED_EDGE('',*,*,#38757,.T.) ;
#51865=ORIENTED_EDGE('',*,*,#38758,.T.) ;
#51866=ORIENTED_EDGE('',*,*,#38759,.T.) ;
#51867=ORIENTED_EDGE('',*,*,#38760,.T.) ;
#51868=ORIENTED_EDGE('',*,*,#38761,.T.) ;
#51869=ORIENTED_EDGE('',*,*,#38762,.T.) ;
#51870=ORIENTED_EDGE('',*,*,#38763,.T.) ;
#51871=ORIENTED_EDGE('',*,*,#38764,.T.) ;
#51872=ORIENTED_EDGE('',*,*,#38765,.T.) ;
#51873=ORIENTED_EDGE('',*,*,#38766,.T.) ;
#51874=ORIENTED_EDGE('',*,*,#38767,.T.) ;
#51875=ORIENTED_EDGE('',*,*,#38768,.T.) ;
#51876=ORIENTED_EDGE('',*,*,#38769,.T.) ;
#51877=ORIENTED_EDGE('',*,*,#38770,.T.) ;
#51878=ORIENTED_EDGE('',*,*,#38771,.T.) ;
#51879=ORIENTED_EDGE('',*,*,#38772,.T.) ;
#51880=ORIENTED_EDGE('',*,*,#38773,.T.) ;
#51881=ORIENTED_EDGE('',*,*,#38774,.T.) ;
#51882=ORIENTED_EDGE('',*,*,#38482,.F.) ;
#51883=ORIENTED_EDGE('',*,*,#38775,.T.) ;
#51884=ORIENTED_EDGE('',*,*,#38776,.T.) ;
#51885=ORIENTED_EDGE('',*,*,#38396,.T.) ;
#51886=ORIENTED_EDGE('',*,*,#38777,.T.) ;
#51887=ORIENTED_EDGE('',*,*,#38460,.F.) ;
#51888=ORIENTED_EDGE('',*,*,#38778,.T.) ;
#51889=ORIENTED_EDGE('',*,*,#38779,.T.) ;
#51890=ORIENTED_EDGE('',*,*,#38780,.T.) ;
#51891=ORIENTED_EDGE('',*,*,#38781,.F.) ;
#51892=ORIENTED_EDGE('',*,*,#38679,.F.) ;
#51893=ORIENTED_EDGE('',*,*,#38492,.F.) ;
#51894=ORIENTED_EDGE('',*,*,#38672,.F.) ;
#51895=ORIENTED_EDGE('',*,*,#38782,.F.) ;
#51896=ORIENTED_EDGE('',*,*,#38781,.T.) ;
#51897=ORIENTED_EDGE('',*,*,#38783,.F.) ;
#51898=ORIENTED_EDGE('',*,*,#38490,.F.) ;
#51899=ORIENTED_EDGE('',*,*,#38547,.F.) ;
#51900=ORIENTED_EDGE('',*,*,#38784,.F.) ;
#51901=ORIENTED_EDGE('',*,*,#38670,.F.) ;
#51902=ORIENTED_EDGE('',*,*,#38783,.T.) ;
#51903=ORIENTED_EDGE('',*,*,#38671,.F.) ;
#51904=ORIENTED_EDGE('',*,*,#38785,.F.) ;
#51905=ORIENTED_EDGE('',*,*,#38667,.F.) ;
#51906=ORIENTED_EDGE('',*,*,#38782,.T.) ;
#51907=ORIENTED_EDGE('',*,*,#38666,.F.) ;
#51908=ORIENTED_EDGE('',*,*,#38786,.F.) ;
#51909=ORIENTED_EDGE('',*,*,#38680,.F.) ;
#51910=ORIENTED_EDGE('',*,*,#38784,.T.) ;
#51911=ORIENTED_EDGE('',*,*,#38546,.T.) ;
#51912=ORIENTED_EDGE('',*,*,#38787,.F.) ;
#51913=ORIENTED_EDGE('',*,*,#38785,.T.) ;
#51914=ORIENTED_EDGE('',*,*,#38788,.F.) ;
#51915=ORIENTED_EDGE('',*,*,#38786,.T.) ;
#51916=ORIENTED_EDGE('',*,*,#38789,.F.) ;
#51917=ORIENTED_EDGE('',*,*,#38450,.F.) ;
#51918=ORIENTED_EDGE('',*,*,#38652,.F.) ;
#51919=ORIENTED_EDGE('',*,*,#38790,.F.) ;
#51920=ORIENTED_EDGE('',*,*,#38657,.F.) ;
#51921=ORIENTED_EDGE('',*,*,#38791,.F.) ;
#51922=ORIENTED_EDGE('',*,*,#38655,.F.) ;
#51923=ORIENTED_EDGE('',*,*,#38792,.F.) ;
#51924=ORIENTED_EDGE('',*,*,#38661,.F.) ;
#51925=ORIENTED_EDGE('',*,*,#38452,.F.) ;
#51926=ORIENTED_EDGE('',*,*,#38656,.F.) ;
#51927=ORIENTED_EDGE('',*,*,#38793,.F.) ;
#51928=ORIENTED_EDGE('',*,*,#38537,.F.) ;
#51929=ORIENTED_EDGE('',*,*,#38787,.T.) ;
#51930=ORIENTED_EDGE('',*,*,#38545,.F.) ;
#51931=ORIENTED_EDGE('',*,*,#38794,.F.) ;
#51932=ORIENTED_EDGE('',*,*,#38668,.F.) ;
#51933=ORIENTED_EDGE('',*,*,#38789,.T.) ;
#51934=ORIENTED_EDGE('',*,*,#38669,.F.) ;
#51935=ORIENTED_EDGE('',*,*,#38795,.F.) ;
#51936=ORIENTED_EDGE('',*,*,#38676,.F.) ;
#51937=ORIENTED_EDGE('',*,*,#38788,.T.) ;
#51938=ORIENTED_EDGE('',*,*,#38675,.F.) ;
#51939=ORIENTED_EDGE('',*,*,#38796,.F.) ;
#51940=ORIENTED_EDGE('',*,*,#38677,.F.) ;
#51941=ORIENTED_EDGE('',*,*,#38494,.F.) ;
#51942=ORIENTED_EDGE('',*,*,#38678,.F.) ;
#51943=ORIENTED_EDGE('',*,*,#38797,.F.) ;
#51944=ORIENTED_EDGE('',*,*,#38528,.F.) ;
#51945=ORIENTED_EDGE('',*,*,#38792,.T.) ;
#51946=ORIENTED_EDGE('',*,*,#38790,.T.) ;
#51947=ORIENTED_EDGE('',*,*,#38798,.F.) ;
#51948=ORIENTED_EDGE('',*,*,#38793,.T.) ;
#51949=ORIENTED_EDGE('',*,*,#38791,.T.) ;
#51950=ORIENTED_EDGE('',*,*,#38799,.F.) ;
#51951=ORIENTED_EDGE('',*,*,#38538,.T.) ;
#51952=ORIENTED_EDGE('',*,*,#38794,.T.) ;
#51953=ORIENTED_EDGE('',*,*,#38544,.T.) ;
#51954=ORIENTED_EDGE('',*,*,#38800,.F.) ;
#51955=ORIENTED_EDGE('',*,*,#38795,.T.) ;
#51956=ORIENTED_EDGE('',*,*,#38797,.T.) ;
#51957=ORIENTED_EDGE('',*,*,#38796,.T.) ;
#51958=ORIENTED_EDGE('',*,*,#38801,.F.) ;
#51959=ORIENTED_EDGE('',*,*,#38798,.T.) ;
#51960=ORIENTED_EDGE('',*,*,#38651,.F.) ;
#51961=ORIENTED_EDGE('',*,*,#38802,.F.) ;
#51962=ORIENTED_EDGE('',*,*,#38658,.F.) ;
#51963=ORIENTED_EDGE('',*,*,#38803,.F.) ;
#51964=ORIENTED_EDGE('',*,*,#38659,.F.) ;
#51965=ORIENTED_EDGE('',*,*,#38804,.F.) ;
#51966=ORIENTED_EDGE('',*,*,#38665,.F.) ;
#51967=ORIENTED_EDGE('',*,*,#38799,.T.) ;
#51968=ORIENTED_EDGE('',*,*,#38660,.F.) ;
#51969=ORIENTED_EDGE('',*,*,#38805,.F.) ;
#51970=ORIENTED_EDGE('',*,*,#38539,.F.) ;
#51971=ORIENTED_EDGE('',*,*,#38800,.T.) ;
#51972=ORIENTED_EDGE('',*,*,#38543,.F.) ;
#51973=ORIENTED_EDGE('',*,*,#38806,.F.) ;
#51974=ORIENTED_EDGE('',*,*,#38673,.F.) ;
#51975=ORIENTED_EDGE('',*,*,#38801,.T.) ;
#51976=ORIENTED_EDGE('',*,*,#38674,.F.) ;
#51977=ORIENTED_EDGE('',*,*,#38807,.F.) ;
#51978=ORIENTED_EDGE('',*,*,#38529,.F.) ;
#51979=ORIENTED_EDGE('',*,*,#38804,.T.) ;
#51980=ORIENTED_EDGE('',*,*,#38802,.T.) ;
#51981=ORIENTED_EDGE('',*,*,#38808,.F.) ;
#51982=ORIENTED_EDGE('',*,*,#38805,.T.) ;
#51983=ORIENTED_EDGE('',*,*,#38803,.T.) ;
#51984=ORIENTED_EDGE('',*,*,#38809,.F.) ;
#51985=ORIENTED_EDGE('',*,*,#38540,.T.) ;
#51986=ORIENTED_EDGE('',*,*,#38807,.T.) ;
#51987=ORIENTED_EDGE('',*,*,#38806,.T.) ;
#51988=ORIENTED_EDGE('',*,*,#38810,.F.) ;
#51989=ORIENTED_EDGE('',*,*,#38530,.T.) ;
#51990=ORIENTED_EDGE('',*,*,#38448,.F.) ;
#51991=ORIENTED_EDGE('',*,*,#38534,.F.) ;
#51992=ORIENTED_EDGE('',*,*,#38811,.F.) ;
#51993=ORIENTED_EDGE('',*,*,#38653,.F.) ;
#51994=ORIENTED_EDGE('',*,*,#38808,.T.) ;
#51995=ORIENTED_EDGE('',*,*,#38654,.F.) ;
#51996=ORIENTED_EDGE('',*,*,#38812,.F.) ;
#51997=ORIENTED_EDGE('',*,*,#38662,.F.) ;
#51998=ORIENTED_EDGE('',*,*,#38809,.T.) ;
#51999=ORIENTED_EDGE('',*,*,#38664,.F.) ;
#52000=ORIENTED_EDGE('',*,*,#38813,.F.) ;
#52001=ORIENTED_EDGE('',*,*,#38541,.F.) ;
#52002=ORIENTED_EDGE('',*,*,#38810,.T.) ;
#52003=ORIENTED_EDGE('',*,*,#38542,.F.) ;
#52004=ORIENTED_EDGE('',*,*,#38814,.F.) ;
#52005=ORIENTED_EDGE('',*,*,#38531,.F.) ;
#52006=ORIENTED_EDGE('',*,*,#38812,.T.) ;
#52007=ORIENTED_EDGE('',*,*,#38811,.T.) ;
#52008=ORIENTED_EDGE('',*,*,#38815,.F.) ;
#52009=ORIENTED_EDGE('',*,*,#38814,.T.) ;
#52010=ORIENTED_EDGE('',*,*,#38813,.T.) ;
#52011=ORIENTED_EDGE('',*,*,#38816,.F.) ;
#52012=ORIENTED_EDGE('',*,*,#38532,.T.) ;
#52013=ORIENTED_EDGE('',*,*,#38815,.T.) ;
#52014=ORIENTED_EDGE('',*,*,#38533,.F.) ;
#52015=ORIENTED_EDGE('',*,*,#38816,.T.) ;
#52016=ORIENTED_EDGE('',*,*,#38663,.F.) ;
#52017=ORIENTED_EDGE('',*,*,#38817,.F.) ;
#52018=ORIENTED_EDGE('',*,*,#38818,.F.) ;
#52019=ORIENTED_EDGE('',*,*,#38819,.F.) ;
#52020=ORIENTED_EDGE('',*,*,#38610,.F.) ;
#52021=ORIENTED_EDGE('',*,*,#38820,.T.) ;
#52022=ORIENTED_EDGE('',*,*,#38821,.T.) ;
#52023=ORIENTED_EDGE('',*,*,#38592,.F.) ;
#52024=ORIENTED_EDGE('',*,*,#38818,.T.) ;
#52025=ORIENTED_EDGE('',*,*,#38591,.F.) ;
#52026=ORIENTED_EDGE('',*,*,#38822,.T.) ;
#52027=ORIENTED_EDGE('',*,*,#38823,.T.) ;
#52028=ORIENTED_EDGE('',*,*,#38584,.F.) ;
#52029=ORIENTED_EDGE('',*,*,#38819,.T.) ;
#52030=ORIENTED_EDGE('',*,*,#38817,.T.) ;
#52031=ORIENTED_EDGE('',*,*,#38583,.F.) ;
#52032=ORIENTED_EDGE('',*,*,#38824,.F.) ;
#52033=ORIENTED_EDGE('',*,*,#38603,.F.) ;
#52034=ORIENTED_EDGE('',*,*,#38599,.F.) ;
#52035=ORIENTED_EDGE('',*,*,#38825,.T.) ;
#52036=ORIENTED_EDGE('',*,*,#38826,.T.) ;
#52037=ORIENTED_EDGE('',*,*,#38609,.F.) ;
#52038=ORIENTED_EDGE('',*,*,#38827,.T.) ;
#52039=ORIENTED_EDGE('',*,*,#38828,.T.) ;
#52040=ORIENTED_EDGE('',*,*,#38577,.F.) ;
#52041=ORIENTED_EDGE('',*,*,#38829,.T.) ;
#52042=ORIENTED_EDGE('',*,*,#38830,.T.) ;
#52043=ORIENTED_EDGE('',*,*,#38593,.F.) ;
#52044=ORIENTED_EDGE('',*,*,#38831,.T.) ;
#52045=ORIENTED_EDGE('',*,*,#38832,.T.) ;
#52046=ORIENTED_EDGE('',*,*,#38833,.F.) ;
#52047=ORIENTED_EDGE('',*,*,#38824,.T.) ;
#52048=ORIENTED_EDGE('',*,*,#38834,.F.) ;
#52049=ORIENTED_EDGE('',*,*,#38574,.T.) ;
#52050=ORIENTED_EDGE('',*,*,#38835,.F.) ;
#52051=ORIENTED_EDGE('',*,*,#38836,.F.) ;
#52052=ORIENTED_EDGE('',*,*,#38604,.F.) ;
#52053=ORIENTED_EDGE('',*,*,#38833,.T.) ;
#52054=ORIENTED_EDGE('',*,*,#38836,.T.) ;
#52055=ORIENTED_EDGE('',*,*,#38837,.F.) ;
#52056=ORIENTED_EDGE('',*,*,#38838,.F.) ;
#52057=ORIENTED_EDGE('',*,*,#38588,.F.) ;
#52058=ORIENTED_EDGE('',*,*,#38839,.T.) ;
#52059=ORIENTED_EDGE('',*,*,#38840,.T.) ;
#52060=ORIENTED_EDGE('',*,*,#38608,.F.) ;
#52061=ORIENTED_EDGE('',*,*,#38841,.F.) ;
#52062=ORIENTED_EDGE('',*,*,#38578,.F.) ;
#52063=ORIENTED_EDGE('',*,*,#38842,.T.) ;
#52064=ORIENTED_EDGE('',*,*,#38843,.T.) ;
#52065=ORIENTED_EDGE('',*,*,#38585,.F.) ;
#52066=ORIENTED_EDGE('',*,*,#38844,.F.) ;
#52067=ORIENTED_EDGE('',*,*,#38834,.T.) ;
#52068=ORIENTED_EDGE('',*,*,#38582,.F.) ;
#52069=ORIENTED_EDGE('',*,*,#38845,.F.) ;
#52070=ORIENTED_EDGE('',*,*,#38846,.F.) ;
#52071=ORIENTED_EDGE('',*,*,#38847,.F.) ;
#52072=ORIENTED_EDGE('',*,*,#38558,.F.) ;
#52073=ORIENTED_EDGE('',*,*,#38848,.F.) ;
#52074=ORIENTED_EDGE('',*,*,#38835,.T.) ;
#52075=ORIENTED_EDGE('',*,*,#38576,.F.) ;
#52076=ORIENTED_EDGE('',*,*,#38848,.T.) ;
#52077=ORIENTED_EDGE('',*,*,#38557,.T.) ;
#52078=ORIENTED_EDGE('',*,*,#38849,.F.) ;
#52079=ORIENTED_EDGE('',*,*,#38837,.T.) ;
#52080=ORIENTED_EDGE('',*,*,#38605,.F.) ;
#52081=ORIENTED_EDGE('',*,*,#38838,.T.) ;
#52082=ORIENTED_EDGE('',*,*,#38850,.F.) ;
#52083=ORIENTED_EDGE('',*,*,#38851,.F.) ;
#52084=ORIENTED_EDGE('',*,*,#38844,.T.) ;
#52085=ORIENTED_EDGE('',*,*,#38841,.T.) ;
#52086=ORIENTED_EDGE('',*,*,#38852,.F.) ;
#52087=ORIENTED_EDGE('',*,*,#38853,.F.) ;
#52088=ORIENTED_EDGE('',*,*,#38845,.T.) ;
#52089=ORIENTED_EDGE('',*,*,#38854,.F.) ;
#52090=ORIENTED_EDGE('',*,*,#38575,.F.) ;
#52091=ORIENTED_EDGE('',*,*,#38846,.T.) ;
#52092=ORIENTED_EDGE('',*,*,#38855,.F.) ;
#52093=ORIENTED_EDGE('',*,*,#38568,.F.) ;
#52094=ORIENTED_EDGE('',*,*,#38847,.T.) ;
#52095=ORIENTED_EDGE('',*,*,#38856,.F.) ;
#52096=ORIENTED_EDGE('',*,*,#38850,.T.) ;
#52097=ORIENTED_EDGE('',*,*,#38849,.T.) ;
#52098=ORIENTED_EDGE('',*,*,#38564,.F.) ;
#52099=ORIENTED_EDGE('',*,*,#38851,.T.) ;
#52100=ORIENTED_EDGE('',*,*,#38857,.F.) ;
#52101=ORIENTED_EDGE('',*,*,#38858,.F.) ;
#52102=ORIENTED_EDGE('',*,*,#38852,.T.) ;
#52103=ORIENTED_EDGE('',*,*,#38607,.F.) ;
#52104=ORIENTED_EDGE('',*,*,#38859,.F.) ;
#52105=ORIENTED_EDGE('',*,*,#38579,.F.) ;
#52106=ORIENTED_EDGE('',*,*,#38854,.T.) ;
#52107=ORIENTED_EDGE('',*,*,#38581,.F.) ;
#52108=ORIENTED_EDGE('',*,*,#38860,.F.) ;
#52109=ORIENTED_EDGE('',*,*,#38861,.F.) ;
#52110=ORIENTED_EDGE('',*,*,#38855,.T.) ;
#52111=ORIENTED_EDGE('',*,*,#38853,.T.) ;
#52112=ORIENTED_EDGE('',*,*,#38862,.F.) ;
#52113=ORIENTED_EDGE('',*,*,#38569,.T.) ;
#52114=ORIENTED_EDGE('',*,*,#38856,.T.) ;
#52115=ORIENTED_EDGE('',*,*,#38563,.T.) ;
#52116=ORIENTED_EDGE('',*,*,#38863,.F.) ;
#52117=ORIENTED_EDGE('',*,*,#38857,.T.) ;
#52118=ORIENTED_EDGE('',*,*,#38864,.F.) ;
#52119=ORIENTED_EDGE('',*,*,#38865,.F.) ;
#52120=ORIENTED_EDGE('',*,*,#38606,.F.) ;
#52121=ORIENTED_EDGE('',*,*,#38858,.T.) ;
#52122=ORIENTED_EDGE('',*,*,#38865,.T.) ;
#52123=ORIENTED_EDGE('',*,*,#38573,.T.) ;
#52124=ORIENTED_EDGE('',*,*,#38866,.F.) ;
#52125=ORIENTED_EDGE('',*,*,#38859,.T.) ;
#52126=ORIENTED_EDGE('',*,*,#38867,.F.) ;
#52127=ORIENTED_EDGE('',*,*,#38860,.T.) ;
#52128=ORIENTED_EDGE('',*,*,#38868,.F.) ;
#52129=ORIENTED_EDGE('',*,*,#38862,.T.) ;
#52130=ORIENTED_EDGE('',*,*,#38861,.T.) ;
#52131=ORIENTED_EDGE('',*,*,#38869,.F.) ;
#52132=ORIENTED_EDGE('',*,*,#38570,.F.) ;
#52133=ORIENTED_EDGE('',*,*,#38863,.T.) ;
#52134=ORIENTED_EDGE('',*,*,#38562,.F.) ;
#52135=ORIENTED_EDGE('',*,*,#38870,.F.) ;
#52136=ORIENTED_EDGE('',*,*,#38571,.F.) ;
#52137=ORIENTED_EDGE('',*,*,#38864,.T.) ;
#52138=ORIENTED_EDGE('',*,*,#38580,.F.) ;
#52139=ORIENTED_EDGE('',*,*,#38866,.T.) ;
#52140=ORIENTED_EDGE('',*,*,#38871,.F.) ;
#52141=ORIENTED_EDGE('',*,*,#38868,.T.) ;
#52142=ORIENTED_EDGE('',*,*,#38869,.T.) ;
#52143=ORIENTED_EDGE('',*,*,#38867,.T.) ;
#52144=ORIENTED_EDGE('',*,*,#38872,.F.) ;
#52145=ORIENTED_EDGE('',*,*,#38565,.T.) ;
#52146=ORIENTED_EDGE('',*,*,#38870,.T.) ;
#52147=ORIENTED_EDGE('',*,*,#38566,.F.) ;
#52148=ORIENTED_EDGE('',*,*,#38872,.T.) ;
#52149=ORIENTED_EDGE('',*,*,#38871,.T.) ;
#52150=ORIENTED_EDGE('',*,*,#38572,.F.) ;
#52151=ORIENTED_EDGE('',*,*,#38873,.F.) ;
#52152=ORIENTED_EDGE('',*,*,#38621,.F.) ;
#52153=ORIENTED_EDGE('',*,*,#38456,.F.) ;
#52154=ORIENTED_EDGE('',*,*,#38627,.F.) ;
#52155=ORIENTED_EDGE('',*,*,#38874,.F.) ;
#52156=ORIENTED_EDGE('',*,*,#38873,.T.) ;
#52157=ORIENTED_EDGE('',*,*,#38875,.F.) ;
#52158=ORIENTED_EDGE('',*,*,#38454,.F.) ;
#52159=ORIENTED_EDGE('',*,*,#38536,.F.) ;
#52160=ORIENTED_EDGE('',*,*,#38876,.F.) ;
#52161=ORIENTED_EDGE('',*,*,#38625,.F.) ;
#52162=ORIENTED_EDGE('',*,*,#38875,.T.) ;
#52163=ORIENTED_EDGE('',*,*,#38626,.F.) ;
#52164=ORIENTED_EDGE('',*,*,#38877,.F.) ;
#52165=ORIENTED_EDGE('',*,*,#38632,.F.) ;
#52166=ORIENTED_EDGE('',*,*,#38874,.T.) ;
#52167=ORIENTED_EDGE('',*,*,#38631,.F.) ;
#52168=ORIENTED_EDGE('',*,*,#38878,.F.) ;
#52169=ORIENTED_EDGE('',*,*,#38622,.F.) ;
#52170=ORIENTED_EDGE('',*,*,#38458,.F.) ;
#52171=ORIENTED_EDGE('',*,*,#38620,.F.) ;
#52172=ORIENTED_EDGE('',*,*,#38879,.F.) ;
#52173=ORIENTED_EDGE('',*,*,#38431,.F.) ;
#52174=ORIENTED_EDGE('',*,*,#38399,.F.) ;
#52175=ORIENTED_EDGE('',*,*,#38880,.T.) ;
#52176=ORIENTED_EDGE('',*,*,#38428,.F.) ;
#52177=ORIENTED_EDGE('',*,*,#38881,.F.) ;
#52178=ORIENTED_EDGE('',*,*,#38876,.T.) ;
#52179=ORIENTED_EDGE('',*,*,#38535,.T.) ;
#52180=ORIENTED_EDGE('',*,*,#38882,.F.) ;
#52181=ORIENTED_EDGE('',*,*,#38877,.T.) ;
#52182=ORIENTED_EDGE('',*,*,#38883,.F.) ;
#52183=ORIENTED_EDGE('',*,*,#38878,.T.) ;
#52184=ORIENTED_EDGE('',*,*,#38884,.F.) ;
#52185=ORIENTED_EDGE('',*,*,#38879,.T.) ;
#52186=ORIENTED_EDGE('',*,*,#38619,.T.) ;
#52187=ORIENTED_EDGE('',*,*,#38885,.F.) ;
#52188=ORIENTED_EDGE('',*,*,#38881,.T.) ;
#52189=ORIENTED_EDGE('',*,*,#38882,.T.) ;
#52190=ORIENTED_EDGE('',*,*,#38556,.F.) ;
#52191=ORIENTED_EDGE('',*,*,#38886,.F.) ;
#52192=ORIENTED_EDGE('',*,*,#38633,.F.) ;
#52193=ORIENTED_EDGE('',*,*,#38884,.T.) ;
#52194=ORIENTED_EDGE('',*,*,#38634,.F.) ;
#52195=ORIENTED_EDGE('',*,*,#38887,.F.) ;
#52196=ORIENTED_EDGE('',*,*,#38628,.F.) ;
#52197=ORIENTED_EDGE('',*,*,#38883,.T.) ;
#52198=ORIENTED_EDGE('',*,*,#38630,.F.) ;
#52199=ORIENTED_EDGE('',*,*,#38888,.F.) ;
#52200=ORIENTED_EDGE('',*,*,#38623,.F.) ;
#52201=ORIENTED_EDGE('',*,*,#38885,.T.) ;
#52202=ORIENTED_EDGE('',*,*,#38624,.F.) ;
#52203=ORIENTED_EDGE('',*,*,#38889,.F.) ;
#52204=ORIENTED_EDGE('',*,*,#38400,.F.) ;
#52205=ORIENTED_EDGE('',*,*,#38434,.F.) ;
#52206=ORIENTED_EDGE('',*,*,#38890,.T.) ;
#52207=ORIENTED_EDGE('',*,*,#38405,.F.) ;
#52208=ORIENTED_EDGE('',*,*,#38891,.F.) ;
#52209=ORIENTED_EDGE('',*,*,#38484,.F.) ;
#52210=ORIENTED_EDGE('',*,*,#38435,.F.) ;
#52211=ORIENTED_EDGE('',*,*,#38892,.F.) ;
#52212=ORIENTED_EDGE('',*,*,#38647,.F.) ;
#52213=ORIENTED_EDGE('',*,*,#38486,.F.) ;
#52214=ORIENTED_EDGE('',*,*,#38646,.F.) ;
#52215=ORIENTED_EDGE('',*,*,#38893,.F.) ;
#52216=ORIENTED_EDGE('',*,*,#38644,.F.) ;
#52217=ORIENTED_EDGE('',*,*,#38886,.T.) ;
#52218=ORIENTED_EDGE('',*,*,#38555,.T.) ;
#52219=ORIENTED_EDGE('',*,*,#38894,.F.) ;
#52220=ORIENTED_EDGE('',*,*,#38887,.T.) ;
#52221=ORIENTED_EDGE('',*,*,#38889,.T.) ;
#52222=ORIENTED_EDGE('',*,*,#38888,.T.) ;
#52223=ORIENTED_EDGE('',*,*,#38392,.F.) ;
#52224=ORIENTED_EDGE('',*,*,#38892,.T.) ;
#52225=ORIENTED_EDGE('',*,*,#38891,.T.) ;
#52226=ORIENTED_EDGE('',*,*,#38895,.F.) ;
#52227=ORIENTED_EDGE('',*,*,#38648,.T.) ;
#52228=ORIENTED_EDGE('',*,*,#38896,.F.) ;
#52229=ORIENTED_EDGE('',*,*,#38893,.T.) ;
#52230=ORIENTED_EDGE('',*,*,#38897,.F.) ;
#52231=ORIENTED_EDGE('',*,*,#38894,.T.) ;
#52232=ORIENTED_EDGE('',*,*,#38554,.F.) ;
#52233=ORIENTED_EDGE('',*,*,#38898,.F.) ;
#52234=ORIENTED_EDGE('',*,*,#38629,.F.) ;
#52235=ORIENTED_EDGE('',*,*,#38895,.T.) ;
#52236=ORIENTED_EDGE('',*,*,#38404,.F.) ;
#52237=ORIENTED_EDGE('',*,*,#38899,.F.) ;
#52238=ORIENTED_EDGE('',*,*,#38649,.F.) ;
#52239=ORIENTED_EDGE('',*,*,#38900,.F.) ;
#52240=ORIENTED_EDGE('',*,*,#38650,.F.) ;
#52241=ORIENTED_EDGE('',*,*,#38901,.F.) ;
#52242=ORIENTED_EDGE('',*,*,#38641,.F.) ;
#52243=ORIENTED_EDGE('',*,*,#38897,.T.) ;
#52244=ORIENTED_EDGE('',*,*,#38645,.F.) ;
#52245=ORIENTED_EDGE('',*,*,#38902,.F.) ;
#52246=ORIENTED_EDGE('',*,*,#38635,.F.) ;
#52247=ORIENTED_EDGE('',*,*,#38896,.T.) ;
#52248=ORIENTED_EDGE('',*,*,#38638,.F.) ;
#52249=ORIENTED_EDGE('',*,*,#38903,.F.) ;
#52250=ORIENTED_EDGE('',*,*,#38642,.F.) ;
#52251=ORIENTED_EDGE('',*,*,#38488,.F.) ;
#52252=ORIENTED_EDGE('',*,*,#38643,.F.) ;
#52253=ORIENTED_EDGE('',*,*,#38904,.F.) ;
#52254=ORIENTED_EDGE('',*,*,#38548,.F.) ;
#52255=ORIENTED_EDGE('',*,*,#38390,.T.) ;
#52256=ORIENTED_EDGE('',*,*,#38898,.T.) ;
#52257=ORIENTED_EDGE('',*,*,#38905,.F.) ;
#52258=ORIENTED_EDGE('',*,*,#38401,.T.) ;
#52259=ORIENTED_EDGE('',*,*,#38901,.T.) ;
#52260=ORIENTED_EDGE('',*,*,#38899,.T.) ;
#52261=ORIENTED_EDGE('',*,*,#38388,.F.) ;
#52262=ORIENTED_EDGE('',*,*,#38906,.F.) ;
#52263=ORIENTED_EDGE('',*,*,#38906,.T.) ;
#52264=ORIENTED_EDGE('',*,*,#38387,.F.) ;
#52265=ORIENTED_EDGE('',*,*,#38902,.T.) ;
#52266=ORIENTED_EDGE('',*,*,#38900,.T.) ;
#52267=ORIENTED_EDGE('',*,*,#38907,.F.) ;
#52268=ORIENTED_EDGE('',*,*,#38904,.T.) ;
#52269=ORIENTED_EDGE('',*,*,#38903,.T.) ;
#52270=ORIENTED_EDGE('',*,*,#38908,.F.) ;
#52271=ORIENTED_EDGE('',*,*,#38549,.T.) ;
#52272=ORIENTED_EDGE('',*,*,#38905,.T.) ;
#52273=ORIENTED_EDGE('',*,*,#38553,.F.) ;
#52274=ORIENTED_EDGE('',*,*,#38909,.F.) ;
#52275=ORIENTED_EDGE('',*,*,#38402,.F.) ;
#52276=ORIENTED_EDGE('',*,*,#38907,.T.) ;
#52277=ORIENTED_EDGE('',*,*,#38640,.F.) ;
#52278=ORIENTED_EDGE('',*,*,#38910,.F.) ;
#52279=ORIENTED_EDGE('',*,*,#38636,.F.) ;
#52280=ORIENTED_EDGE('',*,*,#38908,.T.) ;
#52281=ORIENTED_EDGE('',*,*,#38637,.F.) ;
#52282=ORIENTED_EDGE('',*,*,#38911,.F.) ;
#52283=ORIENTED_EDGE('',*,*,#38550,.F.) ;
#52284=ORIENTED_EDGE('',*,*,#38403,.T.) ;
#52285=ORIENTED_EDGE('',*,*,#38909,.T.) ;
#52286=ORIENTED_EDGE('',*,*,#38912,.F.) ;
#52287=ORIENTED_EDGE('',*,*,#38385,.T.) ;
#52288=ORIENTED_EDGE('',*,*,#38911,.T.) ;
#52289=ORIENTED_EDGE('',*,*,#38910,.T.) ;
#52290=ORIENTED_EDGE('',*,*,#38913,.F.) ;
#52291=ORIENTED_EDGE('',*,*,#38551,.T.) ;
#52292=ORIENTED_EDGE('',*,*,#38912,.T.) ;
#52293=ORIENTED_EDGE('',*,*,#38552,.F.) ;
#52294=ORIENTED_EDGE('',*,*,#38913,.T.) ;
#52295=ORIENTED_EDGE('',*,*,#38639,.F.) ;
#52296=ORIENTED_EDGE('',*,*,#38408,.F.) ;
#52297=ORIENTED_EDGE('',*,*,#38914,.T.) ;
#52298=ORIENTED_EDGE('',*,*,#38729,.F.) ;
#52299=ORIENTED_EDGE('',*,*,#38915,.F.) ;
#52300=ORIENTED_EDGE('',*,*,#38734,.F.) ;
#52301=ORIENTED_EDGE('',*,*,#38728,.F.) ;
#52302=ORIENTED_EDGE('',*,*,#38916,.T.) ;
#52303=ORIENTED_EDGE('',*,*,#38735,.F.) ;
#52304=ORIENTED_EDGE('',*,*,#38915,.T.) ;
#52305=ORIENTED_EDGE('',*,*,#38731,.F.) ;
#52306=ORIENTED_EDGE('',*,*,#38917,.T.) ;
#52307=ORIENTED_EDGE('',*,*,#38597,.F.) ;
#52308=ORIENTED_EDGE('',*,*,#38755,.F.) ;
#52309=ORIENTED_EDGE('',*,*,#38918,.F.) ;
#52310=ORIENTED_EDGE('',*,*,#38740,.F.) ;
#52311=ORIENTED_EDGE('',*,*,#38919,.T.) ;
#52312=ORIENTED_EDGE('',*,*,#38768,.F.) ;
#52313=ORIENTED_EDGE('',*,*,#38920,.F.) ;
#52314=ORIENTED_EDGE('',*,*,#38725,.F.) ;
#52315=ORIENTED_EDGE('',*,*,#38921,.T.) ;
#52316=ORIENTED_EDGE('',*,*,#38410,.F.) ;
#52317=ORIENTED_EDGE('',*,*,#38733,.F.) ;
#52318=ORIENTED_EDGE('',*,*,#38922,.F.) ;
#52319=ORIENTED_EDGE('',*,*,#38752,.F.) ;
#52320=ORIENTED_EDGE('',*,*,#38923,.T.) ;
#52321=ORIENTED_EDGE('',*,*,#38726,.F.) ;
#52322=ORIENTED_EDGE('',*,*,#38918,.T.) ;
#52323=ORIENTED_EDGE('',*,*,#38924,.F.) ;
#52324=ORIENTED_EDGE('',*,*,#38920,.T.) ;
#52325=ORIENTED_EDGE('',*,*,#38925,.F.) ;
#52326=ORIENTED_EDGE('',*,*,#38737,.F.) ;
#52327=ORIENTED_EDGE('',*,*,#38926,.T.) ;
#52328=ORIENTED_EDGE('',*,*,#38720,.F.) ;
#52329=ORIENTED_EDGE('',*,*,#38922,.T.) ;
#52330=ORIENTED_EDGE('',*,*,#38770,.F.) ;
#52331=ORIENTED_EDGE('',*,*,#38927,.T.) ;
#52332=ORIENTED_EDGE('',*,*,#38746,.F.) ;
#52333=ORIENTED_EDGE('',*,*,#38928,.F.) ;
#52334=ORIENTED_EDGE('',*,*,#38925,.T.) ;
#52335=ORIENTED_EDGE('',*,*,#38771,.F.) ;
#52336=ORIENTED_EDGE('',*,*,#38929,.F.) ;
#52337=ORIENTED_EDGE('',*,*,#38745,.F.) ;
#52338=ORIENTED_EDGE('',*,*,#38924,.T.) ;
#52339=ORIENTED_EDGE('',*,*,#38744,.F.) ;
#52340=ORIENTED_EDGE('',*,*,#38930,.F.) ;
#52341=ORIENTED_EDGE('',*,*,#38741,.F.) ;
#52342=ORIENTED_EDGE('',*,*,#38766,.F.) ;
#52343=ORIENTED_EDGE('',*,*,#38931,.T.) ;
#52344=ORIENTED_EDGE('',*,*,#38738,.F.) ;
#52345=ORIENTED_EDGE('',*,*,#38932,.F.) ;
#52346=ORIENTED_EDGE('',*,*,#38929,.T.) ;
#52347=ORIENTED_EDGE('',*,*,#38928,.T.) ;
#52348=ORIENTED_EDGE('',*,*,#38933,.F.) ;
#52349=ORIENTED_EDGE('',*,*,#38932,.T.) ;
#52350=ORIENTED_EDGE('',*,*,#38930,.T.) ;
#52351=ORIENTED_EDGE('',*,*,#38934,.F.) ;
#52352=ORIENTED_EDGE('',*,*,#38933,.T.) ;
#52353=ORIENTED_EDGE('',*,*,#38749,.F.) ;
#52354=ORIENTED_EDGE('',*,*,#38935,.F.) ;
#52355=ORIENTED_EDGE('',*,*,#38742,.F.) ;
#52356=ORIENTED_EDGE('',*,*,#38934,.T.) ;
#52357=ORIENTED_EDGE('',*,*,#38743,.F.) ;
#52358=ORIENTED_EDGE('',*,*,#38936,.F.) ;
#52359=ORIENTED_EDGE('',*,*,#38767,.F.) ;
#52360=ORIENTED_EDGE('',*,*,#38936,.T.) ;
#52361=ORIENTED_EDGE('',*,*,#38935,.T.) ;
#52362=ORIENTED_EDGE('',*,*,#38937,.F.) ;
#52363=ORIENTED_EDGE('',*,*,#38748,.F.) ;
#52364=ORIENTED_EDGE('',*,*,#38938,.T.) ;
#52365=ORIENTED_EDGE('',*,*,#38764,.F.) ;
#52366=ORIENTED_EDGE('',*,*,#38937,.T.) ;
#52367=ORIENTED_EDGE('',*,*,#38722,.F.) ;
#52368=ORIENTED_EDGE('',*,*,#38939,.T.) ;
#52369=ORIENTED_EDGE('',*,*,#38750,.F.) ;
#52370=ORIENTED_EDGE('',*,*,#38940,.F.) ;
#52371=ORIENTED_EDGE('',*,*,#38601,.F.) ;
#52372=ORIENTED_EDGE('',*,*,#38941,.T.) ;
#52373=ORIENTED_EDGE('',*,*,#38723,.F.) ;
#52374=ORIENTED_EDGE('',*,*,#38940,.T.) ;
#52375=ORIENTED_EDGE('',*,*,#38754,.F.) ;
#52376=ORIENTED_EDGE('',*,*,#38713,.F.) ;
#52377=ORIENTED_EDGE('',*,*,#38942,.T.) ;
#52378=ORIENTED_EDGE('',*,*,#38714,.F.) ;
#52379=ORIENTED_EDGE('',*,*,#38616,.F.) ;
#52380=ORIENTED_EDGE('',*,*,#38719,.F.) ;
#52381=ORIENTED_EDGE('',*,*,#38943,.T.) ;
#52382=ORIENTED_EDGE('',*,*,#38711,.F.) ;
#52383=ORIENTED_EDGE('',*,*,#38614,.F.) ;
#52384=ORIENTED_EDGE('',*,*,#38698,.F.) ;
#52385=ORIENTED_EDGE('',*,*,#38944,.T.) ;
#52386=ORIENTED_EDGE('',*,*,#38756,.F.) ;
#52387=ORIENTED_EDGE('',*,*,#38945,.F.) ;
#52388=ORIENTED_EDGE('',*,*,#38758,.F.) ;
#52389=ORIENTED_EDGE('',*,*,#38946,.T.) ;
#52390=ORIENTED_EDGE('',*,*,#38704,.F.) ;
#52391=ORIENTED_EDGE('',*,*,#38947,.F.) ;
#52392=ORIENTED_EDGE('',*,*,#38948,.F.) ;
#52393=ORIENTED_EDGE('',*,*,#38759,.F.) ;
#52394=ORIENTED_EDGE('',*,*,#38949,.F.) ;
#52395=ORIENTED_EDGE('',*,*,#38703,.F.) ;
#52396=ORIENTED_EDGE('',*,*,#38945,.T.) ;
#52397=ORIENTED_EDGE('',*,*,#38948,.T.) ;
#52398=ORIENTED_EDGE('',*,*,#38950,.F.) ;
#52399=ORIENTED_EDGE('',*,*,#38716,.F.) ;
#52400=ORIENTED_EDGE('',*,*,#38951,.T.) ;
#52401=ORIENTED_EDGE('',*,*,#38708,.F.) ;
#52402=ORIENTED_EDGE('',*,*,#38618,.F.) ;
#52403=ORIENTED_EDGE('',*,*,#38710,.F.) ;
#52404=ORIENTED_EDGE('',*,*,#38952,.T.) ;
#52405=ORIENTED_EDGE('',*,*,#38717,.F.) ;
#52406=ORIENTED_EDGE('',*,*,#38612,.F.) ;
#52407=ORIENTED_EDGE('',*,*,#38949,.T.) ;
#52408=ORIENTED_EDGE('',*,*,#38947,.T.) ;
#52409=ORIENTED_EDGE('',*,*,#38953,.F.) ;
#52410=ORIENTED_EDGE('',*,*,#38950,.T.) ;
#52411=ORIENTED_EDGE('',*,*,#38702,.F.) ;
#52412=ORIENTED_EDGE('',*,*,#38954,.F.) ;
#52413=ORIENTED_EDGE('',*,*,#38699,.F.) ;
#52414=ORIENTED_EDGE('',*,*,#38762,.F.) ;
#52415=ORIENTED_EDGE('',*,*,#38955,.T.) ;
#52416=ORIENTED_EDGE('',*,*,#38696,.F.) ;
#52417=ORIENTED_EDGE('',*,*,#38956,.F.) ;
#52418=ORIENTED_EDGE('',*,*,#38706,.F.) ;
#52419=ORIENTED_EDGE('',*,*,#38957,.T.) ;
#52420=ORIENTED_EDGE('',*,*,#38760,.F.) ;
#52421=ORIENTED_EDGE('',*,*,#38958,.F.) ;
#52422=ORIENTED_EDGE('',*,*,#38953,.T.) ;
#52423=ORIENTED_EDGE('',*,*,#38707,.F.) ;
#52424=ORIENTED_EDGE('',*,*,#38959,.F.) ;
#52425=ORIENTED_EDGE('',*,*,#38700,.F.) ;
#52426=ORIENTED_EDGE('',*,*,#38956,.T.) ;
#52427=ORIENTED_EDGE('',*,*,#38954,.T.) ;
#52428=ORIENTED_EDGE('',*,*,#38960,.F.) ;
#52429=ORIENTED_EDGE('',*,*,#38959,.T.) ;
#52430=ORIENTED_EDGE('',*,*,#38958,.T.) ;
#52431=ORIENTED_EDGE('',*,*,#38961,.F.) ;
#52432=ORIENTED_EDGE('',*,*,#38960,.T.) ;
#52433=ORIENTED_EDGE('',*,*,#38701,.F.) ;
#52434=ORIENTED_EDGE('',*,*,#38961,.T.) ;
#52435=ORIENTED_EDGE('',*,*,#38763,.F.) ;
#52436=ORIENTED_EDGE('',*,*,#38445,.F.) ;
#52437=ORIENTED_EDGE('',*,*,#38421,.F.) ;
#52438=ORIENTED_EDGE('',*,*,#38962,.F.) ;
#52439=ORIENTED_EDGE('',*,*,#38427,.F.) ;
#52440=ORIENTED_EDGE('',*,*,#38683,.F.) ;
#52441=ORIENTED_EDGE('',*,*,#38963,.T.) ;
#52442=ORIENTED_EDGE('',*,*,#38422,.F.) ;
#52443=ORIENTED_EDGE('',*,*,#38964,.F.) ;
#52444=ORIENTED_EDGE('',*,*,#38964,.T.) ;
#52445=ORIENTED_EDGE('',*,*,#38962,.T.) ;
#52446=ORIENTED_EDGE('',*,*,#38965,.F.) ;
#52447=ORIENTED_EDGE('',*,*,#38444,.F.) ;
#52448=ORIENTED_EDGE('',*,*,#38417,.F.) ;
#52449=ORIENTED_EDGE('',*,*,#38966,.F.) ;
#52450=ORIENTED_EDGE('',*,*,#38419,.F.) ;
#52451=ORIENTED_EDGE('',*,*,#38965,.T.) ;
#52452=ORIENTED_EDGE('',*,*,#38420,.F.) ;
#52453=ORIENTED_EDGE('',*,*,#38967,.F.) ;
#52454=ORIENTED_EDGE('',*,*,#38684,.F.) ;
#52455=ORIENTED_EDGE('',*,*,#38967,.T.) ;
#52456=ORIENTED_EDGE('',*,*,#38966,.T.) ;
#52457=ORIENTED_EDGE('',*,*,#38968,.F.) ;
#52458=ORIENTED_EDGE('',*,*,#38416,.F.) ;
#52459=ORIENTED_EDGE('',*,*,#38969,.T.) ;
#52460=ORIENTED_EDGE('',*,*,#38681,.F.) ;
#52461=ORIENTED_EDGE('',*,*,#38968,.T.) ;
#52462=ORIENTED_EDGE('',*,*,#38520,.F.) ;
#52463=ORIENTED_EDGE('',*,*,#38372,.T.) ;
#52464=ORIENTED_EDGE('',*,*,#38970,.T.) ;
#52465=ORIENTED_EDGE('',*,*,#38692,.F.) ;
#52466=ORIENTED_EDGE('',*,*,#38971,.F.) ;
#52467=ORIENTED_EDGE('',*,*,#38498,.F.) ;
#52468=ORIENTED_EDGE('',*,*,#38521,.F.) ;
#52469=ORIENTED_EDGE('',*,*,#38972,.F.) ;
#52470=ORIENTED_EDGE('',*,*,#38518,.F.) ;
#52471=ORIENTED_EDGE('',*,*,#38972,.T.) ;
#52472=ORIENTED_EDGE('',*,*,#38971,.T.) ;
#52473=ORIENTED_EDGE('',*,*,#38973,.F.) ;
#52474=ORIENTED_EDGE('',*,*,#38973,.T.) ;
#52475=ORIENTED_EDGE('',*,*,#38695,.F.) ;
#52476=ORIENTED_EDGE('',*,*,#38974,.F.) ;
#52477=ORIENTED_EDGE('',*,*,#38516,.F.) ;
#52478=ORIENTED_EDGE('',*,*,#38500,.F.) ;
#52479=ORIENTED_EDGE('',*,*,#38517,.F.) ;
#52480=ORIENTED_EDGE('',*,*,#38975,.F.) ;
#52481=ORIENTED_EDGE('',*,*,#38514,.F.) ;
#52482=ORIENTED_EDGE('',*,*,#38975,.T.) ;
#52483=ORIENTED_EDGE('',*,*,#38974,.T.) ;
#52484=ORIENTED_EDGE('',*,*,#38976,.F.) ;
#52485=ORIENTED_EDGE('',*,*,#38694,.F.) ;
#52486=ORIENTED_EDGE('',*,*,#38376,.T.) ;
#52487=ORIENTED_EDGE('',*,*,#38977,.T.) ;
#52488=ORIENTED_EDGE('',*,*,#38515,.F.) ;
#52489=ORIENTED_EDGE('',*,*,#38976,.T.) ;
#52490=ORIENTED_EDGE('',*,*,#38595,.F.) ;
#52491=ORIENTED_EDGE('',*,*,#38978,.T.) ;
#52492=ORIENTED_EDGE('',*,*,#38406,.F.) ;
#52493=ORIENTED_EDGE('',*,*,#38979,.T.) ;
#52494=ORIENTED_EDGE('',*,*,#38465,.F.) ;
#52495=ORIENTED_EDGE('',*,*,#38567,.F.) ;
#52496=ORIENTED_EDGE('',*,*,#38477,.F.) ;
#52497=ORIENTED_EDGE('',*,*,#38501,.F.) ;
#52498=ORIENTED_EDGE('',*,*,#38467,.F.) ;
#52499=ORIENTED_EDGE('',*,*,#38502,.F.) ;
#52500=ORIENTED_EDGE('',*,*,#38475,.F.) ;
#52501=ORIENTED_EDGE('',*,*,#38503,.F.) ;
#52502=ORIENTED_EDGE('',*,*,#38469,.F.) ;
#52503=ORIENTED_EDGE('',*,*,#38504,.F.) ;
#52504=ORIENTED_EDGE('',*,*,#38473,.F.) ;
#52505=ORIENTED_EDGE('',*,*,#38507,.F.) ;
#52506=ORIENTED_EDGE('',*,*,#38462,.F.) ;
#52507=ORIENTED_EDGE('',*,*,#38437,.F.) ;
#52508=ORIENTED_EDGE('',*,*,#38480,.F.) ;
#52509=ORIENTED_EDGE('',*,*,#38560,.F.) ;
#52510=ORIENTED_EDGE('',*,*,#38780,.F.) ;
#52511=ORIENTED_EDGE('',*,*,#38980,.T.) ;
#52512=ORIENTED_EDGE('',*,*,#38439,.F.) ;
#52513=ORIENTED_EDGE('',*,*,#38461,.F.) ;
#52514=ORIENTED_EDGE('',*,*,#38775,.F.) ;
#52515=ORIENTED_EDGE('',*,*,#38981,.T.) ;
#52516=ORIENTED_EDGE('',*,*,#38440,.F.) ;
#52517=ORIENTED_EDGE('',*,*,#38982,.T.) ;
#52518=ORIENTED_EDGE('',*,*,#38441,.F.) ;
#52519=ORIENTED_EDGE('',*,*,#38983,.T.) ;
#52520=ORIENTED_EDGE('',*,*,#38772,.F.) ;
#52521=ORIENTED_EDGE('',*,*,#38481,.F.) ;
#52522=ORIENTED_EDGE('',*,*,#38820,.F.) ;
#52523=ORIENTED_EDGE('',*,*,#38826,.F.) ;
#52524=ORIENTED_EDGE('',*,*,#38825,.F.) ;
#52525=ORIENTED_EDGE('',*,*,#38984,.F.) ;
#52526=ORIENTED_EDGE('',*,*,#38821,.F.) ;
#52527=ORIENTED_EDGE('',*,*,#38914,.F.) ;
#52528=ORIENTED_EDGE('',*,*,#38407,.F.) ;
#52529=ORIENTED_EDGE('',*,*,#38985,.F.) ;
#52530=ORIENTED_EDGE('',*,*,#38589,.F.) ;
#52531=ORIENTED_EDGE('',*,*,#38984,.T.) ;
#52532=ORIENTED_EDGE('',*,*,#38598,.F.) ;
#52533=ORIENTED_EDGE('',*,*,#38917,.F.) ;
#52534=ORIENTED_EDGE('',*,*,#38730,.F.) ;
#52535=ORIENTED_EDGE('',*,*,#38985,.T.) ;
#52536=ORIENTED_EDGE('',*,*,#38978,.F.) ;
#52537=ORIENTED_EDGE('',*,*,#38986,.F.) ;
#52538=ORIENTED_EDGE('',*,*,#38986,.T.) ;
#52539=ORIENTED_EDGE('',*,*,#38594,.F.) ;
#52540=ORIENTED_EDGE('',*,*,#38987,.F.) ;
#52541=ORIENTED_EDGE('',*,*,#38590,.F.) ;
#52542=ORIENTED_EDGE('',*,*,#38829,.F.) ;
#52543=ORIENTED_EDGE('',*,*,#38823,.F.) ;
#52544=ORIENTED_EDGE('',*,*,#38822,.F.) ;
#52545=ORIENTED_EDGE('',*,*,#38987,.T.) ;
#52546=ORIENTED_EDGE('',*,*,#38830,.F.) ;
#52547=ORIENTED_EDGE('',*,*,#38842,.F.) ;
#52548=ORIENTED_EDGE('',*,*,#38832,.F.) ;
#52549=ORIENTED_EDGE('',*,*,#38831,.F.) ;
#52550=ORIENTED_EDGE('',*,*,#38988,.F.) ;
#52551=ORIENTED_EDGE('',*,*,#38843,.F.) ;
#52552=ORIENTED_EDGE('',*,*,#38988,.T.) ;
#52553=ORIENTED_EDGE('',*,*,#38596,.F.) ;
#52554=ORIENTED_EDGE('',*,*,#38989,.F.) ;
#52555=ORIENTED_EDGE('',*,*,#38586,.F.) ;
#52556=ORIENTED_EDGE('',*,*,#38989,.T.) ;
#52557=ORIENTED_EDGE('',*,*,#38979,.F.) ;
#52558=ORIENTED_EDGE('',*,*,#38990,.F.) ;
#52559=ORIENTED_EDGE('',*,*,#38941,.F.) ;
#52560=ORIENTED_EDGE('',*,*,#38600,.F.) ;
#52561=ORIENTED_EDGE('',*,*,#38991,.F.) ;
#52562=ORIENTED_EDGE('',*,*,#38587,.F.) ;
#52563=ORIENTED_EDGE('',*,*,#38990,.T.) ;
#52564=ORIENTED_EDGE('',*,*,#38411,.F.) ;
#52565=ORIENTED_EDGE('',*,*,#38921,.F.) ;
#52566=ORIENTED_EDGE('',*,*,#38724,.F.) ;
#52567=ORIENTED_EDGE('',*,*,#38991,.T.) ;
#52568=ORIENTED_EDGE('',*,*,#38828,.F.) ;
#52569=ORIENTED_EDGE('',*,*,#38827,.F.) ;
#52570=ORIENTED_EDGE('',*,*,#38840,.F.) ;
#52571=ORIENTED_EDGE('',*,*,#38839,.F.) ;
#52572=ORIENTED_EDGE('',*,*,#38415,.F.) ;
#52573=ORIENTED_EDGE('',*,*,#38992,.T.) ;
#52574=ORIENTED_EDGE('',*,*,#38685,.F.) ;
#52575=ORIENTED_EDGE('',*,*,#38993,.F.) ;
#52576=ORIENTED_EDGE('',*,*,#38969,.F.) ;
#52577=ORIENTED_EDGE('',*,*,#38993,.T.) ;
#52578=ORIENTED_EDGE('',*,*,#38691,.F.) ;
#52579=ORIENTED_EDGE('',*,*,#38994,.F.) ;
#52580=ORIENTED_EDGE('',*,*,#38682,.F.) ;
#52581=ORIENTED_EDGE('',*,*,#38994,.T.) ;
#52582=ORIENTED_EDGE('',*,*,#38690,.F.) ;
#52583=ORIENTED_EDGE('',*,*,#38995,.F.) ;
#52584=ORIENTED_EDGE('',*,*,#38996,.F.) ;
#52585=ORIENTED_EDGE('',*,*,#38997,.F.) ;
#52586=ORIENTED_EDGE('',*,*,#38998,.F.) ;
#52587=ORIENTED_EDGE('',*,*,#38423,.F.) ;
#52588=ORIENTED_EDGE('',*,*,#38963,.F.) ;
#52589=ORIENTED_EDGE('',*,*,#38446,.F.) ;
#52590=ORIENTED_EDGE('',*,*,#38425,.F.) ;
#52591=ORIENTED_EDGE('',*,*,#38999,.F.) ;
#52592=ORIENTED_EDGE('',*,*,#38523,.F.) ;
#52593=ORIENTED_EDGE('',*,*,#38424,.F.) ;
#52594=ORIENTED_EDGE('',*,*,#38998,.T.) ;
#52595=ORIENTED_EDGE('',*,*,#38997,.T.) ;
#52596=ORIENTED_EDGE('',*,*,#38996,.T.) ;
#52597=ORIENTED_EDGE('',*,*,#38995,.T.) ;
#52598=ORIENTED_EDGE('',*,*,#39000,.F.) ;
#52599=ORIENTED_EDGE('',*,*,#38524,.F.) ;
#52600=ORIENTED_EDGE('',*,*,#38999,.T.) ;
#52601=ORIENTED_EDGE('',*,*,#38375,.F.) ;
#52602=ORIENTED_EDGE('',*,*,#39001,.T.) ;
#52603=ORIENTED_EDGE('',*,*,#38511,.F.) ;
#52604=ORIENTED_EDGE('',*,*,#38977,.F.) ;
#52605=ORIENTED_EDGE('',*,*,#39000,.T.) ;
#52606=ORIENTED_EDGE('',*,*,#38689,.F.) ;
#52607=ORIENTED_EDGE('',*,*,#39002,.F.) ;
#52608=ORIENTED_EDGE('',*,*,#38525,.F.) ;
#52609=ORIENTED_EDGE('',*,*,#38496,.F.) ;
#52610=ORIENTED_EDGE('',*,*,#38527,.F.) ;
#52611=ORIENTED_EDGE('',*,*,#39003,.F.) ;
#52612=ORIENTED_EDGE('',*,*,#38522,.F.) ;
#52613=ORIENTED_EDGE('',*,*,#38377,.T.) ;
#52614=ORIENTED_EDGE('',*,*,#38693,.F.) ;
#52615=ORIENTED_EDGE('',*,*,#39004,.F.) ;
#52616=ORIENTED_EDGE('',*,*,#38687,.F.) ;
#52617=ORIENTED_EDGE('',*,*,#38526,.F.) ;
#52618=ORIENTED_EDGE('',*,*,#39002,.T.) ;
#52619=ORIENTED_EDGE('',*,*,#39005,.F.) ;
#52620=ORIENTED_EDGE('',*,*,#39006,.F.) ;
#52621=ORIENTED_EDGE('',*,*,#39007,.F.) ;
#52622=ORIENTED_EDGE('',*,*,#38370,.F.) ;
#52623=ORIENTED_EDGE('',*,*,#38369,.F.) ;
#52624=ORIENTED_EDGE('',*,*,#38519,.F.) ;
#52625=ORIENTED_EDGE('',*,*,#39003,.T.) ;
#52626=ORIENTED_EDGE('',*,*,#38371,.F.) ;
#52627=ORIENTED_EDGE('',*,*,#39007,.T.) ;
#52628=ORIENTED_EDGE('',*,*,#39006,.T.) ;
#52629=ORIENTED_EDGE('',*,*,#39005,.T.) ;
#52630=ORIENTED_EDGE('',*,*,#38688,.F.) ;
#52631=ORIENTED_EDGE('',*,*,#39004,.T.) ;
#52632=ORIENTED_EDGE('',*,*,#38970,.F.) ;
#52633=ORIENTED_EDGE('',*,*,#39008,.F.) ;
#52634=ORIENTED_EDGE('',*,*,#38433,.F.) ;
#52635=ORIENTED_EDGE('',*,*,#38483,.F.) ;
#52636=ORIENTED_EDGE('',*,*,#38774,.F.) ;
#52637=ORIENTED_EDGE('',*,*,#38890,.F.) ;
#52638=ORIENTED_EDGE('',*,*,#39008,.T.) ;
#52639=ORIENTED_EDGE('',*,*,#39009,.F.) ;
#52640=ORIENTED_EDGE('',*,*,#38395,.F.) ;
#52641=ORIENTED_EDGE('',*,*,#39009,.T.) ;
#52642=ORIENTED_EDGE('',*,*,#38773,.F.) ;
#52643=ORIENTED_EDGE('',*,*,#39010,.F.) ;
#52644=ORIENTED_EDGE('',*,*,#38777,.F.) ;
#52645=ORIENTED_EDGE('',*,*,#38983,.F.) ;
#52646=ORIENTED_EDGE('',*,*,#38981,.F.) ;
#52647=ORIENTED_EDGE('',*,*,#39010,.T.) ;
#52648=ORIENTED_EDGE('',*,*,#39011,.T.) ;
#52649=ORIENTED_EDGE('',*,*,#38916,.F.) ;
#52650=ORIENTED_EDGE('',*,*,#39012,.F.) ;
#52651=ORIENTED_EDGE('',*,*,#38919,.F.) ;
#52652=ORIENTED_EDGE('',*,*,#39011,.F.) ;
#52653=ORIENTED_EDGE('',*,*,#38739,.F.) ;
#52654=ORIENTED_EDGE('',*,*,#39013,.F.) ;
#52655=ORIENTED_EDGE('',*,*,#38736,.F.) ;
#52656=ORIENTED_EDGE('',*,*,#39012,.T.) ;
#52657=ORIENTED_EDGE('',*,*,#38727,.F.) ;
#52658=ORIENTED_EDGE('',*,*,#39014,.F.) ;
#52659=ORIENTED_EDGE('',*,*,#38769,.F.) ;
#52660=ORIENTED_EDGE('',*,*,#39013,.T.) ;
#52661=ORIENTED_EDGE('',*,*,#38931,.F.) ;
#52662=ORIENTED_EDGE('',*,*,#39015,.F.) ;
#52663=ORIENTED_EDGE('',*,*,#38926,.F.) ;
#52664=ORIENTED_EDGE('',*,*,#39014,.T.) ;
#52665=ORIENTED_EDGE('',*,*,#38923,.F.) ;
#52666=ORIENTED_EDGE('',*,*,#39016,.F.) ;
#52667=ORIENTED_EDGE('',*,*,#38927,.F.) ;
#52668=ORIENTED_EDGE('',*,*,#39015,.T.) ;
#52669=ORIENTED_EDGE('',*,*,#38765,.F.) ;
#52670=ORIENTED_EDGE('',*,*,#39017,.F.) ;
#52671=ORIENTED_EDGE('',*,*,#38721,.F.) ;
#52672=ORIENTED_EDGE('',*,*,#39016,.T.) ;
#52673=ORIENTED_EDGE('',*,*,#38751,.F.) ;
#52674=ORIENTED_EDGE('',*,*,#39018,.F.) ;
#52675=ORIENTED_EDGE('',*,*,#38747,.F.) ;
#52676=ORIENTED_EDGE('',*,*,#39017,.T.) ;
#52677=ORIENTED_EDGE('',*,*,#38938,.F.) ;
#52678=ORIENTED_EDGE('',*,*,#39018,.T.) ;
#52679=ORIENTED_EDGE('',*,*,#38939,.F.) ;
#52680=ORIENTED_EDGE('',*,*,#39019,.T.) ;
#52681=ORIENTED_EDGE('',*,*,#38942,.F.) ;
#52682=ORIENTED_EDGE('',*,*,#39020,.F.) ;
#52683=ORIENTED_EDGE('',*,*,#38944,.F.) ;
#52684=ORIENTED_EDGE('',*,*,#39019,.F.) ;
#52685=ORIENTED_EDGE('',*,*,#38697,.F.) ;
#52686=ORIENTED_EDGE('',*,*,#39021,.F.) ;
#52687=ORIENTED_EDGE('',*,*,#38715,.F.) ;
#52688=ORIENTED_EDGE('',*,*,#39020,.T.) ;
#52689=ORIENTED_EDGE('',*,*,#38712,.F.) ;
#52690=ORIENTED_EDGE('',*,*,#39022,.F.) ;
#52691=ORIENTED_EDGE('',*,*,#38757,.F.) ;
#52692=ORIENTED_EDGE('',*,*,#39021,.T.) ;
#52693=ORIENTED_EDGE('',*,*,#38955,.F.) ;
#52694=ORIENTED_EDGE('',*,*,#39023,.F.) ;
#52695=ORIENTED_EDGE('',*,*,#38951,.F.) ;
#52696=ORIENTED_EDGE('',*,*,#39022,.T.) ;
#52697=ORIENTED_EDGE('',*,*,#38943,.F.) ;
#52698=ORIENTED_EDGE('',*,*,#39024,.F.) ;
#52699=ORIENTED_EDGE('',*,*,#38946,.F.) ;
#52700=ORIENTED_EDGE('',*,*,#39023,.T.) ;
#52701=ORIENTED_EDGE('',*,*,#38761,.F.) ;
#52702=ORIENTED_EDGE('',*,*,#39025,.F.) ;
#52703=ORIENTED_EDGE('',*,*,#38709,.F.) ;
#52704=ORIENTED_EDGE('',*,*,#39024,.T.) ;
#52705=ORIENTED_EDGE('',*,*,#38718,.F.) ;
#52706=ORIENTED_EDGE('',*,*,#39026,.F.) ;
#52707=ORIENTED_EDGE('',*,*,#38705,.F.) ;
#52708=ORIENTED_EDGE('',*,*,#39025,.T.) ;
#52709=ORIENTED_EDGE('',*,*,#38957,.F.) ;
#52710=ORIENTED_EDGE('',*,*,#39026,.T.) ;
#52711=ORIENTED_EDGE('',*,*,#38952,.F.) ;
#52712=ORIENTED_EDGE('',*,*,#38459,.F.) ;
#52713=ORIENTED_EDGE('',*,*,#38429,.F.) ;
#52714=ORIENTED_EDGE('',*,*,#39027,.F.) ;
#52715=ORIENTED_EDGE('',*,*,#38778,.F.) ;
#52716=ORIENTED_EDGE('',*,*,#39027,.T.) ;
#52717=ORIENTED_EDGE('',*,*,#38880,.F.) ;
#52718=ORIENTED_EDGE('',*,*,#38397,.F.) ;
#52719=ORIENTED_EDGE('',*,*,#39028,.F.) ;
#52720=ORIENTED_EDGE('',*,*,#39028,.T.) ;
#52721=ORIENTED_EDGE('',*,*,#38776,.F.) ;
#52722=ORIENTED_EDGE('',*,*,#39029,.F.) ;
#52723=ORIENTED_EDGE('',*,*,#38779,.F.) ;
#52724=ORIENTED_EDGE('',*,*,#38982,.F.) ;
#52725=ORIENTED_EDGE('',*,*,#38980,.F.) ;
#52726=ORIENTED_EDGE('',*,*,#39029,.T.) ;
#52727=ORIENTED_EDGE('',*,*,#38513,.F.) ;
#52728=ORIENTED_EDGE('',*,*,#39030,.F.) ;
#52729=ORIENTED_EDGE('',*,*,#38508,.F.) ;
#52730=ORIENTED_EDGE('',*,*,#38471,.F.) ;
#52731=ORIENTED_EDGE('',*,*,#38512,.F.) ;
#52732=ORIENTED_EDGE('',*,*,#39001,.F.) ;
#52733=ORIENTED_EDGE('',*,*,#38374,.F.) ;
#52734=ORIENTED_EDGE('',*,*,#39031,.F.) ;
#52735=ORIENTED_EDGE('',*,*,#38509,.F.) ;
#52736=ORIENTED_EDGE('',*,*,#39030,.T.) ;
#52737=ORIENTED_EDGE('',*,*,#39031,.T.) ;
#52738=ORIENTED_EDGE('',*,*,#38686,.F.) ;
#52739=ORIENTED_EDGE('',*,*,#39032,.F.) ;
#52740=ORIENTED_EDGE('',*,*,#38510,.F.) ;
#52741=ORIENTED_EDGE('',*,*,#38992,.F.) ;
#52742=ORIENTED_EDGE('',*,*,#38414,.F.) ;
#52743=ORIENTED_EDGE('',*,*,#39033,.F.) ;
#52744=ORIENTED_EDGE('',*,*,#38505,.F.) ;
#52745=ORIENTED_EDGE('',*,*,#39032,.T.) ;
#52746=ORIENTED_EDGE('',*,*,#38443,.F.) ;
#52747=ORIENTED_EDGE('',*,*,#38506,.F.) ;
#52748=ORIENTED_EDGE('',*,*,#39033,.T.) ;
#52749=ORIENTED_EDGE('',*,*,#38413,.F.) ;
#62932=TOROIDAL_SURFACE('',#68786,1.4,0.1) ;
#62933=TOROIDAL_SURFACE('',#68790,1.6,0.1) ;
#62934=TOROIDAL_SURFACE('',#68801,3.1,0.1) ;
#62935=TOROIDAL_SURFACE('',#68982,1.85,0.1) ;
#62936=TOROIDAL_SURFACE('',#68984,0.2,0.1) ;
#62937=TOROIDAL_SURFACE('',#68996,1.65,0.1) ;
#62938=TOROIDAL_SURFACE('',#69006,0.2,0.1) ;
#62939=TOROIDAL_SURFACE('',#69008,0.2,0.1) ;
#62940=TOROIDAL_SURFACE('',#69012,1.85,0.1) ;
#62941=TOROIDAL_SURFACE('',#69017,1.65,0.1) ;
#62942=TOROIDAL_SURFACE('',#69025,0.2,0.1) ;
#62943=TOROIDAL_SURFACE('',#69027,0.2,0.1) ;
#62944=TOROIDAL_SURFACE('',#69039,0.2,0.1) ;
#62945=TOROIDAL_SURFACE('',#69058,0.2,0.1) ;
#62946=TOROIDAL_SURFACE('',#69077,0.2,0.1) ;
#62947=TOROIDAL_SURFACE('',#69097,0.2,0.1) ;
#62948=TOROIDAL_SURFACE('',#69099,0.2,0.1) ;
#62949=TOROIDAL_SURFACE('',#69103,0.2,0.1) ;
#62950=TOROIDAL_SURFACE('',#69113,0.2,0.1) ;
#62951=TOROIDAL_SURFACE('',#69125,1.85,0.1) ;
#62952=TOROIDAL_SURFACE('',#69132,0.2,0.1) ;
#62953=TOROIDAL_SURFACE('',#69137,0.2,0.1) ;
#62954=TOROIDAL_SURFACE('',#69139,1.65,0.1) ;
#62955=TOROIDAL_SURFACE('',#69145,2.9,0.1) ;
#62956=TOROIDAL_SURFACE('',#69154,0.2,0.1) ;
#62957=TOROIDAL_SURFACE('',#69157,0.2,0.1) ;
#62958=TOROIDAL_SURFACE('',#69163,2.9,0.1) ;
#62959=TOROIDAL_SURFACE('',#69168,1.85,0.1) ;
#62960=TOROIDAL_SURFACE('',#69179,0.2,0.1) ;
#62961=TOROIDAL_SURFACE('',#69181,2.9,0.1) ;
#62962=TOROIDAL_SURFACE('',#69185,1.65,0.1) ;
#62963=TOROIDAL_SURFACE('',#69187,0.2,0.1) ;
#62964=TOROIDAL_SURFACE('',#69190,1.9,0.1) ;
#62965=TOROIDAL_SURFACE('',#69194,1.1,0.1) ;
#62966=TOROIDAL_SURFACE('',#69199,1.9,0.1) ;
#62967=TOROIDAL_SURFACE('',#69233,1.1,0.1) ;
#62968=TOROIDAL_SURFACE('',#69307,3.33471270883832,0.1) ;
#62969=TOROIDAL_SURFACE('',#69396,1.4,0.1) ;
#62970=TOROIDAL_SURFACE('',#69400,1.6,0.1) ;
#62971=TOROIDAL_SURFACE('',#69411,3.1,0.1) ;
#62972=TOROIDAL_SURFACE('',#69592,1.85,0.1) ;
#62973=TOROIDAL_SURFACE('',#69594,0.2,0.1) ;
#62974=TOROIDAL_SURFACE('',#69606,1.65,0.1) ;
#62975=TOROIDAL_SURFACE('',#69616,0.2,0.1) ;
#62976=TOROIDAL_SURFACE('',#69618,0.2,0.1) ;
#62977=TOROIDAL_SURFACE('',#69622,1.85,0.1) ;
#62978=TOROIDAL_SURFACE('',#69627,1.65,0.1) ;
#62979=TOROIDAL_SURFACE('',#69635,0.2,0.1) ;
#62980=TOROIDAL_SURFACE('',#69637,0.2,0.1) ;
#62981=TOROIDAL_SURFACE('',#69649,0.2,0.1) ;
#62982=TOROIDAL_SURFACE('',#69668,0.2,0.1) ;
#62983=TOROIDAL_SURFACE('',#69687,0.2,0.1) ;
#62984=TOROIDAL_SURFACE('',#69707,0.2,0.1) ;
#62985=TOROIDAL_SURFACE('',#69709,0.2,0.1) ;
#62986=TOROIDAL_SURFACE('',#69713,0.2,0.1) ;
#62987=TOROIDAL_SURFACE('',#69723,0.2,0.1) ;
#62988=TOROIDAL_SURFACE('',#69735,1.85,0.1) ;
#62989=TOROIDAL_SURFACE('',#69742,0.2,0.1) ;
#62990=TOROIDAL_SURFACE('',#69747,0.2,0.1) ;
#62991=TOROIDAL_SURFACE('',#69749,1.65,0.1) ;
#62992=TOROIDAL_SURFACE('',#69755,2.9,0.1) ;
#62993=TOROIDAL_SURFACE('',#69764,0.2,0.1) ;
#62994=TOROIDAL_SURFACE('',#69767,0.2,0.1) ;
#62995=TOROIDAL_SURFACE('',#69773,2.9,0.1) ;
#62996=TOROIDAL_SURFACE('',#69778,1.85,0.1) ;
#62997=TOROIDAL_SURFACE('',#69789,0.2,0.1) ;
#62998=TOROIDAL_SURFACE('',#69791,2.9,0.1) ;
#62999=TOROIDAL_SURFACE('',#69795,1.65,0.1) ;
#63000=TOROIDAL_SURFACE('',#69797,0.2,0.1) ;
#63001=TOROIDAL_SURFACE('',#69800,1.9,0.1) ;
#63002=TOROIDAL_SURFACE('',#69804,1.1,0.1) ;
#63003=TOROIDAL_SURFACE('',#69809,1.9,0.1) ;
#63004=TOROIDAL_SURFACE('',#69843,1.1,0.1) ;
#63005=TOROIDAL_SURFACE('',#69917,3.33471270883832,0.1) ;
#63006=TOROIDAL_SURFACE('',#70006,1.4,0.1) ;
#63007=TOROIDAL_SURFACE('',#70010,1.6,0.1) ;
#63008=TOROIDAL_SURFACE('',#70021,3.1,0.1) ;
#63009=TOROIDAL_SURFACE('',#70202,1.85,0.1) ;
#63010=TOROIDAL_SURFACE('',#70204,0.2,0.1) ;
#63011=TOROIDAL_SURFACE('',#70216,1.65,0.1) ;
#63012=TOROIDAL_SURFACE('',#70226,0.2,0.1) ;
#63013=TOROIDAL_SURFACE('',#70228,0.2,0.1) ;
#63014=TOROIDAL_SURFACE('',#70232,1.85,0.1) ;
#63015=TOROIDAL_SURFACE('',#70237,1.65,0.1) ;
#63016=TOROIDAL_SURFACE('',#70245,0.2,0.1) ;
#63017=TOROIDAL_SURFACE('',#70247,0.2,0.1) ;
#63018=TOROIDAL_SURFACE('',#70259,0.2,0.1) ;
#63019=TOROIDAL_SURFACE('',#70278,0.2,0.1) ;
#63020=TOROIDAL_SURFACE('',#70297,0.2,0.1) ;
#63021=TOROIDAL_SURFACE('',#70317,0.2,0.1) ;
#63022=TOROIDAL_SURFACE('',#70319,0.2,0.1) ;
#63023=TOROIDAL_SURFACE('',#70323,0.2,0.1) ;
#63024=TOROIDAL_SURFACE('',#70333,0.2,0.1) ;
#63025=TOROIDAL_SURFACE('',#70345,1.85,0.1) ;
#63026=TOROIDAL_SURFACE('',#70352,0.2,0.1) ;
#63027=TOROIDAL_SURFACE('',#70357,0.2,0.1) ;
#63028=TOROIDAL_SURFACE('',#70359,1.65,0.1) ;
#63029=TOROIDAL_SURFACE('',#70365,2.9,0.1) ;
#63030=TOROIDAL_SURFACE('',#70374,0.2,0.1) ;
#63031=TOROIDAL_SURFACE('',#70377,0.2,0.1) ;
#63032=TOROIDAL_SURFACE('',#70383,2.9,0.1) ;
#63033=TOROIDAL_SURFACE('',#70388,1.85,0.1) ;
#63034=TOROIDAL_SURFACE('',#70399,0.2,0.1) ;
#63035=TOROIDAL_SURFACE('',#70401,2.9,0.1) ;
#63036=TOROIDAL_SURFACE('',#70405,1.65,0.1) ;
#63037=TOROIDAL_SURFACE('',#70407,0.2,0.1) ;
#63038=TOROIDAL_SURFACE('',#70410,1.9,0.1) ;
#63039=TOROIDAL_SURFACE('',#70414,1.1,0.1) ;
#63040=TOROIDAL_SURFACE('',#70419,1.9,0.1) ;
#63041=TOROIDAL_SURFACE('',#70453,1.1,0.1) ;
#63042=TOROIDAL_SURFACE('',#70527,3.33471270883832,0.1) ;
#63043=TOROIDAL_SURFACE('',#70616,1.4,0.1) ;
#63044=TOROIDAL_SURFACE('',#70620,1.6,0.1) ;
#63045=TOROIDAL_SURFACE('',#70631,3.1,0.1) ;
#63046=TOROIDAL_SURFACE('',#70812,1.85,0.1) ;
#63047=TOROIDAL_SURFACE('',#70814,0.2,0.1) ;
#63048=TOROIDAL_SURFACE('',#70826,1.65,0.1) ;
#63049=TOROIDAL_SURFACE('',#70836,0.2,0.1) ;
#63050=TOROIDAL_SURFACE('',#70838,0.2,0.1) ;
#63051=TOROIDAL_SURFACE('',#70842,1.85,0.1) ;
#63052=TOROIDAL_SURFACE('',#70847,1.65,0.1) ;
#63053=TOROIDAL_SURFACE('',#70855,0.2,0.1) ;
#63054=TOROIDAL_SURFACE('',#70857,0.2,0.1) ;
#63055=TOROIDAL_SURFACE('',#70869,0.2,0.1) ;
#63056=TOROIDAL_SURFACE('',#70888,0.2,0.1) ;
#63057=TOROIDAL_SURFACE('',#70907,0.2,0.1) ;
#63058=TOROIDAL_SURFACE('',#70927,0.2,0.1) ;
#63059=TOROIDAL_SURFACE('',#70929,0.2,0.1) ;
#63060=TOROIDAL_SURFACE('',#70933,0.2,0.1) ;
#63061=TOROIDAL_SURFACE('',#70943,0.2,0.1) ;
#63062=TOROIDAL_SURFACE('',#70955,1.85,0.1) ;
#63063=TOROIDAL_SURFACE('',#70962,0.2,0.1) ;
#63064=TOROIDAL_SURFACE('',#70967,0.2,0.1) ;
#63065=TOROIDAL_SURFACE('',#70969,1.65,0.1) ;
#63066=TOROIDAL_SURFACE('',#70975,2.9,0.1) ;
#63067=TOROIDAL_SURFACE('',#70984,0.2,0.1) ;
#63068=TOROIDAL_SURFACE('',#70987,0.2,0.1) ;
#63069=TOROIDAL_SURFACE('',#70993,2.9,0.1) ;
#63070=TOROIDAL_SURFACE('',#70998,1.85,0.1) ;
#63071=TOROIDAL_SURFACE('',#71009,0.2,0.1) ;
#63072=TOROIDAL_SURFACE('',#71011,2.9,0.1) ;
#63073=TOROIDAL_SURFACE('',#71015,1.65,0.1) ;
#63074=TOROIDAL_SURFACE('',#71017,0.2,0.1) ;
#63075=TOROIDAL_SURFACE('',#71020,1.9,0.1) ;
#63076=TOROIDAL_SURFACE('',#71024,1.1,0.1) ;
#63077=TOROIDAL_SURFACE('',#71029,1.9,0.1) ;
#63078=TOROIDAL_SURFACE('',#71063,1.1,0.1) ;
#63079=TOROIDAL_SURFACE('',#71137,3.33471270883832,0.1) ;
#63080=TOROIDAL_SURFACE('',#71226,1.4,0.1) ;
#63081=TOROIDAL_SURFACE('',#71230,1.6,0.1) ;
#63082=TOROIDAL_SURFACE('',#71241,3.1,0.1) ;
#63083=TOROIDAL_SURFACE('',#71422,1.85,0.1) ;
#63084=TOROIDAL_SURFACE('',#71424,0.2,0.1) ;
#63085=TOROIDAL_SURFACE('',#71436,1.65,0.1) ;
#63086=TOROIDAL_SURFACE('',#71446,0.2,0.1) ;
#63087=TOROIDAL_SURFACE('',#71448,0.2,0.1) ;
#63088=TOROIDAL_SURFACE('',#71452,1.85,0.1) ;
#63089=TOROIDAL_SURFACE('',#71457,1.65,0.1) ;
#63090=TOROIDAL_SURFACE('',#71465,0.2,0.1) ;
#63091=TOROIDAL_SURFACE('',#71467,0.2,0.1) ;
#63092=TOROIDAL_SURFACE('',#71479,0.2,0.1) ;
#63093=TOROIDAL_SURFACE('',#71498,0.2,0.1) ;
#63094=TOROIDAL_SURFACE('',#71517,0.2,0.1) ;
#63095=TOROIDAL_SURFACE('',#71537,0.2,0.1) ;
#63096=TOROIDAL_SURFACE('',#71539,0.2,0.1) ;
#63097=TOROIDAL_SURFACE('',#71543,0.2,0.1) ;
#63098=TOROIDAL_SURFACE('',#71553,0.2,0.1) ;
#63099=TOROIDAL_SURFACE('',#71565,1.85,0.1) ;
#63100=TOROIDAL_SURFACE('',#71572,0.2,0.1) ;
#63101=TOROIDAL_SURFACE('',#71577,0.2,0.1) ;
#63102=TOROIDAL_SURFACE('',#71579,1.65,0.1) ;
#63103=TOROIDAL_SURFACE('',#71585,2.9,0.1) ;
#63104=TOROIDAL_SURFACE('',#71594,0.2,0.1) ;
#63105=TOROIDAL_SURFACE('',#71597,0.2,0.1) ;
#63106=TOROIDAL_SURFACE('',#71603,2.9,0.1) ;
#63107=TOROIDAL_SURFACE('',#71608,1.85,0.1) ;
#63108=TOROIDAL_SURFACE('',#71619,0.2,0.1) ;
#63109=TOROIDAL_SURFACE('',#71621,2.9,0.1) ;
#63110=TOROIDAL_SURFACE('',#71625,1.65,0.1) ;
#63111=TOROIDAL_SURFACE('',#71627,0.2,0.1) ;
#63112=TOROIDAL_SURFACE('',#71630,1.9,0.1) ;
#63113=TOROIDAL_SURFACE('',#71634,1.1,0.1) ;
#63114=TOROIDAL_SURFACE('',#71639,1.9,0.1) ;
#63115=TOROIDAL_SURFACE('',#71673,1.1,0.1) ;
#63116=TOROIDAL_SURFACE('',#71747,3.33471270883832,0.1) ;
#63895=ADVANCED_FACE('',(#16610),#377,.F.) ;
#63896=ADVANCED_FACE('',(#16611),#378,.F.) ;
#63897=ADVANCED_FACE('',(#16612),#62932,.T.) ;
#63898=ADVANCED_FACE('',(#16613),#62933,.F.) ;
#63899=ADVANCED_FACE('',(#16614),#6166,.F.) ;
#63900=ADVANCED_FACE('',(#16615),#6167,.F.) ;
#63901=ADVANCED_FACE('',(#16616),#62934,.T.) ;
#63902=ADVANCED_FACE('',(#16617),#6168,.T.) ;
#63903=ADVANCED_FACE('',(#16618),#6169,.F.) ;
#63904=ADVANCED_FACE('',(#16619),#5153,.T.) ;
#63905=ADVANCED_FACE('',(#16620),#5154,.T.) ;
#63906=ADVANCED_FACE('',(#16621),#5155,.T.) ;
#63907=ADVANCED_FACE('',(#16622),#5156,.T.) ;
#63908=ADVANCED_FACE('',(#16623),#5157,.T.) ;
#63909=ADVANCED_FACE('',(#16624),#5158,.T.) ;
#63910=ADVANCED_FACE('',(#16625),#5159,.T.) ;
#63911=ADVANCED_FACE('',(#16626),#5160,.F.) ;
#63912=ADVANCED_FACE('',(#16627),#5161,.T.) ;
#63913=ADVANCED_FACE('',(#16628),#5162,.T.) ;
#63914=ADVANCED_FACE('',(#16629),#5163,.T.) ;
#63915=ADVANCED_FACE('',(#16630),#5164,.T.) ;
#63916=ADVANCED_FACE('',(#16631),#5165,.T.) ;
#63917=ADVANCED_FACE('',(#16632),#5166,.T.) ;
#63918=ADVANCED_FACE('',(#16633),#5167,.T.) ;
#63919=ADVANCED_FACE('',(#16634),#5168,.T.) ;
#63920=ADVANCED_FACE('',(#16635,#5019),#5169,.T.) ;
#63921=ADVANCED_FACE('',(#16636),#5170,.T.) ;
#63922=ADVANCED_FACE('',(#16637),#5171,.T.) ;
#63923=ADVANCED_FACE('',(#16638),#5172,.F.) ;
#63924=ADVANCED_FACE('',(#16639),#5173,.F.) ;
#63925=ADVANCED_FACE('',(#16640),#5174,.T.) ;
#63926=ADVANCED_FACE('',(#16641),#5175,.F.) ;
#63927=ADVANCED_FACE('',(#16642),#5176,.F.) ;
#63928=ADVANCED_FACE('',(#16643),#5177,.F.) ;
#63929=ADVANCED_FACE('',(#16644),#5178,.T.) ;
#63930=ADVANCED_FACE('',(#16645),#5179,.F.) ;
#63931=ADVANCED_FACE('',(#16646,#5020),#5180,.T.) ;
#63932=ADVANCED_FACE('',(#16647),#5181,.T.) ;
#63933=ADVANCED_FACE('',(#16648),#5182,.F.) ;
#63934=ADVANCED_FACE('',(#16649),#5183,.F.) ;
#63935=ADVANCED_FACE('',(#16650),#6170,.T.) ;
#63936=ADVANCED_FACE('',(#16651),#6171,.T.) ;
#63937=ADVANCED_FACE('',(#16652),#5184,.F.) ;
#63938=ADVANCED_FACE('',(#16653),#5185,.F.) ;
#63939=ADVANCED_FACE('',(#16654),#5186,.F.) ;
#63940=ADVANCED_FACE('',(#16655),#5187,.T.) ;
#63941=ADVANCED_FACE('',(#16656),#5188,.F.) ;
#63942=ADVANCED_FACE('',(#16657),#6172,.T.) ;
#63943=ADVANCED_FACE('',(#16658),#5189,.F.) ;
#63944=ADVANCED_FACE('',(#16659),#6173,.T.) ;
#63945=ADVANCED_FACE('',(#16660),#5190,.F.) ;
#63946=ADVANCED_FACE('',(#16661),#5191,.F.) ;
#63947=ADVANCED_FACE('',(#16662),#5192,.F.) ;
#63948=ADVANCED_FACE('',(#16663),#5193,.F.) ;
#63949=ADVANCED_FACE('',(#16664),#5194,.F.) ;
#63950=ADVANCED_FACE('',(#16665),#5195,.F.) ;
#63951=ADVANCED_FACE('',(#16666),#5196,.F.) ;
#63952=ADVANCED_FACE('',(#16667),#5197,.F.) ;
#63953=ADVANCED_FACE('',(#16668),#5198,.F.) ;
#63954=ADVANCED_FACE('',(#16669),#5199,.T.) ;
#63955=ADVANCED_FACE('',(#16670),#5200,.F.) ;
#63956=ADVANCED_FACE('',(#16671),#5201,.F.) ;
#63957=ADVANCED_FACE('',(#16672),#5202,.F.) ;
#63958=ADVANCED_FACE('',(#16673),#5203,.T.) ;
#63959=ADVANCED_FACE('',(#16674),#5204,.F.) ;
#63960=ADVANCED_FACE('',(#16675),#6174,.T.) ;
#63961=ADVANCED_FACE('',(#16676),#5205,.F.) ;
#63962=ADVANCED_FACE('',(#16677),#5206,.F.) ;
#63963=ADVANCED_FACE('',(#16678),#5207,.F.) ;
#63964=ADVANCED_FACE('',(#16679),#5208,.F.) ;
#63965=ADVANCED_FACE('',(#16680),#5209,.F.) ;
#63966=ADVANCED_FACE('',(#16681),#6175,.F.) ;
#63967=ADVANCED_FACE('',(#16682),#5210,.F.) ;
#63968=ADVANCED_FACE('',(#16683),#5211,.F.) ;
#63969=ADVANCED_FACE('',(#16684),#5212,.F.) ;
#63970=ADVANCED_FACE('',(#16685),#5213,.F.) ;
#63971=ADVANCED_FACE('',(#16686),#5214,.F.) ;
#63972=ADVANCED_FACE('',(#16687),#16130,.F.) ;
#63973=ADVANCED_FACE('',(#16688),#5215,.F.) ;
#63974=ADVANCED_FACE('',(#16689),#6176,.F.) ;
#63975=ADVANCED_FACE('',(#16690),#4206,.F.) ;
#63976=ADVANCED_FACE('',(#16691),#6177,.T.) ;
#63977=ADVANCED_FACE('',(#16692),#6178,.F.) ;
#63978=ADVANCED_FACE('',(#16693),#62935,.F.) ;
#63979=ADVANCED_FACE('',(#16694),#62936,.T.) ;
#63980=ADVANCED_FACE('',(#16695),#4207,.F.) ;
#63981=ADVANCED_FACE('',(#16696),#6179,.F.) ;
#63982=ADVANCED_FACE('',(#16697),#6180,.F.) ;
#63983=ADVANCED_FACE('',(#16698),#6181,.T.) ;
#63984=ADVANCED_FACE('',(#16699),#62937,.T.) ;
#63985=ADVANCED_FACE('',(#16700),#6182,.F.) ;
#63986=ADVANCED_FACE('',(#16701),#6183,.F.) ;
#63987=ADVANCED_FACE('',(#16702),#6184,.F.) ;
#63988=ADVANCED_FACE('',(#16703),#4208,.F.) ;
#63989=ADVANCED_FACE('',(#16704),#62938,.T.) ;
#63990=ADVANCED_FACE('',(#16705),#62939,.T.) ;
#63991=ADVANCED_FACE('',(#16706),#4209,.F.) ;
#63992=ADVANCED_FACE('',(#16707),#62940,.F.) ;
#63993=ADVANCED_FACE('',(#16708),#6185,.F.) ;
#63994=ADVANCED_FACE('',(#16709),#62941,.T.) ;
#63995=ADVANCED_FACE('',(#16710),#6186,.T.) ;
#63996=ADVANCED_FACE('',(#16711),#6187,.F.) ;
#63997=ADVANCED_FACE('',(#16712),#4210,.F.) ;
#63998=ADVANCED_FACE('',(#16713),#62942,.T.) ;
#63999=ADVANCED_FACE('',(#16714),#62943,.F.) ;
#64000=ADVANCED_FACE('',(#16715),#6188,.F.) ;
#64001=ADVANCED_FACE('',(#16716),#6189,.F.) ;
#64002=ADVANCED_FACE('',(#16717),#6190,.T.) ;
#64003=ADVANCED_FACE('',(#16718),#6191,.F.) ;
#64004=ADVANCED_FACE('',(#16719),#4211,.F.) ;
#64005=ADVANCED_FACE('',(#16720),#62944,.F.) ;
#64006=ADVANCED_FACE('',(#16721),#6192,.F.) ;
#64007=ADVANCED_FACE('',(#16722),#4212,.T.) ;
#64008=ADVANCED_FACE('',(#16723),#6193,.T.) ;
#64009=ADVANCED_FACE('',(#16724),#6194,.T.) ;
#64010=ADVANCED_FACE('',(#16725),#6195,.T.) ;
#64011=ADVANCED_FACE('',(#16726),#6196,.T.) ;
#64012=ADVANCED_FACE('',(#16727),#6197,.T.) ;
#64013=ADVANCED_FACE('',(#16728),#62945,.F.) ;
#64014=ADVANCED_FACE('',(#16729),#6198,.F.) ;
#64015=ADVANCED_FACE('',(#16730),#4213,.F.) ;
#64016=ADVANCED_FACE('',(#16731),#6199,.T.) ;
#64017=ADVANCED_FACE('',(#16732),#6200,.T.) ;
#64018=ADVANCED_FACE('',(#16733),#6201,.F.) ;
#64019=ADVANCED_FACE('',(#16734),#6202,.T.) ;
#64020=ADVANCED_FACE('',(#16735),#62946,.T.) ;
#64021=ADVANCED_FACE('',(#16736),#6203,.F.) ;
#64022=ADVANCED_FACE('',(#16737),#4214,.T.) ;
#64023=ADVANCED_FACE('',(#16738),#4215,.F.) ;
#64024=ADVANCED_FACE('',(#16739),#6204,.T.) ;
#64025=ADVANCED_FACE('',(#16740),#6205,.T.) ;
#64026=ADVANCED_FACE('',(#16741),#4216,.F.) ;
#64027=ADVANCED_FACE('',(#16742),#6206,.T.) ;
#64028=ADVANCED_FACE('',(#16743),#6207,.F.) ;
#64029=ADVANCED_FACE('',(#16744),#62947,.T.) ;
#64030=ADVANCED_FACE('',(#16745),#62948,.T.) ;
#64031=ADVANCED_FACE('',(#16746),#6208,.F.) ;
#64032=ADVANCED_FACE('',(#16747),#62949,.F.) ;
#64033=ADVANCED_FACE('',(#16748),#4217,.F.) ;
#64034=ADVANCED_FACE('',(#16749),#6209,.T.) ;
#64035=ADVANCED_FACE('',(#16750),#6210,.T.) ;
#64036=ADVANCED_FACE('',(#16751),#6211,.F.) ;
#64037=ADVANCED_FACE('',(#16752),#62950,.T.) ;
#64038=ADVANCED_FACE('',(#16753),#6212,.T.) ;
#64039=ADVANCED_FACE('',(#16754),#6213,.F.) ;
#64040=ADVANCED_FACE('',(#16755),#4218,.F.) ;
#64041=ADVANCED_FACE('',(#16756),#6214,.T.) ;
#64042=ADVANCED_FACE('',(#16757),#6215,.F.) ;
#64043=ADVANCED_FACE('',(#16758),#62951,.F.) ;
#64044=ADVANCED_FACE('',(#16759),#6216,.F.) ;
#64045=ADVANCED_FACE('',(#16760),#6217,.T.) ;
#64046=ADVANCED_FACE('',(#16761),#62952,.T.) ;
#64047=ADVANCED_FACE('',(#16762),#4219,.F.) ;
#64048=ADVANCED_FACE('',(#16763),#62953,.F.) ;
#64049=ADVANCED_FACE('',(#16764),#62954,.T.) ;
#64050=ADVANCED_FACE('',(#16765),#6218,.F.) ;
#64051=ADVANCED_FACE('',(#16766),#6219,.F.) ;
#64052=ADVANCED_FACE('',(#16767),#62955,.F.) ;
#64053=ADVANCED_FACE('',(#16768),#6220,.T.) ;
#64054=ADVANCED_FACE('',(#16769),#6221,.F.) ;
#64055=ADVANCED_FACE('',(#16770),#6222,.F.) ;
#64056=ADVANCED_FACE('',(#16771),#62956,.T.) ;
#64057=ADVANCED_FACE('',(#16772),#4220,.F.) ;
#64058=ADVANCED_FACE('',(#16773),#62957,.F.) ;
#64059=ADVANCED_FACE('',(#16774),#4221,.F.) ;
#64060=ADVANCED_FACE('',(#16775),#6223,.T.) ;
#64061=ADVANCED_FACE('',(#16776),#62958,.F.) ;
#64062=ADVANCED_FACE('',(#16777),#6224,.F.) ;
#64063=ADVANCED_FACE('',(#16778),#62959,.F.) ;
#64064=ADVANCED_FACE('',(#16779),#6225,.F.) ;
#64065=ADVANCED_FACE('',(#16780),#6226,.T.) ;
#64066=ADVANCED_FACE('',(#16781),#379,.F.) ;
#64067=ADVANCED_FACE('',(#16782),#4222,.F.) ;
#64068=ADVANCED_FACE('',(#16783),#4223,.F.) ;
#64069=ADVANCED_FACE('',(#16784),#62960,.T.) ;
#64070=ADVANCED_FACE('',(#16785),#62961,.F.) ;
#64071=ADVANCED_FACE('',(#16786),#6227,.F.) ;
#64072=ADVANCED_FACE('',(#16787),#62962,.T.) ;
#64073=ADVANCED_FACE('',(#16788),#380,.F.) ;
#64074=ADVANCED_FACE('',(#16789),#62963,.T.) ;
#64075=ADVANCED_FACE('',(#16790),#6228,.T.) ;
#64076=ADVANCED_FACE('',(#16791),#62964,.T.) ;
#64077=ADVANCED_FACE('',(#16792),#6229,.T.) ;
#64078=ADVANCED_FACE('',(#16793),#62965,.T.) ;
#64079=ADVANCED_FACE('',(#16794),#6230,.T.) ;
#64080=ADVANCED_FACE('',(#16795),#62966,.T.) ;
#64081=ADVANCED_FACE('',(#16796),#6231,.T.) ;
#64082=ADVANCED_FACE('',(#16797),#4224,.T.) ;
#64083=ADVANCED_FACE('',(#16798),#6232,.T.) ;
#64084=ADVANCED_FACE('',(#16799),#6233,.T.) ;
#64085=ADVANCED_FACE('',(#16800),#6234,.T.) ;
#64086=ADVANCED_FACE('',(#16801),#6235,.T.) ;
#64087=ADVANCED_FACE('',(#16802),#6236,.T.) ;
#64088=ADVANCED_FACE('',(#16803),#4225,.T.) ;
#64089=ADVANCED_FACE('',(#16804),#4226,.T.) ;
#64090=ADVANCED_FACE('',(#16805),#6237,.T.) ;
#64091=ADVANCED_FACE('',(#16806),#6238,.T.) ;
#64092=ADVANCED_FACE('',(#16807),#4227,.T.) ;
#64093=ADVANCED_FACE('',(#16808),#6239,.T.) ;
#64094=ADVANCED_FACE('',(#16809),#6240,.T.) ;
#64095=ADVANCED_FACE('',(#16810),#62967,.T.) ;
#64096=ADVANCED_FACE('',(#16811),#6241,.T.) ;
#64097=ADVANCED_FACE('',(#16812),#6242,.T.) ;
#64098=ADVANCED_FACE('',(#16813),#6243,.T.) ;
#64099=ADVANCED_FACE('',(#16814),#6244,.T.) ;
#64100=ADVANCED_FACE('',(#16815),#6245,.T.) ;
#64101=ADVANCED_FACE('',(#16816),#4228,.T.) ;
#64102=ADVANCED_FACE('',(#16817),#6246,.T.) ;
#64103=ADVANCED_FACE('',(#16818),#6247,.T.) ;
#64104=ADVANCED_FACE('',(#16819),#4229,.T.) ;
#64105=ADVANCED_FACE('',(#16820),#6248,.T.) ;
#64106=ADVANCED_FACE('',(#16821),#6249,.T.) ;
#64107=ADVANCED_FACE('',(#16822),#6250,.T.) ;
#64108=ADVANCED_FACE('',(#16823),#6251,.T.) ;
#64109=ADVANCED_FACE('',(#16824),#4230,.T.) ;
#64110=ADVANCED_FACE('',(#16825),#4231,.T.) ;
#64111=ADVANCED_FACE('',(#16826),#6252,.T.) ;
#64112=ADVANCED_FACE('',(#16827),#6253,.T.) ;
#64113=ADVANCED_FACE('',(#16828),#6254,.T.) ;
#64114=ADVANCED_FACE('',(#16829),#4232,.T.) ;
#64115=ADVANCED_FACE('',(#16830),#6255,.T.) ;
#64116=ADVANCED_FACE('',(#16831),#6256,.T.) ;
#64117=ADVANCED_FACE('',(#16832),#4233,.T.) ;
#64118=ADVANCED_FACE('',(#16833),#6257,.T.) ;
#64119=ADVANCED_FACE('',(#16834),#6258,.T.) ;
#64120=ADVANCED_FACE('',(#16835),#6259,.T.) ;
#64121=ADVANCED_FACE('',(#16836),#4234,.T.) ;
#64122=ADVANCED_FACE('',(#16837),#6260,.T.) ;
#64123=ADVANCED_FACE('',(#16838),#6261,.T.) ;
#64124=ADVANCED_FACE('',(#16839),#4235,.T.) ;
#64125=ADVANCED_FACE('',(#16840),#6262,.T.) ;
#64126=ADVANCED_FACE('',(#16841),#6263,.F.) ;
#64127=ADVANCED_FACE('',(#16842),#6264,.T.) ;
#64128=ADVANCED_FACE('',(#16843),#6265,.F.) ;
#64129=ADVANCED_FACE('',(#16844),#6266,.T.) ;
#64130=ADVANCED_FACE('',(#16845),#6267,.T.) ;
#64131=ADVANCED_FACE('',(#16846),#6268,.T.) ;
#64132=ADVANCED_FACE('',(#16847),#62968,.T.) ;
#64133=ADVANCED_FACE('',(#16848),#6269,.T.) ;
#64134=ADVANCED_FACE('',(#16849),#381,.F.) ;
#64135=ADVANCED_FACE('',(#16850),#6270,.F.) ;
#64136=ADVANCED_FACE('',(#16851),#4236,.F.) ;
#64137=ADVANCED_FACE('',(#16852),#6271,.F.) ;
#64138=ADVANCED_FACE('',(#16853),#382,.F.) ;
#64139=ADVANCED_FACE('',(#16854),#383,.F.) ;
#64140=ADVANCED_FACE('',(#16855),#6272,.F.) ;
#64141=ADVANCED_FACE('',(#16856),#4237,.F.) ;
#64142=ADVANCED_FACE('',(#16857),#6273,.F.) ;
#64143=ADVANCED_FACE('',(#16858),#384,.F.) ;
#64144=ADVANCED_FACE('',(#16859),#385,.F.) ;
#64145=ADVANCED_FACE('',(#16860),#6274,.F.) ;
#64146=ADVANCED_FACE('',(#16861),#386,.F.) ;
#64147=ADVANCED_FACE('',(#16862),#6275,.T.) ;
#64148=ADVANCED_FACE('',(#16863),#387,.T.) ;
#64149=ADVANCED_FACE('',(#16864),#388,.F.) ;
#64150=ADVANCED_FACE('',(#16865),#6276,.T.) ;
#64151=ADVANCED_FACE('',(#16866),#6277,.T.) ;
#64152=ADVANCED_FACE('',(#16867),#6278,.F.) ;
#64153=ADVANCED_FACE('',(#16868),#389,.T.) ;
#64154=ADVANCED_FACE('',(#16869),#390,.F.) ;
#64155=ADVANCED_FACE('',(#16870),#6279,.T.) ;
#64156=ADVANCED_FACE('',(#16871),#4238,.T.) ;
#64157=ADVANCED_FACE('',(#16872),#391,.T.) ;
#64158=ADVANCED_FACE('',(#16873),#4239,.T.) ;
#64159=ADVANCED_FACE('',(#16874),#4240,.T.) ;
#64160=ADVANCED_FACE('',(#16875),#6280,.T.) ;
#64161=ADVANCED_FACE('',(#16876),#6281,.T.) ;
#64162=ADVANCED_FACE('',(#16877),#4241,.T.) ;
#64163=ADVANCED_FACE('',(#16878),#4242,.T.) ;
#64164=ADVANCED_FACE('',(#16879),#6282,.T.) ;
#64165=ADVANCED_FACE('',(#16880),#6283,.T.) ;
#64166=ADVANCED_FACE('',(#16881),#4243,.T.) ;
#64167=ADVANCED_FACE('',(#16882),#4244,.T.) ;
#64168=ADVANCED_FACE('',(#16883),#6284,.T.) ;
#64169=ADVANCED_FACE('',(#16884),#6285,.T.) ;
#64170=ADVANCED_FACE('',(#16885),#4245,.T.) ;
#64171=ADVANCED_FACE('',(#16886),#4246,.T.) ;
#64172=ADVANCED_FACE('',(#16887),#6286,.T.) ;
#64173=ADVANCED_FACE('',(#16888),#6287,.T.) ;
#64174=ADVANCED_FACE('',(#16889),#4247,.T.) ;
#64175=ADVANCED_FACE('',(#16890),#6288,.T.) ;
#64176=ADVANCED_FACE('',(#16891),#4248,.T.) ;
#64177=ADVANCED_FACE('',(#16892),#392,.T.) ;
#64178=ADVANCED_FACE('',(#16893),#4249,.T.) ;
#64179=ADVANCED_FACE('',(#16894),#6289,.T.) ;
#64180=ADVANCED_FACE('',(#16895),#393,.T.) ;
#64181=ADVANCED_FACE('',(#16896),#6290,.T.) ;
#64182=ADVANCED_FACE('',(#16897),#394,.T.) ;
#64183=ADVANCED_FACE('',(#16898),#6291,.T.) ;
#64184=ADVANCED_FACE('',(#16899),#395,.F.) ;
#64185=ADVANCED_FACE('',(#16900),#396,.F.) ;
#64186=ADVANCED_FACE('',(#16901),#62969,.T.) ;
#64187=ADVANCED_FACE('',(#16902),#62970,.F.) ;
#64188=ADVANCED_FACE('',(#16903),#6292,.F.) ;
#64189=ADVANCED_FACE('',(#16904),#6293,.F.) ;
#64190=ADVANCED_FACE('',(#16905),#62971,.T.) ;
#64191=ADVANCED_FACE('',(#16906),#6294,.T.) ;
#64192=ADVANCED_FACE('',(#16907),#6295,.F.) ;
#64193=ADVANCED_FACE('',(#16908),#5216,.T.) ;
#64194=ADVANCED_FACE('',(#16909),#5217,.T.) ;
#64195=ADVANCED_FACE('',(#16910),#5218,.T.) ;
#64196=ADVANCED_FACE('',(#16911),#5219,.T.) ;
#64197=ADVANCED_FACE('',(#16912),#5220,.T.) ;
#64198=ADVANCED_FACE('',(#16913),#5221,.T.) ;
#64199=ADVANCED_FACE('',(#16914),#5222,.T.) ;
#64200=ADVANCED_FACE('',(#16915),#5223,.F.) ;
#64201=ADVANCED_FACE('',(#16916),#5224,.T.) ;
#64202=ADVANCED_FACE('',(#16917),#5225,.T.) ;
#64203=ADVANCED_FACE('',(#16918),#5226,.T.) ;
#64204=ADVANCED_FACE('',(#16919),#5227,.T.) ;
#64205=ADVANCED_FACE('',(#16920),#5228,.T.) ;
#64206=ADVANCED_FACE('',(#16921),#5229,.T.) ;
#64207=ADVANCED_FACE('',(#16922),#5230,.T.) ;
#64208=ADVANCED_FACE('',(#16923),#5231,.T.) ;
#64209=ADVANCED_FACE('',(#16924,#5021),#5232,.T.) ;
#64210=ADVANCED_FACE('',(#16925),#5233,.T.) ;
#64211=ADVANCED_FACE('',(#16926),#5234,.T.) ;
#64212=ADVANCED_FACE('',(#16927),#5235,.F.) ;
#64213=ADVANCED_FACE('',(#16928),#5236,.F.) ;
#64214=ADVANCED_FACE('',(#16929),#5237,.T.) ;
#64215=ADVANCED_FACE('',(#16930),#5238,.F.) ;
#64216=ADVANCED_FACE('',(#16931),#5239,.F.) ;
#64217=ADVANCED_FACE('',(#16932),#5240,.F.) ;
#64218=ADVANCED_FACE('',(#16933),#5241,.T.) ;
#64219=ADVANCED_FACE('',(#16934),#5242,.F.) ;
#64220=ADVANCED_FACE('',(#16935,#5022),#5243,.T.) ;
#64221=ADVANCED_FACE('',(#16936),#5244,.T.) ;
#64222=ADVANCED_FACE('',(#16937),#5245,.F.) ;
#64223=ADVANCED_FACE('',(#16938),#5246,.F.) ;
#64224=ADVANCED_FACE('',(#16939),#6296,.T.) ;
#64225=ADVANCED_FACE('',(#16940),#6297,.T.) ;
#64226=ADVANCED_FACE('',(#16941),#5247,.F.) ;
#64227=ADVANCED_FACE('',(#16942),#5248,.F.) ;
#64228=ADVANCED_FACE('',(#16943),#5249,.F.) ;
#64229=ADVANCED_FACE('',(#16944),#5250,.T.) ;
#64230=ADVANCED_FACE('',(#16945),#5251,.F.) ;
#64231=ADVANCED_FACE('',(#16946),#6298,.T.) ;
#64232=ADVANCED_FACE('',(#16947),#5252,.F.) ;
#64233=ADVANCED_FACE('',(#16948),#6299,.T.) ;
#64234=ADVANCED_FACE('',(#16949),#5253,.F.) ;
#64235=ADVANCED_FACE('',(#16950),#5254,.F.) ;
#64236=ADVANCED_FACE('',(#16951),#5255,.F.) ;
#64237=ADVANCED_FACE('',(#16952),#5256,.F.) ;
#64238=ADVANCED_FACE('',(#16953),#5257,.F.) ;
#64239=ADVANCED_FACE('',(#16954),#5258,.F.) ;
#64240=ADVANCED_FACE('',(#16955),#5259,.F.) ;
#64241=ADVANCED_FACE('',(#16956),#5260,.F.) ;
#64242=ADVANCED_FACE('',(#16957),#5261,.F.) ;
#64243=ADVANCED_FACE('',(#16958),#5262,.T.) ;
#64244=ADVANCED_FACE('',(#16959),#5263,.F.) ;
#64245=ADVANCED_FACE('',(#16960),#5264,.F.) ;
#64246=ADVANCED_FACE('',(#16961),#5265,.F.) ;
#64247=ADVANCED_FACE('',(#16962),#5266,.T.) ;
#64248=ADVANCED_FACE('',(#16963),#5267,.F.) ;
#64249=ADVANCED_FACE('',(#16964),#6300,.T.) ;
#64250=ADVANCED_FACE('',(#16965),#5268,.F.) ;
#64251=ADVANCED_FACE('',(#16966),#5269,.F.) ;
#64252=ADVANCED_FACE('',(#16967),#5270,.F.) ;
#64253=ADVANCED_FACE('',(#16968),#5271,.F.) ;
#64254=ADVANCED_FACE('',(#16969),#5272,.F.) ;
#64255=ADVANCED_FACE('',(#16970),#6301,.F.) ;
#64256=ADVANCED_FACE('',(#16971),#5273,.F.) ;
#64257=ADVANCED_FACE('',(#16972),#5274,.F.) ;
#64258=ADVANCED_FACE('',(#16973),#5275,.F.) ;
#64259=ADVANCED_FACE('',(#16974),#5276,.F.) ;
#64260=ADVANCED_FACE('',(#16975),#5277,.F.) ;
#64261=ADVANCED_FACE('',(#16976),#16131,.F.) ;
#64262=ADVANCED_FACE('',(#16977),#5278,.F.) ;
#64263=ADVANCED_FACE('',(#16978),#6302,.F.) ;
#64264=ADVANCED_FACE('',(#16979),#4250,.F.) ;
#64265=ADVANCED_FACE('',(#16980),#6303,.T.) ;
#64266=ADVANCED_FACE('',(#16981),#6304,.F.) ;
#64267=ADVANCED_FACE('',(#16982),#62972,.F.) ;
#64268=ADVANCED_FACE('',(#16983),#62973,.T.) ;
#64269=ADVANCED_FACE('',(#16984),#4251,.F.) ;
#64270=ADVANCED_FACE('',(#16985),#6305,.F.) ;
#64271=ADVANCED_FACE('',(#16986),#6306,.F.) ;
#64272=ADVANCED_FACE('',(#16987),#6307,.T.) ;
#64273=ADVANCED_FACE('',(#16988),#62974,.T.) ;
#64274=ADVANCED_FACE('',(#16989),#6308,.F.) ;
#64275=ADVANCED_FACE('',(#16990),#6309,.F.) ;
#64276=ADVANCED_FACE('',(#16991),#6310,.F.) ;
#64277=ADVANCED_FACE('',(#16992),#4252,.F.) ;
#64278=ADVANCED_FACE('',(#16993),#62975,.T.) ;
#64279=ADVANCED_FACE('',(#16994),#62976,.T.) ;
#64280=ADVANCED_FACE('',(#16995),#4253,.F.) ;
#64281=ADVANCED_FACE('',(#16996),#62977,.F.) ;
#64282=ADVANCED_FACE('',(#16997),#6311,.F.) ;
#64283=ADVANCED_FACE('',(#16998),#62978,.T.) ;
#64284=ADVANCED_FACE('',(#16999),#6312,.T.) ;
#64285=ADVANCED_FACE('',(#17000),#6313,.F.) ;
#64286=ADVANCED_FACE('',(#17001),#4254,.F.) ;
#64287=ADVANCED_FACE('',(#17002),#62979,.T.) ;
#64288=ADVANCED_FACE('',(#17003),#62980,.F.) ;
#64289=ADVANCED_FACE('',(#17004),#6314,.F.) ;
#64290=ADVANCED_FACE('',(#17005),#6315,.F.) ;
#64291=ADVANCED_FACE('',(#17006),#6316,.T.) ;
#64292=ADVANCED_FACE('',(#17007),#6317,.F.) ;
#64293=ADVANCED_FACE('',(#17008),#4255,.F.) ;
#64294=ADVANCED_FACE('',(#17009),#62981,.F.) ;
#64295=ADVANCED_FACE('',(#17010),#6318,.F.) ;
#64296=ADVANCED_FACE('',(#17011),#4256,.T.) ;
#64297=ADVANCED_FACE('',(#17012),#6319,.T.) ;
#64298=ADVANCED_FACE('',(#17013),#6320,.T.) ;
#64299=ADVANCED_FACE('',(#17014),#6321,.T.) ;
#64300=ADVANCED_FACE('',(#17015),#6322,.T.) ;
#64301=ADVANCED_FACE('',(#17016),#6323,.T.) ;
#64302=ADVANCED_FACE('',(#17017),#62982,.F.) ;
#64303=ADVANCED_FACE('',(#17018),#6324,.F.) ;
#64304=ADVANCED_FACE('',(#17019),#4257,.F.) ;
#64305=ADVANCED_FACE('',(#17020),#6325,.T.) ;
#64306=ADVANCED_FACE('',(#17021),#6326,.T.) ;
#64307=ADVANCED_FACE('',(#17022),#6327,.F.) ;
#64308=ADVANCED_FACE('',(#17023),#6328,.T.) ;
#64309=ADVANCED_FACE('',(#17024),#62983,.T.) ;
#64310=ADVANCED_FACE('',(#17025),#6329,.F.) ;
#64311=ADVANCED_FACE('',(#17026),#4258,.T.) ;
#64312=ADVANCED_FACE('',(#17027),#4259,.F.) ;
#64313=ADVANCED_FACE('',(#17028),#6330,.T.) ;
#64314=ADVANCED_FACE('',(#17029),#6331,.T.) ;
#64315=ADVANCED_FACE('',(#17030),#4260,.F.) ;
#64316=ADVANCED_FACE('',(#17031),#6332,.T.) ;
#64317=ADVANCED_FACE('',(#17032),#6333,.F.) ;
#64318=ADVANCED_FACE('',(#17033),#62984,.T.) ;
#64319=ADVANCED_FACE('',(#17034),#62985,.T.) ;
#64320=ADVANCED_FACE('',(#17035),#6334,.F.) ;
#64321=ADVANCED_FACE('',(#17036),#62986,.F.) ;
#64322=ADVANCED_FACE('',(#17037),#4261,.F.) ;
#64323=ADVANCED_FACE('',(#17038),#6335,.T.) ;
#64324=ADVANCED_FACE('',(#17039),#6336,.T.) ;
#64325=ADVANCED_FACE('',(#17040),#6337,.F.) ;
#64326=ADVANCED_FACE('',(#17041),#62987,.T.) ;
#64327=ADVANCED_FACE('',(#17042),#6338,.T.) ;
#64328=ADVANCED_FACE('',(#17043),#6339,.F.) ;
#64329=ADVANCED_FACE('',(#17044),#4262,.F.) ;
#64330=ADVANCED_FACE('',(#17045),#6340,.T.) ;
#64331=ADVANCED_FACE('',(#17046),#6341,.F.) ;
#64332=ADVANCED_FACE('',(#17047),#62988,.F.) ;
#64333=ADVANCED_FACE('',(#17048),#6342,.F.) ;
#64334=ADVANCED_FACE('',(#17049),#6343,.T.) ;
#64335=ADVANCED_FACE('',(#17050),#62989,.T.) ;
#64336=ADVANCED_FACE('',(#17051),#4263,.F.) ;
#64337=ADVANCED_FACE('',(#17052),#62990,.F.) ;
#64338=ADVANCED_FACE('',(#17053),#62991,.T.) ;
#64339=ADVANCED_FACE('',(#17054),#6344,.F.) ;
#64340=ADVANCED_FACE('',(#17055),#6345,.F.) ;
#64341=ADVANCED_FACE('',(#17056),#62992,.F.) ;
#64342=ADVANCED_FACE('',(#17057),#6346,.T.) ;
#64343=ADVANCED_FACE('',(#17058),#6347,.F.) ;
#64344=ADVANCED_FACE('',(#17059),#6348,.F.) ;
#64345=ADVANCED_FACE('',(#17060),#62993,.T.) ;
#64346=ADVANCED_FACE('',(#17061),#4264,.F.) ;
#64347=ADVANCED_FACE('',(#17062),#62994,.F.) ;
#64348=ADVANCED_FACE('',(#17063),#4265,.F.) ;
#64349=ADVANCED_FACE('',(#17064),#6349,.T.) ;
#64350=ADVANCED_FACE('',(#17065),#62995,.F.) ;
#64351=ADVANCED_FACE('',(#17066),#6350,.F.) ;
#64352=ADVANCED_FACE('',(#17067),#62996,.F.) ;
#64353=ADVANCED_FACE('',(#17068),#6351,.F.) ;
#64354=ADVANCED_FACE('',(#17069),#6352,.T.) ;
#64355=ADVANCED_FACE('',(#17070),#397,.F.) ;
#64356=ADVANCED_FACE('',(#17071),#4266,.F.) ;
#64357=ADVANCED_FACE('',(#17072),#4267,.F.) ;
#64358=ADVANCED_FACE('',(#17073),#62997,.T.) ;
#64359=ADVANCED_FACE('',(#17074),#62998,.F.) ;
#64360=ADVANCED_FACE('',(#17075),#6353,.F.) ;
#64361=ADVANCED_FACE('',(#17076),#62999,.T.) ;
#64362=ADVANCED_FACE('',(#17077),#398,.F.) ;
#64363=ADVANCED_FACE('',(#17078),#63000,.T.) ;
#64364=ADVANCED_FACE('',(#17079),#6354,.T.) ;
#64365=ADVANCED_FACE('',(#17080),#63001,.T.) ;
#64366=ADVANCED_FACE('',(#17081),#6355,.T.) ;
#64367=ADVANCED_FACE('',(#17082),#63002,.T.) ;
#64368=ADVANCED_FACE('',(#17083),#6356,.T.) ;
#64369=ADVANCED_FACE('',(#17084),#63003,.T.) ;
#64370=ADVANCED_FACE('',(#17085),#6357,.T.) ;
#64371=ADVANCED_FACE('',(#17086),#4268,.T.) ;
#64372=ADVANCED_FACE('',(#17087),#6358,.T.) ;
#64373=ADVANCED_FACE('',(#17088),#6359,.T.) ;
#64374=ADVANCED_FACE('',(#17089),#6360,.T.) ;
#64375=ADVANCED_FACE('',(#17090),#6361,.T.) ;
#64376=ADVANCED_FACE('',(#17091),#6362,.T.) ;
#64377=ADVANCED_FACE('',(#17092),#4269,.T.) ;
#64378=ADVANCED_FACE('',(#17093),#4270,.T.) ;
#64379=ADVANCED_FACE('',(#17094),#6363,.T.) ;
#64380=ADVANCED_FACE('',(#17095),#6364,.T.) ;
#64381=ADVANCED_FACE('',(#17096),#4271,.T.) ;
#64382=ADVANCED_FACE('',(#17097),#6365,.T.) ;
#64383=ADVANCED_FACE('',(#17098),#6366,.T.) ;
#64384=ADVANCED_FACE('',(#17099),#63004,.T.) ;
#64385=ADVANCED_FACE('',(#17100),#6367,.T.) ;
#64386=ADVANCED_FACE('',(#17101),#6368,.T.) ;
#64387=ADVANCED_FACE('',(#17102),#6369,.T.) ;
#64388=ADVANCED_FACE('',(#17103),#6370,.T.) ;
#64389=ADVANCED_FACE('',(#17104),#6371,.T.) ;
#64390=ADVANCED_FACE('',(#17105),#4272,.T.) ;
#64391=ADVANCED_FACE('',(#17106),#6372,.T.) ;
#64392=ADVANCED_FACE('',(#17107),#6373,.T.) ;
#64393=ADVANCED_FACE('',(#17108),#4273,.T.) ;
#64394=ADVANCED_FACE('',(#17109),#6374,.T.) ;
#64395=ADVANCED_FACE('',(#17110),#6375,.T.) ;
#64396=ADVANCED_FACE('',(#17111),#6376,.T.) ;
#64397=ADVANCED_FACE('',(#17112),#6377,.T.) ;
#64398=ADVANCED_FACE('',(#17113),#4274,.T.) ;
#64399=ADVANCED_FACE('',(#17114),#4275,.T.) ;
#64400=ADVANCED_FACE('',(#17115),#6378,.T.) ;
#64401=ADVANCED_FACE('',(#17116),#6379,.T.) ;
#64402=ADVANCED_FACE('',(#17117),#6380,.T.) ;
#64403=ADVANCED_FACE('',(#17118),#4276,.T.) ;
#64404=ADVANCED_FACE('',(#17119),#6381,.T.) ;
#64405=ADVANCED_FACE('',(#17120),#6382,.T.) ;
#64406=ADVANCED_FACE('',(#17121),#4277,.T.) ;
#64407=ADVANCED_FACE('',(#17122),#6383,.T.) ;
#64408=ADVANCED_FACE('',(#17123),#6384,.T.) ;
#64409=ADVANCED_FACE('',(#17124),#6385,.T.) ;
#64410=ADVANCED_FACE('',(#17125),#4278,.T.) ;
#64411=ADVANCED_FACE('',(#17126),#6386,.T.) ;
#64412=ADVANCED_FACE('',(#17127),#6387,.T.) ;
#64413=ADVANCED_FACE('',(#17128),#4279,.T.) ;
#64414=ADVANCED_FACE('',(#17129),#6388,.T.) ;
#64415=ADVANCED_FACE('',(#17130),#6389,.F.) ;
#64416=ADVANCED_FACE('',(#17131),#6390,.T.) ;
#64417=ADVANCED_FACE('',(#17132),#6391,.F.) ;
#64418=ADVANCED_FACE('',(#17133),#6392,.T.) ;
#64419=ADVANCED_FACE('',(#17134),#6393,.T.) ;
#64420=ADVANCED_FACE('',(#17135),#6394,.T.) ;
#64421=ADVANCED_FACE('',(#17136),#63005,.T.) ;
#64422=ADVANCED_FACE('',(#17137),#6395,.T.) ;
#64423=ADVANCED_FACE('',(#17138),#399,.F.) ;
#64424=ADVANCED_FACE('',(#17139),#6396,.F.) ;
#64425=ADVANCED_FACE('',(#17140),#4280,.F.) ;
#64426=ADVANCED_FACE('',(#17141),#6397,.F.) ;
#64427=ADVANCED_FACE('',(#17142),#400,.F.) ;
#64428=ADVANCED_FACE('',(#17143),#401,.F.) ;
#64429=ADVANCED_FACE('',(#17144),#6398,.F.) ;
#64430=ADVANCED_FACE('',(#17145),#4281,.F.) ;
#64431=ADVANCED_FACE('',(#17146),#6399,.F.) ;
#64432=ADVANCED_FACE('',(#17147),#402,.F.) ;
#64433=ADVANCED_FACE('',(#17148),#403,.F.) ;
#64434=ADVANCED_FACE('',(#17149),#6400,.F.) ;
#64435=ADVANCED_FACE('',(#17150),#404,.F.) ;
#64436=ADVANCED_FACE('',(#17151),#6401,.T.) ;
#64437=ADVANCED_FACE('',(#17152),#405,.T.) ;
#64438=ADVANCED_FACE('',(#17153),#406,.F.) ;
#64439=ADVANCED_FACE('',(#17154),#6402,.T.) ;
#64440=ADVANCED_FACE('',(#17155),#6403,.T.) ;
#64441=ADVANCED_FACE('',(#17156),#6404,.F.) ;
#64442=ADVANCED_FACE('',(#17157),#407,.T.) ;
#64443=ADVANCED_FACE('',(#17158),#408,.F.) ;
#64444=ADVANCED_FACE('',(#17159),#6405,.T.) ;
#64445=ADVANCED_FACE('',(#17160),#4282,.T.) ;
#64446=ADVANCED_FACE('',(#17161),#409,.T.) ;
#64447=ADVANCED_FACE('',(#17162),#4283,.T.) ;
#64448=ADVANCED_FACE('',(#17163),#4284,.T.) ;
#64449=ADVANCED_FACE('',(#17164),#6406,.T.) ;
#64450=ADVANCED_FACE('',(#17165),#6407,.T.) ;
#64451=ADVANCED_FACE('',(#17166),#4285,.T.) ;
#64452=ADVANCED_FACE('',(#17167),#4286,.T.) ;
#64453=ADVANCED_FACE('',(#17168),#6408,.T.) ;
#64454=ADVANCED_FACE('',(#17169),#6409,.T.) ;
#64455=ADVANCED_FACE('',(#17170),#4287,.T.) ;
#64456=ADVANCED_FACE('',(#17171),#4288,.T.) ;
#64457=ADVANCED_FACE('',(#17172),#6410,.T.) ;
#64458=ADVANCED_FACE('',(#17173),#6411,.T.) ;
#64459=ADVANCED_FACE('',(#17174),#4289,.T.) ;
#64460=ADVANCED_FACE('',(#17175),#4290,.T.) ;
#64461=ADVANCED_FACE('',(#17176),#6412,.T.) ;
#64462=ADVANCED_FACE('',(#17177),#6413,.T.) ;
#64463=ADVANCED_FACE('',(#17178),#4291,.T.) ;
#64464=ADVANCED_FACE('',(#17179),#6414,.T.) ;
#64465=ADVANCED_FACE('',(#17180),#4292,.T.) ;
#64466=ADVANCED_FACE('',(#17181),#410,.T.) ;
#64467=ADVANCED_FACE('',(#17182),#4293,.T.) ;
#64468=ADVANCED_FACE('',(#17183),#6415,.T.) ;
#64469=ADVANCED_FACE('',(#17184),#411,.T.) ;
#64470=ADVANCED_FACE('',(#17185),#6416,.T.) ;
#64471=ADVANCED_FACE('',(#17186),#412,.T.) ;
#64472=ADVANCED_FACE('',(#17187),#6417,.T.) ;
#64473=ADVANCED_FACE('',(#17188),#413,.F.) ;
#64474=ADVANCED_FACE('',(#17189),#414,.F.) ;
#64475=ADVANCED_FACE('',(#17190),#63006,.T.) ;
#64476=ADVANCED_FACE('',(#17191),#63007,.F.) ;
#64477=ADVANCED_FACE('',(#17192),#6418,.F.) ;
#64478=ADVANCED_FACE('',(#17193),#6419,.F.) ;
#64479=ADVANCED_FACE('',(#17194),#63008,.T.) ;
#64480=ADVANCED_FACE('',(#17195),#6420,.T.) ;
#64481=ADVANCED_FACE('',(#17196),#6421,.F.) ;
#64482=ADVANCED_FACE('',(#17197),#5279,.T.) ;
#64483=ADVANCED_FACE('',(#17198),#5280,.T.) ;
#64484=ADVANCED_FACE('',(#17199),#5281,.T.) ;
#64485=ADVANCED_FACE('',(#17200),#5282,.T.) ;
#64486=ADVANCED_FACE('',(#17201),#5283,.T.) ;
#64487=ADVANCED_FACE('',(#17202),#5284,.T.) ;
#64488=ADVANCED_FACE('',(#17203),#5285,.T.) ;
#64489=ADVANCED_FACE('',(#17204),#5286,.F.) ;
#64490=ADVANCED_FACE('',(#17205),#5287,.T.) ;
#64491=ADVANCED_FACE('',(#17206),#5288,.T.) ;
#64492=ADVANCED_FACE('',(#17207),#5289,.T.) ;
#64493=ADVANCED_FACE('',(#17208),#5290,.T.) ;
#64494=ADVANCED_FACE('',(#17209),#5291,.T.) ;
#64495=ADVANCED_FACE('',(#17210),#5292,.T.) ;
#64496=ADVANCED_FACE('',(#17211),#5293,.T.) ;
#64497=ADVANCED_FACE('',(#17212),#5294,.T.) ;
#64498=ADVANCED_FACE('',(#17213,#5023),#5295,.T.) ;
#64499=ADVANCED_FACE('',(#17214),#5296,.T.) ;
#64500=ADVANCED_FACE('',(#17215),#5297,.T.) ;
#64501=ADVANCED_FACE('',(#17216),#5298,.F.) ;
#64502=ADVANCED_FACE('',(#17217),#5299,.F.) ;
#64503=ADVANCED_FACE('',(#17218),#5300,.T.) ;
#64504=ADVANCED_FACE('',(#17219),#5301,.F.) ;
#64505=ADVANCED_FACE('',(#17220),#5302,.F.) ;
#64506=ADVANCED_FACE('',(#17221),#5303,.F.) ;
#64507=ADVANCED_FACE('',(#17222),#5304,.T.) ;
#64508=ADVANCED_FACE('',(#17223),#5305,.F.) ;
#64509=ADVANCED_FACE('',(#17224,#5024),#5306,.T.) ;
#64510=ADVANCED_FACE('',(#17225),#5307,.T.) ;
#64511=ADVANCED_FACE('',(#17226),#5308,.F.) ;
#64512=ADVANCED_FACE('',(#17227),#5309,.F.) ;
#64513=ADVANCED_FACE('',(#17228),#6422,.T.) ;
#64514=ADVANCED_FACE('',(#17229),#6423,.T.) ;
#64515=ADVANCED_FACE('',(#17230),#5310,.F.) ;
#64516=ADVANCED_FACE('',(#17231),#5311,.F.) ;
#64517=ADVANCED_FACE('',(#17232),#5312,.F.) ;
#64518=ADVANCED_FACE('',(#17233),#5313,.T.) ;
#64519=ADVANCED_FACE('',(#17234),#5314,.F.) ;
#64520=ADVANCED_FACE('',(#17235),#6424,.T.) ;
#64521=ADVANCED_FACE('',(#17236),#5315,.F.) ;
#64522=ADVANCED_FACE('',(#17237),#6425,.T.) ;
#64523=ADVANCED_FACE('',(#17238),#5316,.F.) ;
#64524=ADVANCED_FACE('',(#17239),#5317,.F.) ;
#64525=ADVANCED_FACE('',(#17240),#5318,.F.) ;
#64526=ADVANCED_FACE('',(#17241),#5319,.F.) ;
#64527=ADVANCED_FACE('',(#17242),#5320,.F.) ;
#64528=ADVANCED_FACE('',(#17243),#5321,.F.) ;
#64529=ADVANCED_FACE('',(#17244),#5322,.F.) ;
#64530=ADVANCED_FACE('',(#17245),#5323,.F.) ;
#64531=ADVANCED_FACE('',(#17246),#5324,.F.) ;
#64532=ADVANCED_FACE('',(#17247),#5325,.T.) ;
#64533=ADVANCED_FACE('',(#17248),#5326,.F.) ;
#64534=ADVANCED_FACE('',(#17249),#5327,.F.) ;
#64535=ADVANCED_FACE('',(#17250),#5328,.F.) ;
#64536=ADVANCED_FACE('',(#17251),#5329,.T.) ;
#64537=ADVANCED_FACE('',(#17252),#5330,.F.) ;
#64538=ADVANCED_FACE('',(#17253),#6426,.T.) ;
#64539=ADVANCED_FACE('',(#17254),#5331,.F.) ;
#64540=ADVANCED_FACE('',(#17255),#5332,.F.) ;
#64541=ADVANCED_FACE('',(#17256),#5333,.F.) ;
#64542=ADVANCED_FACE('',(#17257),#5334,.F.) ;
#64543=ADVANCED_FACE('',(#17258),#5335,.F.) ;
#64544=ADVANCED_FACE('',(#17259),#6427,.F.) ;
#64545=ADVANCED_FACE('',(#17260),#5336,.F.) ;
#64546=ADVANCED_FACE('',(#17261),#5337,.F.) ;
#64547=ADVANCED_FACE('',(#17262),#5338,.F.) ;
#64548=ADVANCED_FACE('',(#17263),#5339,.F.) ;
#64549=ADVANCED_FACE('',(#17264),#5340,.F.) ;
#64550=ADVANCED_FACE('',(#17265),#16132,.F.) ;
#64551=ADVANCED_FACE('',(#17266),#5341,.F.) ;
#64552=ADVANCED_FACE('',(#17267),#6428,.F.) ;
#64553=ADVANCED_FACE('',(#17268),#4294,.F.) ;
#64554=ADVANCED_FACE('',(#17269),#6429,.T.) ;
#64555=ADVANCED_FACE('',(#17270),#6430,.F.) ;
#64556=ADVANCED_FACE('',(#17271),#63009,.F.) ;
#64557=ADVANCED_FACE('',(#17272),#63010,.T.) ;
#64558=ADVANCED_FACE('',(#17273),#4295,.F.) ;
#64559=ADVANCED_FACE('',(#17274),#6431,.F.) ;
#64560=ADVANCED_FACE('',(#17275),#6432,.F.) ;
#64561=ADVANCED_FACE('',(#17276),#6433,.T.) ;
#64562=ADVANCED_FACE('',(#17277),#63011,.T.) ;
#64563=ADVANCED_FACE('',(#17278),#6434,.F.) ;
#64564=ADVANCED_FACE('',(#17279),#6435,.F.) ;
#64565=ADVANCED_FACE('',(#17280),#6436,.F.) ;
#64566=ADVANCED_FACE('',(#17281),#4296,.F.) ;
#64567=ADVANCED_FACE('',(#17282),#63012,.T.) ;
#64568=ADVANCED_FACE('',(#17283),#63013,.T.) ;
#64569=ADVANCED_FACE('',(#17284),#4297,.F.) ;
#64570=ADVANCED_FACE('',(#17285),#63014,.F.) ;
#64571=ADVANCED_FACE('',(#17286),#6437,.F.) ;
#64572=ADVANCED_FACE('',(#17287),#63015,.T.) ;
#64573=ADVANCED_FACE('',(#17288),#6438,.T.) ;
#64574=ADVANCED_FACE('',(#17289),#6439,.F.) ;
#64575=ADVANCED_FACE('',(#17290),#4298,.F.) ;
#64576=ADVANCED_FACE('',(#17291),#63016,.T.) ;
#64577=ADVANCED_FACE('',(#17292),#63017,.F.) ;
#64578=ADVANCED_FACE('',(#17293),#6440,.F.) ;
#64579=ADVANCED_FACE('',(#17294),#6441,.F.) ;
#64580=ADVANCED_FACE('',(#17295),#6442,.T.) ;
#64581=ADVANCED_FACE('',(#17296),#6443,.F.) ;
#64582=ADVANCED_FACE('',(#17297),#4299,.F.) ;
#64583=ADVANCED_FACE('',(#17298),#63018,.F.) ;
#64584=ADVANCED_FACE('',(#17299),#6444,.F.) ;
#64585=ADVANCED_FACE('',(#17300),#4300,.T.) ;
#64586=ADVANCED_FACE('',(#17301),#6445,.T.) ;
#64587=ADVANCED_FACE('',(#17302),#6446,.T.) ;
#64588=ADVANCED_FACE('',(#17303),#6447,.T.) ;
#64589=ADVANCED_FACE('',(#17304),#6448,.T.) ;
#64590=ADVANCED_FACE('',(#17305),#6449,.T.) ;
#64591=ADVANCED_FACE('',(#17306),#63019,.F.) ;
#64592=ADVANCED_FACE('',(#17307),#6450,.F.) ;
#64593=ADVANCED_FACE('',(#17308),#4301,.F.) ;
#64594=ADVANCED_FACE('',(#17309),#6451,.T.) ;
#64595=ADVANCED_FACE('',(#17310),#6452,.T.) ;
#64596=ADVANCED_FACE('',(#17311),#6453,.F.) ;
#64597=ADVANCED_FACE('',(#17312),#6454,.T.) ;
#64598=ADVANCED_FACE('',(#17313),#63020,.T.) ;
#64599=ADVANCED_FACE('',(#17314),#6455,.F.) ;
#64600=ADVANCED_FACE('',(#17315),#4302,.T.) ;
#64601=ADVANCED_FACE('',(#17316),#4303,.F.) ;
#64602=ADVANCED_FACE('',(#17317),#6456,.T.) ;
#64603=ADVANCED_FACE('',(#17318),#6457,.T.) ;
#64604=ADVANCED_FACE('',(#17319),#4304,.F.) ;
#64605=ADVANCED_FACE('',(#17320),#6458,.T.) ;
#64606=ADVANCED_FACE('',(#17321),#6459,.F.) ;
#64607=ADVANCED_FACE('',(#17322),#63021,.T.) ;
#64608=ADVANCED_FACE('',(#17323),#63022,.T.) ;
#64609=ADVANCED_FACE('',(#17324),#6460,.F.) ;
#64610=ADVANCED_FACE('',(#17325),#63023,.F.) ;
#64611=ADVANCED_FACE('',(#17326),#4305,.F.) ;
#64612=ADVANCED_FACE('',(#17327),#6461,.T.) ;
#64613=ADVANCED_FACE('',(#17328),#6462,.T.) ;
#64614=ADVANCED_FACE('',(#17329),#6463,.F.) ;
#64615=ADVANCED_FACE('',(#17330),#63024,.T.) ;
#64616=ADVANCED_FACE('',(#17331),#6464,.T.) ;
#64617=ADVANCED_FACE('',(#17332),#6465,.F.) ;
#64618=ADVANCED_FACE('',(#17333),#4306,.F.) ;
#64619=ADVANCED_FACE('',(#17334),#6466,.T.) ;
#64620=ADVANCED_FACE('',(#17335),#6467,.F.) ;
#64621=ADVANCED_FACE('',(#17336),#63025,.F.) ;
#64622=ADVANCED_FACE('',(#17337),#6468,.F.) ;
#64623=ADVANCED_FACE('',(#17338),#6469,.T.) ;
#64624=ADVANCED_FACE('',(#17339),#63026,.T.) ;
#64625=ADVANCED_FACE('',(#17340),#4307,.F.) ;
#64626=ADVANCED_FACE('',(#17341),#63027,.F.) ;
#64627=ADVANCED_FACE('',(#17342),#63028,.T.) ;
#64628=ADVANCED_FACE('',(#17343),#6470,.F.) ;
#64629=ADVANCED_FACE('',(#17344),#6471,.F.) ;
#64630=ADVANCED_FACE('',(#17345),#63029,.F.) ;
#64631=ADVANCED_FACE('',(#17346),#6472,.T.) ;
#64632=ADVANCED_FACE('',(#17347),#6473,.F.) ;
#64633=ADVANCED_FACE('',(#17348),#6474,.F.) ;
#64634=ADVANCED_FACE('',(#17349),#63030,.T.) ;
#64635=ADVANCED_FACE('',(#17350),#4308,.F.) ;
#64636=ADVANCED_FACE('',(#17351),#63031,.F.) ;
#64637=ADVANCED_FACE('',(#17352),#4309,.F.) ;
#64638=ADVANCED_FACE('',(#17353),#6475,.T.) ;
#64639=ADVANCED_FACE('',(#17354),#63032,.F.) ;
#64640=ADVANCED_FACE('',(#17355),#6476,.F.) ;
#64641=ADVANCED_FACE('',(#17356),#63033,.F.) ;
#64642=ADVANCED_FACE('',(#17357),#6477,.F.) ;
#64643=ADVANCED_FACE('',(#17358),#6478,.T.) ;
#64644=ADVANCED_FACE('',(#17359),#415,.F.) ;
#64645=ADVANCED_FACE('',(#17360),#4310,.F.) ;
#64646=ADVANCED_FACE('',(#17361),#4311,.F.) ;
#64647=ADVANCED_FACE('',(#17362),#63034,.T.) ;
#64648=ADVANCED_FACE('',(#17363),#63035,.F.) ;
#64649=ADVANCED_FACE('',(#17364),#6479,.F.) ;
#64650=ADVANCED_FACE('',(#17365),#63036,.T.) ;
#64651=ADVANCED_FACE('',(#17366),#416,.F.) ;
#64652=ADVANCED_FACE('',(#17367),#63037,.T.) ;
#64653=ADVANCED_FACE('',(#17368),#6480,.T.) ;
#64654=ADVANCED_FACE('',(#17369),#63038,.T.) ;
#64655=ADVANCED_FACE('',(#17370),#6481,.T.) ;
#64656=ADVANCED_FACE('',(#17371),#63039,.T.) ;
#64657=ADVANCED_FACE('',(#17372),#6482,.T.) ;
#64658=ADVANCED_FACE('',(#17373),#63040,.T.) ;
#64659=ADVANCED_FACE('',(#17374),#6483,.T.) ;
#64660=ADVANCED_FACE('',(#17375),#4312,.T.) ;
#64661=ADVANCED_FACE('',(#17376),#6484,.T.) ;
#64662=ADVANCED_FACE('',(#17377),#6485,.T.) ;
#64663=ADVANCED_FACE('',(#17378),#6486,.T.) ;
#64664=ADVANCED_FACE('',(#17379),#6487,.T.) ;
#64665=ADVANCED_FACE('',(#17380),#6488,.T.) ;
#64666=ADVANCED_FACE('',(#17381),#4313,.T.) ;
#64667=ADVANCED_FACE('',(#17382),#4314,.T.) ;
#64668=ADVANCED_FACE('',(#17383),#6489,.T.) ;
#64669=ADVANCED_FACE('',(#17384),#6490,.T.) ;
#64670=ADVANCED_FACE('',(#17385),#4315,.T.) ;
#64671=ADVANCED_FACE('',(#17386),#6491,.T.) ;
#64672=ADVANCED_FACE('',(#17387),#6492,.T.) ;
#64673=ADVANCED_FACE('',(#17388),#63041,.T.) ;
#64674=ADVANCED_FACE('',(#17389),#6493,.T.) ;
#64675=ADVANCED_FACE('',(#17390),#6494,.T.) ;
#64676=ADVANCED_FACE('',(#17391),#6495,.T.) ;
#64677=ADVANCED_FACE('',(#17392),#6496,.T.) ;
#64678=ADVANCED_FACE('',(#17393),#6497,.T.) ;
#64679=ADVANCED_FACE('',(#17394),#4316,.T.) ;
#64680=ADVANCED_FACE('',(#17395),#6498,.T.) ;
#64681=ADVANCED_FACE('',(#17396),#6499,.T.) ;
#64682=ADVANCED_FACE('',(#17397),#4317,.T.) ;
#64683=ADVANCED_FACE('',(#17398),#6500,.T.) ;
#64684=ADVANCED_FACE('',(#17399),#6501,.T.) ;
#64685=ADVANCED_FACE('',(#17400),#6502,.T.) ;
#64686=ADVANCED_FACE('',(#17401),#6503,.T.) ;
#64687=ADVANCED_FACE('',(#17402),#4318,.T.) ;
#64688=ADVANCED_FACE('',(#17403),#4319,.T.) ;
#64689=ADVANCED_FACE('',(#17404),#6504,.T.) ;
#64690=ADVANCED_FACE('',(#17405),#6505,.T.) ;
#64691=ADVANCED_FACE('',(#17406),#6506,.T.) ;
#64692=ADVANCED_FACE('',(#17407),#4320,.T.) ;
#64693=ADVANCED_FACE('',(#17408),#6507,.T.) ;
#64694=ADVANCED_FACE('',(#17409),#6508,.T.) ;
#64695=ADVANCED_FACE('',(#17410),#4321,.T.) ;
#64696=ADVANCED_FACE('',(#17411),#6509,.T.) ;
#64697=ADVANCED_FACE('',(#17412),#6510,.T.) ;
#64698=ADVANCED_FACE('',(#17413),#6511,.T.) ;
#64699=ADVANCED_FACE('',(#17414),#4322,.T.) ;
#64700=ADVANCED_FACE('',(#17415),#6512,.T.) ;
#64701=ADVANCED_FACE('',(#17416),#6513,.T.) ;
#64702=ADVANCED_FACE('',(#17417),#4323,.T.) ;
#64703=ADVANCED_FACE('',(#17418),#6514,.T.) ;
#64704=ADVANCED_FACE('',(#17419),#6515,.F.) ;
#64705=ADVANCED_FACE('',(#17420),#6516,.T.) ;
#64706=ADVANCED_FACE('',(#17421),#6517,.F.) ;
#64707=ADVANCED_FACE('',(#17422),#6518,.T.) ;
#64708=ADVANCED_FACE('',(#17423),#6519,.T.) ;
#64709=ADVANCED_FACE('',(#17424),#6520,.T.) ;
#64710=ADVANCED_FACE('',(#17425),#63042,.T.) ;
#64711=ADVANCED_FACE('',(#17426),#6521,.T.) ;
#64712=ADVANCED_FACE('',(#17427),#417,.F.) ;
#64713=ADVANCED_FACE('',(#17428),#6522,.F.) ;
#64714=ADVANCED_FACE('',(#17429),#4324,.F.) ;
#64715=ADVANCED_FACE('',(#17430),#6523,.F.) ;
#64716=ADVANCED_FACE('',(#17431),#418,.F.) ;
#64717=ADVANCED_FACE('',(#17432),#419,.F.) ;
#64718=ADVANCED_FACE('',(#17433),#6524,.F.) ;
#64719=ADVANCED_FACE('',(#17434),#4325,.F.) ;
#64720=ADVANCED_FACE('',(#17435),#6525,.F.) ;
#64721=ADVANCED_FACE('',(#17436),#420,.F.) ;
#64722=ADVANCED_FACE('',(#17437),#421,.F.) ;
#64723=ADVANCED_FACE('',(#17438),#6526,.F.) ;
#64724=ADVANCED_FACE('',(#17439),#422,.F.) ;
#64725=ADVANCED_FACE('',(#17440),#6527,.T.) ;
#64726=ADVANCED_FACE('',(#17441),#423,.T.) ;
#64727=ADVANCED_FACE('',(#17442),#424,.F.) ;
#64728=ADVANCED_FACE('',(#17443),#6528,.T.) ;
#64729=ADVANCED_FACE('',(#17444),#6529,.T.) ;
#64730=ADVANCED_FACE('',(#17445),#6530,.F.) ;
#64731=ADVANCED_FACE('',(#17446),#425,.T.) ;
#64732=ADVANCED_FACE('',(#17447),#426,.F.) ;
#64733=ADVANCED_FACE('',(#17448),#6531,.T.) ;
#64734=ADVANCED_FACE('',(#17449),#4326,.T.) ;
#64735=ADVANCED_FACE('',(#17450),#427,.T.) ;
#64736=ADVANCED_FACE('',(#17451),#4327,.T.) ;
#64737=ADVANCED_FACE('',(#17452),#4328,.T.) ;
#64738=ADVANCED_FACE('',(#17453),#6532,.T.) ;
#64739=ADVANCED_FACE('',(#17454),#6533,.T.) ;
#64740=ADVANCED_FACE('',(#17455),#4329,.T.) ;
#64741=ADVANCED_FACE('',(#17456),#4330,.T.) ;
#64742=ADVANCED_FACE('',(#17457),#6534,.T.) ;
#64743=ADVANCED_FACE('',(#17458),#6535,.T.) ;
#64744=ADVANCED_FACE('',(#17459),#4331,.T.) ;
#64745=ADVANCED_FACE('',(#17460),#4332,.T.) ;
#64746=ADVANCED_FACE('',(#17461),#6536,.T.) ;
#64747=ADVANCED_FACE('',(#17462),#6537,.T.) ;
#64748=ADVANCED_FACE('',(#17463),#4333,.T.) ;
#64749=ADVANCED_FACE('',(#17464),#4334,.T.) ;
#64750=ADVANCED_FACE('',(#17465),#6538,.T.) ;
#64751=ADVANCED_FACE('',(#17466),#6539,.T.) ;
#64752=ADVANCED_FACE('',(#17467),#4335,.T.) ;
#64753=ADVANCED_FACE('',(#17468),#6540,.T.) ;
#64754=ADVANCED_FACE('',(#17469),#4336,.T.) ;
#64755=ADVANCED_FACE('',(#17470),#428,.T.) ;
#64756=ADVANCED_FACE('',(#17471),#4337,.T.) ;
#64757=ADVANCED_FACE('',(#17472),#6541,.T.) ;
#64758=ADVANCED_FACE('',(#17473),#429,.T.) ;
#64759=ADVANCED_FACE('',(#17474),#6542,.T.) ;
#64760=ADVANCED_FACE('',(#17475),#430,.T.) ;
#64761=ADVANCED_FACE('',(#17476),#6543,.T.) ;
#64762=ADVANCED_FACE('',(#17477),#431,.F.) ;
#64763=ADVANCED_FACE('',(#17478),#432,.F.) ;
#64764=ADVANCED_FACE('',(#17479),#63043,.T.) ;
#64765=ADVANCED_FACE('',(#17480),#63044,.F.) ;
#64766=ADVANCED_FACE('',(#17481),#6544,.F.) ;
#64767=ADVANCED_FACE('',(#17482),#6545,.F.) ;
#64768=ADVANCED_FACE('',(#17483),#63045,.T.) ;
#64769=ADVANCED_FACE('',(#17484),#6546,.T.) ;
#64770=ADVANCED_FACE('',(#17485),#6547,.F.) ;
#64771=ADVANCED_FACE('',(#17486),#5342,.T.) ;
#64772=ADVANCED_FACE('',(#17487),#5343,.T.) ;
#64773=ADVANCED_FACE('',(#17488),#5344,.T.) ;
#64774=ADVANCED_FACE('',(#17489),#5345,.T.) ;
#64775=ADVANCED_FACE('',(#17490),#5346,.T.) ;
#64776=ADVANCED_FACE('',(#17491),#5347,.T.) ;
#64777=ADVANCED_FACE('',(#17492),#5348,.T.) ;
#64778=ADVANCED_FACE('',(#17493),#5349,.F.) ;
#64779=ADVANCED_FACE('',(#17494),#5350,.T.) ;
#64780=ADVANCED_FACE('',(#17495),#5351,.T.) ;
#64781=ADVANCED_FACE('',(#17496),#5352,.T.) ;
#64782=ADVANCED_FACE('',(#17497),#5353,.T.) ;
#64783=ADVANCED_FACE('',(#17498),#5354,.T.) ;
#64784=ADVANCED_FACE('',(#17499),#5355,.T.) ;
#64785=ADVANCED_FACE('',(#17500),#5356,.T.) ;
#64786=ADVANCED_FACE('',(#17501),#5357,.T.) ;
#64787=ADVANCED_FACE('',(#17502,#5025),#5358,.T.) ;
#64788=ADVANCED_FACE('',(#17503),#5359,.T.) ;
#64789=ADVANCED_FACE('',(#17504),#5360,.T.) ;
#64790=ADVANCED_FACE('',(#17505),#5361,.F.) ;
#64791=ADVANCED_FACE('',(#17506),#5362,.F.) ;
#64792=ADVANCED_FACE('',(#17507),#5363,.T.) ;
#64793=ADVANCED_FACE('',(#17508),#5364,.F.) ;
#64794=ADVANCED_FACE('',(#17509),#5365,.F.) ;
#64795=ADVANCED_FACE('',(#17510),#5366,.F.) ;
#64796=ADVANCED_FACE('',(#17511),#5367,.T.) ;
#64797=ADVANCED_FACE('',(#17512),#5368,.F.) ;
#64798=ADVANCED_FACE('',(#17513,#5026),#5369,.T.) ;
#64799=ADVANCED_FACE('',(#17514),#5370,.T.) ;
#64800=ADVANCED_FACE('',(#17515),#5371,.F.) ;
#64801=ADVANCED_FACE('',(#17516),#5372,.F.) ;
#64802=ADVANCED_FACE('',(#17517),#6548,.T.) ;
#64803=ADVANCED_FACE('',(#17518),#6549,.T.) ;
#64804=ADVANCED_FACE('',(#17519),#5373,.F.) ;
#64805=ADVANCED_FACE('',(#17520),#5374,.F.) ;
#64806=ADVANCED_FACE('',(#17521),#5375,.F.) ;
#64807=ADVANCED_FACE('',(#17522),#5376,.T.) ;
#64808=ADVANCED_FACE('',(#17523),#5377,.F.) ;
#64809=ADVANCED_FACE('',(#17524),#6550,.T.) ;
#64810=ADVANCED_FACE('',(#17525),#5378,.F.) ;
#64811=ADVANCED_FACE('',(#17526),#6551,.T.) ;
#64812=ADVANCED_FACE('',(#17527),#5379,.F.) ;
#64813=ADVANCED_FACE('',(#17528),#5380,.F.) ;
#64814=ADVANCED_FACE('',(#17529),#5381,.F.) ;
#64815=ADVANCED_FACE('',(#17530),#5382,.F.) ;
#64816=ADVANCED_FACE('',(#17531),#5383,.F.) ;
#64817=ADVANCED_FACE('',(#17532),#5384,.F.) ;
#64818=ADVANCED_FACE('',(#17533),#5385,.F.) ;
#64819=ADVANCED_FACE('',(#17534),#5386,.F.) ;
#64820=ADVANCED_FACE('',(#17535),#5387,.F.) ;
#64821=ADVANCED_FACE('',(#17536),#5388,.T.) ;
#64822=ADVANCED_FACE('',(#17537),#5389,.F.) ;
#64823=ADVANCED_FACE('',(#17538),#5390,.F.) ;
#64824=ADVANCED_FACE('',(#17539),#5391,.F.) ;
#64825=ADVANCED_FACE('',(#17540),#5392,.T.) ;
#64826=ADVANCED_FACE('',(#17541),#5393,.F.) ;
#64827=ADVANCED_FACE('',(#17542),#6552,.T.) ;
#64828=ADVANCED_FACE('',(#17543),#5394,.F.) ;
#64829=ADVANCED_FACE('',(#17544),#5395,.F.) ;
#64830=ADVANCED_FACE('',(#17545),#5396,.F.) ;
#64831=ADVANCED_FACE('',(#17546),#5397,.F.) ;
#64832=ADVANCED_FACE('',(#17547),#5398,.F.) ;
#64833=ADVANCED_FACE('',(#17548),#6553,.F.) ;
#64834=ADVANCED_FACE('',(#17549),#5399,.F.) ;
#64835=ADVANCED_FACE('',(#17550),#5400,.F.) ;
#64836=ADVANCED_FACE('',(#17551),#5401,.F.) ;
#64837=ADVANCED_FACE('',(#17552),#5402,.F.) ;
#64838=ADVANCED_FACE('',(#17553),#5403,.F.) ;
#64839=ADVANCED_FACE('',(#17554),#16133,.F.) ;
#64840=ADVANCED_FACE('',(#17555),#5404,.F.) ;
#64841=ADVANCED_FACE('',(#17556),#6554,.F.) ;
#64842=ADVANCED_FACE('',(#17557),#4338,.F.) ;
#64843=ADVANCED_FACE('',(#17558),#6555,.T.) ;
#64844=ADVANCED_FACE('',(#17559),#6556,.F.) ;
#64845=ADVANCED_FACE('',(#17560),#63046,.F.) ;
#64846=ADVANCED_FACE('',(#17561),#63047,.T.) ;
#64847=ADVANCED_FACE('',(#17562),#4339,.F.) ;
#64848=ADVANCED_FACE('',(#17563),#6557,.F.) ;
#64849=ADVANCED_FACE('',(#17564),#6558,.F.) ;
#64850=ADVANCED_FACE('',(#17565),#6559,.T.) ;
#64851=ADVANCED_FACE('',(#17566),#63048,.T.) ;
#64852=ADVANCED_FACE('',(#17567),#6560,.F.) ;
#64853=ADVANCED_FACE('',(#17568),#6561,.F.) ;
#64854=ADVANCED_FACE('',(#17569),#6562,.F.) ;
#64855=ADVANCED_FACE('',(#17570),#4340,.F.) ;
#64856=ADVANCED_FACE('',(#17571),#63049,.T.) ;
#64857=ADVANCED_FACE('',(#17572),#63050,.T.) ;
#64858=ADVANCED_FACE('',(#17573),#4341,.F.) ;
#64859=ADVANCED_FACE('',(#17574),#63051,.F.) ;
#64860=ADVANCED_FACE('',(#17575),#6563,.F.) ;
#64861=ADVANCED_FACE('',(#17576),#63052,.T.) ;
#64862=ADVANCED_FACE('',(#17577),#6564,.T.) ;
#64863=ADVANCED_FACE('',(#17578),#6565,.F.) ;
#64864=ADVANCED_FACE('',(#17579),#4342,.F.) ;
#64865=ADVANCED_FACE('',(#17580),#63053,.T.) ;
#64866=ADVANCED_FACE('',(#17581),#63054,.F.) ;
#64867=ADVANCED_FACE('',(#17582),#6566,.F.) ;
#64868=ADVANCED_FACE('',(#17583),#6567,.F.) ;
#64869=ADVANCED_FACE('',(#17584),#6568,.T.) ;
#64870=ADVANCED_FACE('',(#17585),#6569,.F.) ;
#64871=ADVANCED_FACE('',(#17586),#4343,.F.) ;
#64872=ADVANCED_FACE('',(#17587),#63055,.F.) ;
#64873=ADVANCED_FACE('',(#17588),#6570,.F.) ;
#64874=ADVANCED_FACE('',(#17589),#4344,.T.) ;
#64875=ADVANCED_FACE('',(#17590),#6571,.T.) ;
#64876=ADVANCED_FACE('',(#17591),#6572,.T.) ;
#64877=ADVANCED_FACE('',(#17592),#6573,.T.) ;
#64878=ADVANCED_FACE('',(#17593),#6574,.T.) ;
#64879=ADVANCED_FACE('',(#17594),#6575,.T.) ;
#64880=ADVANCED_FACE('',(#17595),#63056,.F.) ;
#64881=ADVANCED_FACE('',(#17596),#6576,.F.) ;
#64882=ADVANCED_FACE('',(#17597),#4345,.F.) ;
#64883=ADVANCED_FACE('',(#17598),#6577,.T.) ;
#64884=ADVANCED_FACE('',(#17599),#6578,.T.) ;
#64885=ADVANCED_FACE('',(#17600),#6579,.F.) ;
#64886=ADVANCED_FACE('',(#17601),#6580,.T.) ;
#64887=ADVANCED_FACE('',(#17602),#63057,.T.) ;
#64888=ADVANCED_FACE('',(#17603),#6581,.F.) ;
#64889=ADVANCED_FACE('',(#17604),#4346,.T.) ;
#64890=ADVANCED_FACE('',(#17605),#4347,.F.) ;
#64891=ADVANCED_FACE('',(#17606),#6582,.T.) ;
#64892=ADVANCED_FACE('',(#17607),#6583,.T.) ;
#64893=ADVANCED_FACE('',(#17608),#4348,.F.) ;
#64894=ADVANCED_FACE('',(#17609),#6584,.T.) ;
#64895=ADVANCED_FACE('',(#17610),#6585,.F.) ;
#64896=ADVANCED_FACE('',(#17611),#63058,.T.) ;
#64897=ADVANCED_FACE('',(#17612),#63059,.T.) ;
#64898=ADVANCED_FACE('',(#17613),#6586,.F.) ;
#64899=ADVANCED_FACE('',(#17614),#63060,.F.) ;
#64900=ADVANCED_FACE('',(#17615),#4349,.F.) ;
#64901=ADVANCED_FACE('',(#17616),#6587,.T.) ;
#64902=ADVANCED_FACE('',(#17617),#6588,.T.) ;
#64903=ADVANCED_FACE('',(#17618),#6589,.F.) ;
#64904=ADVANCED_FACE('',(#17619),#63061,.T.) ;
#64905=ADVANCED_FACE('',(#17620),#6590,.T.) ;
#64906=ADVANCED_FACE('',(#17621),#6591,.F.) ;
#64907=ADVANCED_FACE('',(#17622),#4350,.F.) ;
#64908=ADVANCED_FACE('',(#17623),#6592,.T.) ;
#64909=ADVANCED_FACE('',(#17624),#6593,.F.) ;
#64910=ADVANCED_FACE('',(#17625),#63062,.F.) ;
#64911=ADVANCED_FACE('',(#17626),#6594,.F.) ;
#64912=ADVANCED_FACE('',(#17627),#6595,.T.) ;
#64913=ADVANCED_FACE('',(#17628),#63063,.T.) ;
#64914=ADVANCED_FACE('',(#17629),#4351,.F.) ;
#64915=ADVANCED_FACE('',(#17630),#63064,.F.) ;
#64916=ADVANCED_FACE('',(#17631),#63065,.T.) ;
#64917=ADVANCED_FACE('',(#17632),#6596,.F.) ;
#64918=ADVANCED_FACE('',(#17633),#6597,.F.) ;
#64919=ADVANCED_FACE('',(#17634),#63066,.F.) ;
#64920=ADVANCED_FACE('',(#17635),#6598,.T.) ;
#64921=ADVANCED_FACE('',(#17636),#6599,.F.) ;
#64922=ADVANCED_FACE('',(#17637),#6600,.F.) ;
#64923=ADVANCED_FACE('',(#17638),#63067,.T.) ;
#64924=ADVANCED_FACE('',(#17639),#4352,.F.) ;
#64925=ADVANCED_FACE('',(#17640),#63068,.F.) ;
#64926=ADVANCED_FACE('',(#17641),#4353,.F.) ;
#64927=ADVANCED_FACE('',(#17642),#6601,.T.) ;
#64928=ADVANCED_FACE('',(#17643),#63069,.F.) ;
#64929=ADVANCED_FACE('',(#17644),#6602,.F.) ;
#64930=ADVANCED_FACE('',(#17645),#63070,.F.) ;
#64931=ADVANCED_FACE('',(#17646),#6603,.F.) ;
#64932=ADVANCED_FACE('',(#17647),#6604,.T.) ;
#64933=ADVANCED_FACE('',(#17648),#433,.F.) ;
#64934=ADVANCED_FACE('',(#17649),#4354,.F.) ;
#64935=ADVANCED_FACE('',(#17650),#4355,.F.) ;
#64936=ADVANCED_FACE('',(#17651),#63071,.T.) ;
#64937=ADVANCED_FACE('',(#17652),#63072,.F.) ;
#64938=ADVANCED_FACE('',(#17653),#6605,.F.) ;
#64939=ADVANCED_FACE('',(#17654),#63073,.T.) ;
#64940=ADVANCED_FACE('',(#17655),#434,.F.) ;
#64941=ADVANCED_FACE('',(#17656),#63074,.T.) ;
#64942=ADVANCED_FACE('',(#17657),#6606,.T.) ;
#64943=ADVANCED_FACE('',(#17658),#63075,.T.) ;
#64944=ADVANCED_FACE('',(#17659),#6607,.T.) ;
#64945=ADVANCED_FACE('',(#17660),#63076,.T.) ;
#64946=ADVANCED_FACE('',(#17661),#6608,.T.) ;
#64947=ADVANCED_FACE('',(#17662),#63077,.T.) ;
#64948=ADVANCED_FACE('',(#17663),#6609,.T.) ;
#64949=ADVANCED_FACE('',(#17664),#4356,.T.) ;
#64950=ADVANCED_FACE('',(#17665),#6610,.T.) ;
#64951=ADVANCED_FACE('',(#17666),#6611,.T.) ;
#64952=ADVANCED_FACE('',(#17667),#6612,.T.) ;
#64953=ADVANCED_FACE('',(#17668),#6613,.T.) ;
#64954=ADVANCED_FACE('',(#17669),#6614,.T.) ;
#64955=ADVANCED_FACE('',(#17670),#4357,.T.) ;
#64956=ADVANCED_FACE('',(#17671),#4358,.T.) ;
#64957=ADVANCED_FACE('',(#17672),#6615,.T.) ;
#64958=ADVANCED_FACE('',(#17673),#6616,.T.) ;
#64959=ADVANCED_FACE('',(#17674),#4359,.T.) ;
#64960=ADVANCED_FACE('',(#17675),#6617,.T.) ;
#64961=ADVANCED_FACE('',(#17676),#6618,.T.) ;
#64962=ADVANCED_FACE('',(#17677),#63078,.T.) ;
#64963=ADVANCED_FACE('',(#17678),#6619,.T.) ;
#64964=ADVANCED_FACE('',(#17679),#6620,.T.) ;
#64965=ADVANCED_FACE('',(#17680),#6621,.T.) ;
#64966=ADVANCED_FACE('',(#17681),#6622,.T.) ;
#64967=ADVANCED_FACE('',(#17682),#6623,.T.) ;
#64968=ADVANCED_FACE('',(#17683),#4360,.T.) ;
#64969=ADVANCED_FACE('',(#17684),#6624,.T.) ;
#64970=ADVANCED_FACE('',(#17685),#6625,.T.) ;
#64971=ADVANCED_FACE('',(#17686),#4361,.T.) ;
#64972=ADVANCED_FACE('',(#17687),#6626,.T.) ;
#64973=ADVANCED_FACE('',(#17688),#6627,.T.) ;
#64974=ADVANCED_FACE('',(#17689),#6628,.T.) ;
#64975=ADVANCED_FACE('',(#17690),#6629,.T.) ;
#64976=ADVANCED_FACE('',(#17691),#4362,.T.) ;
#64977=ADVANCED_FACE('',(#17692),#4363,.T.) ;
#64978=ADVANCED_FACE('',(#17693),#6630,.T.) ;
#64979=ADVANCED_FACE('',(#17694),#6631,.T.) ;
#64980=ADVANCED_FACE('',(#17695),#6632,.T.) ;
#64981=ADVANCED_FACE('',(#17696),#4364,.T.) ;
#64982=ADVANCED_FACE('',(#17697),#6633,.T.) ;
#64983=ADVANCED_FACE('',(#17698),#6634,.T.) ;
#64984=ADVANCED_FACE('',(#17699),#4365,.T.) ;
#64985=ADVANCED_FACE('',(#17700),#6635,.T.) ;
#64986=ADVANCED_FACE('',(#17701),#6636,.T.) ;
#64987=ADVANCED_FACE('',(#17702),#6637,.T.) ;
#64988=ADVANCED_FACE('',(#17703),#4366,.T.) ;
#64989=ADVANCED_FACE('',(#17704),#6638,.T.) ;
#64990=ADVANCED_FACE('',(#17705),#6639,.T.) ;
#64991=ADVANCED_FACE('',(#17706),#4367,.T.) ;
#64992=ADVANCED_FACE('',(#17707),#6640,.T.) ;
#64993=ADVANCED_FACE('',(#17708),#6641,.F.) ;
#64994=ADVANCED_FACE('',(#17709),#6642,.T.) ;
#64995=ADVANCED_FACE('',(#17710),#6643,.F.) ;
#64996=ADVANCED_FACE('',(#17711),#6644,.T.) ;
#64997=ADVANCED_FACE('',(#17712),#6645,.T.) ;
#64998=ADVANCED_FACE('',(#17713),#6646,.T.) ;
#64999=ADVANCED_FACE('',(#17714),#63079,.T.) ;
#65000=ADVANCED_FACE('',(#17715),#6647,.T.) ;
#65001=ADVANCED_FACE('',(#17716),#435,.F.) ;
#65002=ADVANCED_FACE('',(#17717),#6648,.F.) ;
#65003=ADVANCED_FACE('',(#17718),#4368,.F.) ;
#65004=ADVANCED_FACE('',(#17719),#6649,.F.) ;
#65005=ADVANCED_FACE('',(#17720),#436,.F.) ;
#65006=ADVANCED_FACE('',(#17721),#437,.F.) ;
#65007=ADVANCED_FACE('',(#17722),#6650,.F.) ;
#65008=ADVANCED_FACE('',(#17723),#4369,.F.) ;
#65009=ADVANCED_FACE('',(#17724),#6651,.F.) ;
#65010=ADVANCED_FACE('',(#17725),#438,.F.) ;
#65011=ADVANCED_FACE('',(#17726),#439,.F.) ;
#65012=ADVANCED_FACE('',(#17727),#6652,.F.) ;
#65013=ADVANCED_FACE('',(#17728),#440,.F.) ;
#65014=ADVANCED_FACE('',(#17729),#6653,.T.) ;
#65015=ADVANCED_FACE('',(#17730),#441,.T.) ;
#65016=ADVANCED_FACE('',(#17731),#442,.F.) ;
#65017=ADVANCED_FACE('',(#17732),#6654,.T.) ;
#65018=ADVANCED_FACE('',(#17733),#6655,.T.) ;
#65019=ADVANCED_FACE('',(#17734),#6656,.F.) ;
#65020=ADVANCED_FACE('',(#17735),#443,.T.) ;
#65021=ADVANCED_FACE('',(#17736),#444,.F.) ;
#65022=ADVANCED_FACE('',(#17737),#6657,.T.) ;
#65023=ADVANCED_FACE('',(#17738),#4370,.T.) ;
#65024=ADVANCED_FACE('',(#17739),#445,.T.) ;
#65025=ADVANCED_FACE('',(#17740),#4371,.T.) ;
#65026=ADVANCED_FACE('',(#17741),#4372,.T.) ;
#65027=ADVANCED_FACE('',(#17742),#6658,.T.) ;
#65028=ADVANCED_FACE('',(#17743),#6659,.T.) ;
#65029=ADVANCED_FACE('',(#17744),#4373,.T.) ;
#65030=ADVANCED_FACE('',(#17745),#4374,.T.) ;
#65031=ADVANCED_FACE('',(#17746),#6660,.T.) ;
#65032=ADVANCED_FACE('',(#17747),#6661,.T.) ;
#65033=ADVANCED_FACE('',(#17748),#4375,.T.) ;
#65034=ADVANCED_FACE('',(#17749),#4376,.T.) ;
#65035=ADVANCED_FACE('',(#17750),#6662,.T.) ;
#65036=ADVANCED_FACE('',(#17751),#6663,.T.) ;
#65037=ADVANCED_FACE('',(#17752),#4377,.T.) ;
#65038=ADVANCED_FACE('',(#17753),#4378,.T.) ;
#65039=ADVANCED_FACE('',(#17754),#6664,.T.) ;
#65040=ADVANCED_FACE('',(#17755),#6665,.T.) ;
#65041=ADVANCED_FACE('',(#17756),#4379,.T.) ;
#65042=ADVANCED_FACE('',(#17757),#6666,.T.) ;
#65043=ADVANCED_FACE('',(#17758),#4380,.T.) ;
#65044=ADVANCED_FACE('',(#17759),#446,.T.) ;
#65045=ADVANCED_FACE('',(#17760),#4381,.T.) ;
#65046=ADVANCED_FACE('',(#17761),#6667,.T.) ;
#65047=ADVANCED_FACE('',(#17762),#447,.T.) ;
#65048=ADVANCED_FACE('',(#17763),#6668,.T.) ;
#65049=ADVANCED_FACE('',(#17764),#448,.T.) ;
#65050=ADVANCED_FACE('',(#17765),#6669,.T.) ;
#65051=ADVANCED_FACE('',(#17766),#449,.F.) ;
#65052=ADVANCED_FACE('',(#17767),#450,.F.) ;
#65053=ADVANCED_FACE('',(#17768),#63080,.T.) ;
#65054=ADVANCED_FACE('',(#17769),#63081,.F.) ;
#65055=ADVANCED_FACE('',(#17770),#6670,.F.) ;
#65056=ADVANCED_FACE('',(#17771),#6671,.F.) ;
#65057=ADVANCED_FACE('',(#17772),#63082,.T.) ;
#65058=ADVANCED_FACE('',(#17773),#6672,.T.) ;
#65059=ADVANCED_FACE('',(#17774),#6673,.F.) ;
#65060=ADVANCED_FACE('',(#17775),#5405,.T.) ;
#65061=ADVANCED_FACE('',(#17776),#5406,.T.) ;
#65062=ADVANCED_FACE('',(#17777),#5407,.T.) ;
#65063=ADVANCED_FACE('',(#17778),#5408,.T.) ;
#65064=ADVANCED_FACE('',(#17779),#5409,.T.) ;
#65065=ADVANCED_FACE('',(#17780),#5410,.T.) ;
#65066=ADVANCED_FACE('',(#17781),#5411,.T.) ;
#65067=ADVANCED_FACE('',(#17782),#5412,.F.) ;
#65068=ADVANCED_FACE('',(#17783),#5413,.T.) ;
#65069=ADVANCED_FACE('',(#17784),#5414,.T.) ;
#65070=ADVANCED_FACE('',(#17785),#5415,.T.) ;
#65071=ADVANCED_FACE('',(#17786),#5416,.T.) ;
#65072=ADVANCED_FACE('',(#17787),#5417,.T.) ;
#65073=ADVANCED_FACE('',(#17788),#5418,.T.) ;
#65074=ADVANCED_FACE('',(#17789),#5419,.T.) ;
#65075=ADVANCED_FACE('',(#17790),#5420,.T.) ;
#65076=ADVANCED_FACE('',(#17791,#5027),#5421,.T.) ;
#65077=ADVANCED_FACE('',(#17792),#5422,.T.) ;
#65078=ADVANCED_FACE('',(#17793),#5423,.T.) ;
#65079=ADVANCED_FACE('',(#17794),#5424,.F.) ;
#65080=ADVANCED_FACE('',(#17795),#5425,.F.) ;
#65081=ADVANCED_FACE('',(#17796),#5426,.T.) ;
#65082=ADVANCED_FACE('',(#17797),#5427,.F.) ;
#65083=ADVANCED_FACE('',(#17798),#5428,.F.) ;
#65084=ADVANCED_FACE('',(#17799),#5429,.F.) ;
#65085=ADVANCED_FACE('',(#17800),#5430,.T.) ;
#65086=ADVANCED_FACE('',(#17801),#5431,.F.) ;
#65087=ADVANCED_FACE('',(#17802,#5028),#5432,.T.) ;
#65088=ADVANCED_FACE('',(#17803),#5433,.T.) ;
#65089=ADVANCED_FACE('',(#17804),#5434,.F.) ;
#65090=ADVANCED_FACE('',(#17805),#5435,.F.) ;
#65091=ADVANCED_FACE('',(#17806),#6674,.T.) ;
#65092=ADVANCED_FACE('',(#17807),#6675,.T.) ;
#65093=ADVANCED_FACE('',(#17808),#5436,.F.) ;
#65094=ADVANCED_FACE('',(#17809),#5437,.F.) ;
#65095=ADVANCED_FACE('',(#17810),#5438,.F.) ;
#65096=ADVANCED_FACE('',(#17811),#5439,.T.) ;
#65097=ADVANCED_FACE('',(#17812),#5440,.F.) ;
#65098=ADVANCED_FACE('',(#17813),#6676,.T.) ;
#65099=ADVANCED_FACE('',(#17814),#5441,.F.) ;
#65100=ADVANCED_FACE('',(#17815),#6677,.T.) ;
#65101=ADVANCED_FACE('',(#17816),#5442,.F.) ;
#65102=ADVANCED_FACE('',(#17817),#5443,.F.) ;
#65103=ADVANCED_FACE('',(#17818),#5444,.F.) ;
#65104=ADVANCED_FACE('',(#17819),#5445,.F.) ;
#65105=ADVANCED_FACE('',(#17820),#5446,.F.) ;
#65106=ADVANCED_FACE('',(#17821),#5447,.F.) ;
#65107=ADVANCED_FACE('',(#17822),#5448,.F.) ;
#65108=ADVANCED_FACE('',(#17823),#5449,.F.) ;
#65109=ADVANCED_FACE('',(#17824),#5450,.F.) ;
#65110=ADVANCED_FACE('',(#17825),#5451,.T.) ;
#65111=ADVANCED_FACE('',(#17826),#5452,.F.) ;
#65112=ADVANCED_FACE('',(#17827),#5453,.F.) ;
#65113=ADVANCED_FACE('',(#17828),#5454,.F.) ;
#65114=ADVANCED_FACE('',(#17829),#5455,.T.) ;
#65115=ADVANCED_FACE('',(#17830),#5456,.F.) ;
#65116=ADVANCED_FACE('',(#17831),#6678,.T.) ;
#65117=ADVANCED_FACE('',(#17832),#5457,.F.) ;
#65118=ADVANCED_FACE('',(#17833),#5458,.F.) ;
#65119=ADVANCED_FACE('',(#17834),#5459,.F.) ;
#65120=ADVANCED_FACE('',(#17835),#5460,.F.) ;
#65121=ADVANCED_FACE('',(#17836),#5461,.F.) ;
#65122=ADVANCED_FACE('',(#17837),#6679,.F.) ;
#65123=ADVANCED_FACE('',(#17838),#5462,.F.) ;
#65124=ADVANCED_FACE('',(#17839),#5463,.F.) ;
#65125=ADVANCED_FACE('',(#17840),#5464,.F.) ;
#65126=ADVANCED_FACE('',(#17841),#5465,.F.) ;
#65127=ADVANCED_FACE('',(#17842),#5466,.F.) ;
#65128=ADVANCED_FACE('',(#17843),#16134,.F.) ;
#65129=ADVANCED_FACE('',(#17844),#5467,.F.) ;
#65130=ADVANCED_FACE('',(#17845),#6680,.F.) ;
#65131=ADVANCED_FACE('',(#17846),#4382,.F.) ;
#65132=ADVANCED_FACE('',(#17847),#6681,.T.) ;
#65133=ADVANCED_FACE('',(#17848),#6682,.F.) ;
#65134=ADVANCED_FACE('',(#17849),#63083,.F.) ;
#65135=ADVANCED_FACE('',(#17850),#63084,.T.) ;
#65136=ADVANCED_FACE('',(#17851),#4383,.F.) ;
#65137=ADVANCED_FACE('',(#17852),#6683,.F.) ;
#65138=ADVANCED_FACE('',(#17853),#6684,.F.) ;
#65139=ADVANCED_FACE('',(#17854),#6685,.T.) ;
#65140=ADVANCED_FACE('',(#17855),#63085,.T.) ;
#65141=ADVANCED_FACE('',(#17856),#6686,.F.) ;
#65142=ADVANCED_FACE('',(#17857),#6687,.F.) ;
#65143=ADVANCED_FACE('',(#17858),#6688,.F.) ;
#65144=ADVANCED_FACE('',(#17859),#4384,.F.) ;
#65145=ADVANCED_FACE('',(#17860),#63086,.T.) ;
#65146=ADVANCED_FACE('',(#17861),#63087,.T.) ;
#65147=ADVANCED_FACE('',(#17862),#4385,.F.) ;
#65148=ADVANCED_FACE('',(#17863),#63088,.F.) ;
#65149=ADVANCED_FACE('',(#17864),#6689,.F.) ;
#65150=ADVANCED_FACE('',(#17865),#63089,.T.) ;
#65151=ADVANCED_FACE('',(#17866),#6690,.T.) ;
#65152=ADVANCED_FACE('',(#17867),#6691,.F.) ;
#65153=ADVANCED_FACE('',(#17868),#4386,.F.) ;
#65154=ADVANCED_FACE('',(#17869),#63090,.T.) ;
#65155=ADVANCED_FACE('',(#17870),#63091,.F.) ;
#65156=ADVANCED_FACE('',(#17871),#6692,.F.) ;
#65157=ADVANCED_FACE('',(#17872),#6693,.F.) ;
#65158=ADVANCED_FACE('',(#17873),#6694,.T.) ;
#65159=ADVANCED_FACE('',(#17874),#6695,.F.) ;
#65160=ADVANCED_FACE('',(#17875),#4387,.F.) ;
#65161=ADVANCED_FACE('',(#17876),#63092,.F.) ;
#65162=ADVANCED_FACE('',(#17877),#6696,.F.) ;
#65163=ADVANCED_FACE('',(#17878),#4388,.T.) ;
#65164=ADVANCED_FACE('',(#17879),#6697,.T.) ;
#65165=ADVANCED_FACE('',(#17880),#6698,.T.) ;
#65166=ADVANCED_FACE('',(#17881),#6699,.T.) ;
#65167=ADVANCED_FACE('',(#17882),#6700,.T.) ;
#65168=ADVANCED_FACE('',(#17883),#6701,.T.) ;
#65169=ADVANCED_FACE('',(#17884),#63093,.F.) ;
#65170=ADVANCED_FACE('',(#17885),#6702,.F.) ;
#65171=ADVANCED_FACE('',(#17886),#4389,.F.) ;
#65172=ADVANCED_FACE('',(#17887),#6703,.T.) ;
#65173=ADVANCED_FACE('',(#17888),#6704,.T.) ;
#65174=ADVANCED_FACE('',(#17889),#6705,.F.) ;
#65175=ADVANCED_FACE('',(#17890),#6706,.T.) ;
#65176=ADVANCED_FACE('',(#17891),#63094,.T.) ;
#65177=ADVANCED_FACE('',(#17892),#6707,.F.) ;
#65178=ADVANCED_FACE('',(#17893),#4390,.T.) ;
#65179=ADVANCED_FACE('',(#17894),#4391,.F.) ;
#65180=ADVANCED_FACE('',(#17895),#6708,.T.) ;
#65181=ADVANCED_FACE('',(#17896),#6709,.T.) ;
#65182=ADVANCED_FACE('',(#17897),#4392,.F.) ;
#65183=ADVANCED_FACE('',(#17898),#6710,.T.) ;
#65184=ADVANCED_FACE('',(#17899),#6711,.F.) ;
#65185=ADVANCED_FACE('',(#17900),#63095,.T.) ;
#65186=ADVANCED_FACE('',(#17901),#63096,.T.) ;
#65187=ADVANCED_FACE('',(#17902),#6712,.F.) ;
#65188=ADVANCED_FACE('',(#17903),#63097,.F.) ;
#65189=ADVANCED_FACE('',(#17904),#4393,.F.) ;
#65190=ADVANCED_FACE('',(#17905),#6713,.T.) ;
#65191=ADVANCED_FACE('',(#17906),#6714,.T.) ;
#65192=ADVANCED_FACE('',(#17907),#6715,.F.) ;
#65193=ADVANCED_FACE('',(#17908),#63098,.T.) ;
#65194=ADVANCED_FACE('',(#17909),#6716,.T.) ;
#65195=ADVANCED_FACE('',(#17910),#6717,.F.) ;
#65196=ADVANCED_FACE('',(#17911),#4394,.F.) ;
#65197=ADVANCED_FACE('',(#17912),#6718,.T.) ;
#65198=ADVANCED_FACE('',(#17913),#6719,.F.) ;
#65199=ADVANCED_FACE('',(#17914),#63099,.F.) ;
#65200=ADVANCED_FACE('',(#17915),#6720,.F.) ;
#65201=ADVANCED_FACE('',(#17916),#6721,.T.) ;
#65202=ADVANCED_FACE('',(#17917),#63100,.T.) ;
#65203=ADVANCED_FACE('',(#17918),#4395,.F.) ;
#65204=ADVANCED_FACE('',(#17919),#63101,.F.) ;
#65205=ADVANCED_FACE('',(#17920),#63102,.T.) ;
#65206=ADVANCED_FACE('',(#17921),#6722,.F.) ;
#65207=ADVANCED_FACE('',(#17922),#6723,.F.) ;
#65208=ADVANCED_FACE('',(#17923),#63103,.F.) ;
#65209=ADVANCED_FACE('',(#17924),#6724,.T.) ;
#65210=ADVANCED_FACE('',(#17925),#6725,.F.) ;
#65211=ADVANCED_FACE('',(#17926),#6726,.F.) ;
#65212=ADVANCED_FACE('',(#17927),#63104,.T.) ;
#65213=ADVANCED_FACE('',(#17928),#4396,.F.) ;
#65214=ADVANCED_FACE('',(#17929),#63105,.F.) ;
#65215=ADVANCED_FACE('',(#17930),#4397,.F.) ;
#65216=ADVANCED_FACE('',(#17931),#6727,.T.) ;
#65217=ADVANCED_FACE('',(#17932),#63106,.F.) ;
#65218=ADVANCED_FACE('',(#17933),#6728,.F.) ;
#65219=ADVANCED_FACE('',(#17934),#63107,.F.) ;
#65220=ADVANCED_FACE('',(#17935),#6729,.F.) ;
#65221=ADVANCED_FACE('',(#17936),#6730,.T.) ;
#65222=ADVANCED_FACE('',(#17937),#451,.F.) ;
#65223=ADVANCED_FACE('',(#17938),#4398,.F.) ;
#65224=ADVANCED_FACE('',(#17939),#4399,.F.) ;
#65225=ADVANCED_FACE('',(#17940),#63108,.T.) ;
#65226=ADVANCED_FACE('',(#17941),#63109,.F.) ;
#65227=ADVANCED_FACE('',(#17942),#6731,.F.) ;
#65228=ADVANCED_FACE('',(#17943),#63110,.T.) ;
#65229=ADVANCED_FACE('',(#17944),#452,.F.) ;
#65230=ADVANCED_FACE('',(#17945),#63111,.T.) ;
#65231=ADVANCED_FACE('',(#17946),#6732,.T.) ;
#65232=ADVANCED_FACE('',(#17947),#63112,.T.) ;
#65233=ADVANCED_FACE('',(#17948),#6733,.T.) ;
#65234=ADVANCED_FACE('',(#17949),#63113,.T.) ;
#65235=ADVANCED_FACE('',(#17950),#6734,.T.) ;
#65236=ADVANCED_FACE('',(#17951),#63114,.T.) ;
#65237=ADVANCED_FACE('',(#17952),#6735,.T.) ;
#65238=ADVANCED_FACE('',(#17953),#4400,.T.) ;
#65239=ADVANCED_FACE('',(#17954),#6736,.T.) ;
#65240=ADVANCED_FACE('',(#17955),#6737,.T.) ;
#65241=ADVANCED_FACE('',(#17956),#6738,.T.) ;
#65242=ADVANCED_FACE('',(#17957),#6739,.T.) ;
#65243=ADVANCED_FACE('',(#17958),#6740,.T.) ;
#65244=ADVANCED_FACE('',(#17959),#4401,.T.) ;
#65245=ADVANCED_FACE('',(#17960),#4402,.T.) ;
#65246=ADVANCED_FACE('',(#17961),#6741,.T.) ;
#65247=ADVANCED_FACE('',(#17962),#6742,.T.) ;
#65248=ADVANCED_FACE('',(#17963),#4403,.T.) ;
#65249=ADVANCED_FACE('',(#17964),#6743,.T.) ;
#65250=ADVANCED_FACE('',(#17965),#6744,.T.) ;
#65251=ADVANCED_FACE('',(#17966),#63115,.T.) ;
#65252=ADVANCED_FACE('',(#17967),#6745,.T.) ;
#65253=ADVANCED_FACE('',(#17968),#6746,.T.) ;
#65254=ADVANCED_FACE('',(#17969),#6747,.T.) ;
#65255=ADVANCED_FACE('',(#17970),#6748,.T.) ;
#65256=ADVANCED_FACE('',(#17971),#6749,.T.) ;
#65257=ADVANCED_FACE('',(#17972),#4404,.T.) ;
#65258=ADVANCED_FACE('',(#17973),#6750,.T.) ;
#65259=ADVANCED_FACE('',(#17974),#6751,.T.) ;
#65260=ADVANCED_FACE('',(#17975),#4405,.T.) ;
#65261=ADVANCED_FACE('',(#17976),#6752,.T.) ;
#65262=ADVANCED_FACE('',(#17977),#6753,.T.) ;
#65263=ADVANCED_FACE('',(#17978),#6754,.T.) ;
#65264=ADVANCED_FACE('',(#17979),#6755,.T.) ;
#65265=ADVANCED_FACE('',(#17980),#4406,.T.) ;
#65266=ADVANCED_FACE('',(#17981),#4407,.T.) ;
#65267=ADVANCED_FACE('',(#17982),#6756,.T.) ;
#65268=ADVANCED_FACE('',(#17983),#6757,.T.) ;
#65269=ADVANCED_FACE('',(#17984),#6758,.T.) ;
#65270=ADVANCED_FACE('',(#17985),#4408,.T.) ;
#65271=ADVANCED_FACE('',(#17986),#6759,.T.) ;
#65272=ADVANCED_FACE('',(#17987),#6760,.T.) ;
#65273=ADVANCED_FACE('',(#17988),#4409,.T.) ;
#65274=ADVANCED_FACE('',(#17989),#6761,.T.) ;
#65275=ADVANCED_FACE('',(#17990),#6762,.T.) ;
#65276=ADVANCED_FACE('',(#17991),#6763,.T.) ;
#65277=ADVANCED_FACE('',(#17992),#4410,.T.) ;
#65278=ADVANCED_FACE('',(#17993),#6764,.T.) ;
#65279=ADVANCED_FACE('',(#17994),#6765,.T.) ;
#65280=ADVANCED_FACE('',(#17995),#4411,.T.) ;
#65281=ADVANCED_FACE('',(#17996),#6766,.T.) ;
#65282=ADVANCED_FACE('',(#17997),#6767,.F.) ;
#65283=ADVANCED_FACE('',(#17998),#6768,.T.) ;
#65284=ADVANCED_FACE('',(#17999),#6769,.F.) ;
#65285=ADVANCED_FACE('',(#18000),#6770,.T.) ;
#65286=ADVANCED_FACE('',(#18001),#6771,.T.) ;
#65287=ADVANCED_FACE('',(#18002),#6772,.T.) ;
#65288=ADVANCED_FACE('',(#18003),#63116,.T.) ;
#65289=ADVANCED_FACE('',(#18004),#6773,.T.) ;
#65290=ADVANCED_FACE('',(#18005),#453,.F.) ;
#65291=ADVANCED_FACE('',(#18006),#6774,.F.) ;
#65292=ADVANCED_FACE('',(#18007),#4412,.F.) ;
#65293=ADVANCED_FACE('',(#18008),#6775,.F.) ;
#65294=ADVANCED_FACE('',(#18009),#454,.F.) ;
#65295=ADVANCED_FACE('',(#18010),#455,.F.) ;
#65296=ADVANCED_FACE('',(#18011),#6776,.F.) ;
#65297=ADVANCED_FACE('',(#18012),#4413,.F.) ;
#65298=ADVANCED_FACE('',(#18013),#6777,.F.) ;
#65299=ADVANCED_FACE('',(#18014),#456,.F.) ;
#65300=ADVANCED_FACE('',(#18015),#457,.F.) ;
#65301=ADVANCED_FACE('',(#18016),#6778,.F.) ;
#65302=ADVANCED_FACE('',(#18017),#458,.F.) ;
#65303=ADVANCED_FACE('',(#18018),#6779,.T.) ;
#65304=ADVANCED_FACE('',(#18019),#459,.T.) ;
#65305=ADVANCED_FACE('',(#18020),#460,.F.) ;
#65306=ADVANCED_FACE('',(#18021),#6780,.T.) ;
#65307=ADVANCED_FACE('',(#18022),#6781,.T.) ;
#65308=ADVANCED_FACE('',(#18023),#6782,.F.) ;
#65309=ADVANCED_FACE('',(#18024),#461,.T.) ;
#65310=ADVANCED_FACE('',(#18025),#462,.F.) ;
#65311=ADVANCED_FACE('',(#18026),#6783,.T.) ;
#65312=ADVANCED_FACE('',(#18027),#4414,.T.) ;
#65313=ADVANCED_FACE('',(#18028),#463,.T.) ;
#65314=ADVANCED_FACE('',(#18029),#4415,.T.) ;
#65315=ADVANCED_FACE('',(#18030),#4416,.T.) ;
#65316=ADVANCED_FACE('',(#18031),#6784,.T.) ;
#65317=ADVANCED_FACE('',(#18032),#6785,.T.) ;
#65318=ADVANCED_FACE('',(#18033),#4417,.T.) ;
#65319=ADVANCED_FACE('',(#18034),#4418,.T.) ;
#65320=ADVANCED_FACE('',(#18035),#6786,.T.) ;
#65321=ADVANCED_FACE('',(#18036),#6787,.T.) ;
#65322=ADVANCED_FACE('',(#18037),#4419,.T.) ;
#65323=ADVANCED_FACE('',(#18038),#4420,.T.) ;
#65324=ADVANCED_FACE('',(#18039),#6788,.T.) ;
#65325=ADVANCED_FACE('',(#18040),#6789,.T.) ;
#65326=ADVANCED_FACE('',(#18041),#4421,.T.) ;
#65327=ADVANCED_FACE('',(#18042),#4422,.T.) ;
#65328=ADVANCED_FACE('',(#18043),#6790,.T.) ;
#65329=ADVANCED_FACE('',(#18044),#6791,.T.) ;
#65330=ADVANCED_FACE('',(#18045),#4423,.T.) ;
#65331=ADVANCED_FACE('',(#18046),#6792,.T.) ;
#65332=ADVANCED_FACE('',(#18047),#4424,.T.) ;
#65333=ADVANCED_FACE('',(#18048),#464,.T.) ;
#65334=ADVANCED_FACE('',(#18049),#4425,.T.) ;
#65335=ADVANCED_FACE('',(#18050),#6793,.T.) ;
#65336=ADVANCED_FACE('',(#18051),#465,.T.) ;
#65337=ADVANCED_FACE('',(#18052),#6794,.T.) ;
#65338=ADVANCED_FACE('',(#18053),#466,.T.) ;
#65339=ADVANCED_FACE('',(#18054),#6795,.T.) ;
#67687=CLOSED_SHELL('',(#63895,#63896,#63897,#63898,#63899,#63900,#63901,
#63902,#63903,#63904,#63905,#63906,#63907,#63908,#63909,#63910,#63911,#63912,
#63913,#63914,#63915,#63916,#63917,#63918,#63919,#63920,#63921,#63922,#63923,
#63924,#63925,#63926,#63927,#63928,#63929,#63930,#63931,#63932,#63933,#63934,
#63935,#63936,#63937,#63938,#63939,#63940,#63941,#63942,#63943,#63944,#63945,
#63946,#63947,#63948,#63949,#63950,#63951,#63952,#63953,#63954,#63955,#63956,
#63957,#63958,#63959,#63960,#63961,#63962,#63963,#63964,#63965,#63966,#63967,
#63968,#63969,#63970,#63971,#63972,#63973,#63974,#63975,#63976,#63977,#63978,
#63979,#63980,#63981,#63982,#63983,#63984,#63985,#63986,#63987,#63988,#63989,
#63990,#63991,#63992,#63993,#63994,#63995,#63996,#63997,#63998,#63999,#64000,
#64001,#64002,#64003,#64004,#64005,#64006,#64007,#64008,#64009,#64010,#64011,
#64012,#64013,#64014,#64015,#64016,#64017,#64018,#64019,#64020,#64021,#64022,
#64023,#64024,#64025,#64026,#64027,#64028,#64029,#64030,#64031,#64032,#64033,
#64034,#64035,#64036,#64037,#64038,#64039,#64040,#64041,#64042,#64043,#64044,
#64045,#64046,#64047,#64048,#64049,#64050,#64051,#64052,#64053,#64054,#64055,
#64056,#64057,#64058,#64059,#64060,#64061,#64062,#64063,#64064,#64065,#64066,
#64067,#64068,#64069,#64070,#64071,#64072,#64073,#64074,#64075,#64076,#64077,
#64078,#64079,#64080,#64081,#64082,#64083,#64084,#64085,#64086,#64087,#64088,
#64089,#64090,#64091,#64092,#64093,#64094,#64095,#64096,#64097,#64098,#64099,
#64100,#64101,#64102,#64103,#64104,#64105,#64106,#64107,#64108,#64109,#64110,
#64111,#64112,#64113,#64114,#64115,#64116,#64117,#64118,#64119,#64120,#64121,
#64122,#64123,#64124,#64125,#64126,#64127,#64128,#64129,#64130,#64131,#64132,
#64133,#64134,#64135,#64136,#64137,#64138,#64139,#64140,#64141,#64142,#64143,
#64144,#64145,#64146,#64147,#64148,#64149,#64150,#64151,#64152,#64153,#64154,
#64155,#64156,#64157,#64158,#64159,#64160,#64161,#64162,#64163,#64164,#64165,
#64166,#64167,#64168,#64169,#64170,#64171,#64172,#64173,#64174,#64175,#64176,
#64177,#64178,#64179,#64180,#64181,#64182,#64183)) ;
#67688=CLOSED_SHELL('',(#64184,#64185,#64186,#64187,#64188,#64189,#64190,
#64191,#64192,#64193,#64194,#64195,#64196,#64197,#64198,#64199,#64200,#64201,
#64202,#64203,#64204,#64205,#64206,#64207,#64208,#64209,#64210,#64211,#64212,
#64213,#64214,#64215,#64216,#64217,#64218,#64219,#64220,#64221,#64222,#64223,
#64224,#64225,#64226,#64227,#64228,#64229,#64230,#64231,#64232,#64233,#64234,
#64235,#64236,#64237,#64238,#64239,#64240,#64241,#64242,#64243,#64244,#64245,
#64246,#64247,#64248,#64249,#64250,#64251,#64252,#64253,#64254,#64255,#64256,
#64257,#64258,#64259,#64260,#64261,#64262,#64263,#64264,#64265,#64266,#64267,
#64268,#64269,#64270,#64271,#64272,#64273,#64274,#64275,#64276,#64277,#64278,
#64279,#64280,#64281,#64282,#64283,#64284,#64285,#64286,#64287,#64288,#64289,
#64290,#64291,#64292,#64293,#64294,#64295,#64296,#64297,#64298,#64299,#64300,
#64301,#64302,#64303,#64304,#64305,#64306,#64307,#64308,#64309,#64310,#64311,
#64312,#64313,#64314,#64315,#64316,#64317,#64318,#64319,#64320,#64321,#64322,
#64323,#64324,#64325,#64326,#64327,#64328,#64329,#64330,#64331,#64332,#64333,
#64334,#64335,#64336,#64337,#64338,#64339,#64340,#64341,#64342,#64343,#64344,
#64345,#64346,#64347,#64348,#64349,#64350,#64351,#64352,#64353,#64354,#64355,
#64356,#64357,#64358,#64359,#64360,#64361,#64362,#64363,#64364,#64365,#64366,
#64367,#64368,#64369,#64370,#64371,#64372,#64373,#64374,#64375,#64376,#64377,
#64378,#64379,#64380,#64381,#64382,#64383,#64384,#64385,#64386,#64387,#64388,
#64389,#64390,#64391,#64392,#64393,#64394,#64395,#64396,#64397,#64398,#64399,
#64400,#64401,#64402,#64403,#64404,#64405,#64406,#64407,#64408,#64409,#64410,
#64411,#64412,#64413,#64414,#64415,#64416,#64417,#64418,#64419,#64420,#64421,
#64422,#64423,#64424,#64425,#64426,#64427,#64428,#64429,#64430,#64431,#64432,
#64433,#64434,#64435,#64436,#64437,#64438,#64439,#64440,#64441,#64442,#64443,
#64444,#64445,#64446,#64447,#64448,#64449,#64450,#64451,#64452,#64453,#64454,
#64455,#64456,#64457,#64458,#64459,#64460,#64461,#64462,#64463,#64464,#64465,
#64466,#64467,#64468,#64469,#64470,#64471,#64472)) ;
#67689=CLOSED_SHELL('',(#64473,#64474,#64475,#64476,#64477,#64478,#64479,
#64480,#64481,#64482,#64483,#64484,#64485,#64486,#64487,#64488,#64489,#64490,
#64491,#64492,#64493,#64494,#64495,#64496,#64497,#64498,#64499,#64500,#64501,
#64502,#64503,#64504,#64505,#64506,#64507,#64508,#64509,#64510,#64511,#64512,
#64513,#64514,#64515,#64516,#64517,#64518,#64519,#64520,#64521,#64522,#64523,
#64524,#64525,#64526,#64527,#64528,#64529,#64530,#64531,#64532,#64533,#64534,
#64535,#64536,#64537,#64538,#64539,#64540,#64541,#64542,#64543,#64544,#64545,
#64546,#64547,#64548,#64549,#64550,#64551,#64552,#64553,#64554,#64555,#64556,
#64557,#64558,#64559,#64560,#64561,#64562,#64563,#64564,#64565,#64566,#64567,
#64568,#64569,#64570,#64571,#64572,#64573,#64574,#64575,#64576,#64577,#64578,
#64579,#64580,#64581,#64582,#64583,#64584,#64585,#64586,#64587,#64588,#64589,
#64590,#64591,#64592,#64593,#64594,#64595,#64596,#64597,#64598,#64599,#64600,
#64601,#64602,#64603,#64604,#64605,#64606,#64607,#64608,#64609,#64610,#64611,
#64612,#64613,#64614,#64615,#64616,#64617,#64618,#64619,#64620,#64621,#64622,
#64623,#64624,#64625,#64626,#64627,#64628,#64629,#64630,#64631,#64632,#64633,
#64634,#64635,#64636,#64637,#64638,#64639,#64640,#64641,#64642,#64643,#64644,
#64645,#64646,#64647,#64648,#64649,#64650,#64651,#64652,#64653,#64654,#64655,
#64656,#64657,#64658,#64659,#64660,#64661,#64662,#64663,#64664,#64665,#64666,
#64667,#64668,#64669,#64670,#64671,#64672,#64673,#64674,#64675,#64676,#64677,
#64678,#64679,#64680,#64681,#64682,#64683,#64684,#64685,#64686,#64687,#64688,
#64689,#64690,#64691,#64692,#64693,#64694,#64695,#64696,#64697,#64698,#64699,
#64700,#64701,#64702,#64703,#64704,#64705,#64706,#64707,#64708,#64709,#64710,
#64711,#64712,#64713,#64714,#64715,#64716,#64717,#64718,#64719,#64720,#64721,
#64722,#64723,#64724,#64725,#64726,#64727,#64728,#64729,#64730,#64731,#64732,
#64733,#64734,#64735,#64736,#64737,#64738,#64739,#64740,#64741,#64742,#64743,
#64744,#64745,#64746,#64747,#64748,#64749,#64750,#64751,#64752,#64753,#64754,
#64755,#64756,#64757,#64758,#64759,#64760,#64761)) ;
#67690=CLOSED_SHELL('',(#64762,#64763,#64764,#64765,#64766,#64767,#64768,
#64769,#64770,#64771,#64772,#64773,#64774,#64775,#64776,#64777,#64778,#64779,
#64780,#64781,#64782,#64783,#64784,#64785,#64786,#64787,#64788,#64789,#64790,
#64791,#64792,#64793,#64794,#64795,#64796,#64797,#64798,#64799,#64800,#64801,
#64802,#64803,#64804,#64805,#64806,#64807,#64808,#64809,#64810,#64811,#64812,
#64813,#64814,#64815,#64816,#64817,#64818,#64819,#64820,#64821,#64822,#64823,
#64824,#64825,#64826,#64827,#64828,#64829,#64830,#64831,#64832,#64833,#64834,
#64835,#64836,#64837,#64838,#64839,#64840,#64841,#64842,#64843,#64844,#64845,
#64846,#64847,#64848,#64849,#64850,#64851,#64852,#64853,#64854,#64855,#64856,
#64857,#64858,#64859,#64860,#64861,#64862,#64863,#64864,#64865,#64866,#64867,
#64868,#64869,#64870,#64871,#64872,#64873,#64874,#64875,#64876,#64877,#64878,
#64879,#64880,#64881,#64882,#64883,#64884,#64885,#64886,#64887,#64888,#64889,
#64890,#64891,#64892,#64893,#64894,#64895,#64896,#64897,#64898,#64899,#64900,
#64901,#64902,#64903,#64904,#64905,#64906,#64907,#64908,#64909,#64910,#64911,
#64912,#64913,#64914,#64915,#64916,#64917,#64918,#64919,#64920,#64921,#64922,
#64923,#64924,#64925,#64926,#64927,#64928,#64929,#64930,#64931,#64932,#64933,
#64934,#64935,#64936,#64937,#64938,#64939,#64940,#64941,#64942,#64943,#64944,
#64945,#64946,#64947,#64948,#64949,#64950,#64951,#64952,#64953,#64954,#64955,
#64956,#64957,#64958,#64959,#64960,#64961,#64962,#64963,#64964,#64965,#64966,
#64967,#64968,#64969,#64970,#64971,#64972,#64973,#64974,#64975,#64976,#64977,
#64978,#64979,#64980,#64981,#64982,#64983,#64984,#64985,#64986,#64987,#64988,
#64989,#64990,#64991,#64992,#64993,#64994,#64995,#64996,#64997,#64998,#64999,
#65000,#65001,#65002,#65003,#65004,#65005,#65006,#65007,#65008,#65009,#65010,
#65011,#65012,#65013,#65014,#65015,#65016,#65017,#65018,#65019,#65020,#65021,
#65022,#65023,#65024,#65025,#65026,#65027,#65028,#65029,#65030,#65031,#65032,
#65033,#65034,#65035,#65036,#65037,#65038,#65039,#65040,#65041,#65042,#65043,
#65044,#65045,#65046,#65047,#65048,#65049,#65050)) ;
#67691=CLOSED_SHELL('',(#65051,#65052,#65053,#65054,#65055,#65056,#65057,
#65058,#65059,#65060,#65061,#65062,#65063,#65064,#65065,#65066,#65067,#65068,
#65069,#65070,#65071,#65072,#65073,#65074,#65075,#65076,#65077,#65078,#65079,
#65080,#65081,#65082,#65083,#65084,#65085,#65086,#65087,#65088,#65089,#65090,
#65091,#65092,#65093,#65094,#65095,#65096,#65097,#65098,#65099,#65100,#65101,
#65102,#65103,#65104,#65105,#65106,#65107,#65108,#65109,#65110,#65111,#65112,
#65113,#65114,#65115,#65116,#65117,#65118,#65119,#65120,#65121,#65122,#65123,
#65124,#65125,#65126,#65127,#65128,#65129,#65130,#65131,#65132,#65133,#65134,
#65135,#65136,#65137,#65138,#65139,#65140,#65141,#65142,#65143,#65144,#65145,
#65146,#65147,#65148,#65149,#65150,#65151,#65152,#65153,#65154,#65155,#65156,
#65157,#65158,#65159,#65160,#65161,#65162,#65163,#65164,#65165,#65166,#65167,
#65168,#65169,#65170,#65171,#65172,#65173,#65174,#65175,#65176,#65177,#65178,
#65179,#65180,#65181,#65182,#65183,#65184,#65185,#65186,#65187,#65188,#65189,
#65190,#65191,#65192,#65193,#65194,#65195,#65196,#65197,#65198,#65199,#65200,
#65201,#65202,#65203,#65204,#65205,#65206,#65207,#65208,#65209,#65210,#65211,
#65212,#65213,#65214,#65215,#65216,#65217,#65218,#65219,#65220,#65221,#65222,
#65223,#65224,#65225,#65226,#65227,#65228,#65229,#65230,#65231,#65232,#65233,
#65234,#65235,#65236,#65237,#65238,#65239,#65240,#65241,#65242,#65243,#65244,
#65245,#65246,#65247,#65248,#65249,#65250,#65251,#65252,#65253,#65254,#65255,
#65256,#65257,#65258,#65259,#65260,#65261,#65262,#65263,#65264,#65265,#65266,
#65267,#65268,#65269,#65270,#65271,#65272,#65273,#65274,#65275,#65276,#65277,
#65278,#65279,#65280,#65281,#65282,#65283,#65284,#65285,#65286,#65287,#65288,
#65289,#65290,#65291,#65292,#65293,#65294,#65295,#65296,#65297,#65298,#65299,
#65300,#65301,#65302,#65303,#65304,#65305,#65306,#65307,#65308,#65309,#65310,
#65311,#65312,#65313,#65314,#65315,#65316,#65317,#65318,#65319,#65320,#65321,
#65322,#65323,#65324,#65325,#65326,#65327,#65328,#65329,#65330,#65331,#65332,
#65333,#65334,#65335,#65336,#65337,#65338,#65339)) ;
#68778=AXIS2_PLACEMENT_3D('',#101184,#79337,#79338) ;
#68779=AXIS2_PLACEMENT_3D('',#101210,#79339,#79340) ;
#68780=AXIS2_PLACEMENT_3D('',#101212,#79341,#79342) ;
#68781=AXIS2_PLACEMENT_3D('',#101214,#79343,#79344) ;
#68782=AXIS2_PLACEMENT_3D('',#101253,#79345,#79346) ;
#68783=AXIS2_PLACEMENT_3D('',#101255,#79347,#79348) ;
#68784=AXIS2_PLACEMENT_3D('',#101257,#79349,#79350) ;
#68785=AXIS2_PLACEMENT_3D('',#101258,#79351,#79352) ;
#68786=AXIS2_PLACEMENT_3D('',#101259,#79353,#79354) ;
#68787=AXIS2_PLACEMENT_3D('',#101261,#79355,#79356) ;
#68788=AXIS2_PLACEMENT_3D('',#101263,#79357,#79358) ;
#68789=AXIS2_PLACEMENT_3D('',#101264,#79359,#79360) ;
#68790=AXIS2_PLACEMENT_3D('',#101265,#79361,#79362) ;
#68791=AXIS2_PLACEMENT_3D('',#101267,#79363,#79364) ;
#68792=AXIS2_PLACEMENT_3D('',#101269,#79365,#79366) ;
#68793=AXIS2_PLACEMENT_3D('',#101270,#79367,#79368) ;
#68794=AXIS2_PLACEMENT_3D('',#101271,#79369,#79370) ;
#68795=AXIS2_PLACEMENT_3D('',#101274,#79371,#79372) ;
#68796=AXIS2_PLACEMENT_3D('',#101278,#79374,#79375) ;
#68797=AXIS2_PLACEMENT_3D('',#101280,#79376,#79377) ;
#68798=AXIS2_PLACEMENT_3D('',#101282,#79379,#79380) ;
#68799=AXIS2_PLACEMENT_3D('',#101285,#79381,#79382) ;
#68800=AXIS2_PLACEMENT_3D('',#101289,#79384,#79385) ;
#68801=AXIS2_PLACEMENT_3D('',#101291,#79387,#79388) ;
#68802=AXIS2_PLACEMENT_3D('',#101294,#79389,#79390) ;
#68803=AXIS2_PLACEMENT_3D('',#101296,#79391,#79392) ;
#68804=AXIS2_PLACEMENT_3D('',#101298,#79393,#79394) ;
#68805=AXIS2_PLACEMENT_3D('',#101299,#79395,#79396) ;
#68806=AXIS2_PLACEMENT_3D('',#101300,#79397,#79398) ;
#68807=AXIS2_PLACEMENT_3D('',#101302,#79400,#79401) ;
#68808=AXIS2_PLACEMENT_3D('',#101305,#79403,#79404) ;
#68809=AXIS2_PLACEMENT_3D('',#101314,#79405,#79406) ;
#68810=AXIS2_PLACEMENT_3D('',#101322,#79407,#79408) ;
#68811=AXIS2_PLACEMENT_3D('',#101324,#79410,#79411) ;
#68812=AXIS2_PLACEMENT_3D('',#101340,#79415,#79416) ;
#68813=AXIS2_PLACEMENT_3D('',#101342,#79418,#79419) ;
#68814=AXIS2_PLACEMENT_3D('',#101391,#79424,#79425) ;
#68815=AXIS2_PLACEMENT_3D('',#101400,#79430,#79431) ;
#68816=AXIS2_PLACEMENT_3D('',#101430,#79436,#79437) ;
#68817=AXIS2_PLACEMENT_3D('',#101439,#79442,#79443) ;
#68818=AXIS2_PLACEMENT_3D('',#101448,#79448,#79449) ;
#68819=AXIS2_PLACEMENT_3D('',#101459,#79454,#79455) ;
#68820=AXIS2_PLACEMENT_3D('',#101461,#79457,#79458) ;
#68821=AXIS2_PLACEMENT_3D('',#101465,#79460,#79461) ;
#68822=AXIS2_PLACEMENT_3D('',#101466,#79462,#79463) ;
#68823=AXIS2_PLACEMENT_3D('',#101467,#79464,#79465) ;
#68824=AXIS2_PLACEMENT_3D('',#101469,#79466,#79467) ;
#68825=AXIS2_PLACEMENT_3D('',#101473,#79469,#79470) ;
#68826=AXIS2_PLACEMENT_3D('',#101477,#79472,#79473) ;
#68827=AXIS2_PLACEMENT_3D('',#101481,#79475,#79476) ;
#68828=AXIS2_PLACEMENT_3D('',#101485,#79478,#79479) ;
#68829=AXIS2_PLACEMENT_3D('',#101489,#79481,#79482) ;
#68830=AXIS2_PLACEMENT_3D('',#101492,#79484,#79485) ;
#68831=AXIS2_PLACEMENT_3D('',#101494,#79486,#79487) ;
#68832=AXIS2_PLACEMENT_3D('',#101497,#79489,#79490) ;
#68833=AXIS2_PLACEMENT_3D('',#101499,#79491,#79492) ;
#68834=AXIS2_PLACEMENT_3D('',#101505,#79495,#79496) ;
#68835=AXIS2_PLACEMENT_3D('',#101509,#79498,#79499) ;
#68836=AXIS2_PLACEMENT_3D('',#101512,#79501,#79502) ;
#68837=AXIS2_PLACEMENT_3D('',#101513,#79503,#79504) ;
#68838=AXIS2_PLACEMENT_3D('',#101518,#79506,#79507) ;
#68839=AXIS2_PLACEMENT_3D('',#101522,#79509,#79510) ;
#68840=AXIS2_PLACEMENT_3D('',#101526,#79512,#79513) ;
#68841=AXIS2_PLACEMENT_3D('',#101530,#79515,#79516) ;
#68842=AXIS2_PLACEMENT_3D('',#101535,#79519,#79520) ;
#68843=AXIS2_PLACEMENT_3D('',#101537,#79521,#79522) ;
#68844=AXIS2_PLACEMENT_3D('',#101540,#79524,#79525) ;
#68845=AXIS2_PLACEMENT_3D('',#101542,#79526,#79527) ;
#68846=AXIS2_PLACEMENT_3D('',#101546,#79529,#79530) ;
#68847=AXIS2_PLACEMENT_3D('',#101550,#79532,#79533) ;
#68848=AXIS2_PLACEMENT_3D('',#101554,#79535,#79536) ;
#68849=AXIS2_PLACEMENT_3D('',#101558,#79538,#79539) ;
#68850=AXIS2_PLACEMENT_3D('',#101562,#79541,#79542) ;
#68851=AXIS2_PLACEMENT_3D('',#101566,#79544,#79545) ;
#68852=AXIS2_PLACEMENT_3D('',#101570,#79547,#79548) ;
#68853=AXIS2_PLACEMENT_3D('',#101573,#79550,#79551) ;
#68854=AXIS2_PLACEMENT_3D('',#101574,#79552,#79553) ;
#68855=AXIS2_PLACEMENT_3D('',#101577,#79556,#79557) ;
#68856=AXIS2_PLACEMENT_3D('',#101580,#79560,#79561) ;
#68857=AXIS2_PLACEMENT_3D('',#101669,#79566,#79567) ;
#68858=AXIS2_PLACEMENT_3D('',#101680,#79568,#79569) ;
#68859=AXIS2_PLACEMENT_3D('',#101685,#79573,#79574) ;
#68860=AXIS2_PLACEMENT_3D('',#101691,#79578,#79579) ;
#68861=AXIS2_PLACEMENT_3D('',#101711,#79583,#79584) ;
#68862=AXIS2_PLACEMENT_3D('',#101810,#79590,#79591) ;
#68863=AXIS2_PLACEMENT_3D('',#101814,#79593,#79594) ;
#68864=AXIS2_PLACEMENT_3D('',#101818,#79597,#79598) ;
#68865=AXIS2_PLACEMENT_3D('',#101821,#79599,#79600) ;
#68866=AXIS2_PLACEMENT_3D('',#101826,#79603,#79604) ;
#68867=AXIS2_PLACEMENT_3D('',#101828,#79605,#79606) ;
#68868=AXIS2_PLACEMENT_3D('',#101830,#79607,#79608) ;
#68869=AXIS2_PLACEMENT_3D('',#101838,#79612,#79613) ;
#68870=AXIS2_PLACEMENT_3D('',#101840,#79614,#79615) ;
#68871=AXIS2_PLACEMENT_3D('',#101842,#79616,#79617) ;
#68872=AXIS2_PLACEMENT_3D('',#101847,#79620,#79621) ;
#68873=AXIS2_PLACEMENT_3D('',#101849,#79622,#79623) ;
#68874=AXIS2_PLACEMENT_3D('',#101851,#79624,#79625) ;
#68875=AXIS2_PLACEMENT_3D('',#101855,#79627,#79628) ;
#68876=AXIS2_PLACEMENT_3D('',#101859,#79630,#79631) ;
#68877=AXIS2_PLACEMENT_3D('',#101860,#79632,#79633) ;
#68878=AXIS2_PLACEMENT_3D('',#101861,#79634,#79635) ;
#68879=AXIS2_PLACEMENT_3D('',#101864,#79636,#79637) ;
#68880=AXIS2_PLACEMENT_3D('',#101874,#79643,#79644) ;
#68881=AXIS2_PLACEMENT_3D('',#101876,#79646,#79647) ;
#68882=AXIS2_PLACEMENT_3D('',#101879,#79648,#79649) ;
#68883=AXIS2_PLACEMENT_3D('',#101885,#79653,#79654) ;
#68884=AXIS2_PLACEMENT_3D('',#101887,#79656,#79657) ;
#68885=AXIS2_PLACEMENT_3D('',#101893,#79660,#79661) ;
#68886=AXIS2_PLACEMENT_3D('',#101894,#79662,#79663) ;
#68887=AXIS2_PLACEMENT_3D('',#101897,#79664,#79665) ;
#68888=AXIS2_PLACEMENT_3D('',#101901,#79668,#79669) ;
#68889=AXIS2_PLACEMENT_3D('',#101918,#79678,#79679) ;
#68890=AXIS2_PLACEMENT_3D('',#101927,#79684,#79685) ;
#68891=AXIS2_PLACEMENT_3D('',#101936,#79690,#79691) ;
#68892=AXIS2_PLACEMENT_3D('',#101945,#79696,#79697) ;
#68893=AXIS2_PLACEMENT_3D('',#101972,#79702,#79703) ;
#68894=AXIS2_PLACEMENT_3D('',#101989,#79712,#79713) ;
#68895=AXIS2_PLACEMENT_3D('',#101994,#79715,#79716) ;
#68896=AXIS2_PLACEMENT_3D('',#101998,#79718,#79719) ;
#68897=AXIS2_PLACEMENT_3D('',#102002,#79721,#79722) ;
#68898=AXIS2_PLACEMENT_3D('',#102005,#79724,#79725) ;
#68899=AXIS2_PLACEMENT_3D('',#102006,#79726,#79727) ;
#68900=AXIS2_PLACEMENT_3D('',#102009,#79728,#79729) ;
#68901=AXIS2_PLACEMENT_3D('',#102014,#79732,#79733) ;
#68902=AXIS2_PLACEMENT_3D('',#102017,#79735,#79736) ;
#68903=AXIS2_PLACEMENT_3D('',#102018,#79737,#79738) ;
#68904=AXIS2_PLACEMENT_3D('',#102024,#79742,#79743) ;
#68905=AXIS2_PLACEMENT_3D('',#102030,#79747,#79748) ;
#68906=AXIS2_PLACEMENT_3D('',#102033,#79749,#79750) ;
#68907=AXIS2_PLACEMENT_3D('',#102037,#79752,#79753) ;
#68908=AXIS2_PLACEMENT_3D('',#102039,#79755,#79756) ;
#68909=AXIS2_PLACEMENT_3D('',#102042,#79757,#79758) ;
#68910=AXIS2_PLACEMENT_3D('',#102046,#79760,#79761) ;
#68911=AXIS2_PLACEMENT_3D('',#102048,#79763,#79764) ;
#68912=AXIS2_PLACEMENT_3D('',#102054,#79768,#79769) ;
#68913=AXIS2_PLACEMENT_3D('',#102060,#79773,#79774) ;
#68914=AXIS2_PLACEMENT_3D('',#102063,#79775,#79776) ;
#68915=AXIS2_PLACEMENT_3D('',#102068,#79779,#79780) ;
#68916=AXIS2_PLACEMENT_3D('',#102070,#79781,#79782) ;
#68917=AXIS2_PLACEMENT_3D('',#102072,#79784,#79785) ;
#68918=AXIS2_PLACEMENT_3D('',#102075,#79786,#79787) ;
#68919=AXIS2_PLACEMENT_3D('',#102080,#79791,#79792) ;
#68920=AXIS2_PLACEMENT_3D('',#102086,#79796,#79797) ;
#68921=AXIS2_PLACEMENT_3D('',#102089,#79798,#79799) ;
#68922=AXIS2_PLACEMENT_3D('',#102093,#79801,#79802) ;
#68923=AXIS2_PLACEMENT_3D('',#102095,#79804,#79805) ;
#68924=AXIS2_PLACEMENT_3D('',#102104,#79810,#79811) ;
#68925=AXIS2_PLACEMENT_3D('',#102107,#79812,#79813) ;
#68926=AXIS2_PLACEMENT_3D('',#102111,#79815,#79816) ;
#68927=AXIS2_PLACEMENT_3D('',#102113,#79818,#79819) ;
#68928=AXIS2_PLACEMENT_3D('',#102119,#79823,#79824) ;
#68929=AXIS2_PLACEMENT_3D('',#102128,#79829,#79830) ;
#68930=AXIS2_PLACEMENT_3D('',#102135,#79834,#79835) ;
#68931=AXIS2_PLACEMENT_3D('',#102136,#79836,#79837) ;
#68932=AXIS2_PLACEMENT_3D('',#102145,#79842,#79843) ;
#68933=AXIS2_PLACEMENT_3D('',#102148,#79844,#79845) ;
#68934=AXIS2_PLACEMENT_3D('',#102153,#79848,#79849) ;
#68935=AXIS2_PLACEMENT_3D('',#102157,#79851,#79852) ;
#68936=AXIS2_PLACEMENT_3D('',#102159,#79854,#79855) ;
#68937=AXIS2_PLACEMENT_3D('',#102167,#79860,#79861) ;
#68938=AXIS2_PLACEMENT_3D('',#102176,#79866,#79867) ;
#68939=AXIS2_PLACEMENT_3D('',#102185,#79872,#79873) ;
#68940=AXIS2_PLACEMENT_3D('',#102194,#79878,#79879) ;
#68941=AXIS2_PLACEMENT_3D('',#102200,#79883,#79884) ;
#68942=AXIS2_PLACEMENT_3D('',#102206,#79888,#79889) ;
#68943=AXIS2_PLACEMENT_3D('',#102212,#79893,#79894) ;
#68944=AXIS2_PLACEMENT_3D('',#102218,#79898,#79899) ;
#68945=AXIS2_PLACEMENT_3D('',#102227,#79903,#79904) ;
#68946=AXIS2_PLACEMENT_3D('',#102230,#79906,#79907) ;
#68947=AXIS2_PLACEMENT_3D('',#102231,#79908,#79909) ;
#68948=AXIS2_PLACEMENT_3D('',#102240,#79913,#79914) ;
#68949=AXIS2_PLACEMENT_3D('',#102243,#79916,#79917) ;
#68950=AXIS2_PLACEMENT_3D('',#102244,#79918,#79919) ;
#68951=AXIS2_PLACEMENT_3D('',#102248,#79921,#79922) ;
#68952=AXIS2_PLACEMENT_3D('',#102249,#79923,#79924) ;
#68953=AXIS2_PLACEMENT_3D('',#102250,#79925,#79926) ;
#68954=AXIS2_PLACEMENT_3D('',#102256,#79930,#79931) ;
#68955=AXIS2_PLACEMENT_3D('',#102265,#79936,#79937) ;
#68956=AXIS2_PLACEMENT_3D('',#102274,#79942,#79943) ;
#68957=AXIS2_PLACEMENT_3D('',#102283,#79948,#79949) ;
#68958=AXIS2_PLACEMENT_3D('',#102292,#79954,#79955) ;
#68959=AXIS2_PLACEMENT_3D('',#102293,#79956,#79957) ;
#68960=AXIS2_PLACEMENT_3D('',#102294,#79958,#79959) ;
#68961=AXIS2_PLACEMENT_3D('',#102295,#79960,#79961) ;
#68962=AXIS2_PLACEMENT_3D('',#102304,#79966,#79967) ;
#68963=AXIS2_PLACEMENT_3D('',#102313,#79972,#79973) ;
#68964=AXIS2_PLACEMENT_3D('',#102322,#79978,#79979) ;
#68965=AXIS2_PLACEMENT_3D('',#102331,#79984,#79985) ;
#68966=AXIS2_PLACEMENT_3D('',#102335,#79987,#79988) ;
#68967=AXIS2_PLACEMENT_3D('',#102337,#79990,#79991) ;
#68968=AXIS2_PLACEMENT_3D('',#102340,#79992,#79993) ;
#68969=AXIS2_PLACEMENT_3D('',#102341,#79994,#79995) ;
#68970=AXIS2_PLACEMENT_3D('',#102342,#79996,#79997) ;
#68971=AXIS2_PLACEMENT_3D('',#102343,#79998,#79999) ;
#68972=AXIS2_PLACEMENT_3D('',#102347,#80001,#80002) ;
#68973=AXIS2_PLACEMENT_3D('',#102349,#80004,#80005) ;
#68974=AXIS2_PLACEMENT_3D('',#102350,#80006,#80007) ;
#68975=AXIS2_PLACEMENT_3D('',#102351,#80008,#80009) ;
#68976=AXIS2_PLACEMENT_3D('',#102352,#80010,#80011) ;
#68977=AXIS2_PLACEMENT_3D('',#102353,#80012,#80013) ;
#68978=AXIS2_PLACEMENT_3D('',#102354,#80014,#80015) ;
#68979=AXIS2_PLACEMENT_3D('',#102355,#80016,#80017) ;
#68980=AXIS2_PLACEMENT_3D('',#102356,#80018,#80019) ;
#68981=AXIS2_PLACEMENT_3D('',#102357,#80020,#80021) ;
#68982=AXIS2_PLACEMENT_3D('',#102358,#80022,#80023) ;
#68983=AXIS2_PLACEMENT_3D('',#102359,#80024,#80025) ;
#68984=AXIS2_PLACEMENT_3D('',#102360,#80026,#80027) ;
#68985=AXIS2_PLACEMENT_3D('',#102361,#80028,#80029) ;
#68986=AXIS2_PLACEMENT_3D('',#102362,#80030,#80031) ;
#68987=AXIS2_PLACEMENT_3D('',#102363,#80032,#80033) ;
#68988=AXIS2_PLACEMENT_3D('',#102364,#80034,#80035) ;
#68989=AXIS2_PLACEMENT_3D('',#102365,#80036,#80037) ;
#68990=AXIS2_PLACEMENT_3D('',#102366,#80038,#80039) ;
#68991=AXIS2_PLACEMENT_3D('',#102367,#80040,#80041) ;
#68992=AXIS2_PLACEMENT_3D('',#102368,#80042,#80043) ;
#68993=AXIS2_PLACEMENT_3D('',#102369,#80044,#80045) ;
#68994=AXIS2_PLACEMENT_3D('',#102370,#80046,#80047) ;
#68995=AXIS2_PLACEMENT_3D('',#102371,#80048,#80049) ;
#68996=AXIS2_PLACEMENT_3D('',#102372,#80050,#80051) ;
#68997=AXIS2_PLACEMENT_3D('',#102373,#80052,#80053) ;
#68998=AXIS2_PLACEMENT_3D('',#102374,#80054,#80055) ;
#68999=AXIS2_PLACEMENT_3D('',#102375,#80056,#80057) ;
#69000=AXIS2_PLACEMENT_3D('',#102376,#80058,#80059) ;
#69001=AXIS2_PLACEMENT_3D('',#102377,#80060,#80061) ;
#69002=AXIS2_PLACEMENT_3D('',#102378,#80062,#80063) ;
#69003=AXIS2_PLACEMENT_3D('',#102379,#80064,#80065) ;
#69004=AXIS2_PLACEMENT_3D('',#102380,#80066,#80067) ;
#69005=AXIS2_PLACEMENT_3D('',#102381,#80068,#80069) ;
#69006=AXIS2_PLACEMENT_3D('',#102382,#80070,#80071) ;
#69007=AXIS2_PLACEMENT_3D('',#102383,#80072,#80073) ;
#69008=AXIS2_PLACEMENT_3D('',#102384,#80074,#80075) ;
#69009=AXIS2_PLACEMENT_3D('',#102385,#80076,#80077) ;
#69010=AXIS2_PLACEMENT_3D('',#102386,#80078,#80079) ;
#69011=AXIS2_PLACEMENT_3D('',#102387,#80080,#80081) ;
#69012=AXIS2_PLACEMENT_3D('',#102388,#80082,#80083) ;
#69013=AXIS2_PLACEMENT_3D('',#102389,#80084,#80085) ;
#69014=AXIS2_PLACEMENT_3D('',#102390,#80086,#80087) ;
#69015=AXIS2_PLACEMENT_3D('',#102391,#80088,#80089) ;
#69016=AXIS2_PLACEMENT_3D('',#102392,#80090,#80091) ;
#69017=AXIS2_PLACEMENT_3D('',#102393,#80092,#80093) ;
#69018=AXIS2_PLACEMENT_3D('',#102394,#80094,#80095) ;
#69019=AXIS2_PLACEMENT_3D('',#102395,#80096,#80097) ;
#69020=AXIS2_PLACEMENT_3D('',#102396,#80098,#80099) ;
#69021=AXIS2_PLACEMENT_3D('',#102397,#80100,#80101) ;
#69022=AXIS2_PLACEMENT_3D('',#102398,#80102,#80103) ;
#69023=AXIS2_PLACEMENT_3D('',#102399,#80104,#80105) ;
#69024=AXIS2_PLACEMENT_3D('',#102400,#80106,#80107) ;
#69025=AXIS2_PLACEMENT_3D('',#102401,#80108,#80109) ;
#69026=AXIS2_PLACEMENT_3D('',#102402,#80110,#80111) ;
#69027=AXIS2_PLACEMENT_3D('',#102403,#80112,#80113) ;
#69028=AXIS2_PLACEMENT_3D('',#102404,#80114,#80115) ;
#69029=AXIS2_PLACEMENT_3D('',#102405,#80116,#80117) ;
#69030=AXIS2_PLACEMENT_3D('',#102406,#80118,#80119) ;
#69031=AXIS2_PLACEMENT_3D('',#102407,#80120,#80121) ;
#69032=AXIS2_PLACEMENT_3D('',#102408,#80122,#80123) ;
#69033=AXIS2_PLACEMENT_3D('',#102409,#80124,#80125) ;
#69034=AXIS2_PLACEMENT_3D('',#102410,#80126,#80127) ;
#69035=AXIS2_PLACEMENT_3D('',#102411,#80128,#80129) ;
#69036=AXIS2_PLACEMENT_3D('',#102412,#80130,#80131) ;
#69037=AXIS2_PLACEMENT_3D('',#102413,#80132,#80133) ;
#69038=AXIS2_PLACEMENT_3D('',#102414,#80134,#80135) ;
#69039=AXIS2_PLACEMENT_3D('',#102415,#80136,#80137) ;
#69040=AXIS2_PLACEMENT_3D('',#102416,#80138,#80139) ;
#69041=AXIS2_PLACEMENT_3D('',#102417,#80140,#80141) ;
#69042=AXIS2_PLACEMENT_3D('',#102418,#80142,#80143) ;
#69043=AXIS2_PLACEMENT_3D('',#102419,#80144,#80145) ;
#69044=AXIS2_PLACEMENT_3D('',#102420,#80146,#80147) ;
#69045=AXIS2_PLACEMENT_3D('',#102421,#80148,#80149) ;
#69046=AXIS2_PLACEMENT_3D('',#102422,#80150,#80151) ;
#69047=AXIS2_PLACEMENT_3D('',#102438,#80152,#80153) ;
#69048=AXIS2_PLACEMENT_3D('',#102439,#80154,#80155) ;
#69049=AXIS2_PLACEMENT_3D('',#102441,#80156,#80157) ;
#69050=AXIS2_PLACEMENT_3D('',#102456,#80158,#80159) ;
#69051=AXIS2_PLACEMENT_3D('',#102457,#80160,#80161) ;
#69052=AXIS2_PLACEMENT_3D('',#102458,#80162,#80163) ;
#69053=AXIS2_PLACEMENT_3D('',#102460,#80164,#80165) ;
#69054=AXIS2_PLACEMENT_3D('',#102490,#80166,#80167) ;
#69055=AXIS2_PLACEMENT_3D('',#102491,#80168,#80169) ;
#69056=AXIS2_PLACEMENT_3D('',#102507,#80170,#80171) ;
#69057=AXIS2_PLACEMENT_3D('',#102509,#80172,#80173) ;
#69058=AXIS2_PLACEMENT_3D('',#102524,#80174,#80175) ;
#69059=AXIS2_PLACEMENT_3D('',#102525,#80176,#80177) ;
#69060=AXIS2_PLACEMENT_3D('',#102526,#80178,#80179) ;
#69061=AXIS2_PLACEMENT_3D('',#102527,#80180,#80181) ;
#69062=AXIS2_PLACEMENT_3D('',#102530,#80183,#80184) ;
#69063=AXIS2_PLACEMENT_3D('',#102531,#80185,#80186) ;
#69064=AXIS2_PLACEMENT_3D('',#102533,#80187,#80188) ;
#69065=AXIS2_PLACEMENT_3D('',#102534,#80189,#80190) ;
#69066=AXIS2_PLACEMENT_3D('',#102535,#80191,#80192) ;
#69067=AXIS2_PLACEMENT_3D('',#102537,#80193,#80194) ;
#69068=AXIS2_PLACEMENT_3D('',#102552,#80195,#80196) ;
#69069=AXIS2_PLACEMENT_3D('',#102553,#80197,#80198) ;
#69070=AXIS2_PLACEMENT_3D('',#102569,#80199,#80200) ;
#69071=AXIS2_PLACEMENT_3D('',#102570,#80201,#80202) ;
#69072=AXIS2_PLACEMENT_3D('',#102571,#80203,#80204) ;
#69073=AXIS2_PLACEMENT_3D('',#102573,#80205,#80206) ;
#69074=AXIS2_PLACEMENT_3D('',#102575,#80208,#80209) ;
#69075=AXIS2_PLACEMENT_3D('',#102576,#80210,#80211) ;
#69076=AXIS2_PLACEMENT_3D('',#102577,#80212,#80213) ;
#69077=AXIS2_PLACEMENT_3D('',#102578,#80214,#80215) ;
#69078=AXIS2_PLACEMENT_3D('',#102579,#80216,#80217) ;
#69079=AXIS2_PLACEMENT_3D('',#102580,#80218,#80219) ;
#69080=AXIS2_PLACEMENT_3D('',#102583,#80221,#80222) ;
#69081=AXIS2_PLACEMENT_3D('',#102584,#80223,#80224) ;
#69082=AXIS2_PLACEMENT_3D('',#102585,#80225,#80226) ;
#69083=AXIS2_PLACEMENT_3D('',#102586,#80227,#80228) ;
#69084=AXIS2_PLACEMENT_3D('',#102588,#80229,#80230) ;
#69085=AXIS2_PLACEMENT_3D('',#102589,#80231,#80232) ;
#69086=AXIS2_PLACEMENT_3D('',#102590,#80233,#80234) ;
#69087=AXIS2_PLACEMENT_3D('',#102591,#80235,#80236) ;
#69088=AXIS2_PLACEMENT_3D('',#102592,#80237,#80238) ;
#69089=AXIS2_PLACEMENT_3D('',#102593,#80239,#80240) ;
#69090=AXIS2_PLACEMENT_3D('',#102594,#80241,#80242) ;
#69091=AXIS2_PLACEMENT_3D('',#102596,#80243,#80244) ;
#69092=AXIS2_PLACEMENT_3D('',#102597,#80245,#80246) ;
#69093=AXIS2_PLACEMENT_3D('',#102598,#80247,#80248) ;
#69094=AXIS2_PLACEMENT_3D('',#102599,#80249,#80250) ;
#69095=AXIS2_PLACEMENT_3D('',#102600,#80251,#80252) ;
#69096=AXIS2_PLACEMENT_3D('',#102602,#80253,#80254) ;
#69097=AXIS2_PLACEMENT_3D('',#102604,#80256,#80257) ;
#69098=AXIS2_PLACEMENT_3D('',#102605,#80258,#80259) ;
#69099=AXIS2_PLACEMENT_3D('',#102606,#80260,#80261) ;
#69100=AXIS2_PLACEMENT_3D('',#102607,#80262,#80263) ;
#69101=AXIS2_PLACEMENT_3D('',#102608,#80264,#80265) ;
#69102=AXIS2_PLACEMENT_3D('',#102610,#80267,#80268) ;
#69103=AXIS2_PLACEMENT_3D('',#102611,#80269,#80270) ;
#69104=AXIS2_PLACEMENT_3D('',#102612,#80271,#80272) ;
#69105=AXIS2_PLACEMENT_3D('',#102613,#80273,#80274) ;
#69106=AXIS2_PLACEMENT_3D('',#102615,#80275,#80276) ;
#69107=AXIS2_PLACEMENT_3D('',#102616,#80277,#80278) ;
#69108=AXIS2_PLACEMENT_3D('',#102617,#80279,#80280) ;
#69109=AXIS2_PLACEMENT_3D('',#102618,#80281,#80282) ;
#69110=AXIS2_PLACEMENT_3D('',#102619,#80283,#80284) ;
#69111=AXIS2_PLACEMENT_3D('',#102620,#80285,#80286) ;
#69112=AXIS2_PLACEMENT_3D('',#102621,#80287,#80288) ;
#69113=AXIS2_PLACEMENT_3D('',#102623,#80290,#80291) ;
#69114=AXIS2_PLACEMENT_3D('',#102624,#80292,#80293) ;
#69115=AXIS2_PLACEMENT_3D('',#102625,#80294,#80295) ;
#69116=AXIS2_PLACEMENT_3D('',#102626,#80296,#80297) ;
#69117=AXIS2_PLACEMENT_3D('',#102627,#80298,#80299) ;
#69118=AXIS2_PLACEMENT_3D('',#102628,#80300,#80301) ;
#69119=AXIS2_PLACEMENT_3D('',#102629,#80302,#80303) ;
#69120=AXIS2_PLACEMENT_3D('',#102630,#80304,#80305) ;
#69121=AXIS2_PLACEMENT_3D('',#102631,#80306,#80307) ;
#69122=AXIS2_PLACEMENT_3D('',#102632,#80308,#80309) ;
#69123=AXIS2_PLACEMENT_3D('',#102633,#80310,#80311) ;
#69124=AXIS2_PLACEMENT_3D('',#102634,#80312,#80313) ;
#69125=AXIS2_PLACEMENT_3D('',#102635,#80314,#80315) ;
#69126=AXIS2_PLACEMENT_3D('',#102636,#80316,#80317) ;
#69127=AXIS2_PLACEMENT_3D('',#102637,#80318,#80319) ;
#69128=AXIS2_PLACEMENT_3D('',#102638,#80320,#80321) ;
#69129=AXIS2_PLACEMENT_3D('',#102639,#80322,#80323) ;
#69130=AXIS2_PLACEMENT_3D('',#102640,#80324,#80325) ;
#69131=AXIS2_PLACEMENT_3D('',#102641,#80326,#80327) ;
#69132=AXIS2_PLACEMENT_3D('',#102642,#80328,#80329) ;
#69133=AXIS2_PLACEMENT_3D('',#102643,#80330,#80331) ;
#69134=AXIS2_PLACEMENT_3D('',#102644,#80332,#80333) ;
#69135=AXIS2_PLACEMENT_3D('',#102645,#80334,#80335) ;
#69136=AXIS2_PLACEMENT_3D('',#102646,#80336,#80337) ;
#69137=AXIS2_PLACEMENT_3D('',#102647,#80338,#80339) ;
#69138=AXIS2_PLACEMENT_3D('',#102648,#80340,#80341) ;
#69139=AXIS2_PLACEMENT_3D('',#102649,#80342,#80343) ;
#69140=AXIS2_PLACEMENT_3D('',#102650,#80344,#80345) ;
#69141=AXIS2_PLACEMENT_3D('',#102651,#80346,#80347) ;
#69142=AXIS2_PLACEMENT_3D('',#102652,#80348,#80349) ;
#69143=AXIS2_PLACEMENT_3D('',#102653,#80350,#80351) ;
#69144=AXIS2_PLACEMENT_3D('',#102654,#80352,#80353) ;
#69145=AXIS2_PLACEMENT_3D('',#102655,#80354,#80355) ;
#69146=AXIS2_PLACEMENT_3D('',#102656,#80356,#80357) ;
#69147=AXIS2_PLACEMENT_3D('',#102657,#80358,#80359) ;
#69148=AXIS2_PLACEMENT_3D('',#102658,#80360,#80361) ;
#69149=AXIS2_PLACEMENT_3D('',#102659,#80362,#80363) ;
#69150=AXIS2_PLACEMENT_3D('',#102660,#80364,#80365) ;
#69151=AXIS2_PLACEMENT_3D('',#102661,#80366,#80367) ;
#69152=AXIS2_PLACEMENT_3D('',#102662,#80368,#80369) ;
#69153=AXIS2_PLACEMENT_3D('',#102663,#80370,#80371) ;
#69154=AXIS2_PLACEMENT_3D('',#102664,#80372,#80373) ;
#69155=AXIS2_PLACEMENT_3D('',#102665,#80374,#80375) ;
#69156=AXIS2_PLACEMENT_3D('',#102666,#80376,#80377) ;
#69157=AXIS2_PLACEMENT_3D('',#102667,#80378,#80379) ;
#69158=AXIS2_PLACEMENT_3D('',#102668,#80380,#80381) ;
#69159=AXIS2_PLACEMENT_3D('',#102669,#80382,#80383) ;
#69160=AXIS2_PLACEMENT_3D('',#102670,#80384,#80385) ;
#69161=AXIS2_PLACEMENT_3D('',#102671,#80386,#80387) ;
#69162=AXIS2_PLACEMENT_3D('',#102672,#80388,#80389) ;
#69163=AXIS2_PLACEMENT_3D('',#102689,#80390,#80391) ;
#69164=AXIS2_PLACEMENT_3D('',#102690,#80392,#80393) ;
#69165=AXIS2_PLACEMENT_3D('',#102691,#80394,#80395) ;
#69166=AXIS2_PLACEMENT_3D('',#102692,#80396,#80397) ;
#69167=AXIS2_PLACEMENT_3D('',#102693,#80398,#80399) ;
#69168=AXIS2_PLACEMENT_3D('',#102694,#80400,#80401) ;
#69169=AXIS2_PLACEMENT_3D('',#102695,#80402,#80403) ;
#69170=AXIS2_PLACEMENT_3D('',#102696,#80404,#80405) ;
#69171=AXIS2_PLACEMENT_3D('',#102697,#80406,#80407) ;
#69172=AXIS2_PLACEMENT_3D('',#102698,#80408,#80409) ;
#69173=AXIS2_PLACEMENT_3D('',#102699,#80410,#80411) ;
#69174=AXIS2_PLACEMENT_3D('',#102718,#80412,#80413) ;
#69175=AXIS2_PLACEMENT_3D('',#102719,#80414,#80415) ;
#69176=AXIS2_PLACEMENT_3D('',#102721,#80416,#80417) ;
#69177=AXIS2_PLACEMENT_3D('',#102722,#80418,#80419) ;
#69178=AXIS2_PLACEMENT_3D('',#102723,#80420,#80421) ;
#69179=AXIS2_PLACEMENT_3D('',#102724,#80422,#80423) ;
#69180=AXIS2_PLACEMENT_3D('',#102725,#80424,#80425) ;
#69181=AXIS2_PLACEMENT_3D('',#102726,#80426,#80427) ;
#69182=AXIS2_PLACEMENT_3D('',#102727,#80428,#80429) ;
#69183=AXIS2_PLACEMENT_3D('',#102728,#80430,#80431) ;
#69184=AXIS2_PLACEMENT_3D('',#102729,#80432,#80433) ;
#69185=AXIS2_PLACEMENT_3D('',#102730,#80434,#80435) ;
#69186=AXIS2_PLACEMENT_3D('',#102731,#80436,#80437) ;
#69187=AXIS2_PLACEMENT_3D('',#102766,#80438,#80439) ;
#69188=AXIS2_PLACEMENT_3D('',#102767,#80440,#80441) ;
#69189=AXIS2_PLACEMENT_3D('',#102768,#80442,#80443) ;
#69190=AXIS2_PLACEMENT_3D('',#102769,#80444,#80445) ;
#69191=AXIS2_PLACEMENT_3D('',#102780,#80446,#80447) ;
#69192=AXIS2_PLACEMENT_3D('',#102781,#80448,#80449) ;
#69193=AXIS2_PLACEMENT_3D('',#102782,#80450,#80451) ;
#69194=AXIS2_PLACEMENT_3D('',#102783,#80452,#80453) ;
#69195=AXIS2_PLACEMENT_3D('',#102790,#80454,#80455) ;
#69196=AXIS2_PLACEMENT_3D('',#102791,#80456,#80457) ;
#69197=AXIS2_PLACEMENT_3D('',#102792,#80458,#80459) ;
#69198=AXIS2_PLACEMENT_3D('',#102793,#80460,#80461) ;
#69199=AXIS2_PLACEMENT_3D('',#102794,#80462,#80463) ;
#69200=AXIS2_PLACEMENT_3D('',#102805,#80464,#80465) ;
#69201=AXIS2_PLACEMENT_3D('',#102806,#80466,#80467) ;
#69202=AXIS2_PLACEMENT_3D('',#102807,#80468,#80469) ;
#69203=AXIS2_PLACEMENT_3D('',#102808,#80470,#80471) ;
#69204=AXIS2_PLACEMENT_3D('',#102809,#80472,#80473) ;
#69205=AXIS2_PLACEMENT_3D('',#102810,#80474,#80475) ;
#69206=AXIS2_PLACEMENT_3D('',#102811,#80476,#80477) ;
#69207=AXIS2_PLACEMENT_3D('',#102812,#80478,#80479) ;
#69208=AXIS2_PLACEMENT_3D('',#102813,#80480,#80481) ;
#69209=AXIS2_PLACEMENT_3D('',#102814,#80482,#80483) ;
#69210=AXIS2_PLACEMENT_3D('',#102815,#80484,#80485) ;
#69211=AXIS2_PLACEMENT_3D('',#102816,#80486,#80487) ;
#69212=AXIS2_PLACEMENT_3D('',#102817,#80488,#80489) ;
#69213=AXIS2_PLACEMENT_3D('',#102818,#80490,#80491) ;
#69214=AXIS2_PLACEMENT_3D('',#102819,#80492,#80493) ;
#69215=AXIS2_PLACEMENT_3D('',#102820,#80494,#80495) ;
#69216=AXIS2_PLACEMENT_3D('',#102821,#80496,#80497) ;
#69217=AXIS2_PLACEMENT_3D('',#102822,#80498,#80499) ;
#69218=AXIS2_PLACEMENT_3D('',#102823,#80500,#80501) ;
#69219=AXIS2_PLACEMENT_3D('',#102824,#80502,#80503) ;
#69220=AXIS2_PLACEMENT_3D('',#102825,#80504,#80505) ;
#69221=AXIS2_PLACEMENT_3D('',#102826,#80506,#80507) ;
#69222=AXIS2_PLACEMENT_3D('',#102827,#80508,#80509) ;
#69223=AXIS2_PLACEMENT_3D('',#102828,#80510,#80511) ;
#69224=AXIS2_PLACEMENT_3D('',#102829,#80512,#80513) ;
#69225=AXIS2_PLACEMENT_3D('',#102830,#80514,#80515) ;
#69226=AXIS2_PLACEMENT_3D('',#102831,#80516,#80517) ;
#69227=AXIS2_PLACEMENT_3D('',#102832,#80518,#80519) ;
#69228=AXIS2_PLACEMENT_3D('',#102833,#80520,#80521) ;
#69229=AXIS2_PLACEMENT_3D('',#102834,#80522,#80523) ;
#69230=AXIS2_PLACEMENT_3D('',#102835,#80524,#80525) ;
#69231=AXIS2_PLACEMENT_3D('',#102836,#80526,#80527) ;
#69232=AXIS2_PLACEMENT_3D('',#102837,#80528,#80529) ;
#69233=AXIS2_PLACEMENT_3D('',#102838,#80530,#80531) ;
#69234=AXIS2_PLACEMENT_3D('',#102845,#80532,#80533) ;
#69235=AXIS2_PLACEMENT_3D('',#102846,#80534,#80535) ;
#69236=AXIS2_PLACEMENT_3D('',#102847,#80536,#80537) ;
#69237=AXIS2_PLACEMENT_3D('',#102848,#80538,#80539) ;
#69238=AXIS2_PLACEMENT_3D('',#102849,#80540,#80541) ;
#69239=AXIS2_PLACEMENT_3D('',#102850,#80542,#80543) ;
#69240=AXIS2_PLACEMENT_3D('',#102851,#80544,#80545) ;
#69241=AXIS2_PLACEMENT_3D('',#102852,#80546,#80547) ;
#69242=AXIS2_PLACEMENT_3D('',#102853,#80548,#80549) ;
#69243=AXIS2_PLACEMENT_3D('',#102854,#80550,#80551) ;
#69244=AXIS2_PLACEMENT_3D('',#102855,#80552,#80553) ;
#69245=AXIS2_PLACEMENT_3D('',#102856,#80554,#80555) ;
#69246=AXIS2_PLACEMENT_3D('',#102857,#80556,#80557) ;
#69247=AXIS2_PLACEMENT_3D('',#102858,#80558,#80559) ;
#69248=AXIS2_PLACEMENT_3D('',#102859,#80560,#80561) ;
#69249=AXIS2_PLACEMENT_3D('',#102860,#80562,#80563) ;
#69250=AXIS2_PLACEMENT_3D('',#102861,#80564,#80565) ;
#69251=AXIS2_PLACEMENT_3D('',#102862,#80566,#80567) ;
#69252=AXIS2_PLACEMENT_3D('',#102863,#80568,#80569) ;
#69253=AXIS2_PLACEMENT_3D('',#102864,#80570,#80571) ;
#69254=AXIS2_PLACEMENT_3D('',#102865,#80572,#80573) ;
#69255=AXIS2_PLACEMENT_3D('',#102866,#80574,#80575) ;
#69256=AXIS2_PLACEMENT_3D('',#102867,#80576,#80577) ;
#69257=AXIS2_PLACEMENT_3D('',#102868,#80578,#80579) ;
#69258=AXIS2_PLACEMENT_3D('',#102869,#80580,#80581) ;
#69259=AXIS2_PLACEMENT_3D('',#102870,#80582,#80583) ;
#69260=AXIS2_PLACEMENT_3D('',#102871,#80584,#80585) ;
#69261=AXIS2_PLACEMENT_3D('',#102872,#80586,#80587) ;
#69262=AXIS2_PLACEMENT_3D('',#102873,#80588,#80589) ;
#69263=AXIS2_PLACEMENT_3D('',#102874,#80590,#80591) ;
#69264=AXIS2_PLACEMENT_3D('',#102875,#80592,#80593) ;
#69265=AXIS2_PLACEMENT_3D('',#102876,#80594,#80595) ;
#69266=AXIS2_PLACEMENT_3D('',#102877,#80596,#80597) ;
#69267=AXIS2_PLACEMENT_3D('',#102878,#80598,#80599) ;
#69268=AXIS2_PLACEMENT_3D('',#102879,#80600,#80601) ;
#69269=AXIS2_PLACEMENT_3D('',#102880,#80602,#80603) ;
#69270=AXIS2_PLACEMENT_3D('',#102881,#80604,#80605) ;
#69271=AXIS2_PLACEMENT_3D('',#102882,#80606,#80607) ;
#69272=AXIS2_PLACEMENT_3D('',#102883,#80608,#80609) ;
#69273=AXIS2_PLACEMENT_3D('',#102914,#80610,#80611) ;
#69274=AXIS2_PLACEMENT_3D('',#102915,#80612,#80613) ;
#69275=AXIS2_PLACEMENT_3D('',#102916,#80614,#80615) ;
#69276=AXIS2_PLACEMENT_3D('',#102917,#80616,#80617) ;
#69277=AXIS2_PLACEMENT_3D('',#102918,#80618,#80619) ;
#69278=AXIS2_PLACEMENT_3D('',#102919,#80620,#80621) ;
#69279=AXIS2_PLACEMENT_3D('',#102920,#80622,#80623) ;
#69280=AXIS2_PLACEMENT_3D('',#102921,#80624,#80625) ;
#69281=AXIS2_PLACEMENT_3D('',#102922,#80626,#80627) ;
#69282=AXIS2_PLACEMENT_3D('',#102923,#80628,#80629) ;
#69283=AXIS2_PLACEMENT_3D('',#102950,#80630,#80631) ;
#69284=AXIS2_PLACEMENT_3D('',#102951,#80632,#80633) ;
#69285=AXIS2_PLACEMENT_3D('',#102952,#80634,#80635) ;
#69286=AXIS2_PLACEMENT_3D('',#102953,#80636,#80637) ;
#69287=AXIS2_PLACEMENT_3D('',#102954,#80638,#80639) ;
#69288=AXIS2_PLACEMENT_3D('',#102955,#80640,#80641) ;
#69289=AXIS2_PLACEMENT_3D('',#102956,#80642,#80643) ;
#69290=AXIS2_PLACEMENT_3D('',#102957,#80644,#80645) ;
#69291=AXIS2_PLACEMENT_3D('',#102958,#80646,#80647) ;
#69292=AXIS2_PLACEMENT_3D('',#102959,#80648,#80649) ;
#69293=AXIS2_PLACEMENT_3D('',#102960,#80650,#80651) ;
#69294=AXIS2_PLACEMENT_3D('',#102961,#80652,#80653) ;
#69295=AXIS2_PLACEMENT_3D('',#102962,#80654,#80655) ;
#69296=AXIS2_PLACEMENT_3D('',#102963,#80656,#80657) ;
#69297=AXIS2_PLACEMENT_3D('',#102964,#80658,#80659) ;
#69298=AXIS2_PLACEMENT_3D('',#102965,#80660,#80661) ;
#69299=AXIS2_PLACEMENT_3D('',#102966,#80662,#80663) ;
#69300=AXIS2_PLACEMENT_3D('',#102967,#80664,#80665) ;
#69301=AXIS2_PLACEMENT_3D('',#102968,#80666,#80667) ;
#69302=AXIS2_PLACEMENT_3D('',#102969,#80668,#80669) ;
#69303=AXIS2_PLACEMENT_3D('',#102970,#80670,#80671) ;
#69304=AXIS2_PLACEMENT_3D('',#102971,#80672,#80673) ;
#69305=AXIS2_PLACEMENT_3D('',#102972,#80674,#80675) ;
#69306=AXIS2_PLACEMENT_3D('',#102973,#80676,#80677) ;
#69307=AXIS2_PLACEMENT_3D('',#102974,#80678,#80679) ;
#69308=AXIS2_PLACEMENT_3D('',#102975,#80680,#80681) ;
#69309=AXIS2_PLACEMENT_3D('',#102976,#80682,#80683) ;
#69310=AXIS2_PLACEMENT_3D('',#102977,#80684,#80685) ;
#69311=AXIS2_PLACEMENT_3D('',#102978,#80686,#80687) ;
#69312=AXIS2_PLACEMENT_3D('',#103003,#80688,#80689) ;
#69313=AXIS2_PLACEMENT_3D('',#103004,#80690,#80691) ;
#69314=AXIS2_PLACEMENT_3D('',#103005,#80692,#80693) ;
#69315=AXIS2_PLACEMENT_3D('',#103006,#80694,#80695) ;
#69316=AXIS2_PLACEMENT_3D('',#103007,#80696,#80697) ;
#69317=AXIS2_PLACEMENT_3D('',#103008,#80698,#80699) ;
#69318=AXIS2_PLACEMENT_3D('',#103009,#80700,#80701) ;
#69319=AXIS2_PLACEMENT_3D('',#103058,#80702,#80703) ;
#69320=AXIS2_PLACEMENT_3D('',#103059,#80704,#80705) ;
#69321=AXIS2_PLACEMENT_3D('',#103060,#80706,#80707) ;
#69322=AXIS2_PLACEMENT_3D('',#103061,#80708,#80709) ;
#69323=AXIS2_PLACEMENT_3D('',#103062,#80710,#80711) ;
#69324=AXIS2_PLACEMENT_3D('',#103063,#80712,#80713) ;
#69325=AXIS2_PLACEMENT_3D('',#103064,#80714,#80715) ;
#69326=AXIS2_PLACEMENT_3D('',#103126,#80716,#80717) ;
#69327=AXIS2_PLACEMENT_3D('',#103127,#80718,#80719) ;
#69328=AXIS2_PLACEMENT_3D('',#103128,#80720,#80721) ;
#69329=AXIS2_PLACEMENT_3D('',#103301,#80722,#80723) ;
#69330=AXIS2_PLACEMENT_3D('',#103302,#80724,#80725) ;
#69331=AXIS2_PLACEMENT_3D('',#103357,#80726,#80727) ;
#69332=AXIS2_PLACEMENT_3D('',#103404,#80728,#80729) ;
#69333=AXIS2_PLACEMENT_3D('',#103405,#80730,#80731) ;
#69334=AXIS2_PLACEMENT_3D('',#103406,#80732,#80733) ;
#69335=AXIS2_PLACEMENT_3D('',#103407,#80734,#80735) ;
#69336=AXIS2_PLACEMENT_3D('',#103408,#80736,#80737) ;
#69337=AXIS2_PLACEMENT_3D('',#103409,#80738,#80739) ;
#69338=AXIS2_PLACEMENT_3D('',#103514,#80740,#80741) ;
#69339=AXIS2_PLACEMENT_3D('',#103515,#80742,#80743) ;
#69340=AXIS2_PLACEMENT_3D('',#103516,#80744,#80745) ;
#69341=AXIS2_PLACEMENT_3D('',#103517,#80746,#80747) ;
#69342=AXIS2_PLACEMENT_3D('',#103530,#80748,#80749) ;
#69343=AXIS2_PLACEMENT_3D('',#103531,#80750,#80751) ;
#69344=AXIS2_PLACEMENT_3D('',#103532,#80752,#80753) ;
#69345=AXIS2_PLACEMENT_3D('',#103533,#80754,#80755) ;
#69346=AXIS2_PLACEMENT_3D('',#103534,#80756,#80757) ;
#69347=AXIS2_PLACEMENT_3D('',#103535,#80758,#80759) ;
#69348=AXIS2_PLACEMENT_3D('',#103536,#80760,#80761) ;
#69349=AXIS2_PLACEMENT_3D('',#103537,#80762,#80763) ;
#69350=AXIS2_PLACEMENT_3D('',#103538,#80764,#80765) ;
#69351=AXIS2_PLACEMENT_3D('',#103539,#80766,#80767) ;
#69352=AXIS2_PLACEMENT_3D('',#103540,#80768,#80769) ;
#69353=AXIS2_PLACEMENT_3D('',#103541,#80770,#80771) ;
#69354=AXIS2_PLACEMENT_3D('',#103542,#80772,#80773) ;
#69355=AXIS2_PLACEMENT_3D('',#103543,#80774,#80775) ;
#69356=AXIS2_PLACEMENT_3D('',#103544,#80776,#80777) ;
#69357=AXIS2_PLACEMENT_3D('',#103545,#80778,#80779) ;
#69358=AXIS2_PLACEMENT_3D('',#103546,#80780,#80781) ;
#69359=AXIS2_PLACEMENT_3D('',#103547,#80782,#80783) ;
#69360=AXIS2_PLACEMENT_3D('',#103548,#80784,#80785) ;
#69361=AXIS2_PLACEMENT_3D('',#103549,#80786,#80787) ;
#69362=AXIS2_PLACEMENT_3D('',#103550,#80788,#80789) ;
#69363=AXIS2_PLACEMENT_3D('',#103551,#80790,#80791) ;
#69364=AXIS2_PLACEMENT_3D('',#103552,#80792,#80793) ;
#69365=AXIS2_PLACEMENT_3D('',#103553,#80794,#80795) ;
#69366=AXIS2_PLACEMENT_3D('',#103554,#80796,#80797) ;
#69367=AXIS2_PLACEMENT_3D('',#103555,#80798,#80799) ;
#69368=AXIS2_PLACEMENT_3D('',#103556,#80800,#80801) ;
#69369=AXIS2_PLACEMENT_3D('',#103557,#80802,#80803) ;
#69370=AXIS2_PLACEMENT_3D('',#103558,#80804,#80805) ;
#69371=AXIS2_PLACEMENT_3D('',#103559,#80806,#80807) ;
#69372=AXIS2_PLACEMENT_3D('',#103560,#80808,#80809) ;
#69373=AXIS2_PLACEMENT_3D('',#103561,#80810,#80811) ;
#69374=AXIS2_PLACEMENT_3D('',#103562,#80812,#80813) ;
#69375=AXIS2_PLACEMENT_3D('',#103563,#80814,#80815) ;
#69376=AXIS2_PLACEMENT_3D('',#103564,#80816,#80817) ;
#69377=AXIS2_PLACEMENT_3D('',#103565,#80818,#80819) ;
#69378=AXIS2_PLACEMENT_3D('',#103566,#80820,#80821) ;
#69379=AXIS2_PLACEMENT_3D('',#103567,#80822,#80823) ;
#69380=AXIS2_PLACEMENT_3D('',#103580,#80824,#80825) ;
#69381=AXIS2_PLACEMENT_3D('',#103581,#80826,#80827) ;
#69382=AXIS2_PLACEMENT_3D('',#103582,#80828,#80829) ;
#69383=AXIS2_PLACEMENT_3D('',#103583,#80830,#80831) ;
#69384=AXIS2_PLACEMENT_3D('',#103638,#80832,#80833) ;
#69385=AXIS2_PLACEMENT_3D('',#103639,#80834,#80835) ;
#69386=AXIS2_PLACEMENT_3D('',#103640,#80836,#80837) ;
#69387=AXIS2_PLACEMENT_3D('',#103695,#80838,#80839) ;
#69388=AXIS2_PLACEMENT_3D('',#103696,#80840,#80841) ;
#69389=AXIS2_PLACEMENT_3D('',#103722,#80842,#80843) ;
#69390=AXIS2_PLACEMENT_3D('',#103724,#80844,#80845) ;
#69391=AXIS2_PLACEMENT_3D('',#103726,#80846,#80847) ;
#69392=AXIS2_PLACEMENT_3D('',#103765,#80848,#80849) ;
#69393=AXIS2_PLACEMENT_3D('',#103767,#80850,#80851) ;
#69394=AXIS2_PLACEMENT_3D('',#103769,#80852,#80853) ;
#69395=AXIS2_PLACEMENT_3D('',#103770,#80854,#80855) ;
#69396=AXIS2_PLACEMENT_3D('',#103771,#80856,#80857) ;
#69397=AXIS2_PLACEMENT_3D('',#103773,#80858,#80859) ;
#69398=AXIS2_PLACEMENT_3D('',#103775,#80860,#80861) ;
#69399=AXIS2_PLACEMENT_3D('',#103776,#80862,#80863) ;
#69400=AXIS2_PLACEMENT_3D('',#103777,#80864,#80865) ;
#69401=AXIS2_PLACEMENT_3D('',#103779,#80866,#80867) ;
#69402=AXIS2_PLACEMENT_3D('',#103781,#80868,#80869) ;
#69403=AXIS2_PLACEMENT_3D('',#103782,#80870,#80871) ;
#69404=AXIS2_PLACEMENT_3D('',#103783,#80872,#80873) ;
#69405=AXIS2_PLACEMENT_3D('',#103786,#80874,#80875) ;
#69406=AXIS2_PLACEMENT_3D('',#103790,#80877,#80878) ;
#69407=AXIS2_PLACEMENT_3D('',#103792,#80879,#80880) ;
#69408=AXIS2_PLACEMENT_3D('',#103794,#80882,#80883) ;
#69409=AXIS2_PLACEMENT_3D('',#103797,#80884,#80885) ;
#69410=AXIS2_PLACEMENT_3D('',#103801,#80887,#80888) ;
#69411=AXIS2_PLACEMENT_3D('',#103803,#80890,#80891) ;
#69412=AXIS2_PLACEMENT_3D('',#103806,#80892,#80893) ;
#69413=AXIS2_PLACEMENT_3D('',#103808,#80894,#80895) ;
#69414=AXIS2_PLACEMENT_3D('',#103810,#80896,#80897) ;
#69415=AXIS2_PLACEMENT_3D('',#103811,#80898,#80899) ;
#69416=AXIS2_PLACEMENT_3D('',#103812,#80900,#80901) ;
#69417=AXIS2_PLACEMENT_3D('',#103814,#80903,#80904) ;
#69418=AXIS2_PLACEMENT_3D('',#103817,#80906,#80907) ;
#69419=AXIS2_PLACEMENT_3D('',#103826,#80908,#80909) ;
#69420=AXIS2_PLACEMENT_3D('',#103834,#80910,#80911) ;
#69421=AXIS2_PLACEMENT_3D('',#103836,#80913,#80914) ;
#69422=AXIS2_PLACEMENT_3D('',#103852,#80918,#80919) ;
#69423=AXIS2_PLACEMENT_3D('',#103854,#80921,#80922) ;
#69424=AXIS2_PLACEMENT_3D('',#103903,#80927,#80928) ;
#69425=AXIS2_PLACEMENT_3D('',#103912,#80933,#80934) ;
#69426=AXIS2_PLACEMENT_3D('',#103942,#80939,#80940) ;
#69427=AXIS2_PLACEMENT_3D('',#103951,#80945,#80946) ;
#69428=AXIS2_PLACEMENT_3D('',#103960,#80951,#80952) ;
#69429=AXIS2_PLACEMENT_3D('',#103971,#80957,#80958) ;
#69430=AXIS2_PLACEMENT_3D('',#103973,#80960,#80961) ;
#69431=AXIS2_PLACEMENT_3D('',#103977,#80963,#80964) ;
#69432=AXIS2_PLACEMENT_3D('',#103978,#80965,#80966) ;
#69433=AXIS2_PLACEMENT_3D('',#103979,#80967,#80968) ;
#69434=AXIS2_PLACEMENT_3D('',#103981,#80969,#80970) ;
#69435=AXIS2_PLACEMENT_3D('',#103985,#80972,#80973) ;
#69436=AXIS2_PLACEMENT_3D('',#103989,#80975,#80976) ;
#69437=AXIS2_PLACEMENT_3D('',#103993,#80978,#80979) ;
#69438=AXIS2_PLACEMENT_3D('',#103997,#80981,#80982) ;
#69439=AXIS2_PLACEMENT_3D('',#104001,#80984,#80985) ;
#69440=AXIS2_PLACEMENT_3D('',#104004,#80987,#80988) ;
#69441=AXIS2_PLACEMENT_3D('',#104006,#80989,#80990) ;
#69442=AXIS2_PLACEMENT_3D('',#104009,#80992,#80993) ;
#69443=AXIS2_PLACEMENT_3D('',#104011,#80994,#80995) ;
#69444=AXIS2_PLACEMENT_3D('',#104017,#80998,#80999) ;
#69445=AXIS2_PLACEMENT_3D('',#104021,#81001,#81002) ;
#69446=AXIS2_PLACEMENT_3D('',#104024,#81004,#81005) ;
#69447=AXIS2_PLACEMENT_3D('',#104025,#81006,#81007) ;
#69448=AXIS2_PLACEMENT_3D('',#104030,#81009,#81010) ;
#69449=AXIS2_PLACEMENT_3D('',#104034,#81012,#81013) ;
#69450=AXIS2_PLACEMENT_3D('',#104038,#81015,#81016) ;
#69451=AXIS2_PLACEMENT_3D('',#104042,#81018,#81019) ;
#69452=AXIS2_PLACEMENT_3D('',#104047,#81022,#81023) ;
#69453=AXIS2_PLACEMENT_3D('',#104049,#81024,#81025) ;
#69454=AXIS2_PLACEMENT_3D('',#104052,#81027,#81028) ;
#69455=AXIS2_PLACEMENT_3D('',#104054,#81029,#81030) ;
#69456=AXIS2_PLACEMENT_3D('',#104058,#81032,#81033) ;
#69457=AXIS2_PLACEMENT_3D('',#104062,#81035,#81036) ;
#69458=AXIS2_PLACEMENT_3D('',#104066,#81038,#81039) ;
#69459=AXIS2_PLACEMENT_3D('',#104070,#81041,#81042) ;
#69460=AXIS2_PLACEMENT_3D('',#104074,#81044,#81045) ;
#69461=AXIS2_PLACEMENT_3D('',#104078,#81047,#81048) ;
#69462=AXIS2_PLACEMENT_3D('',#104082,#81050,#81051) ;
#69463=AXIS2_PLACEMENT_3D('',#104085,#81053,#81054) ;
#69464=AXIS2_PLACEMENT_3D('',#104086,#81055,#81056) ;
#69465=AXIS2_PLACEMENT_3D('',#104089,#81059,#81060) ;
#69466=AXIS2_PLACEMENT_3D('',#104092,#81063,#81064) ;
#69467=AXIS2_PLACEMENT_3D('',#104181,#81069,#81070) ;
#69468=AXIS2_PLACEMENT_3D('',#104192,#81071,#81072) ;
#69469=AXIS2_PLACEMENT_3D('',#104197,#81076,#81077) ;
#69470=AXIS2_PLACEMENT_3D('',#104203,#81081,#81082) ;
#69471=AXIS2_PLACEMENT_3D('',#104223,#81086,#81087) ;
#69472=AXIS2_PLACEMENT_3D('',#104322,#81093,#81094) ;
#69473=AXIS2_PLACEMENT_3D('',#104326,#81096,#81097) ;
#69474=AXIS2_PLACEMENT_3D('',#104330,#81100,#81101) ;
#69475=AXIS2_PLACEMENT_3D('',#104333,#81102,#81103) ;
#69476=AXIS2_PLACEMENT_3D('',#104338,#81106,#81107) ;
#69477=AXIS2_PLACEMENT_3D('',#104340,#81108,#81109) ;
#69478=AXIS2_PLACEMENT_3D('',#104342,#81110,#81111) ;
#69479=AXIS2_PLACEMENT_3D('',#104350,#81115,#81116) ;
#69480=AXIS2_PLACEMENT_3D('',#104352,#81117,#81118) ;
#69481=AXIS2_PLACEMENT_3D('',#104354,#81119,#81120) ;
#69482=AXIS2_PLACEMENT_3D('',#104359,#81123,#81124) ;
#69483=AXIS2_PLACEMENT_3D('',#104361,#81125,#81126) ;
#69484=AXIS2_PLACEMENT_3D('',#104363,#81127,#81128) ;
#69485=AXIS2_PLACEMENT_3D('',#104367,#81130,#81131) ;
#69486=AXIS2_PLACEMENT_3D('',#104371,#81133,#81134) ;
#69487=AXIS2_PLACEMENT_3D('',#104372,#81135,#81136) ;
#69488=AXIS2_PLACEMENT_3D('',#104373,#81137,#81138) ;
#69489=AXIS2_PLACEMENT_3D('',#104376,#81139,#81140) ;
#69490=AXIS2_PLACEMENT_3D('',#104386,#81146,#81147) ;
#69491=AXIS2_PLACEMENT_3D('',#104388,#81149,#81150) ;
#69492=AXIS2_PLACEMENT_3D('',#104391,#81151,#81152) ;
#69493=AXIS2_PLACEMENT_3D('',#104397,#81156,#81157) ;
#69494=AXIS2_PLACEMENT_3D('',#104399,#81159,#81160) ;
#69495=AXIS2_PLACEMENT_3D('',#104405,#81163,#81164) ;
#69496=AXIS2_PLACEMENT_3D('',#104406,#81165,#81166) ;
#69497=AXIS2_PLACEMENT_3D('',#104409,#81167,#81168) ;
#69498=AXIS2_PLACEMENT_3D('',#104413,#81171,#81172) ;
#69499=AXIS2_PLACEMENT_3D('',#104430,#81181,#81182) ;
#69500=AXIS2_PLACEMENT_3D('',#104439,#81187,#81188) ;
#69501=AXIS2_PLACEMENT_3D('',#104448,#81193,#81194) ;
#69502=AXIS2_PLACEMENT_3D('',#104457,#81199,#81200) ;
#69503=AXIS2_PLACEMENT_3D('',#104484,#81205,#81206) ;
#69504=AXIS2_PLACEMENT_3D('',#104501,#81215,#81216) ;
#69505=AXIS2_PLACEMENT_3D('',#104506,#81218,#81219) ;
#69506=AXIS2_PLACEMENT_3D('',#104510,#81221,#81222) ;
#69507=AXIS2_PLACEMENT_3D('',#104514,#81224,#81225) ;
#69508=AXIS2_PLACEMENT_3D('',#104517,#81227,#81228) ;
#69509=AXIS2_PLACEMENT_3D('',#104518,#81229,#81230) ;
#69510=AXIS2_PLACEMENT_3D('',#104521,#81231,#81232) ;
#69511=AXIS2_PLACEMENT_3D('',#104526,#81235,#81236) ;
#69512=AXIS2_PLACEMENT_3D('',#104529,#81238,#81239) ;
#69513=AXIS2_PLACEMENT_3D('',#104530,#81240,#81241) ;
#69514=AXIS2_PLACEMENT_3D('',#104536,#81245,#81246) ;
#69515=AXIS2_PLACEMENT_3D('',#104542,#81250,#81251) ;
#69516=AXIS2_PLACEMENT_3D('',#104545,#81252,#81253) ;
#69517=AXIS2_PLACEMENT_3D('',#104549,#81255,#81256) ;
#69518=AXIS2_PLACEMENT_3D('',#104551,#81258,#81259) ;
#69519=AXIS2_PLACEMENT_3D('',#104554,#81260,#81261) ;
#69520=AXIS2_PLACEMENT_3D('',#104558,#81263,#81264) ;
#69521=AXIS2_PLACEMENT_3D('',#104560,#81266,#81267) ;
#69522=AXIS2_PLACEMENT_3D('',#104566,#81271,#81272) ;
#69523=AXIS2_PLACEMENT_3D('',#104572,#81276,#81277) ;
#69524=AXIS2_PLACEMENT_3D('',#104575,#81278,#81279) ;
#69525=AXIS2_PLACEMENT_3D('',#104580,#81282,#81283) ;
#69526=AXIS2_PLACEMENT_3D('',#104582,#81284,#81285) ;
#69527=AXIS2_PLACEMENT_3D('',#104584,#81287,#81288) ;
#69528=AXIS2_PLACEMENT_3D('',#104587,#81289,#81290) ;
#69529=AXIS2_PLACEMENT_3D('',#104592,#81294,#81295) ;
#69530=AXIS2_PLACEMENT_3D('',#104598,#81299,#81300) ;
#69531=AXIS2_PLACEMENT_3D('',#104601,#81301,#81302) ;
#69532=AXIS2_PLACEMENT_3D('',#104605,#81304,#81305) ;
#69533=AXIS2_PLACEMENT_3D('',#104607,#81307,#81308) ;
#69534=AXIS2_PLACEMENT_3D('',#104616,#81313,#81314) ;
#69535=AXIS2_PLACEMENT_3D('',#104619,#81315,#81316) ;
#69536=AXIS2_PLACEMENT_3D('',#104623,#81318,#81319) ;
#69537=AXIS2_PLACEMENT_3D('',#104625,#81321,#81322) ;
#69538=AXIS2_PLACEMENT_3D('',#104631,#81326,#81327) ;
#69539=AXIS2_PLACEMENT_3D('',#104640,#81332,#81333) ;
#69540=AXIS2_PLACEMENT_3D('',#104647,#81337,#81338) ;
#69541=AXIS2_PLACEMENT_3D('',#104648,#81339,#81340) ;
#69542=AXIS2_PLACEMENT_3D('',#104657,#81345,#81346) ;
#69543=AXIS2_PLACEMENT_3D('',#104660,#81347,#81348) ;
#69544=AXIS2_PLACEMENT_3D('',#104665,#81351,#81352) ;
#69545=AXIS2_PLACEMENT_3D('',#104669,#81354,#81355) ;
#69546=AXIS2_PLACEMENT_3D('',#104671,#81357,#81358) ;
#69547=AXIS2_PLACEMENT_3D('',#104679,#81363,#81364) ;
#69548=AXIS2_PLACEMENT_3D('',#104688,#81369,#81370) ;
#69549=AXIS2_PLACEMENT_3D('',#104697,#81375,#81376) ;
#69550=AXIS2_PLACEMENT_3D('',#104706,#81381,#81382) ;
#69551=AXIS2_PLACEMENT_3D('',#104712,#81386,#81387) ;
#69552=AXIS2_PLACEMENT_3D('',#104718,#81391,#81392) ;
#69553=AXIS2_PLACEMENT_3D('',#104724,#81396,#81397) ;
#69554=AXIS2_PLACEMENT_3D('',#104730,#81401,#81402) ;
#69555=AXIS2_PLACEMENT_3D('',#104739,#81406,#81407) ;
#69556=AXIS2_PLACEMENT_3D('',#104742,#81409,#81410) ;
#69557=AXIS2_PLACEMENT_3D('',#104743,#81411,#81412) ;
#69558=AXIS2_PLACEMENT_3D('',#104752,#81416,#81417) ;
#69559=AXIS2_PLACEMENT_3D('',#104755,#81419,#81420) ;
#69560=AXIS2_PLACEMENT_3D('',#104756,#81421,#81422) ;
#69561=AXIS2_PLACEMENT_3D('',#104760,#81424,#81425) ;
#69562=AXIS2_PLACEMENT_3D('',#104761,#81426,#81427) ;
#69563=AXIS2_PLACEMENT_3D('',#104762,#81428,#81429) ;
#69564=AXIS2_PLACEMENT_3D('',#104768,#81433,#81434) ;
#69565=AXIS2_PLACEMENT_3D('',#104777,#81439,#81440) ;
#69566=AXIS2_PLACEMENT_3D('',#104786,#81445,#81446) ;
#69567=AXIS2_PLACEMENT_3D('',#104795,#81451,#81452) ;
#69568=AXIS2_PLACEMENT_3D('',#104804,#81457,#81458) ;
#69569=AXIS2_PLACEMENT_3D('',#104805,#81459,#81460) ;
#69570=AXIS2_PLACEMENT_3D('',#104806,#81461,#81462) ;
#69571=AXIS2_PLACEMENT_3D('',#104807,#81463,#81464) ;
#69572=AXIS2_PLACEMENT_3D('',#104816,#81469,#81470) ;
#69573=AXIS2_PLACEMENT_3D('',#104825,#81475,#81476) ;
#69574=AXIS2_PLACEMENT_3D('',#104834,#81481,#81482) ;
#69575=AXIS2_PLACEMENT_3D('',#104843,#81487,#81488) ;
#69576=AXIS2_PLACEMENT_3D('',#104847,#81490,#81491) ;
#69577=AXIS2_PLACEMENT_3D('',#104849,#81493,#81494) ;
#69578=AXIS2_PLACEMENT_3D('',#104852,#81495,#81496) ;
#69579=AXIS2_PLACEMENT_3D('',#104853,#81497,#81498) ;
#69580=AXIS2_PLACEMENT_3D('',#104854,#81499,#81500) ;
#69581=AXIS2_PLACEMENT_3D('',#104855,#81501,#81502) ;
#69582=AXIS2_PLACEMENT_3D('',#104859,#81504,#81505) ;
#69583=AXIS2_PLACEMENT_3D('',#104861,#81507,#81508) ;
#69584=AXIS2_PLACEMENT_3D('',#104862,#81509,#81510) ;
#69585=AXIS2_PLACEMENT_3D('',#104863,#81511,#81512) ;
#69586=AXIS2_PLACEMENT_3D('',#104864,#81513,#81514) ;
#69587=AXIS2_PLACEMENT_3D('',#104865,#81515,#81516) ;
#69588=AXIS2_PLACEMENT_3D('',#104866,#81517,#81518) ;
#69589=AXIS2_PLACEMENT_3D('',#104867,#81519,#81520) ;
#69590=AXIS2_PLACEMENT_3D('',#104868,#81521,#81522) ;
#69591=AXIS2_PLACEMENT_3D('',#104869,#81523,#81524) ;
#69592=AXIS2_PLACEMENT_3D('',#104870,#81525,#81526) ;
#69593=AXIS2_PLACEMENT_3D('',#104871,#81527,#81528) ;
#69594=AXIS2_PLACEMENT_3D('',#104872,#81529,#81530) ;
#69595=AXIS2_PLACEMENT_3D('',#104873,#81531,#81532) ;
#69596=AXIS2_PLACEMENT_3D('',#104874,#81533,#81534) ;
#69597=AXIS2_PLACEMENT_3D('',#104875,#81535,#81536) ;
#69598=AXIS2_PLACEMENT_3D('',#104876,#81537,#81538) ;
#69599=AXIS2_PLACEMENT_3D('',#104877,#81539,#81540) ;
#69600=AXIS2_PLACEMENT_3D('',#104878,#81541,#81542) ;
#69601=AXIS2_PLACEMENT_3D('',#104879,#81543,#81544) ;
#69602=AXIS2_PLACEMENT_3D('',#104880,#81545,#81546) ;
#69603=AXIS2_PLACEMENT_3D('',#104881,#81547,#81548) ;
#69604=AXIS2_PLACEMENT_3D('',#104882,#81549,#81550) ;
#69605=AXIS2_PLACEMENT_3D('',#104883,#81551,#81552) ;
#69606=AXIS2_PLACEMENT_3D('',#104884,#81553,#81554) ;
#69607=AXIS2_PLACEMENT_3D('',#104885,#81555,#81556) ;
#69608=AXIS2_PLACEMENT_3D('',#104886,#81557,#81558) ;
#69609=AXIS2_PLACEMENT_3D('',#104887,#81559,#81560) ;
#69610=AXIS2_PLACEMENT_3D('',#104888,#81561,#81562) ;
#69611=AXIS2_PLACEMENT_3D('',#104889,#81563,#81564) ;
#69612=AXIS2_PLACEMENT_3D('',#104890,#81565,#81566) ;
#69613=AXIS2_PLACEMENT_3D('',#104891,#81567,#81568) ;
#69614=AXIS2_PLACEMENT_3D('',#104892,#81569,#81570) ;
#69615=AXIS2_PLACEMENT_3D('',#104893,#81571,#81572) ;
#69616=AXIS2_PLACEMENT_3D('',#104894,#81573,#81574) ;
#69617=AXIS2_PLACEMENT_3D('',#104895,#81575,#81576) ;
#69618=AXIS2_PLACEMENT_3D('',#104896,#81577,#81578) ;
#69619=AXIS2_PLACEMENT_3D('',#104897,#81579,#81580) ;
#69620=AXIS2_PLACEMENT_3D('',#104898,#81581,#81582) ;
#69621=AXIS2_PLACEMENT_3D('',#104899,#81583,#81584) ;
#69622=AXIS2_PLACEMENT_3D('',#104900,#81585,#81586) ;
#69623=AXIS2_PLACEMENT_3D('',#104901,#81587,#81588) ;
#69624=AXIS2_PLACEMENT_3D('',#104902,#81589,#81590) ;
#69625=AXIS2_PLACEMENT_3D('',#104903,#81591,#81592) ;
#69626=AXIS2_PLACEMENT_3D('',#104904,#81593,#81594) ;
#69627=AXIS2_PLACEMENT_3D('',#104905,#81595,#81596) ;
#69628=AXIS2_PLACEMENT_3D('',#104906,#81597,#81598) ;
#69629=AXIS2_PLACEMENT_3D('',#104907,#81599,#81600) ;
#69630=AXIS2_PLACEMENT_3D('',#104908,#81601,#81602) ;
#69631=AXIS2_PLACEMENT_3D('',#104909,#81603,#81604) ;
#69632=AXIS2_PLACEMENT_3D('',#104910,#81605,#81606) ;
#69633=AXIS2_PLACEMENT_3D('',#104911,#81607,#81608) ;
#69634=AXIS2_PLACEMENT_3D('',#104912,#81609,#81610) ;
#69635=AXIS2_PLACEMENT_3D('',#104913,#81611,#81612) ;
#69636=AXIS2_PLACEMENT_3D('',#104914,#81613,#81614) ;
#69637=AXIS2_PLACEMENT_3D('',#104915,#81615,#81616) ;
#69638=AXIS2_PLACEMENT_3D('',#104916,#81617,#81618) ;
#69639=AXIS2_PLACEMENT_3D('',#104917,#81619,#81620) ;
#69640=AXIS2_PLACEMENT_3D('',#104918,#81621,#81622) ;
#69641=AXIS2_PLACEMENT_3D('',#104919,#81623,#81624) ;
#69642=AXIS2_PLACEMENT_3D('',#104920,#81625,#81626) ;
#69643=AXIS2_PLACEMENT_3D('',#104921,#81627,#81628) ;
#69644=AXIS2_PLACEMENT_3D('',#104922,#81629,#81630) ;
#69645=AXIS2_PLACEMENT_3D('',#104923,#81631,#81632) ;
#69646=AXIS2_PLACEMENT_3D('',#104924,#81633,#81634) ;
#69647=AXIS2_PLACEMENT_3D('',#104925,#81635,#81636) ;
#69648=AXIS2_PLACEMENT_3D('',#104926,#81637,#81638) ;
#69649=AXIS2_PLACEMENT_3D('',#104927,#81639,#81640) ;
#69650=AXIS2_PLACEMENT_3D('',#104928,#81641,#81642) ;
#69651=AXIS2_PLACEMENT_3D('',#104929,#81643,#81644) ;
#69652=AXIS2_PLACEMENT_3D('',#104930,#81645,#81646) ;
#69653=AXIS2_PLACEMENT_3D('',#104931,#81647,#81648) ;
#69654=AXIS2_PLACEMENT_3D('',#104932,#81649,#81650) ;
#69655=AXIS2_PLACEMENT_3D('',#104933,#81651,#81652) ;
#69656=AXIS2_PLACEMENT_3D('',#104934,#81653,#81654) ;
#69657=AXIS2_PLACEMENT_3D('',#104950,#81655,#81656) ;
#69658=AXIS2_PLACEMENT_3D('',#104951,#81657,#81658) ;
#69659=AXIS2_PLACEMENT_3D('',#104953,#81659,#81660) ;
#69660=AXIS2_PLACEMENT_3D('',#104968,#81661,#81662) ;
#69661=AXIS2_PLACEMENT_3D('',#104969,#81663,#81664) ;
#69662=AXIS2_PLACEMENT_3D('',#104970,#81665,#81666) ;
#69663=AXIS2_PLACEMENT_3D('',#104972,#81667,#81668) ;
#69664=AXIS2_PLACEMENT_3D('',#105002,#81669,#81670) ;
#69665=AXIS2_PLACEMENT_3D('',#105003,#81671,#81672) ;
#69666=AXIS2_PLACEMENT_3D('',#105019,#81673,#81674) ;
#69667=AXIS2_PLACEMENT_3D('',#105021,#81675,#81676) ;
#69668=AXIS2_PLACEMENT_3D('',#105036,#81677,#81678) ;
#69669=AXIS2_PLACEMENT_3D('',#105037,#81679,#81680) ;
#69670=AXIS2_PLACEMENT_3D('',#105038,#81681,#81682) ;
#69671=AXIS2_PLACEMENT_3D('',#105039,#81683,#81684) ;
#69672=AXIS2_PLACEMENT_3D('',#105042,#81686,#81687) ;
#69673=AXIS2_PLACEMENT_3D('',#105043,#81688,#81689) ;
#69674=AXIS2_PLACEMENT_3D('',#105045,#81690,#81691) ;
#69675=AXIS2_PLACEMENT_3D('',#105046,#81692,#81693) ;
#69676=AXIS2_PLACEMENT_3D('',#105047,#81694,#81695) ;
#69677=AXIS2_PLACEMENT_3D('',#105049,#81696,#81697) ;
#69678=AXIS2_PLACEMENT_3D('',#105064,#81698,#81699) ;
#69679=AXIS2_PLACEMENT_3D('',#105065,#81700,#81701) ;
#69680=AXIS2_PLACEMENT_3D('',#105081,#81702,#81703) ;
#69681=AXIS2_PLACEMENT_3D('',#105082,#81704,#81705) ;
#69682=AXIS2_PLACEMENT_3D('',#105083,#81706,#81707) ;
#69683=AXIS2_PLACEMENT_3D('',#105085,#81708,#81709) ;
#69684=AXIS2_PLACEMENT_3D('',#105087,#81711,#81712) ;
#69685=AXIS2_PLACEMENT_3D('',#105088,#81713,#81714) ;
#69686=AXIS2_PLACEMENT_3D('',#105089,#81715,#81716) ;
#69687=AXIS2_PLACEMENT_3D('',#105090,#81717,#81718) ;
#69688=AXIS2_PLACEMENT_3D('',#105091,#81719,#81720) ;
#69689=AXIS2_PLACEMENT_3D('',#105092,#81721,#81722) ;
#69690=AXIS2_PLACEMENT_3D('',#105095,#81724,#81725) ;
#69691=AXIS2_PLACEMENT_3D('',#105096,#81726,#81727) ;
#69692=AXIS2_PLACEMENT_3D('',#105097,#81728,#81729) ;
#69693=AXIS2_PLACEMENT_3D('',#105098,#81730,#81731) ;
#69694=AXIS2_PLACEMENT_3D('',#105100,#81732,#81733) ;
#69695=AXIS2_PLACEMENT_3D('',#105101,#81734,#81735) ;
#69696=AXIS2_PLACEMENT_3D('',#105102,#81736,#81737) ;
#69697=AXIS2_PLACEMENT_3D('',#105103,#81738,#81739) ;
#69698=AXIS2_PLACEMENT_3D('',#105104,#81740,#81741) ;
#69699=AXIS2_PLACEMENT_3D('',#105105,#81742,#81743) ;
#69700=AXIS2_PLACEMENT_3D('',#105106,#81744,#81745) ;
#69701=AXIS2_PLACEMENT_3D('',#105108,#81746,#81747) ;
#69702=AXIS2_PLACEMENT_3D('',#105109,#81748,#81749) ;
#69703=AXIS2_PLACEMENT_3D('',#105110,#81750,#81751) ;
#69704=AXIS2_PLACEMENT_3D('',#105111,#81752,#81753) ;
#69705=AXIS2_PLACEMENT_3D('',#105112,#81754,#81755) ;
#69706=AXIS2_PLACEMENT_3D('',#105114,#81756,#81757) ;
#69707=AXIS2_PLACEMENT_3D('',#105116,#81759,#81760) ;
#69708=AXIS2_PLACEMENT_3D('',#105117,#81761,#81762) ;
#69709=AXIS2_PLACEMENT_3D('',#105118,#81763,#81764) ;
#69710=AXIS2_PLACEMENT_3D('',#105119,#81765,#81766) ;
#69711=AXIS2_PLACEMENT_3D('',#105120,#81767,#81768) ;
#69712=AXIS2_PLACEMENT_3D('',#105122,#81770,#81771) ;
#69713=AXIS2_PLACEMENT_3D('',#105123,#81772,#81773) ;
#69714=AXIS2_PLACEMENT_3D('',#105124,#81774,#81775) ;
#69715=AXIS2_PLACEMENT_3D('',#105125,#81776,#81777) ;
#69716=AXIS2_PLACEMENT_3D('',#105127,#81778,#81779) ;
#69717=AXIS2_PLACEMENT_3D('',#105128,#81780,#81781) ;
#69718=AXIS2_PLACEMENT_3D('',#105129,#81782,#81783) ;
#69719=AXIS2_PLACEMENT_3D('',#105130,#81784,#81785) ;
#69720=AXIS2_PLACEMENT_3D('',#105131,#81786,#81787) ;
#69721=AXIS2_PLACEMENT_3D('',#105132,#81788,#81789) ;
#69722=AXIS2_PLACEMENT_3D('',#105133,#81790,#81791) ;
#69723=AXIS2_PLACEMENT_3D('',#105135,#81793,#81794) ;
#69724=AXIS2_PLACEMENT_3D('',#105136,#81795,#81796) ;
#69725=AXIS2_PLACEMENT_3D('',#105137,#81797,#81798) ;
#69726=AXIS2_PLACEMENT_3D('',#105138,#81799,#81800) ;
#69727=AXIS2_PLACEMENT_3D('',#105139,#81801,#81802) ;
#69728=AXIS2_PLACEMENT_3D('',#105140,#81803,#81804) ;
#69729=AXIS2_PLACEMENT_3D('',#105141,#81805,#81806) ;
#69730=AXIS2_PLACEMENT_3D('',#105142,#81807,#81808) ;
#69731=AXIS2_PLACEMENT_3D('',#105143,#81809,#81810) ;
#69732=AXIS2_PLACEMENT_3D('',#105144,#81811,#81812) ;
#69733=AXIS2_PLACEMENT_3D('',#105145,#81813,#81814) ;
#69734=AXIS2_PLACEMENT_3D('',#105146,#81815,#81816) ;
#69735=AXIS2_PLACEMENT_3D('',#105147,#81817,#81818) ;
#69736=AXIS2_PLACEMENT_3D('',#105148,#81819,#81820) ;
#69737=AXIS2_PLACEMENT_3D('',#105149,#81821,#81822) ;
#69738=AXIS2_PLACEMENT_3D('',#105150,#81823,#81824) ;
#69739=AXIS2_PLACEMENT_3D('',#105151,#81825,#81826) ;
#69740=AXIS2_PLACEMENT_3D('',#105152,#81827,#81828) ;
#69741=AXIS2_PLACEMENT_3D('',#105153,#81829,#81830) ;
#69742=AXIS2_PLACEMENT_3D('',#105154,#81831,#81832) ;
#69743=AXIS2_PLACEMENT_3D('',#105155,#81833,#81834) ;
#69744=AXIS2_PLACEMENT_3D('',#105156,#81835,#81836) ;
#69745=AXIS2_PLACEMENT_3D('',#105157,#81837,#81838) ;
#69746=AXIS2_PLACEMENT_3D('',#105158,#81839,#81840) ;
#69747=AXIS2_PLACEMENT_3D('',#105159,#81841,#81842) ;
#69748=AXIS2_PLACEMENT_3D('',#105160,#81843,#81844) ;
#69749=AXIS2_PLACEMENT_3D('',#105161,#81845,#81846) ;
#69750=AXIS2_PLACEMENT_3D('',#105162,#81847,#81848) ;
#69751=AXIS2_PLACEMENT_3D('',#105163,#81849,#81850) ;
#69752=AXIS2_PLACEMENT_3D('',#105164,#81851,#81852) ;
#69753=AXIS2_PLACEMENT_3D('',#105165,#81853,#81854) ;
#69754=AXIS2_PLACEMENT_3D('',#105166,#81855,#81856) ;
#69755=AXIS2_PLACEMENT_3D('',#105167,#81857,#81858) ;
#69756=AXIS2_PLACEMENT_3D('',#105168,#81859,#81860) ;
#69757=AXIS2_PLACEMENT_3D('',#105169,#81861,#81862) ;
#69758=AXIS2_PLACEMENT_3D('',#105170,#81863,#81864) ;
#69759=AXIS2_PLACEMENT_3D('',#105171,#81865,#81866) ;
#69760=AXIS2_PLACEMENT_3D('',#105172,#81867,#81868) ;
#69761=AXIS2_PLACEMENT_3D('',#105173,#81869,#81870) ;
#69762=AXIS2_PLACEMENT_3D('',#105174,#81871,#81872) ;
#69763=AXIS2_PLACEMENT_3D('',#105175,#81873,#81874) ;
#69764=AXIS2_PLACEMENT_3D('',#105176,#81875,#81876) ;
#69765=AXIS2_PLACEMENT_3D('',#105177,#81877,#81878) ;
#69766=AXIS2_PLACEMENT_3D('',#105178,#81879,#81880) ;
#69767=AXIS2_PLACEMENT_3D('',#105179,#81881,#81882) ;
#69768=AXIS2_PLACEMENT_3D('',#105180,#81883,#81884) ;
#69769=AXIS2_PLACEMENT_3D('',#105181,#81885,#81886) ;
#69770=AXIS2_PLACEMENT_3D('',#105182,#81887,#81888) ;
#69771=AXIS2_PLACEMENT_3D('',#105183,#81889,#81890) ;
#69772=AXIS2_PLACEMENT_3D('',#105184,#81891,#81892) ;
#69773=AXIS2_PLACEMENT_3D('',#105201,#81893,#81894) ;
#69774=AXIS2_PLACEMENT_3D('',#105202,#81895,#81896) ;
#69775=AXIS2_PLACEMENT_3D('',#105203,#81897,#81898) ;
#69776=AXIS2_PLACEMENT_3D('',#105204,#81899,#81900) ;
#69777=AXIS2_PLACEMENT_3D('',#105205,#81901,#81902) ;
#69778=AXIS2_PLACEMENT_3D('',#105206,#81903,#81904) ;
#69779=AXIS2_PLACEMENT_3D('',#105207,#81905,#81906) ;
#69780=AXIS2_PLACEMENT_3D('',#105208,#81907,#81908) ;
#69781=AXIS2_PLACEMENT_3D('',#105209,#81909,#81910) ;
#69782=AXIS2_PLACEMENT_3D('',#105210,#81911,#81912) ;
#69783=AXIS2_PLACEMENT_3D('',#105211,#81913,#81914) ;
#69784=AXIS2_PLACEMENT_3D('',#105230,#81915,#81916) ;
#69785=AXIS2_PLACEMENT_3D('',#105231,#81917,#81918) ;
#69786=AXIS2_PLACEMENT_3D('',#105233,#81919,#81920) ;
#69787=AXIS2_PLACEMENT_3D('',#105234,#81921,#81922) ;
#69788=AXIS2_PLACEMENT_3D('',#105235,#81923,#81924) ;
#69789=AXIS2_PLACEMENT_3D('',#105236,#81925,#81926) ;
#69790=AXIS2_PLACEMENT_3D('',#105237,#81927,#81928) ;
#69791=AXIS2_PLACEMENT_3D('',#105238,#81929,#81930) ;
#69792=AXIS2_PLACEMENT_3D('',#105239,#81931,#81932) ;
#69793=AXIS2_PLACEMENT_3D('',#105240,#81933,#81934) ;
#69794=AXIS2_PLACEMENT_3D('',#105241,#81935,#81936) ;
#69795=AXIS2_PLACEMENT_3D('',#105242,#81937,#81938) ;
#69796=AXIS2_PLACEMENT_3D('',#105243,#81939,#81940) ;
#69797=AXIS2_PLACEMENT_3D('',#105278,#81941,#81942) ;
#69798=AXIS2_PLACEMENT_3D('',#105279,#81943,#81944) ;
#69799=AXIS2_PLACEMENT_3D('',#105280,#81945,#81946) ;
#69800=AXIS2_PLACEMENT_3D('',#105281,#81947,#81948) ;
#69801=AXIS2_PLACEMENT_3D('',#105292,#81949,#81950) ;
#69802=AXIS2_PLACEMENT_3D('',#105293,#81951,#81952) ;
#69803=AXIS2_PLACEMENT_3D('',#105294,#81953,#81954) ;
#69804=AXIS2_PLACEMENT_3D('',#105295,#81955,#81956) ;
#69805=AXIS2_PLACEMENT_3D('',#105302,#81957,#81958) ;
#69806=AXIS2_PLACEMENT_3D('',#105303,#81959,#81960) ;
#69807=AXIS2_PLACEMENT_3D('',#105304,#81961,#81962) ;
#69808=AXIS2_PLACEMENT_3D('',#105305,#81963,#81964) ;
#69809=AXIS2_PLACEMENT_3D('',#105306,#81965,#81966) ;
#69810=AXIS2_PLACEMENT_3D('',#105317,#81967,#81968) ;
#69811=AXIS2_PLACEMENT_3D('',#105318,#81969,#81970) ;
#69812=AXIS2_PLACEMENT_3D('',#105319,#81971,#81972) ;
#69813=AXIS2_PLACEMENT_3D('',#105320,#81973,#81974) ;
#69814=AXIS2_PLACEMENT_3D('',#105321,#81975,#81976) ;
#69815=AXIS2_PLACEMENT_3D('',#105322,#81977,#81978) ;
#69816=AXIS2_PLACEMENT_3D('',#105323,#81979,#81980) ;
#69817=AXIS2_PLACEMENT_3D('',#105324,#81981,#81982) ;
#69818=AXIS2_PLACEMENT_3D('',#105325,#81983,#81984) ;
#69819=AXIS2_PLACEMENT_3D('',#105326,#81985,#81986) ;
#69820=AXIS2_PLACEMENT_3D('',#105327,#81987,#81988) ;
#69821=AXIS2_PLACEMENT_3D('',#105328,#81989,#81990) ;
#69822=AXIS2_PLACEMENT_3D('',#105329,#81991,#81992) ;
#69823=AXIS2_PLACEMENT_3D('',#105330,#81993,#81994) ;
#69824=AXIS2_PLACEMENT_3D('',#105331,#81995,#81996) ;
#69825=AXIS2_PLACEMENT_3D('',#105332,#81997,#81998) ;
#69826=AXIS2_PLACEMENT_3D('',#105333,#81999,#82000) ;
#69827=AXIS2_PLACEMENT_3D('',#105334,#82001,#82002) ;
#69828=AXIS2_PLACEMENT_3D('',#105335,#82003,#82004) ;
#69829=AXIS2_PLACEMENT_3D('',#105336,#82005,#82006) ;
#69830=AXIS2_PLACEMENT_3D('',#105337,#82007,#82008) ;
#69831=AXIS2_PLACEMENT_3D('',#105338,#82009,#82010) ;
#69832=AXIS2_PLACEMENT_3D('',#105339,#82011,#82012) ;
#69833=AXIS2_PLACEMENT_3D('',#105340,#82013,#82014) ;
#69834=AXIS2_PLACEMENT_3D('',#105341,#82015,#82016) ;
#69835=AXIS2_PLACEMENT_3D('',#105342,#82017,#82018) ;
#69836=AXIS2_PLACEMENT_3D('',#105343,#82019,#82020) ;
#69837=AXIS2_PLACEMENT_3D('',#105344,#82021,#82022) ;
#69838=AXIS2_PLACEMENT_3D('',#105345,#82023,#82024) ;
#69839=AXIS2_PLACEMENT_3D('',#105346,#82025,#82026) ;
#69840=AXIS2_PLACEMENT_3D('',#105347,#82027,#82028) ;
#69841=AXIS2_PLACEMENT_3D('',#105348,#82029,#82030) ;
#69842=AXIS2_PLACEMENT_3D('',#105349,#82031,#82032) ;
#69843=AXIS2_PLACEMENT_3D('',#105350,#82033,#82034) ;
#69844=AXIS2_PLACEMENT_3D('',#105357,#82035,#82036) ;
#69845=AXIS2_PLACEMENT_3D('',#105358,#82037,#82038) ;
#69846=AXIS2_PLACEMENT_3D('',#105359,#82039,#82040) ;
#69847=AXIS2_PLACEMENT_3D('',#105360,#82041,#82042) ;
#69848=AXIS2_PLACEMENT_3D('',#105361,#82043,#82044) ;
#69849=AXIS2_PLACEMENT_3D('',#105362,#82045,#82046) ;
#69850=AXIS2_PLACEMENT_3D('',#105363,#82047,#82048) ;
#69851=AXIS2_PLACEMENT_3D('',#105364,#82049,#82050) ;
#69852=AXIS2_PLACEMENT_3D('',#105365,#82051,#82052) ;
#69853=AXIS2_PLACEMENT_3D('',#105366,#82053,#82054) ;
#69854=AXIS2_PLACEMENT_3D('',#105367,#82055,#82056) ;
#69855=AXIS2_PLACEMENT_3D('',#105368,#82057,#82058) ;
#69856=AXIS2_PLACEMENT_3D('',#105369,#82059,#82060) ;
#69857=AXIS2_PLACEMENT_3D('',#105370,#82061,#82062) ;
#69858=AXIS2_PLACEMENT_3D('',#105371,#82063,#82064) ;
#69859=AXIS2_PLACEMENT_3D('',#105372,#82065,#82066) ;
#69860=AXIS2_PLACEMENT_3D('',#105373,#82067,#82068) ;
#69861=AXIS2_PLACEMENT_3D('',#105374,#82069,#82070) ;
#69862=AXIS2_PLACEMENT_3D('',#105375,#82071,#82072) ;
#69863=AXIS2_PLACEMENT_3D('',#105376,#82073,#82074) ;
#69864=AXIS2_PLACEMENT_3D('',#105377,#82075,#82076) ;
#69865=AXIS2_PLACEMENT_3D('',#105378,#82077,#82078) ;
#69866=AXIS2_PLACEMENT_3D('',#105379,#82079,#82080) ;
#69867=AXIS2_PLACEMENT_3D('',#105380,#82081,#82082) ;
#69868=AXIS2_PLACEMENT_3D('',#105381,#82083,#82084) ;
#69869=AXIS2_PLACEMENT_3D('',#105382,#82085,#82086) ;
#69870=AXIS2_PLACEMENT_3D('',#105383,#82087,#82088) ;
#69871=AXIS2_PLACEMENT_3D('',#105384,#82089,#82090) ;
#69872=AXIS2_PLACEMENT_3D('',#105385,#82091,#82092) ;
#69873=AXIS2_PLACEMENT_3D('',#105386,#82093,#82094) ;
#69874=AXIS2_PLACEMENT_3D('',#105387,#82095,#82096) ;
#69875=AXIS2_PLACEMENT_3D('',#105388,#82097,#82098) ;
#69876=AXIS2_PLACEMENT_3D('',#105389,#82099,#82100) ;
#69877=AXIS2_PLACEMENT_3D('',#105390,#82101,#82102) ;
#69878=AXIS2_PLACEMENT_3D('',#105391,#82103,#82104) ;
#69879=AXIS2_PLACEMENT_3D('',#105392,#82105,#82106) ;
#69880=AXIS2_PLACEMENT_3D('',#105393,#82107,#82108) ;
#69881=AXIS2_PLACEMENT_3D('',#105394,#82109,#82110) ;
#69882=AXIS2_PLACEMENT_3D('',#105395,#82111,#82112) ;
#69883=AXIS2_PLACEMENT_3D('',#105426,#82113,#82114) ;
#69884=AXIS2_PLACEMENT_3D('',#105427,#82115,#82116) ;
#69885=AXIS2_PLACEMENT_3D('',#105428,#82117,#82118) ;
#69886=AXIS2_PLACEMENT_3D('',#105429,#82119,#82120) ;
#69887=AXIS2_PLACEMENT_3D('',#105430,#82121,#82122) ;
#69888=AXIS2_PLACEMENT_3D('',#105431,#82123,#82124) ;
#69889=AXIS2_PLACEMENT_3D('',#105432,#82125,#82126) ;
#69890=AXIS2_PLACEMENT_3D('',#105433,#82127,#82128) ;
#69891=AXIS2_PLACEMENT_3D('',#105434,#82129,#82130) ;
#69892=AXIS2_PLACEMENT_3D('',#105435,#82131,#82132) ;
#69893=AXIS2_PLACEMENT_3D('',#105462,#82133,#82134) ;
#69894=AXIS2_PLACEMENT_3D('',#105463,#82135,#82136) ;
#69895=AXIS2_PLACEMENT_3D('',#105464,#82137,#82138) ;
#69896=AXIS2_PLACEMENT_3D('',#105465,#82139,#82140) ;
#69897=AXIS2_PLACEMENT_3D('',#105466,#82141,#82142) ;
#69898=AXIS2_PLACEMENT_3D('',#105467,#82143,#82144) ;
#69899=AXIS2_PLACEMENT_3D('',#105468,#82145,#82146) ;
#69900=AXIS2_PLACEMENT_3D('',#105469,#82147,#82148) ;
#69901=AXIS2_PLACEMENT_3D('',#105470,#82149,#82150) ;
#69902=AXIS2_PLACEMENT_3D('',#105471,#82151,#82152) ;
#69903=AXIS2_PLACEMENT_3D('',#105472,#82153,#82154) ;
#69904=AXIS2_PLACEMENT_3D('',#105473,#82155,#82156) ;
#69905=AXIS2_PLACEMENT_3D('',#105474,#82157,#82158) ;
#69906=AXIS2_PLACEMENT_3D('',#105475,#82159,#82160) ;
#69907=AXIS2_PLACEMENT_3D('',#105476,#82161,#82162) ;
#69908=AXIS2_PLACEMENT_3D('',#105477,#82163,#82164) ;
#69909=AXIS2_PLACEMENT_3D('',#105478,#82165,#82166) ;
#69910=AXIS2_PLACEMENT_3D('',#105479,#82167,#82168) ;
#69911=AXIS2_PLACEMENT_3D('',#105480,#82169,#82170) ;
#69912=AXIS2_PLACEMENT_3D('',#105481,#82171,#82172) ;
#69913=AXIS2_PLACEMENT_3D('',#105482,#82173,#82174) ;
#69914=AXIS2_PLACEMENT_3D('',#105483,#82175,#82176) ;
#69915=AXIS2_PLACEMENT_3D('',#105484,#82177,#82178) ;
#69916=AXIS2_PLACEMENT_3D('',#105485,#82179,#82180) ;
#69917=AXIS2_PLACEMENT_3D('',#105486,#82181,#82182) ;
#69918=AXIS2_PLACEMENT_3D('',#105487,#82183,#82184) ;
#69919=AXIS2_PLACEMENT_3D('',#105488,#82185,#82186) ;
#69920=AXIS2_PLACEMENT_3D('',#105489,#82187,#82188) ;
#69921=AXIS2_PLACEMENT_3D('',#105490,#82189,#82190) ;
#69922=AXIS2_PLACEMENT_3D('',#105515,#82191,#82192) ;
#69923=AXIS2_PLACEMENT_3D('',#105516,#82193,#82194) ;
#69924=AXIS2_PLACEMENT_3D('',#105517,#82195,#82196) ;
#69925=AXIS2_PLACEMENT_3D('',#105518,#82197,#82198) ;
#69926=AXIS2_PLACEMENT_3D('',#105519,#82199,#82200) ;
#69927=AXIS2_PLACEMENT_3D('',#105520,#82201,#82202) ;
#69928=AXIS2_PLACEMENT_3D('',#105521,#82203,#82204) ;
#69929=AXIS2_PLACEMENT_3D('',#105570,#82205,#82206) ;
#69930=AXIS2_PLACEMENT_3D('',#105571,#82207,#82208) ;
#69931=AXIS2_PLACEMENT_3D('',#105572,#82209,#82210) ;
#69932=AXIS2_PLACEMENT_3D('',#105573,#82211,#82212) ;
#69933=AXIS2_PLACEMENT_3D('',#105574,#82213,#82214) ;
#69934=AXIS2_PLACEMENT_3D('',#105575,#82215,#82216) ;
#69935=AXIS2_PLACEMENT_3D('',#105576,#82217,#82218) ;
#69936=AXIS2_PLACEMENT_3D('',#105638,#82219,#82220) ;
#69937=AXIS2_PLACEMENT_3D('',#105639,#82221,#82222) ;
#69938=AXIS2_PLACEMENT_3D('',#105640,#82223,#82224) ;
#69939=AXIS2_PLACEMENT_3D('',#105813,#82225,#82226) ;
#69940=AXIS2_PLACEMENT_3D('',#105814,#82227,#82228) ;
#69941=AXIS2_PLACEMENT_3D('',#105869,#82229,#82230) ;
#69942=AXIS2_PLACEMENT_3D('',#105916,#82231,#82232) ;
#69943=AXIS2_PLACEMENT_3D('',#105917,#82233,#82234) ;
#69944=AXIS2_PLACEMENT_3D('',#105918,#82235,#82236) ;
#69945=AXIS2_PLACEMENT_3D('',#105919,#82237,#82238) ;
#69946=AXIS2_PLACEMENT_3D('',#105920,#82239,#82240) ;
#69947=AXIS2_PLACEMENT_3D('',#105921,#82241,#82242) ;
#69948=AXIS2_PLACEMENT_3D('',#106026,#82243,#82244) ;
#69949=AXIS2_PLACEMENT_3D('',#106027,#82245,#82246) ;
#69950=AXIS2_PLACEMENT_3D('',#106028,#82247,#82248) ;
#69951=AXIS2_PLACEMENT_3D('',#106029,#82249,#82250) ;
#69952=AXIS2_PLACEMENT_3D('',#106042,#82251,#82252) ;
#69953=AXIS2_PLACEMENT_3D('',#106043,#82253,#82254) ;
#69954=AXIS2_PLACEMENT_3D('',#106044,#82255,#82256) ;
#69955=AXIS2_PLACEMENT_3D('',#106045,#82257,#82258) ;
#69956=AXIS2_PLACEMENT_3D('',#106046,#82259,#82260) ;
#69957=AXIS2_PLACEMENT_3D('',#106047,#82261,#82262) ;
#69958=AXIS2_PLACEMENT_3D('',#106048,#82263,#82264) ;
#69959=AXIS2_PLACEMENT_3D('',#106049,#82265,#82266) ;
#69960=AXIS2_PLACEMENT_3D('',#106050,#82267,#82268) ;
#69961=AXIS2_PLACEMENT_3D('',#106051,#82269,#82270) ;
#69962=AXIS2_PLACEMENT_3D('',#106052,#82271,#82272) ;
#69963=AXIS2_PLACEMENT_3D('',#106053,#82273,#82274) ;
#69964=AXIS2_PLACEMENT_3D('',#106054,#82275,#82276) ;
#69965=AXIS2_PLACEMENT_3D('',#106055,#82277,#82278) ;
#69966=AXIS2_PLACEMENT_3D('',#106056,#82279,#82280) ;
#69967=AXIS2_PLACEMENT_3D('',#106057,#82281,#82282) ;
#69968=AXIS2_PLACEMENT_3D('',#106058,#82283,#82284) ;
#69969=AXIS2_PLACEMENT_3D('',#106059,#82285,#82286) ;
#69970=AXIS2_PLACEMENT_3D('',#106060,#82287,#82288) ;
#69971=AXIS2_PLACEMENT_3D('',#106061,#82289,#82290) ;
#69972=AXIS2_PLACEMENT_3D('',#106062,#82291,#82292) ;
#69973=AXIS2_PLACEMENT_3D('',#106063,#82293,#82294) ;
#69974=AXIS2_PLACEMENT_3D('',#106064,#82295,#82296) ;
#69975=AXIS2_PLACEMENT_3D('',#106065,#82297,#82298) ;
#69976=AXIS2_PLACEMENT_3D('',#106066,#82299,#82300) ;
#69977=AXIS2_PLACEMENT_3D('',#106067,#82301,#82302) ;
#69978=AXIS2_PLACEMENT_3D('',#106068,#82303,#82304) ;
#69979=AXIS2_PLACEMENT_3D('',#106069,#82305,#82306) ;
#69980=AXIS2_PLACEMENT_3D('',#106070,#82307,#82308) ;
#69981=AXIS2_PLACEMENT_3D('',#106071,#82309,#82310) ;
#69982=AXIS2_PLACEMENT_3D('',#106072,#82311,#82312) ;
#69983=AXIS2_PLACEMENT_3D('',#106073,#82313,#82314) ;
#69984=AXIS2_PLACEMENT_3D('',#106074,#82315,#82316) ;
#69985=AXIS2_PLACEMENT_3D('',#106075,#82317,#82318) ;
#69986=AXIS2_PLACEMENT_3D('',#106076,#82319,#82320) ;
#69987=AXIS2_PLACEMENT_3D('',#106077,#82321,#82322) ;
#69988=AXIS2_PLACEMENT_3D('',#106078,#82323,#82324) ;
#69989=AXIS2_PLACEMENT_3D('',#106079,#82325,#82326) ;
#69990=AXIS2_PLACEMENT_3D('',#106092,#82327,#82328) ;
#69991=AXIS2_PLACEMENT_3D('',#106093,#82329,#82330) ;
#69992=AXIS2_PLACEMENT_3D('',#106094,#82331,#82332) ;
#69993=AXIS2_PLACEMENT_3D('',#106095,#82333,#82334) ;
#69994=AXIS2_PLACEMENT_3D('',#106150,#82335,#82336) ;
#69995=AXIS2_PLACEMENT_3D('',#106151,#82337,#82338) ;
#69996=AXIS2_PLACEMENT_3D('',#106152,#82339,#82340) ;
#69997=AXIS2_PLACEMENT_3D('',#106207,#82341,#82342) ;
#69998=AXIS2_PLACEMENT_3D('',#106208,#82343,#82344) ;
#69999=AXIS2_PLACEMENT_3D('',#106234,#82345,#82346) ;
#70000=AXIS2_PLACEMENT_3D('',#106236,#82347,#82348) ;
#70001=AXIS2_PLACEMENT_3D('',#106238,#82349,#82350) ;
#70002=AXIS2_PLACEMENT_3D('',#106277,#82351,#82352) ;
#70003=AXIS2_PLACEMENT_3D('',#106279,#82353,#82354) ;
#70004=AXIS2_PLACEMENT_3D('',#106281,#82355,#82356) ;
#70005=AXIS2_PLACEMENT_3D('',#106282,#82357,#82358) ;
#70006=AXIS2_PLACEMENT_3D('',#106283,#82359,#82360) ;
#70007=AXIS2_PLACEMENT_3D('',#106285,#82361,#82362) ;
#70008=AXIS2_PLACEMENT_3D('',#106287,#82363,#82364) ;
#70009=AXIS2_PLACEMENT_3D('',#106288,#82365,#82366) ;
#70010=AXIS2_PLACEMENT_3D('',#106289,#82367,#82368) ;
#70011=AXIS2_PLACEMENT_3D('',#106291,#82369,#82370) ;
#70012=AXIS2_PLACEMENT_3D('',#106293,#82371,#82372) ;
#70013=AXIS2_PLACEMENT_3D('',#106294,#82373,#82374) ;
#70014=AXIS2_PLACEMENT_3D('',#106295,#82375,#82376) ;
#70015=AXIS2_PLACEMENT_3D('',#106298,#82377,#82378) ;
#70016=AXIS2_PLACEMENT_3D('',#106302,#82380,#82381) ;
#70017=AXIS2_PLACEMENT_3D('',#106304,#82382,#82383) ;
#70018=AXIS2_PLACEMENT_3D('',#106306,#82385,#82386) ;
#70019=AXIS2_PLACEMENT_3D('',#106309,#82387,#82388) ;
#70020=AXIS2_PLACEMENT_3D('',#106313,#82390,#82391) ;
#70021=AXIS2_PLACEMENT_3D('',#106315,#82393,#82394) ;
#70022=AXIS2_PLACEMENT_3D('',#106318,#82395,#82396) ;
#70023=AXIS2_PLACEMENT_3D('',#106320,#82397,#82398) ;
#70024=AXIS2_PLACEMENT_3D('',#106322,#82399,#82400) ;
#70025=AXIS2_PLACEMENT_3D('',#106323,#82401,#82402) ;
#70026=AXIS2_PLACEMENT_3D('',#106324,#82403,#82404) ;
#70027=AXIS2_PLACEMENT_3D('',#106326,#82406,#82407) ;
#70028=AXIS2_PLACEMENT_3D('',#106329,#82409,#82410) ;
#70029=AXIS2_PLACEMENT_3D('',#106338,#82411,#82412) ;
#70030=AXIS2_PLACEMENT_3D('',#106346,#82413,#82414) ;
#70031=AXIS2_PLACEMENT_3D('',#106348,#82416,#82417) ;
#70032=AXIS2_PLACEMENT_3D('',#106364,#82421,#82422) ;
#70033=AXIS2_PLACEMENT_3D('',#106366,#82424,#82425) ;
#70034=AXIS2_PLACEMENT_3D('',#106415,#82430,#82431) ;
#70035=AXIS2_PLACEMENT_3D('',#106424,#82436,#82437) ;
#70036=AXIS2_PLACEMENT_3D('',#106454,#82442,#82443) ;
#70037=AXIS2_PLACEMENT_3D('',#106463,#82448,#82449) ;
#70038=AXIS2_PLACEMENT_3D('',#106472,#82454,#82455) ;
#70039=AXIS2_PLACEMENT_3D('',#106483,#82460,#82461) ;
#70040=AXIS2_PLACEMENT_3D('',#106485,#82463,#82464) ;
#70041=AXIS2_PLACEMENT_3D('',#106489,#82466,#82467) ;
#70042=AXIS2_PLACEMENT_3D('',#106490,#82468,#82469) ;
#70043=AXIS2_PLACEMENT_3D('',#106491,#82470,#82471) ;
#70044=AXIS2_PLACEMENT_3D('',#106493,#82472,#82473) ;
#70045=AXIS2_PLACEMENT_3D('',#106497,#82475,#82476) ;
#70046=AXIS2_PLACEMENT_3D('',#106501,#82478,#82479) ;
#70047=AXIS2_PLACEMENT_3D('',#106505,#82481,#82482) ;
#70048=AXIS2_PLACEMENT_3D('',#106509,#82484,#82485) ;
#70049=AXIS2_PLACEMENT_3D('',#106513,#82487,#82488) ;
#70050=AXIS2_PLACEMENT_3D('',#106516,#82490,#82491) ;
#70051=AXIS2_PLACEMENT_3D('',#106518,#82492,#82493) ;
#70052=AXIS2_PLACEMENT_3D('',#106521,#82495,#82496) ;
#70053=AXIS2_PLACEMENT_3D('',#106523,#82497,#82498) ;
#70054=AXIS2_PLACEMENT_3D('',#106529,#82501,#82502) ;
#70055=AXIS2_PLACEMENT_3D('',#106533,#82504,#82505) ;
#70056=AXIS2_PLACEMENT_3D('',#106536,#82507,#82508) ;
#70057=AXIS2_PLACEMENT_3D('',#106537,#82509,#82510) ;
#70058=AXIS2_PLACEMENT_3D('',#106542,#82512,#82513) ;
#70059=AXIS2_PLACEMENT_3D('',#106546,#82515,#82516) ;
#70060=AXIS2_PLACEMENT_3D('',#106550,#82518,#82519) ;
#70061=AXIS2_PLACEMENT_3D('',#106554,#82521,#82522) ;
#70062=AXIS2_PLACEMENT_3D('',#106559,#82525,#82526) ;
#70063=AXIS2_PLACEMENT_3D('',#106561,#82527,#82528) ;
#70064=AXIS2_PLACEMENT_3D('',#106564,#82530,#82531) ;
#70065=AXIS2_PLACEMENT_3D('',#106566,#82532,#82533) ;
#70066=AXIS2_PLACEMENT_3D('',#106570,#82535,#82536) ;
#70067=AXIS2_PLACEMENT_3D('',#106574,#82538,#82539) ;
#70068=AXIS2_PLACEMENT_3D('',#106578,#82541,#82542) ;
#70069=AXIS2_PLACEMENT_3D('',#106582,#82544,#82545) ;
#70070=AXIS2_PLACEMENT_3D('',#106586,#82547,#82548) ;
#70071=AXIS2_PLACEMENT_3D('',#106590,#82550,#82551) ;
#70072=AXIS2_PLACEMENT_3D('',#106594,#82553,#82554) ;
#70073=AXIS2_PLACEMENT_3D('',#106597,#82556,#82557) ;
#70074=AXIS2_PLACEMENT_3D('',#106598,#82558,#82559) ;
#70075=AXIS2_PLACEMENT_3D('',#106601,#82562,#82563) ;
#70076=AXIS2_PLACEMENT_3D('',#106604,#82566,#82567) ;
#70077=AXIS2_PLACEMENT_3D('',#106693,#82572,#82573) ;
#70078=AXIS2_PLACEMENT_3D('',#106704,#82574,#82575) ;
#70079=AXIS2_PLACEMENT_3D('',#106709,#82579,#82580) ;
#70080=AXIS2_PLACEMENT_3D('',#106715,#82584,#82585) ;
#70081=AXIS2_PLACEMENT_3D('',#106735,#82589,#82590) ;
#70082=AXIS2_PLACEMENT_3D('',#106834,#82596,#82597) ;
#70083=AXIS2_PLACEMENT_3D('',#106838,#82599,#82600) ;
#70084=AXIS2_PLACEMENT_3D('',#106842,#82603,#82604) ;
#70085=AXIS2_PLACEMENT_3D('',#106845,#82605,#82606) ;
#70086=AXIS2_PLACEMENT_3D('',#106850,#82609,#82610) ;
#70087=AXIS2_PLACEMENT_3D('',#106852,#82611,#82612) ;
#70088=AXIS2_PLACEMENT_3D('',#106854,#82613,#82614) ;
#70089=AXIS2_PLACEMENT_3D('',#106862,#82618,#82619) ;
#70090=AXIS2_PLACEMENT_3D('',#106864,#82620,#82621) ;
#70091=AXIS2_PLACEMENT_3D('',#106866,#82622,#82623) ;
#70092=AXIS2_PLACEMENT_3D('',#106871,#82626,#82627) ;
#70093=AXIS2_PLACEMENT_3D('',#106873,#82628,#82629) ;
#70094=AXIS2_PLACEMENT_3D('',#106875,#82630,#82631) ;
#70095=AXIS2_PLACEMENT_3D('',#106879,#82633,#82634) ;
#70096=AXIS2_PLACEMENT_3D('',#106883,#82636,#82637) ;
#70097=AXIS2_PLACEMENT_3D('',#106884,#82638,#82639) ;
#70098=AXIS2_PLACEMENT_3D('',#106885,#82640,#82641) ;
#70099=AXIS2_PLACEMENT_3D('',#106888,#82642,#82643) ;
#70100=AXIS2_PLACEMENT_3D('',#106898,#82649,#82650) ;
#70101=AXIS2_PLACEMENT_3D('',#106900,#82652,#82653) ;
#70102=AXIS2_PLACEMENT_3D('',#106903,#82654,#82655) ;
#70103=AXIS2_PLACEMENT_3D('',#106909,#82659,#82660) ;
#70104=AXIS2_PLACEMENT_3D('',#106911,#82662,#82663) ;
#70105=AXIS2_PLACEMENT_3D('',#106917,#82666,#82667) ;
#70106=AXIS2_PLACEMENT_3D('',#106918,#82668,#82669) ;
#70107=AXIS2_PLACEMENT_3D('',#106921,#82670,#82671) ;
#70108=AXIS2_PLACEMENT_3D('',#106925,#82674,#82675) ;
#70109=AXIS2_PLACEMENT_3D('',#106942,#82684,#82685) ;
#70110=AXIS2_PLACEMENT_3D('',#106951,#82690,#82691) ;
#70111=AXIS2_PLACEMENT_3D('',#106960,#82696,#82697) ;
#70112=AXIS2_PLACEMENT_3D('',#106969,#82702,#82703) ;
#70113=AXIS2_PLACEMENT_3D('',#106996,#82708,#82709) ;
#70114=AXIS2_PLACEMENT_3D('',#107013,#82718,#82719) ;
#70115=AXIS2_PLACEMENT_3D('',#107018,#82721,#82722) ;
#70116=AXIS2_PLACEMENT_3D('',#107022,#82724,#82725) ;
#70117=AXIS2_PLACEMENT_3D('',#107026,#82727,#82728) ;
#70118=AXIS2_PLACEMENT_3D('',#107029,#82730,#82731) ;
#70119=AXIS2_PLACEMENT_3D('',#107030,#82732,#82733) ;
#70120=AXIS2_PLACEMENT_3D('',#107033,#82734,#82735) ;
#70121=AXIS2_PLACEMENT_3D('',#107038,#82738,#82739) ;
#70122=AXIS2_PLACEMENT_3D('',#107041,#82741,#82742) ;
#70123=AXIS2_PLACEMENT_3D('',#107042,#82743,#82744) ;
#70124=AXIS2_PLACEMENT_3D('',#107048,#82748,#82749) ;
#70125=AXIS2_PLACEMENT_3D('',#107054,#82753,#82754) ;
#70126=AXIS2_PLACEMENT_3D('',#107057,#82755,#82756) ;
#70127=AXIS2_PLACEMENT_3D('',#107061,#82758,#82759) ;
#70128=AXIS2_PLACEMENT_3D('',#107063,#82761,#82762) ;
#70129=AXIS2_PLACEMENT_3D('',#107066,#82763,#82764) ;
#70130=AXIS2_PLACEMENT_3D('',#107070,#82766,#82767) ;
#70131=AXIS2_PLACEMENT_3D('',#107072,#82769,#82770) ;
#70132=AXIS2_PLACEMENT_3D('',#107078,#82774,#82775) ;
#70133=AXIS2_PLACEMENT_3D('',#107084,#82779,#82780) ;
#70134=AXIS2_PLACEMENT_3D('',#107087,#82781,#82782) ;
#70135=AXIS2_PLACEMENT_3D('',#107092,#82785,#82786) ;
#70136=AXIS2_PLACEMENT_3D('',#107094,#82787,#82788) ;
#70137=AXIS2_PLACEMENT_3D('',#107096,#82790,#82791) ;
#70138=AXIS2_PLACEMENT_3D('',#107099,#82792,#82793) ;
#70139=AXIS2_PLACEMENT_3D('',#107104,#82797,#82798) ;
#70140=AXIS2_PLACEMENT_3D('',#107110,#82802,#82803) ;
#70141=AXIS2_PLACEMENT_3D('',#107113,#82804,#82805) ;
#70142=AXIS2_PLACEMENT_3D('',#107117,#82807,#82808) ;
#70143=AXIS2_PLACEMENT_3D('',#107119,#82810,#82811) ;
#70144=AXIS2_PLACEMENT_3D('',#107128,#82816,#82817) ;
#70145=AXIS2_PLACEMENT_3D('',#107131,#82818,#82819) ;
#70146=AXIS2_PLACEMENT_3D('',#107135,#82821,#82822) ;
#70147=AXIS2_PLACEMENT_3D('',#107137,#82824,#82825) ;
#70148=AXIS2_PLACEMENT_3D('',#107143,#82829,#82830) ;
#70149=AXIS2_PLACEMENT_3D('',#107152,#82835,#82836) ;
#70150=AXIS2_PLACEMENT_3D('',#107159,#82840,#82841) ;
#70151=AXIS2_PLACEMENT_3D('',#107160,#82842,#82843) ;
#70152=AXIS2_PLACEMENT_3D('',#107169,#82848,#82849) ;
#70153=AXIS2_PLACEMENT_3D('',#107172,#82850,#82851) ;
#70154=AXIS2_PLACEMENT_3D('',#107177,#82854,#82855) ;
#70155=AXIS2_PLACEMENT_3D('',#107181,#82857,#82858) ;
#70156=AXIS2_PLACEMENT_3D('',#107183,#82860,#82861) ;
#70157=AXIS2_PLACEMENT_3D('',#107191,#82866,#82867) ;
#70158=AXIS2_PLACEMENT_3D('',#107200,#82872,#82873) ;
#70159=AXIS2_PLACEMENT_3D('',#107209,#82878,#82879) ;
#70160=AXIS2_PLACEMENT_3D('',#107218,#82884,#82885) ;
#70161=AXIS2_PLACEMENT_3D('',#107224,#82889,#82890) ;
#70162=AXIS2_PLACEMENT_3D('',#107230,#82894,#82895) ;
#70163=AXIS2_PLACEMENT_3D('',#107236,#82899,#82900) ;
#70164=AXIS2_PLACEMENT_3D('',#107242,#82904,#82905) ;
#70165=AXIS2_PLACEMENT_3D('',#107251,#82909,#82910) ;
#70166=AXIS2_PLACEMENT_3D('',#107254,#82912,#82913) ;
#70167=AXIS2_PLACEMENT_3D('',#107255,#82914,#82915) ;
#70168=AXIS2_PLACEMENT_3D('',#107264,#82919,#82920) ;
#70169=AXIS2_PLACEMENT_3D('',#107267,#82922,#82923) ;
#70170=AXIS2_PLACEMENT_3D('',#107268,#82924,#82925) ;
#70171=AXIS2_PLACEMENT_3D('',#107272,#82927,#82928) ;
#70172=AXIS2_PLACEMENT_3D('',#107273,#82929,#82930) ;
#70173=AXIS2_PLACEMENT_3D('',#107274,#82931,#82932) ;
#70174=AXIS2_PLACEMENT_3D('',#107280,#82936,#82937) ;
#70175=AXIS2_PLACEMENT_3D('',#107289,#82942,#82943) ;
#70176=AXIS2_PLACEMENT_3D('',#107298,#82948,#82949) ;
#70177=AXIS2_PLACEMENT_3D('',#107307,#82954,#82955) ;
#70178=AXIS2_PLACEMENT_3D('',#107316,#82960,#82961) ;
#70179=AXIS2_PLACEMENT_3D('',#107317,#82962,#82963) ;
#70180=AXIS2_PLACEMENT_3D('',#107318,#82964,#82965) ;
#70181=AXIS2_PLACEMENT_3D('',#107319,#82966,#82967) ;
#70182=AXIS2_PLACEMENT_3D('',#107328,#82972,#82973) ;
#70183=AXIS2_PLACEMENT_3D('',#107337,#82978,#82979) ;
#70184=AXIS2_PLACEMENT_3D('',#107346,#82984,#82985) ;
#70185=AXIS2_PLACEMENT_3D('',#107355,#82990,#82991) ;
#70186=AXIS2_PLACEMENT_3D('',#107359,#82993,#82994) ;
#70187=AXIS2_PLACEMENT_3D('',#107361,#82996,#82997) ;
#70188=AXIS2_PLACEMENT_3D('',#107364,#82998,#82999) ;
#70189=AXIS2_PLACEMENT_3D('',#107365,#83000,#83001) ;
#70190=AXIS2_PLACEMENT_3D('',#107366,#83002,#83003) ;
#70191=AXIS2_PLACEMENT_3D('',#107367,#83004,#83005) ;
#70192=AXIS2_PLACEMENT_3D('',#107371,#83007,#83008) ;
#70193=AXIS2_PLACEMENT_3D('',#107373,#83010,#83011) ;
#70194=AXIS2_PLACEMENT_3D('',#107374,#83012,#83013) ;
#70195=AXIS2_PLACEMENT_3D('',#107375,#83014,#83015) ;
#70196=AXIS2_PLACEMENT_3D('',#107376,#83016,#83017) ;
#70197=AXIS2_PLACEMENT_3D('',#107377,#83018,#83019) ;
#70198=AXIS2_PLACEMENT_3D('',#107378,#83020,#83021) ;
#70199=AXIS2_PLACEMENT_3D('',#107379,#83022,#83023) ;
#70200=AXIS2_PLACEMENT_3D('',#107380,#83024,#83025) ;
#70201=AXIS2_PLACEMENT_3D('',#107381,#83026,#83027) ;
#70202=AXIS2_PLACEMENT_3D('',#107382,#83028,#83029) ;
#70203=AXIS2_PLACEMENT_3D('',#107383,#83030,#83031) ;
#70204=AXIS2_PLACEMENT_3D('',#107384,#83032,#83033) ;
#70205=AXIS2_PLACEMENT_3D('',#107385,#83034,#83035) ;
#70206=AXIS2_PLACEMENT_3D('',#107386,#83036,#83037) ;
#70207=AXIS2_PLACEMENT_3D('',#107387,#83038,#83039) ;
#70208=AXIS2_PLACEMENT_3D('',#107388,#83040,#83041) ;
#70209=AXIS2_PLACEMENT_3D('',#107389,#83042,#83043) ;
#70210=AXIS2_PLACEMENT_3D('',#107390,#83044,#83045) ;
#70211=AXIS2_PLACEMENT_3D('',#107391,#83046,#83047) ;
#70212=AXIS2_PLACEMENT_3D('',#107392,#83048,#83049) ;
#70213=AXIS2_PLACEMENT_3D('',#107393,#83050,#83051) ;
#70214=AXIS2_PLACEMENT_3D('',#107394,#83052,#83053) ;
#70215=AXIS2_PLACEMENT_3D('',#107395,#83054,#83055) ;
#70216=AXIS2_PLACEMENT_3D('',#107396,#83056,#83057) ;
#70217=AXIS2_PLACEMENT_3D('',#107397,#83058,#83059) ;
#70218=AXIS2_PLACEMENT_3D('',#107398,#83060,#83061) ;
#70219=AXIS2_PLACEMENT_3D('',#107399,#83062,#83063) ;
#70220=AXIS2_PLACEMENT_3D('',#107400,#83064,#83065) ;
#70221=AXIS2_PLACEMENT_3D('',#107401,#83066,#83067) ;
#70222=AXIS2_PLACEMENT_3D('',#107402,#83068,#83069) ;
#70223=AXIS2_PLACEMENT_3D('',#107403,#83070,#83071) ;
#70224=AXIS2_PLACEMENT_3D('',#107404,#83072,#83073) ;
#70225=AXIS2_PLACEMENT_3D('',#107405,#83074,#83075) ;
#70226=AXIS2_PLACEMENT_3D('',#107406,#83076,#83077) ;
#70227=AXIS2_PLACEMENT_3D('',#107407,#83078,#83079) ;
#70228=AXIS2_PLACEMENT_3D('',#107408,#83080,#83081) ;
#70229=AXIS2_PLACEMENT_3D('',#107409,#83082,#83083) ;
#70230=AXIS2_PLACEMENT_3D('',#107410,#83084,#83085) ;
#70231=AXIS2_PLACEMENT_3D('',#107411,#83086,#83087) ;
#70232=AXIS2_PLACEMENT_3D('',#107412,#83088,#83089) ;
#70233=AXIS2_PLACEMENT_3D('',#107413,#83090,#83091) ;
#70234=AXIS2_PLACEMENT_3D('',#107414,#83092,#83093) ;
#70235=AXIS2_PLACEMENT_3D('',#107415,#83094,#83095) ;
#70236=AXIS2_PLACEMENT_3D('',#107416,#83096,#83097) ;
#70237=AXIS2_PLACEMENT_3D('',#107417,#83098,#83099) ;
#70238=AXIS2_PLACEMENT_3D('',#107418,#83100,#83101) ;
#70239=AXIS2_PLACEMENT_3D('',#107419,#83102,#83103) ;
#70240=AXIS2_PLACEMENT_3D('',#107420,#83104,#83105) ;
#70241=AXIS2_PLACEMENT_3D('',#107421,#83106,#83107) ;
#70242=AXIS2_PLACEMENT_3D('',#107422,#83108,#83109) ;
#70243=AXIS2_PLACEMENT_3D('',#107423,#83110,#83111) ;
#70244=AXIS2_PLACEMENT_3D('',#107424,#83112,#83113) ;
#70245=AXIS2_PLACEMENT_3D('',#107425,#83114,#83115) ;
#70246=AXIS2_PLACEMENT_3D('',#107426,#83116,#83117) ;
#70247=AXIS2_PLACEMENT_3D('',#107427,#83118,#83119) ;
#70248=AXIS2_PLACEMENT_3D('',#107428,#83120,#83121) ;
#70249=AXIS2_PLACEMENT_3D('',#107429,#83122,#83123) ;
#70250=AXIS2_PLACEMENT_3D('',#107430,#83124,#83125) ;
#70251=AXIS2_PLACEMENT_3D('',#107431,#83126,#83127) ;
#70252=AXIS2_PLACEMENT_3D('',#107432,#83128,#83129) ;
#70253=AXIS2_PLACEMENT_3D('',#107433,#83130,#83131) ;
#70254=AXIS2_PLACEMENT_3D('',#107434,#83132,#83133) ;
#70255=AXIS2_PLACEMENT_3D('',#107435,#83134,#83135) ;
#70256=AXIS2_PLACEMENT_3D('',#107436,#83136,#83137) ;
#70257=AXIS2_PLACEMENT_3D('',#107437,#83138,#83139) ;
#70258=AXIS2_PLACEMENT_3D('',#107438,#83140,#83141) ;
#70259=AXIS2_PLACEMENT_3D('',#107439,#83142,#83143) ;
#70260=AXIS2_PLACEMENT_3D('',#107440,#83144,#83145) ;
#70261=AXIS2_PLACEMENT_3D('',#107441,#83146,#83147) ;
#70262=AXIS2_PLACEMENT_3D('',#107442,#83148,#83149) ;
#70263=AXIS2_PLACEMENT_3D('',#107443,#83150,#83151) ;
#70264=AXIS2_PLACEMENT_3D('',#107444,#83152,#83153) ;
#70265=AXIS2_PLACEMENT_3D('',#107445,#83154,#83155) ;
#70266=AXIS2_PLACEMENT_3D('',#107446,#83156,#83157) ;
#70267=AXIS2_PLACEMENT_3D('',#107462,#83158,#83159) ;
#70268=AXIS2_PLACEMENT_3D('',#107463,#83160,#83161) ;
#70269=AXIS2_PLACEMENT_3D('',#107465,#83162,#83163) ;
#70270=AXIS2_PLACEMENT_3D('',#107480,#83164,#83165) ;
#70271=AXIS2_PLACEMENT_3D('',#107481,#83166,#83167) ;
#70272=AXIS2_PLACEMENT_3D('',#107482,#83168,#83169) ;
#70273=AXIS2_PLACEMENT_3D('',#107484,#83170,#83171) ;
#70274=AXIS2_PLACEMENT_3D('',#107514,#83172,#83173) ;
#70275=AXIS2_PLACEMENT_3D('',#107515,#83174,#83175) ;
#70276=AXIS2_PLACEMENT_3D('',#107531,#83176,#83177) ;
#70277=AXIS2_PLACEMENT_3D('',#107533,#83178,#83179) ;
#70278=AXIS2_PLACEMENT_3D('',#107548,#83180,#83181) ;
#70279=AXIS2_PLACEMENT_3D('',#107549,#83182,#83183) ;
#70280=AXIS2_PLACEMENT_3D('',#107550,#83184,#83185) ;
#70281=AXIS2_PLACEMENT_3D('',#107551,#83186,#83187) ;
#70282=AXIS2_PLACEMENT_3D('',#107554,#83189,#83190) ;
#70283=AXIS2_PLACEMENT_3D('',#107555,#83191,#83192) ;
#70284=AXIS2_PLACEMENT_3D('',#107557,#83193,#83194) ;
#70285=AXIS2_PLACEMENT_3D('',#107558,#83195,#83196) ;
#70286=AXIS2_PLACEMENT_3D('',#107559,#83197,#83198) ;
#70287=AXIS2_PLACEMENT_3D('',#107561,#83199,#83200) ;
#70288=AXIS2_PLACEMENT_3D('',#107576,#83201,#83202) ;
#70289=AXIS2_PLACEMENT_3D('',#107577,#83203,#83204) ;
#70290=AXIS2_PLACEMENT_3D('',#107593,#83205,#83206) ;
#70291=AXIS2_PLACEMENT_3D('',#107594,#83207,#83208) ;
#70292=AXIS2_PLACEMENT_3D('',#107595,#83209,#83210) ;
#70293=AXIS2_PLACEMENT_3D('',#107597,#83211,#83212) ;
#70294=AXIS2_PLACEMENT_3D('',#107599,#83214,#83215) ;
#70295=AXIS2_PLACEMENT_3D('',#107600,#83216,#83217) ;
#70296=AXIS2_PLACEMENT_3D('',#107601,#83218,#83219) ;
#70297=AXIS2_PLACEMENT_3D('',#107602,#83220,#83221) ;
#70298=AXIS2_PLACEMENT_3D('',#107603,#83222,#83223) ;
#70299=AXIS2_PLACEMENT_3D('',#107604,#83224,#83225) ;
#70300=AXIS2_PLACEMENT_3D('',#107607,#83227,#83228) ;
#70301=AXIS2_PLACEMENT_3D('',#107608,#83229,#83230) ;
#70302=AXIS2_PLACEMENT_3D('',#107609,#83231,#83232) ;
#70303=AXIS2_PLACEMENT_3D('',#107610,#83233,#83234) ;
#70304=AXIS2_PLACEMENT_3D('',#107612,#83235,#83236) ;
#70305=AXIS2_PLACEMENT_3D('',#107613,#83237,#83238) ;
#70306=AXIS2_PLACEMENT_3D('',#107614,#83239,#83240) ;
#70307=AXIS2_PLACEMENT_3D('',#107615,#83241,#83242) ;
#70308=AXIS2_PLACEMENT_3D('',#107616,#83243,#83244) ;
#70309=AXIS2_PLACEMENT_3D('',#107617,#83245,#83246) ;
#70310=AXIS2_PLACEMENT_3D('',#107618,#83247,#83248) ;
#70311=AXIS2_PLACEMENT_3D('',#107620,#83249,#83250) ;
#70312=AXIS2_PLACEMENT_3D('',#107621,#83251,#83252) ;
#70313=AXIS2_PLACEMENT_3D('',#107622,#83253,#83254) ;
#70314=AXIS2_PLACEMENT_3D('',#107623,#83255,#83256) ;
#70315=AXIS2_PLACEMENT_3D('',#107624,#83257,#83258) ;
#70316=AXIS2_PLACEMENT_3D('',#107626,#83259,#83260) ;
#70317=AXIS2_PLACEMENT_3D('',#107628,#83262,#83263) ;
#70318=AXIS2_PLACEMENT_3D('',#107629,#83264,#83265) ;
#70319=AXIS2_PLACEMENT_3D('',#107630,#83266,#83267) ;
#70320=AXIS2_PLACEMENT_3D('',#107631,#83268,#83269) ;
#70321=AXIS2_PLACEMENT_3D('',#107632,#83270,#83271) ;
#70322=AXIS2_PLACEMENT_3D('',#107634,#83273,#83274) ;
#70323=AXIS2_PLACEMENT_3D('',#107635,#83275,#83276) ;
#70324=AXIS2_PLACEMENT_3D('',#107636,#83277,#83278) ;
#70325=AXIS2_PLACEMENT_3D('',#107637,#83279,#83280) ;
#70326=AXIS2_PLACEMENT_3D('',#107639,#83281,#83282) ;
#70327=AXIS2_PLACEMENT_3D('',#107640,#83283,#83284) ;
#70328=AXIS2_PLACEMENT_3D('',#107641,#83285,#83286) ;
#70329=AXIS2_PLACEMENT_3D('',#107642,#83287,#83288) ;
#70330=AXIS2_PLACEMENT_3D('',#107643,#83289,#83290) ;
#70331=AXIS2_PLACEMENT_3D('',#107644,#83291,#83292) ;
#70332=AXIS2_PLACEMENT_3D('',#107645,#83293,#83294) ;
#70333=AXIS2_PLACEMENT_3D('',#107647,#83296,#83297) ;
#70334=AXIS2_PLACEMENT_3D('',#107648,#83298,#83299) ;
#70335=AXIS2_PLACEMENT_3D('',#107649,#83300,#83301) ;
#70336=AXIS2_PLACEMENT_3D('',#107650,#83302,#83303) ;
#70337=AXIS2_PLACEMENT_3D('',#107651,#83304,#83305) ;
#70338=AXIS2_PLACEMENT_3D('',#107652,#83306,#83307) ;
#70339=AXIS2_PLACEMENT_3D('',#107653,#83308,#83309) ;
#70340=AXIS2_PLACEMENT_3D('',#107654,#83310,#83311) ;
#70341=AXIS2_PLACEMENT_3D('',#107655,#83312,#83313) ;
#70342=AXIS2_PLACEMENT_3D('',#107656,#83314,#83315) ;
#70343=AXIS2_PLACEMENT_3D('',#107657,#83316,#83317) ;
#70344=AXIS2_PLACEMENT_3D('',#107658,#83318,#83319) ;
#70345=AXIS2_PLACEMENT_3D('',#107659,#83320,#83321) ;
#70346=AXIS2_PLACEMENT_3D('',#107660,#83322,#83323) ;
#70347=AXIS2_PLACEMENT_3D('',#107661,#83324,#83325) ;
#70348=AXIS2_PLACEMENT_3D('',#107662,#83326,#83327) ;
#70349=AXIS2_PLACEMENT_3D('',#107663,#83328,#83329) ;
#70350=AXIS2_PLACEMENT_3D('',#107664,#83330,#83331) ;
#70351=AXIS2_PLACEMENT_3D('',#107665,#83332,#83333) ;
#70352=AXIS2_PLACEMENT_3D('',#107666,#83334,#83335) ;
#70353=AXIS2_PLACEMENT_3D('',#107667,#83336,#83337) ;
#70354=AXIS2_PLACEMENT_3D('',#107668,#83338,#83339) ;
#70355=AXIS2_PLACEMENT_3D('',#107669,#83340,#83341) ;
#70356=AXIS2_PLACEMENT_3D('',#107670,#83342,#83343) ;
#70357=AXIS2_PLACEMENT_3D('',#107671,#83344,#83345) ;
#70358=AXIS2_PLACEMENT_3D('',#107672,#83346,#83347) ;
#70359=AXIS2_PLACEMENT_3D('',#107673,#83348,#83349) ;
#70360=AXIS2_PLACEMENT_3D('',#107674,#83350,#83351) ;
#70361=AXIS2_PLACEMENT_3D('',#107675,#83352,#83353) ;
#70362=AXIS2_PLACEMENT_3D('',#107676,#83354,#83355) ;
#70363=AXIS2_PLACEMENT_3D('',#107677,#83356,#83357) ;
#70364=AXIS2_PLACEMENT_3D('',#107678,#83358,#83359) ;
#70365=AXIS2_PLACEMENT_3D('',#107679,#83360,#83361) ;
#70366=AXIS2_PLACEMENT_3D('',#107680,#83362,#83363) ;
#70367=AXIS2_PLACEMENT_3D('',#107681,#83364,#83365) ;
#70368=AXIS2_PLACEMENT_3D('',#107682,#83366,#83367) ;
#70369=AXIS2_PLACEMENT_3D('',#107683,#83368,#83369) ;
#70370=AXIS2_PLACEMENT_3D('',#107684,#83370,#83371) ;
#70371=AXIS2_PLACEMENT_3D('',#107685,#83372,#83373) ;
#70372=AXIS2_PLACEMENT_3D('',#107686,#83374,#83375) ;
#70373=AXIS2_PLACEMENT_3D('',#107687,#83376,#83377) ;
#70374=AXIS2_PLACEMENT_3D('',#107688,#83378,#83379) ;
#70375=AXIS2_PLACEMENT_3D('',#107689,#83380,#83381) ;
#70376=AXIS2_PLACEMENT_3D('',#107690,#83382,#83383) ;
#70377=AXIS2_PLACEMENT_3D('',#107691,#83384,#83385) ;
#70378=AXIS2_PLACEMENT_3D('',#107692,#83386,#83387) ;
#70379=AXIS2_PLACEMENT_3D('',#107693,#83388,#83389) ;
#70380=AXIS2_PLACEMENT_3D('',#107694,#83390,#83391) ;
#70381=AXIS2_PLACEMENT_3D('',#107695,#83392,#83393) ;
#70382=AXIS2_PLACEMENT_3D('',#107696,#83394,#83395) ;
#70383=AXIS2_PLACEMENT_3D('',#107713,#83396,#83397) ;
#70384=AXIS2_PLACEMENT_3D('',#107714,#83398,#83399) ;
#70385=AXIS2_PLACEMENT_3D('',#107715,#83400,#83401) ;
#70386=AXIS2_PLACEMENT_3D('',#107716,#83402,#83403) ;
#70387=AXIS2_PLACEMENT_3D('',#107717,#83404,#83405) ;
#70388=AXIS2_PLACEMENT_3D('',#107718,#83406,#83407) ;
#70389=AXIS2_PLACEMENT_3D('',#107719,#83408,#83409) ;
#70390=AXIS2_PLACEMENT_3D('',#107720,#83410,#83411) ;
#70391=AXIS2_PLACEMENT_3D('',#107721,#83412,#83413) ;
#70392=AXIS2_PLACEMENT_3D('',#107722,#83414,#83415) ;
#70393=AXIS2_PLACEMENT_3D('',#107723,#83416,#83417) ;
#70394=AXIS2_PLACEMENT_3D('',#107742,#83418,#83419) ;
#70395=AXIS2_PLACEMENT_3D('',#107743,#83420,#83421) ;
#70396=AXIS2_PLACEMENT_3D('',#107745,#83422,#83423) ;
#70397=AXIS2_PLACEMENT_3D('',#107746,#83424,#83425) ;
#70398=AXIS2_PLACEMENT_3D('',#107747,#83426,#83427) ;
#70399=AXIS2_PLACEMENT_3D('',#107748,#83428,#83429) ;
#70400=AXIS2_PLACEMENT_3D('',#107749,#83430,#83431) ;
#70401=AXIS2_PLACEMENT_3D('',#107750,#83432,#83433) ;
#70402=AXIS2_PLACEMENT_3D('',#107751,#83434,#83435) ;
#70403=AXIS2_PLACEMENT_3D('',#107752,#83436,#83437) ;
#70404=AXIS2_PLACEMENT_3D('',#107753,#83438,#83439) ;
#70405=AXIS2_PLACEMENT_3D('',#107754,#83440,#83441) ;
#70406=AXIS2_PLACEMENT_3D('',#107755,#83442,#83443) ;
#70407=AXIS2_PLACEMENT_3D('',#107790,#83444,#83445) ;
#70408=AXIS2_PLACEMENT_3D('',#107791,#83446,#83447) ;
#70409=AXIS2_PLACEMENT_3D('',#107792,#83448,#83449) ;
#70410=AXIS2_PLACEMENT_3D('',#107793,#83450,#83451) ;
#70411=AXIS2_PLACEMENT_3D('',#107804,#83452,#83453) ;
#70412=AXIS2_PLACEMENT_3D('',#107805,#83454,#83455) ;
#70413=AXIS2_PLACEMENT_3D('',#107806,#83456,#83457) ;
#70414=AXIS2_PLACEMENT_3D('',#107807,#83458,#83459) ;
#70415=AXIS2_PLACEMENT_3D('',#107814,#83460,#83461) ;
#70416=AXIS2_PLACEMENT_3D('',#107815,#83462,#83463) ;
#70417=AXIS2_PLACEMENT_3D('',#107816,#83464,#83465) ;
#70418=AXIS2_PLACEMENT_3D('',#107817,#83466,#83467) ;
#70419=AXIS2_PLACEMENT_3D('',#107818,#83468,#83469) ;
#70420=AXIS2_PLACEMENT_3D('',#107829,#83470,#83471) ;
#70421=AXIS2_PLACEMENT_3D('',#107830,#83472,#83473) ;
#70422=AXIS2_PLACEMENT_3D('',#107831,#83474,#83475) ;
#70423=AXIS2_PLACEMENT_3D('',#107832,#83476,#83477) ;
#70424=AXIS2_PLACEMENT_3D('',#107833,#83478,#83479) ;
#70425=AXIS2_PLACEMENT_3D('',#107834,#83480,#83481) ;
#70426=AXIS2_PLACEMENT_3D('',#107835,#83482,#83483) ;
#70427=AXIS2_PLACEMENT_3D('',#107836,#83484,#83485) ;
#70428=AXIS2_PLACEMENT_3D('',#107837,#83486,#83487) ;
#70429=AXIS2_PLACEMENT_3D('',#107838,#83488,#83489) ;
#70430=AXIS2_PLACEMENT_3D('',#107839,#83490,#83491) ;
#70431=AXIS2_PLACEMENT_3D('',#107840,#83492,#83493) ;
#70432=AXIS2_PLACEMENT_3D('',#107841,#83494,#83495) ;
#70433=AXIS2_PLACEMENT_3D('',#107842,#83496,#83497) ;
#70434=AXIS2_PLACEMENT_3D('',#107843,#83498,#83499) ;
#70435=AXIS2_PLACEMENT_3D('',#107844,#83500,#83501) ;
#70436=AXIS2_PLACEMENT_3D('',#107845,#83502,#83503) ;
#70437=AXIS2_PLACEMENT_3D('',#107846,#83504,#83505) ;
#70438=AXIS2_PLACEMENT_3D('',#107847,#83506,#83507) ;
#70439=AXIS2_PLACEMENT_3D('',#107848,#83508,#83509) ;
#70440=AXIS2_PLACEMENT_3D('',#107849,#83510,#83511) ;
#70441=AXIS2_PLACEMENT_3D('',#107850,#83512,#83513) ;
#70442=AXIS2_PLACEMENT_3D('',#107851,#83514,#83515) ;
#70443=AXIS2_PLACEMENT_3D('',#107852,#83516,#83517) ;
#70444=AXIS2_PLACEMENT_3D('',#107853,#83518,#83519) ;
#70445=AXIS2_PLACEMENT_3D('',#107854,#83520,#83521) ;
#70446=AXIS2_PLACEMENT_3D('',#107855,#83522,#83523) ;
#70447=AXIS2_PLACEMENT_3D('',#107856,#83524,#83525) ;
#70448=AXIS2_PLACEMENT_3D('',#107857,#83526,#83527) ;
#70449=AXIS2_PLACEMENT_3D('',#107858,#83528,#83529) ;
#70450=AXIS2_PLACEMENT_3D('',#107859,#83530,#83531) ;
#70451=AXIS2_PLACEMENT_3D('',#107860,#83532,#83533) ;
#70452=AXIS2_PLACEMENT_3D('',#107861,#83534,#83535) ;
#70453=AXIS2_PLACEMENT_3D('',#107862,#83536,#83537) ;
#70454=AXIS2_PLACEMENT_3D('',#107869,#83538,#83539) ;
#70455=AXIS2_PLACEMENT_3D('',#107870,#83540,#83541) ;
#70456=AXIS2_PLACEMENT_3D('',#107871,#83542,#83543) ;
#70457=AXIS2_PLACEMENT_3D('',#107872,#83544,#83545) ;
#70458=AXIS2_PLACEMENT_3D('',#107873,#83546,#83547) ;
#70459=AXIS2_PLACEMENT_3D('',#107874,#83548,#83549) ;
#70460=AXIS2_PLACEMENT_3D('',#107875,#83550,#83551) ;
#70461=AXIS2_PLACEMENT_3D('',#107876,#83552,#83553) ;
#70462=AXIS2_PLACEMENT_3D('',#107877,#83554,#83555) ;
#70463=AXIS2_PLACEMENT_3D('',#107878,#83556,#83557) ;
#70464=AXIS2_PLACEMENT_3D('',#107879,#83558,#83559) ;
#70465=AXIS2_PLACEMENT_3D('',#107880,#83560,#83561) ;
#70466=AXIS2_PLACEMENT_3D('',#107881,#83562,#83563) ;
#70467=AXIS2_PLACEMENT_3D('',#107882,#83564,#83565) ;
#70468=AXIS2_PLACEMENT_3D('',#107883,#83566,#83567) ;
#70469=AXIS2_PLACEMENT_3D('',#107884,#83568,#83569) ;
#70470=AXIS2_PLACEMENT_3D('',#107885,#83570,#83571) ;
#70471=AXIS2_PLACEMENT_3D('',#107886,#83572,#83573) ;
#70472=AXIS2_PLACEMENT_3D('',#107887,#83574,#83575) ;
#70473=AXIS2_PLACEMENT_3D('',#107888,#83576,#83577) ;
#70474=AXIS2_PLACEMENT_3D('',#107889,#83578,#83579) ;
#70475=AXIS2_PLACEMENT_3D('',#107890,#83580,#83581) ;
#70476=AXIS2_PLACEMENT_3D('',#107891,#83582,#83583) ;
#70477=AXIS2_PLACEMENT_3D('',#107892,#83584,#83585) ;
#70478=AXIS2_PLACEMENT_3D('',#107893,#83586,#83587) ;
#70479=AXIS2_PLACEMENT_3D('',#107894,#83588,#83589) ;
#70480=AXIS2_PLACEMENT_3D('',#107895,#83590,#83591) ;
#70481=AXIS2_PLACEMENT_3D('',#107896,#83592,#83593) ;
#70482=AXIS2_PLACEMENT_3D('',#107897,#83594,#83595) ;
#70483=AXIS2_PLACEMENT_3D('',#107898,#83596,#83597) ;
#70484=AXIS2_PLACEMENT_3D('',#107899,#83598,#83599) ;
#70485=AXIS2_PLACEMENT_3D('',#107900,#83600,#83601) ;
#70486=AXIS2_PLACEMENT_3D('',#107901,#83602,#83603) ;
#70487=AXIS2_PLACEMENT_3D('',#107902,#83604,#83605) ;
#70488=AXIS2_PLACEMENT_3D('',#107903,#83606,#83607) ;
#70489=AXIS2_PLACEMENT_3D('',#107904,#83608,#83609) ;
#70490=AXIS2_PLACEMENT_3D('',#107905,#83610,#83611) ;
#70491=AXIS2_PLACEMENT_3D('',#107906,#83612,#83613) ;
#70492=AXIS2_PLACEMENT_3D('',#107907,#83614,#83615) ;
#70493=AXIS2_PLACEMENT_3D('',#107938,#83616,#83617) ;
#70494=AXIS2_PLACEMENT_3D('',#107939,#83618,#83619) ;
#70495=AXIS2_PLACEMENT_3D('',#107940,#83620,#83621) ;
#70496=AXIS2_PLACEMENT_3D('',#107941,#83622,#83623) ;
#70497=AXIS2_PLACEMENT_3D('',#107942,#83624,#83625) ;
#70498=AXIS2_PLACEMENT_3D('',#107943,#83626,#83627) ;
#70499=AXIS2_PLACEMENT_3D('',#107944,#83628,#83629) ;
#70500=AXIS2_PLACEMENT_3D('',#107945,#83630,#83631) ;
#70501=AXIS2_PLACEMENT_3D('',#107946,#83632,#83633) ;
#70502=AXIS2_PLACEMENT_3D('',#107947,#83634,#83635) ;
#70503=AXIS2_PLACEMENT_3D('',#107974,#83636,#83637) ;
#70504=AXIS2_PLACEMENT_3D('',#107975,#83638,#83639) ;
#70505=AXIS2_PLACEMENT_3D('',#107976,#83640,#83641) ;
#70506=AXIS2_PLACEMENT_3D('',#107977,#83642,#83643) ;
#70507=AXIS2_PLACEMENT_3D('',#107978,#83644,#83645) ;
#70508=AXIS2_PLACEMENT_3D('',#107979,#83646,#83647) ;
#70509=AXIS2_PLACEMENT_3D('',#107980,#83648,#83649) ;
#70510=AXIS2_PLACEMENT_3D('',#107981,#83650,#83651) ;
#70511=AXIS2_PLACEMENT_3D('',#107982,#83652,#83653) ;
#70512=AXIS2_PLACEMENT_3D('',#107983,#83654,#83655) ;
#70513=AXIS2_PLACEMENT_3D('',#107984,#83656,#83657) ;
#70514=AXIS2_PLACEMENT_3D('',#107985,#83658,#83659) ;
#70515=AXIS2_PLACEMENT_3D('',#107986,#83660,#83661) ;
#70516=AXIS2_PLACEMENT_3D('',#107987,#83662,#83663) ;
#70517=AXIS2_PLACEMENT_3D('',#107988,#83664,#83665) ;
#70518=AXIS2_PLACEMENT_3D('',#107989,#83666,#83667) ;
#70519=AXIS2_PLACEMENT_3D('',#107990,#83668,#83669) ;
#70520=AXIS2_PLACEMENT_3D('',#107991,#83670,#83671) ;
#70521=AXIS2_PLACEMENT_3D('',#107992,#83672,#83673) ;
#70522=AXIS2_PLACEMENT_3D('',#107993,#83674,#83675) ;
#70523=AXIS2_PLACEMENT_3D('',#107994,#83676,#83677) ;
#70524=AXIS2_PLACEMENT_3D('',#107995,#83678,#83679) ;
#70525=AXIS2_PLACEMENT_3D('',#107996,#83680,#83681) ;
#70526=AXIS2_PLACEMENT_3D('',#107997,#83682,#83683) ;
#70527=AXIS2_PLACEMENT_3D('',#107998,#83684,#83685) ;
#70528=AXIS2_PLACEMENT_3D('',#107999,#83686,#83687) ;
#70529=AXIS2_PLACEMENT_3D('',#108000,#83688,#83689) ;
#70530=AXIS2_PLACEMENT_3D('',#108001,#83690,#83691) ;
#70531=AXIS2_PLACEMENT_3D('',#108002,#83692,#83693) ;
#70532=AXIS2_PLACEMENT_3D('',#108027,#83694,#83695) ;
#70533=AXIS2_PLACEMENT_3D('',#108028,#83696,#83697) ;
#70534=AXIS2_PLACEMENT_3D('',#108029,#83698,#83699) ;
#70535=AXIS2_PLACEMENT_3D('',#108030,#83700,#83701) ;
#70536=AXIS2_PLACEMENT_3D('',#108031,#83702,#83703) ;
#70537=AXIS2_PLACEMENT_3D('',#108032,#83704,#83705) ;
#70538=AXIS2_PLACEMENT_3D('',#108033,#83706,#83707) ;
#70539=AXIS2_PLACEMENT_3D('',#108082,#83708,#83709) ;
#70540=AXIS2_PLACEMENT_3D('',#108083,#83710,#83711) ;
#70541=AXIS2_PLACEMENT_3D('',#108084,#83712,#83713) ;
#70542=AXIS2_PLACEMENT_3D('',#108085,#83714,#83715) ;
#70543=AXIS2_PLACEMENT_3D('',#108086,#83716,#83717) ;
#70544=AXIS2_PLACEMENT_3D('',#108087,#83718,#83719) ;
#70545=AXIS2_PLACEMENT_3D('',#108088,#83720,#83721) ;
#70546=AXIS2_PLACEMENT_3D('',#108150,#83722,#83723) ;
#70547=AXIS2_PLACEMENT_3D('',#108151,#83724,#83725) ;
#70548=AXIS2_PLACEMENT_3D('',#108152,#83726,#83727) ;
#70549=AXIS2_PLACEMENT_3D('',#108325,#83728,#83729) ;
#70550=AXIS2_PLACEMENT_3D('',#108326,#83730,#83731) ;
#70551=AXIS2_PLACEMENT_3D('',#108381,#83732,#83733) ;
#70552=AXIS2_PLACEMENT_3D('',#108428,#83734,#83735) ;
#70553=AXIS2_PLACEMENT_3D('',#108429,#83736,#83737) ;
#70554=AXIS2_PLACEMENT_3D('',#108430,#83738,#83739) ;
#70555=AXIS2_PLACEMENT_3D('',#108431,#83740,#83741) ;
#70556=AXIS2_PLACEMENT_3D('',#108432,#83742,#83743) ;
#70557=AXIS2_PLACEMENT_3D('',#108433,#83744,#83745) ;
#70558=AXIS2_PLACEMENT_3D('',#108538,#83746,#83747) ;
#70559=AXIS2_PLACEMENT_3D('',#108539,#83748,#83749) ;
#70560=AXIS2_PLACEMENT_3D('',#108540,#83750,#83751) ;
#70561=AXIS2_PLACEMENT_3D('',#108541,#83752,#83753) ;
#70562=AXIS2_PLACEMENT_3D('',#108554,#83754,#83755) ;
#70563=AXIS2_PLACEMENT_3D('',#108555,#83756,#83757) ;
#70564=AXIS2_PLACEMENT_3D('',#108556,#83758,#83759) ;
#70565=AXIS2_PLACEMENT_3D('',#108557,#83760,#83761) ;
#70566=AXIS2_PLACEMENT_3D('',#108558,#83762,#83763) ;
#70567=AXIS2_PLACEMENT_3D('',#108559,#83764,#83765) ;
#70568=AXIS2_PLACEMENT_3D('',#108560,#83766,#83767) ;
#70569=AXIS2_PLACEMENT_3D('',#108561,#83768,#83769) ;
#70570=AXIS2_PLACEMENT_3D('',#108562,#83770,#83771) ;
#70571=AXIS2_PLACEMENT_3D('',#108563,#83772,#83773) ;
#70572=AXIS2_PLACEMENT_3D('',#108564,#83774,#83775) ;
#70573=AXIS2_PLACEMENT_3D('',#108565,#83776,#83777) ;
#70574=AXIS2_PLACEMENT_3D('',#108566,#83778,#83779) ;
#70575=AXIS2_PLACEMENT_3D('',#108567,#83780,#83781) ;
#70576=AXIS2_PLACEMENT_3D('',#108568,#83782,#83783) ;
#70577=AXIS2_PLACEMENT_3D('',#108569,#83784,#83785) ;
#70578=AXIS2_PLACEMENT_3D('',#108570,#83786,#83787) ;
#70579=AXIS2_PLACEMENT_3D('',#108571,#83788,#83789) ;
#70580=AXIS2_PLACEMENT_3D('',#108572,#83790,#83791) ;
#70581=AXIS2_PLACEMENT_3D('',#108573,#83792,#83793) ;
#70582=AXIS2_PLACEMENT_3D('',#108574,#83794,#83795) ;
#70583=AXIS2_PLACEMENT_3D('',#108575,#83796,#83797) ;
#70584=AXIS2_PLACEMENT_3D('',#108576,#83798,#83799) ;
#70585=AXIS2_PLACEMENT_3D('',#108577,#83800,#83801) ;
#70586=AXIS2_PLACEMENT_3D('',#108578,#83802,#83803) ;
#70587=AXIS2_PLACEMENT_3D('',#108579,#83804,#83805) ;
#70588=AXIS2_PLACEMENT_3D('',#108580,#83806,#83807) ;
#70589=AXIS2_PLACEMENT_3D('',#108581,#83808,#83809) ;
#70590=AXIS2_PLACEMENT_3D('',#108582,#83810,#83811) ;
#70591=AXIS2_PLACEMENT_3D('',#108583,#83812,#83813) ;
#70592=AXIS2_PLACEMENT_3D('',#108584,#83814,#83815) ;
#70593=AXIS2_PLACEMENT_3D('',#108585,#83816,#83817) ;
#70594=AXIS2_PLACEMENT_3D('',#108586,#83818,#83819) ;
#70595=AXIS2_PLACEMENT_3D('',#108587,#83820,#83821) ;
#70596=AXIS2_PLACEMENT_3D('',#108588,#83822,#83823) ;
#70597=AXIS2_PLACEMENT_3D('',#108589,#83824,#83825) ;
#70598=AXIS2_PLACEMENT_3D('',#108590,#83826,#83827) ;
#70599=AXIS2_PLACEMENT_3D('',#108591,#83828,#83829) ;
#70600=AXIS2_PLACEMENT_3D('',#108604,#83830,#83831) ;
#70601=AXIS2_PLACEMENT_3D('',#108605,#83832,#83833) ;
#70602=AXIS2_PLACEMENT_3D('',#108606,#83834,#83835) ;
#70603=AXIS2_PLACEMENT_3D('',#108607,#83836,#83837) ;
#70604=AXIS2_PLACEMENT_3D('',#108662,#83838,#83839) ;
#70605=AXIS2_PLACEMENT_3D('',#108663,#83840,#83841) ;
#70606=AXIS2_PLACEMENT_3D('',#108664,#83842,#83843) ;
#70607=AXIS2_PLACEMENT_3D('',#108719,#83844,#83845) ;
#70608=AXIS2_PLACEMENT_3D('',#108720,#83846,#83847) ;
#70609=AXIS2_PLACEMENT_3D('',#108746,#83848,#83849) ;
#70610=AXIS2_PLACEMENT_3D('',#108748,#83850,#83851) ;
#70611=AXIS2_PLACEMENT_3D('',#108750,#83852,#83853) ;
#70612=AXIS2_PLACEMENT_3D('',#108789,#83854,#83855) ;
#70613=AXIS2_PLACEMENT_3D('',#108791,#83856,#83857) ;
#70614=AXIS2_PLACEMENT_3D('',#108793,#83858,#83859) ;
#70615=AXIS2_PLACEMENT_3D('',#108794,#83860,#83861) ;
#70616=AXIS2_PLACEMENT_3D('',#108795,#83862,#83863) ;
#70617=AXIS2_PLACEMENT_3D('',#108797,#83864,#83865) ;
#70618=AXIS2_PLACEMENT_3D('',#108799,#83866,#83867) ;
#70619=AXIS2_PLACEMENT_3D('',#108800,#83868,#83869) ;
#70620=AXIS2_PLACEMENT_3D('',#108801,#83870,#83871) ;
#70621=AXIS2_PLACEMENT_3D('',#108803,#83872,#83873) ;
#70622=AXIS2_PLACEMENT_3D('',#108805,#83874,#83875) ;
#70623=AXIS2_PLACEMENT_3D('',#108806,#83876,#83877) ;
#70624=AXIS2_PLACEMENT_3D('',#108807,#83878,#83879) ;
#70625=AXIS2_PLACEMENT_3D('',#108810,#83880,#83881) ;
#70626=AXIS2_PLACEMENT_3D('',#108814,#83883,#83884) ;
#70627=AXIS2_PLACEMENT_3D('',#108816,#83885,#83886) ;
#70628=AXIS2_PLACEMENT_3D('',#108818,#83888,#83889) ;
#70629=AXIS2_PLACEMENT_3D('',#108821,#83890,#83891) ;
#70630=AXIS2_PLACEMENT_3D('',#108825,#83893,#83894) ;
#70631=AXIS2_PLACEMENT_3D('',#108827,#83896,#83897) ;
#70632=AXIS2_PLACEMENT_3D('',#108830,#83898,#83899) ;
#70633=AXIS2_PLACEMENT_3D('',#108832,#83900,#83901) ;
#70634=AXIS2_PLACEMENT_3D('',#108834,#83902,#83903) ;
#70635=AXIS2_PLACEMENT_3D('',#108835,#83904,#83905) ;
#70636=AXIS2_PLACEMENT_3D('',#108836,#83906,#83907) ;
#70637=AXIS2_PLACEMENT_3D('',#108838,#83909,#83910) ;
#70638=AXIS2_PLACEMENT_3D('',#108841,#83912,#83913) ;
#70639=AXIS2_PLACEMENT_3D('',#108850,#83914,#83915) ;
#70640=AXIS2_PLACEMENT_3D('',#108858,#83916,#83917) ;
#70641=AXIS2_PLACEMENT_3D('',#108860,#83919,#83920) ;
#70642=AXIS2_PLACEMENT_3D('',#108876,#83924,#83925) ;
#70643=AXIS2_PLACEMENT_3D('',#108878,#83927,#83928) ;
#70644=AXIS2_PLACEMENT_3D('',#108927,#83933,#83934) ;
#70645=AXIS2_PLACEMENT_3D('',#108936,#83939,#83940) ;
#70646=AXIS2_PLACEMENT_3D('',#108966,#83945,#83946) ;
#70647=AXIS2_PLACEMENT_3D('',#108975,#83951,#83952) ;
#70648=AXIS2_PLACEMENT_3D('',#108984,#83957,#83958) ;
#70649=AXIS2_PLACEMENT_3D('',#108995,#83963,#83964) ;
#70650=AXIS2_PLACEMENT_3D('',#108997,#83966,#83967) ;
#70651=AXIS2_PLACEMENT_3D('',#109001,#83969,#83970) ;
#70652=AXIS2_PLACEMENT_3D('',#109002,#83971,#83972) ;
#70653=AXIS2_PLACEMENT_3D('',#109003,#83973,#83974) ;
#70654=AXIS2_PLACEMENT_3D('',#109005,#83975,#83976) ;
#70655=AXIS2_PLACEMENT_3D('',#109009,#83978,#83979) ;
#70656=AXIS2_PLACEMENT_3D('',#109013,#83981,#83982) ;
#70657=AXIS2_PLACEMENT_3D('',#109017,#83984,#83985) ;
#70658=AXIS2_PLACEMENT_3D('',#109021,#83987,#83988) ;
#70659=AXIS2_PLACEMENT_3D('',#109025,#83990,#83991) ;
#70660=AXIS2_PLACEMENT_3D('',#109028,#83993,#83994) ;
#70661=AXIS2_PLACEMENT_3D('',#109030,#83995,#83996) ;
#70662=AXIS2_PLACEMENT_3D('',#109033,#83998,#83999) ;
#70663=AXIS2_PLACEMENT_3D('',#109035,#84000,#84001) ;
#70664=AXIS2_PLACEMENT_3D('',#109041,#84004,#84005) ;
#70665=AXIS2_PLACEMENT_3D('',#109045,#84007,#84008) ;
#70666=AXIS2_PLACEMENT_3D('',#109048,#84010,#84011) ;
#70667=AXIS2_PLACEMENT_3D('',#109049,#84012,#84013) ;
#70668=AXIS2_PLACEMENT_3D('',#109054,#84015,#84016) ;
#70669=AXIS2_PLACEMENT_3D('',#109058,#84018,#84019) ;
#70670=AXIS2_PLACEMENT_3D('',#109062,#84021,#84022) ;
#70671=AXIS2_PLACEMENT_3D('',#109066,#84024,#84025) ;
#70672=AXIS2_PLACEMENT_3D('',#109071,#84028,#84029) ;
#70673=AXIS2_PLACEMENT_3D('',#109073,#84030,#84031) ;
#70674=AXIS2_PLACEMENT_3D('',#109076,#84033,#84034) ;
#70675=AXIS2_PLACEMENT_3D('',#109078,#84035,#84036) ;
#70676=AXIS2_PLACEMENT_3D('',#109082,#84038,#84039) ;
#70677=AXIS2_PLACEMENT_3D('',#109086,#84041,#84042) ;
#70678=AXIS2_PLACEMENT_3D('',#109090,#84044,#84045) ;
#70679=AXIS2_PLACEMENT_3D('',#109094,#84047,#84048) ;
#70680=AXIS2_PLACEMENT_3D('',#109098,#84050,#84051) ;
#70681=AXIS2_PLACEMENT_3D('',#109102,#84053,#84054) ;
#70682=AXIS2_PLACEMENT_3D('',#109106,#84056,#84057) ;
#70683=AXIS2_PLACEMENT_3D('',#109109,#84059,#84060) ;
#70684=AXIS2_PLACEMENT_3D('',#109110,#84061,#84062) ;
#70685=AXIS2_PLACEMENT_3D('',#109113,#84065,#84066) ;
#70686=AXIS2_PLACEMENT_3D('',#109116,#84069,#84070) ;
#70687=AXIS2_PLACEMENT_3D('',#109205,#84075,#84076) ;
#70688=AXIS2_PLACEMENT_3D('',#109216,#84077,#84078) ;
#70689=AXIS2_PLACEMENT_3D('',#109221,#84082,#84083) ;
#70690=AXIS2_PLACEMENT_3D('',#109227,#84087,#84088) ;
#70691=AXIS2_PLACEMENT_3D('',#109247,#84092,#84093) ;
#70692=AXIS2_PLACEMENT_3D('',#109346,#84099,#84100) ;
#70693=AXIS2_PLACEMENT_3D('',#109350,#84102,#84103) ;
#70694=AXIS2_PLACEMENT_3D('',#109354,#84106,#84107) ;
#70695=AXIS2_PLACEMENT_3D('',#109357,#84108,#84109) ;
#70696=AXIS2_PLACEMENT_3D('',#109362,#84112,#84113) ;
#70697=AXIS2_PLACEMENT_3D('',#109364,#84114,#84115) ;
#70698=AXIS2_PLACEMENT_3D('',#109366,#84116,#84117) ;
#70699=AXIS2_PLACEMENT_3D('',#109374,#84121,#84122) ;
#70700=AXIS2_PLACEMENT_3D('',#109376,#84123,#84124) ;
#70701=AXIS2_PLACEMENT_3D('',#109378,#84125,#84126) ;
#70702=AXIS2_PLACEMENT_3D('',#109383,#84129,#84130) ;
#70703=AXIS2_PLACEMENT_3D('',#109385,#84131,#84132) ;
#70704=AXIS2_PLACEMENT_3D('',#109387,#84133,#84134) ;
#70705=AXIS2_PLACEMENT_3D('',#109391,#84136,#84137) ;
#70706=AXIS2_PLACEMENT_3D('',#109395,#84139,#84140) ;
#70707=AXIS2_PLACEMENT_3D('',#109396,#84141,#84142) ;
#70708=AXIS2_PLACEMENT_3D('',#109397,#84143,#84144) ;
#70709=AXIS2_PLACEMENT_3D('',#109400,#84145,#84146) ;
#70710=AXIS2_PLACEMENT_3D('',#109410,#84152,#84153) ;
#70711=AXIS2_PLACEMENT_3D('',#109412,#84155,#84156) ;
#70712=AXIS2_PLACEMENT_3D('',#109415,#84157,#84158) ;
#70713=AXIS2_PLACEMENT_3D('',#109421,#84162,#84163) ;
#70714=AXIS2_PLACEMENT_3D('',#109423,#84165,#84166) ;
#70715=AXIS2_PLACEMENT_3D('',#109429,#84169,#84170) ;
#70716=AXIS2_PLACEMENT_3D('',#109430,#84171,#84172) ;
#70717=AXIS2_PLACEMENT_3D('',#109433,#84173,#84174) ;
#70718=AXIS2_PLACEMENT_3D('',#109437,#84177,#84178) ;
#70719=AXIS2_PLACEMENT_3D('',#109454,#84187,#84188) ;
#70720=AXIS2_PLACEMENT_3D('',#109463,#84193,#84194) ;
#70721=AXIS2_PLACEMENT_3D('',#109472,#84199,#84200) ;
#70722=AXIS2_PLACEMENT_3D('',#109481,#84205,#84206) ;
#70723=AXIS2_PLACEMENT_3D('',#109508,#84211,#84212) ;
#70724=AXIS2_PLACEMENT_3D('',#109525,#84221,#84222) ;
#70725=AXIS2_PLACEMENT_3D('',#109530,#84224,#84225) ;
#70726=AXIS2_PLACEMENT_3D('',#109534,#84227,#84228) ;
#70727=AXIS2_PLACEMENT_3D('',#109538,#84230,#84231) ;
#70728=AXIS2_PLACEMENT_3D('',#109541,#84233,#84234) ;
#70729=AXIS2_PLACEMENT_3D('',#109542,#84235,#84236) ;
#70730=AXIS2_PLACEMENT_3D('',#109545,#84237,#84238) ;
#70731=AXIS2_PLACEMENT_3D('',#109550,#84241,#84242) ;
#70732=AXIS2_PLACEMENT_3D('',#109553,#84244,#84245) ;
#70733=AXIS2_PLACEMENT_3D('',#109554,#84246,#84247) ;
#70734=AXIS2_PLACEMENT_3D('',#109560,#84251,#84252) ;
#70735=AXIS2_PLACEMENT_3D('',#109566,#84256,#84257) ;
#70736=AXIS2_PLACEMENT_3D('',#109569,#84258,#84259) ;
#70737=AXIS2_PLACEMENT_3D('',#109573,#84261,#84262) ;
#70738=AXIS2_PLACEMENT_3D('',#109575,#84264,#84265) ;
#70739=AXIS2_PLACEMENT_3D('',#109578,#84266,#84267) ;
#70740=AXIS2_PLACEMENT_3D('',#109582,#84269,#84270) ;
#70741=AXIS2_PLACEMENT_3D('',#109584,#84272,#84273) ;
#70742=AXIS2_PLACEMENT_3D('',#109590,#84277,#84278) ;
#70743=AXIS2_PLACEMENT_3D('',#109596,#84282,#84283) ;
#70744=AXIS2_PLACEMENT_3D('',#109599,#84284,#84285) ;
#70745=AXIS2_PLACEMENT_3D('',#109604,#84288,#84289) ;
#70746=AXIS2_PLACEMENT_3D('',#109606,#84290,#84291) ;
#70747=AXIS2_PLACEMENT_3D('',#109608,#84293,#84294) ;
#70748=AXIS2_PLACEMENT_3D('',#109611,#84295,#84296) ;
#70749=AXIS2_PLACEMENT_3D('',#109616,#84300,#84301) ;
#70750=AXIS2_PLACEMENT_3D('',#109622,#84305,#84306) ;
#70751=AXIS2_PLACEMENT_3D('',#109625,#84307,#84308) ;
#70752=AXIS2_PLACEMENT_3D('',#109629,#84310,#84311) ;
#70753=AXIS2_PLACEMENT_3D('',#109631,#84313,#84314) ;
#70754=AXIS2_PLACEMENT_3D('',#109640,#84319,#84320) ;
#70755=AXIS2_PLACEMENT_3D('',#109643,#84321,#84322) ;
#70756=AXIS2_PLACEMENT_3D('',#109647,#84324,#84325) ;
#70757=AXIS2_PLACEMENT_3D('',#109649,#84327,#84328) ;
#70758=AXIS2_PLACEMENT_3D('',#109655,#84332,#84333) ;
#70759=AXIS2_PLACEMENT_3D('',#109664,#84338,#84339) ;
#70760=AXIS2_PLACEMENT_3D('',#109671,#84343,#84344) ;
#70761=AXIS2_PLACEMENT_3D('',#109672,#84345,#84346) ;
#70762=AXIS2_PLACEMENT_3D('',#109681,#84351,#84352) ;
#70763=AXIS2_PLACEMENT_3D('',#109684,#84353,#84354) ;
#70764=AXIS2_PLACEMENT_3D('',#109689,#84357,#84358) ;
#70765=AXIS2_PLACEMENT_3D('',#109693,#84360,#84361) ;
#70766=AXIS2_PLACEMENT_3D('',#109695,#84363,#84364) ;
#70767=AXIS2_PLACEMENT_3D('',#109703,#84369,#84370) ;
#70768=AXIS2_PLACEMENT_3D('',#109712,#84375,#84376) ;
#70769=AXIS2_PLACEMENT_3D('',#109721,#84381,#84382) ;
#70770=AXIS2_PLACEMENT_3D('',#109730,#84387,#84388) ;
#70771=AXIS2_PLACEMENT_3D('',#109736,#84392,#84393) ;
#70772=AXIS2_PLACEMENT_3D('',#109742,#84397,#84398) ;
#70773=AXIS2_PLACEMENT_3D('',#109748,#84402,#84403) ;
#70774=AXIS2_PLACEMENT_3D('',#109754,#84407,#84408) ;
#70775=AXIS2_PLACEMENT_3D('',#109763,#84412,#84413) ;
#70776=AXIS2_PLACEMENT_3D('',#109766,#84415,#84416) ;
#70777=AXIS2_PLACEMENT_3D('',#109767,#84417,#84418) ;
#70778=AXIS2_PLACEMENT_3D('',#109776,#84422,#84423) ;
#70779=AXIS2_PLACEMENT_3D('',#109779,#84425,#84426) ;
#70780=AXIS2_PLACEMENT_3D('',#109780,#84427,#84428) ;
#70781=AXIS2_PLACEMENT_3D('',#109784,#84430,#84431) ;
#70782=AXIS2_PLACEMENT_3D('',#109785,#84432,#84433) ;
#70783=AXIS2_PLACEMENT_3D('',#109786,#84434,#84435) ;
#70784=AXIS2_PLACEMENT_3D('',#109792,#84439,#84440) ;
#70785=AXIS2_PLACEMENT_3D('',#109801,#84445,#84446) ;
#70786=AXIS2_PLACEMENT_3D('',#109810,#84451,#84452) ;
#70787=AXIS2_PLACEMENT_3D('',#109819,#84457,#84458) ;
#70788=AXIS2_PLACEMENT_3D('',#109828,#84463,#84464) ;
#70789=AXIS2_PLACEMENT_3D('',#109829,#84465,#84466) ;
#70790=AXIS2_PLACEMENT_3D('',#109830,#84467,#84468) ;
#70791=AXIS2_PLACEMENT_3D('',#109831,#84469,#84470) ;
#70792=AXIS2_PLACEMENT_3D('',#109840,#84475,#84476) ;
#70793=AXIS2_PLACEMENT_3D('',#109849,#84481,#84482) ;
#70794=AXIS2_PLACEMENT_3D('',#109858,#84487,#84488) ;
#70795=AXIS2_PLACEMENT_3D('',#109867,#84493,#84494) ;
#70796=AXIS2_PLACEMENT_3D('',#109871,#84496,#84497) ;
#70797=AXIS2_PLACEMENT_3D('',#109873,#84499,#84500) ;
#70798=AXIS2_PLACEMENT_3D('',#109876,#84501,#84502) ;
#70799=AXIS2_PLACEMENT_3D('',#109877,#84503,#84504) ;
#70800=AXIS2_PLACEMENT_3D('',#109878,#84505,#84506) ;
#70801=AXIS2_PLACEMENT_3D('',#109879,#84507,#84508) ;
#70802=AXIS2_PLACEMENT_3D('',#109883,#84510,#84511) ;
#70803=AXIS2_PLACEMENT_3D('',#109885,#84513,#84514) ;
#70804=AXIS2_PLACEMENT_3D('',#109886,#84515,#84516) ;
#70805=AXIS2_PLACEMENT_3D('',#109887,#84517,#84518) ;
#70806=AXIS2_PLACEMENT_3D('',#109888,#84519,#84520) ;
#70807=AXIS2_PLACEMENT_3D('',#109889,#84521,#84522) ;
#70808=AXIS2_PLACEMENT_3D('',#109890,#84523,#84524) ;
#70809=AXIS2_PLACEMENT_3D('',#109891,#84525,#84526) ;
#70810=AXIS2_PLACEMENT_3D('',#109892,#84527,#84528) ;
#70811=AXIS2_PLACEMENT_3D('',#109893,#84529,#84530) ;
#70812=AXIS2_PLACEMENT_3D('',#109894,#84531,#84532) ;
#70813=AXIS2_PLACEMENT_3D('',#109895,#84533,#84534) ;
#70814=AXIS2_PLACEMENT_3D('',#109896,#84535,#84536) ;
#70815=AXIS2_PLACEMENT_3D('',#109897,#84537,#84538) ;
#70816=AXIS2_PLACEMENT_3D('',#109898,#84539,#84540) ;
#70817=AXIS2_PLACEMENT_3D('',#109899,#84541,#84542) ;
#70818=AXIS2_PLACEMENT_3D('',#109900,#84543,#84544) ;
#70819=AXIS2_PLACEMENT_3D('',#109901,#84545,#84546) ;
#70820=AXIS2_PLACEMENT_3D('',#109902,#84547,#84548) ;
#70821=AXIS2_PLACEMENT_3D('',#109903,#84549,#84550) ;
#70822=AXIS2_PLACEMENT_3D('',#109904,#84551,#84552) ;
#70823=AXIS2_PLACEMENT_3D('',#109905,#84553,#84554) ;
#70824=AXIS2_PLACEMENT_3D('',#109906,#84555,#84556) ;
#70825=AXIS2_PLACEMENT_3D('',#109907,#84557,#84558) ;
#70826=AXIS2_PLACEMENT_3D('',#109908,#84559,#84560) ;
#70827=AXIS2_PLACEMENT_3D('',#109909,#84561,#84562) ;
#70828=AXIS2_PLACEMENT_3D('',#109910,#84563,#84564) ;
#70829=AXIS2_PLACEMENT_3D('',#109911,#84565,#84566) ;
#70830=AXIS2_PLACEMENT_3D('',#109912,#84567,#84568) ;
#70831=AXIS2_PLACEMENT_3D('',#109913,#84569,#84570) ;
#70832=AXIS2_PLACEMENT_3D('',#109914,#84571,#84572) ;
#70833=AXIS2_PLACEMENT_3D('',#109915,#84573,#84574) ;
#70834=AXIS2_PLACEMENT_3D('',#109916,#84575,#84576) ;
#70835=AXIS2_PLACEMENT_3D('',#109917,#84577,#84578) ;
#70836=AXIS2_PLACEMENT_3D('',#109918,#84579,#84580) ;
#70837=AXIS2_PLACEMENT_3D('',#109919,#84581,#84582) ;
#70838=AXIS2_PLACEMENT_3D('',#109920,#84583,#84584) ;
#70839=AXIS2_PLACEMENT_3D('',#109921,#84585,#84586) ;
#70840=AXIS2_PLACEMENT_3D('',#109922,#84587,#84588) ;
#70841=AXIS2_PLACEMENT_3D('',#109923,#84589,#84590) ;
#70842=AXIS2_PLACEMENT_3D('',#109924,#84591,#84592) ;
#70843=AXIS2_PLACEMENT_3D('',#109925,#84593,#84594) ;
#70844=AXIS2_PLACEMENT_3D('',#109926,#84595,#84596) ;
#70845=AXIS2_PLACEMENT_3D('',#109927,#84597,#84598) ;
#70846=AXIS2_PLACEMENT_3D('',#109928,#84599,#84600) ;
#70847=AXIS2_PLACEMENT_3D('',#109929,#84601,#84602) ;
#70848=AXIS2_PLACEMENT_3D('',#109930,#84603,#84604) ;
#70849=AXIS2_PLACEMENT_3D('',#109931,#84605,#84606) ;
#70850=AXIS2_PLACEMENT_3D('',#109932,#84607,#84608) ;
#70851=AXIS2_PLACEMENT_3D('',#109933,#84609,#84610) ;
#70852=AXIS2_PLACEMENT_3D('',#109934,#84611,#84612) ;
#70853=AXIS2_PLACEMENT_3D('',#109935,#84613,#84614) ;
#70854=AXIS2_PLACEMENT_3D('',#109936,#84615,#84616) ;
#70855=AXIS2_PLACEMENT_3D('',#109937,#84617,#84618) ;
#70856=AXIS2_PLACEMENT_3D('',#109938,#84619,#84620) ;
#70857=AXIS2_PLACEMENT_3D('',#109939,#84621,#84622) ;
#70858=AXIS2_PLACEMENT_3D('',#109940,#84623,#84624) ;
#70859=AXIS2_PLACEMENT_3D('',#109941,#84625,#84626) ;
#70860=AXIS2_PLACEMENT_3D('',#109942,#84627,#84628) ;
#70861=AXIS2_PLACEMENT_3D('',#109943,#84629,#84630) ;
#70862=AXIS2_PLACEMENT_3D('',#109944,#84631,#84632) ;
#70863=AXIS2_PLACEMENT_3D('',#109945,#84633,#84634) ;
#70864=AXIS2_PLACEMENT_3D('',#109946,#84635,#84636) ;
#70865=AXIS2_PLACEMENT_3D('',#109947,#84637,#84638) ;
#70866=AXIS2_PLACEMENT_3D('',#109948,#84639,#84640) ;
#70867=AXIS2_PLACEMENT_3D('',#109949,#84641,#84642) ;
#70868=AXIS2_PLACEMENT_3D('',#109950,#84643,#84644) ;
#70869=AXIS2_PLACEMENT_3D('',#109951,#84645,#84646) ;
#70870=AXIS2_PLACEMENT_3D('',#109952,#84647,#84648) ;
#70871=AXIS2_PLACEMENT_3D('',#109953,#84649,#84650) ;
#70872=AXIS2_PLACEMENT_3D('',#109954,#84651,#84652) ;
#70873=AXIS2_PLACEMENT_3D('',#109955,#84653,#84654) ;
#70874=AXIS2_PLACEMENT_3D('',#109956,#84655,#84656) ;
#70875=AXIS2_PLACEMENT_3D('',#109957,#84657,#84658) ;
#70876=AXIS2_PLACEMENT_3D('',#109958,#84659,#84660) ;
#70877=AXIS2_PLACEMENT_3D('',#109974,#84661,#84662) ;
#70878=AXIS2_PLACEMENT_3D('',#109975,#84663,#84664) ;
#70879=AXIS2_PLACEMENT_3D('',#109977,#84665,#84666) ;
#70880=AXIS2_PLACEMENT_3D('',#109992,#84667,#84668) ;
#70881=AXIS2_PLACEMENT_3D('',#109993,#84669,#84670) ;
#70882=AXIS2_PLACEMENT_3D('',#109994,#84671,#84672) ;
#70883=AXIS2_PLACEMENT_3D('',#109996,#84673,#84674) ;
#70884=AXIS2_PLACEMENT_3D('',#110026,#84675,#84676) ;
#70885=AXIS2_PLACEMENT_3D('',#110027,#84677,#84678) ;
#70886=AXIS2_PLACEMENT_3D('',#110043,#84679,#84680) ;
#70887=AXIS2_PLACEMENT_3D('',#110045,#84681,#84682) ;
#70888=AXIS2_PLACEMENT_3D('',#110060,#84683,#84684) ;
#70889=AXIS2_PLACEMENT_3D('',#110061,#84685,#84686) ;
#70890=AXIS2_PLACEMENT_3D('',#110062,#84687,#84688) ;
#70891=AXIS2_PLACEMENT_3D('',#110063,#84689,#84690) ;
#70892=AXIS2_PLACEMENT_3D('',#110066,#84692,#84693) ;
#70893=AXIS2_PLACEMENT_3D('',#110067,#84694,#84695) ;
#70894=AXIS2_PLACEMENT_3D('',#110069,#84696,#84697) ;
#70895=AXIS2_PLACEMENT_3D('',#110070,#84698,#84699) ;
#70896=AXIS2_PLACEMENT_3D('',#110071,#84700,#84701) ;
#70897=AXIS2_PLACEMENT_3D('',#110073,#84702,#84703) ;
#70898=AXIS2_PLACEMENT_3D('',#110088,#84704,#84705) ;
#70899=AXIS2_PLACEMENT_3D('',#110089,#84706,#84707) ;
#70900=AXIS2_PLACEMENT_3D('',#110105,#84708,#84709) ;
#70901=AXIS2_PLACEMENT_3D('',#110106,#84710,#84711) ;
#70902=AXIS2_PLACEMENT_3D('',#110107,#84712,#84713) ;
#70903=AXIS2_PLACEMENT_3D('',#110109,#84714,#84715) ;
#70904=AXIS2_PLACEMENT_3D('',#110111,#84717,#84718) ;
#70905=AXIS2_PLACEMENT_3D('',#110112,#84719,#84720) ;
#70906=AXIS2_PLACEMENT_3D('',#110113,#84721,#84722) ;
#70907=AXIS2_PLACEMENT_3D('',#110114,#84723,#84724) ;
#70908=AXIS2_PLACEMENT_3D('',#110115,#84725,#84726) ;
#70909=AXIS2_PLACEMENT_3D('',#110116,#84727,#84728) ;
#70910=AXIS2_PLACEMENT_3D('',#110119,#84730,#84731) ;
#70911=AXIS2_PLACEMENT_3D('',#110120,#84732,#84733) ;
#70912=AXIS2_PLACEMENT_3D('',#110121,#84734,#84735) ;
#70913=AXIS2_PLACEMENT_3D('',#110122,#84736,#84737) ;
#70914=AXIS2_PLACEMENT_3D('',#110124,#84738,#84739) ;
#70915=AXIS2_PLACEMENT_3D('',#110125,#84740,#84741) ;
#70916=AXIS2_PLACEMENT_3D('',#110126,#84742,#84743) ;
#70917=AXIS2_PLACEMENT_3D('',#110127,#84744,#84745) ;
#70918=AXIS2_PLACEMENT_3D('',#110128,#84746,#84747) ;
#70919=AXIS2_PLACEMENT_3D('',#110129,#84748,#84749) ;
#70920=AXIS2_PLACEMENT_3D('',#110130,#84750,#84751) ;
#70921=AXIS2_PLACEMENT_3D('',#110132,#84752,#84753) ;
#70922=AXIS2_PLACEMENT_3D('',#110133,#84754,#84755) ;
#70923=AXIS2_PLACEMENT_3D('',#110134,#84756,#84757) ;
#70924=AXIS2_PLACEMENT_3D('',#110135,#84758,#84759) ;
#70925=AXIS2_PLACEMENT_3D('',#110136,#84760,#84761) ;
#70926=AXIS2_PLACEMENT_3D('',#110138,#84762,#84763) ;
#70927=AXIS2_PLACEMENT_3D('',#110140,#84765,#84766) ;
#70928=AXIS2_PLACEMENT_3D('',#110141,#84767,#84768) ;
#70929=AXIS2_PLACEMENT_3D('',#110142,#84769,#84770) ;
#70930=AXIS2_PLACEMENT_3D('',#110143,#84771,#84772) ;
#70931=AXIS2_PLACEMENT_3D('',#110144,#84773,#84774) ;
#70932=AXIS2_PLACEMENT_3D('',#110146,#84776,#84777) ;
#70933=AXIS2_PLACEMENT_3D('',#110147,#84778,#84779) ;
#70934=AXIS2_PLACEMENT_3D('',#110148,#84780,#84781) ;
#70935=AXIS2_PLACEMENT_3D('',#110149,#84782,#84783) ;
#70936=AXIS2_PLACEMENT_3D('',#110151,#84784,#84785) ;
#70937=AXIS2_PLACEMENT_3D('',#110152,#84786,#84787) ;
#70938=AXIS2_PLACEMENT_3D('',#110153,#84788,#84789) ;
#70939=AXIS2_PLACEMENT_3D('',#110154,#84790,#84791) ;
#70940=AXIS2_PLACEMENT_3D('',#110155,#84792,#84793) ;
#70941=AXIS2_PLACEMENT_3D('',#110156,#84794,#84795) ;
#70942=AXIS2_PLACEMENT_3D('',#110157,#84796,#84797) ;
#70943=AXIS2_PLACEMENT_3D('',#110159,#84799,#84800) ;
#70944=AXIS2_PLACEMENT_3D('',#110160,#84801,#84802) ;
#70945=AXIS2_PLACEMENT_3D('',#110161,#84803,#84804) ;
#70946=AXIS2_PLACEMENT_3D('',#110162,#84805,#84806) ;
#70947=AXIS2_PLACEMENT_3D('',#110163,#84807,#84808) ;
#70948=AXIS2_PLACEMENT_3D('',#110164,#84809,#84810) ;
#70949=AXIS2_PLACEMENT_3D('',#110165,#84811,#84812) ;
#70950=AXIS2_PLACEMENT_3D('',#110166,#84813,#84814) ;
#70951=AXIS2_PLACEMENT_3D('',#110167,#84815,#84816) ;
#70952=AXIS2_PLACEMENT_3D('',#110168,#84817,#84818) ;
#70953=AXIS2_PLACEMENT_3D('',#110169,#84819,#84820) ;
#70954=AXIS2_PLACEMENT_3D('',#110170,#84821,#84822) ;
#70955=AXIS2_PLACEMENT_3D('',#110171,#84823,#84824) ;
#70956=AXIS2_PLACEMENT_3D('',#110172,#84825,#84826) ;
#70957=AXIS2_PLACEMENT_3D('',#110173,#84827,#84828) ;
#70958=AXIS2_PLACEMENT_3D('',#110174,#84829,#84830) ;
#70959=AXIS2_PLACEMENT_3D('',#110175,#84831,#84832) ;
#70960=AXIS2_PLACEMENT_3D('',#110176,#84833,#84834) ;
#70961=AXIS2_PLACEMENT_3D('',#110177,#84835,#84836) ;
#70962=AXIS2_PLACEMENT_3D('',#110178,#84837,#84838) ;
#70963=AXIS2_PLACEMENT_3D('',#110179,#84839,#84840) ;
#70964=AXIS2_PLACEMENT_3D('',#110180,#84841,#84842) ;
#70965=AXIS2_PLACEMENT_3D('',#110181,#84843,#84844) ;
#70966=AXIS2_PLACEMENT_3D('',#110182,#84845,#84846) ;
#70967=AXIS2_PLACEMENT_3D('',#110183,#84847,#84848) ;
#70968=AXIS2_PLACEMENT_3D('',#110184,#84849,#84850) ;
#70969=AXIS2_PLACEMENT_3D('',#110185,#84851,#84852) ;
#70970=AXIS2_PLACEMENT_3D('',#110186,#84853,#84854) ;
#70971=AXIS2_PLACEMENT_3D('',#110187,#84855,#84856) ;
#70972=AXIS2_PLACEMENT_3D('',#110188,#84857,#84858) ;
#70973=AXIS2_PLACEMENT_3D('',#110189,#84859,#84860) ;
#70974=AXIS2_PLACEMENT_3D('',#110190,#84861,#84862) ;
#70975=AXIS2_PLACEMENT_3D('',#110191,#84863,#84864) ;
#70976=AXIS2_PLACEMENT_3D('',#110192,#84865,#84866) ;
#70977=AXIS2_PLACEMENT_3D('',#110193,#84867,#84868) ;
#70978=AXIS2_PLACEMENT_3D('',#110194,#84869,#84870) ;
#70979=AXIS2_PLACEMENT_3D('',#110195,#84871,#84872) ;
#70980=AXIS2_PLACEMENT_3D('',#110196,#84873,#84874) ;
#70981=AXIS2_PLACEMENT_3D('',#110197,#84875,#84876) ;
#70982=AXIS2_PLACEMENT_3D('',#110198,#84877,#84878) ;
#70983=AXIS2_PLACEMENT_3D('',#110199,#84879,#84880) ;
#70984=AXIS2_PLACEMENT_3D('',#110200,#84881,#84882) ;
#70985=AXIS2_PLACEMENT_3D('',#110201,#84883,#84884) ;
#70986=AXIS2_PLACEMENT_3D('',#110202,#84885,#84886) ;
#70987=AXIS2_PLACEMENT_3D('',#110203,#84887,#84888) ;
#70988=AXIS2_PLACEMENT_3D('',#110204,#84889,#84890) ;
#70989=AXIS2_PLACEMENT_3D('',#110205,#84891,#84892) ;
#70990=AXIS2_PLACEMENT_3D('',#110206,#84893,#84894) ;
#70991=AXIS2_PLACEMENT_3D('',#110207,#84895,#84896) ;
#70992=AXIS2_PLACEMENT_3D('',#110208,#84897,#84898) ;
#70993=AXIS2_PLACEMENT_3D('',#110225,#84899,#84900) ;
#70994=AXIS2_PLACEMENT_3D('',#110226,#84901,#84902) ;
#70995=AXIS2_PLACEMENT_3D('',#110227,#84903,#84904) ;
#70996=AXIS2_PLACEMENT_3D('',#110228,#84905,#84906) ;
#70997=AXIS2_PLACEMENT_3D('',#110229,#84907,#84908) ;
#70998=AXIS2_PLACEMENT_3D('',#110230,#84909,#84910) ;
#70999=AXIS2_PLACEMENT_3D('',#110231,#84911,#84912) ;
#71000=AXIS2_PLACEMENT_3D('',#110232,#84913,#84914) ;
#71001=AXIS2_PLACEMENT_3D('',#110233,#84915,#84916) ;
#71002=AXIS2_PLACEMENT_3D('',#110234,#84917,#84918) ;
#71003=AXIS2_PLACEMENT_3D('',#110235,#84919,#84920) ;
#71004=AXIS2_PLACEMENT_3D('',#110254,#84921,#84922) ;
#71005=AXIS2_PLACEMENT_3D('',#110255,#84923,#84924) ;
#71006=AXIS2_PLACEMENT_3D('',#110257,#84925,#84926) ;
#71007=AXIS2_PLACEMENT_3D('',#110258,#84927,#84928) ;
#71008=AXIS2_PLACEMENT_3D('',#110259,#84929,#84930) ;
#71009=AXIS2_PLACEMENT_3D('',#110260,#84931,#84932) ;
#71010=AXIS2_PLACEMENT_3D('',#110261,#84933,#84934) ;
#71011=AXIS2_PLACEMENT_3D('',#110262,#84935,#84936) ;
#71012=AXIS2_PLACEMENT_3D('',#110263,#84937,#84938) ;
#71013=AXIS2_PLACEMENT_3D('',#110264,#84939,#84940) ;
#71014=AXIS2_PLACEMENT_3D('',#110265,#84941,#84942) ;
#71015=AXIS2_PLACEMENT_3D('',#110266,#84943,#84944) ;
#71016=AXIS2_PLACEMENT_3D('',#110267,#84945,#84946) ;
#71017=AXIS2_PLACEMENT_3D('',#110302,#84947,#84948) ;
#71018=AXIS2_PLACEMENT_3D('',#110303,#84949,#84950) ;
#71019=AXIS2_PLACEMENT_3D('',#110304,#84951,#84952) ;
#71020=AXIS2_PLACEMENT_3D('',#110305,#84953,#84954) ;
#71021=AXIS2_PLACEMENT_3D('',#110316,#84955,#84956) ;
#71022=AXIS2_PLACEMENT_3D('',#110317,#84957,#84958) ;
#71023=AXIS2_PLACEMENT_3D('',#110318,#84959,#84960) ;
#71024=AXIS2_PLACEMENT_3D('',#110319,#84961,#84962) ;
#71025=AXIS2_PLACEMENT_3D('',#110326,#84963,#84964) ;
#71026=AXIS2_PLACEMENT_3D('',#110327,#84965,#84966) ;
#71027=AXIS2_PLACEMENT_3D('',#110328,#84967,#84968) ;
#71028=AXIS2_PLACEMENT_3D('',#110329,#84969,#84970) ;
#71029=AXIS2_PLACEMENT_3D('',#110330,#84971,#84972) ;
#71030=AXIS2_PLACEMENT_3D('',#110341,#84973,#84974) ;
#71031=AXIS2_PLACEMENT_3D('',#110342,#84975,#84976) ;
#71032=AXIS2_PLACEMENT_3D('',#110343,#84977,#84978) ;
#71033=AXIS2_PLACEMENT_3D('',#110344,#84979,#84980) ;
#71034=AXIS2_PLACEMENT_3D('',#110345,#84981,#84982) ;
#71035=AXIS2_PLACEMENT_3D('',#110346,#84983,#84984) ;
#71036=AXIS2_PLACEMENT_3D('',#110347,#84985,#84986) ;
#71037=AXIS2_PLACEMENT_3D('',#110348,#84987,#84988) ;
#71038=AXIS2_PLACEMENT_3D('',#110349,#84989,#84990) ;
#71039=AXIS2_PLACEMENT_3D('',#110350,#84991,#84992) ;
#71040=AXIS2_PLACEMENT_3D('',#110351,#84993,#84994) ;
#71041=AXIS2_PLACEMENT_3D('',#110352,#84995,#84996) ;
#71042=AXIS2_PLACEMENT_3D('',#110353,#84997,#84998) ;
#71043=AXIS2_PLACEMENT_3D('',#110354,#84999,#85000) ;
#71044=AXIS2_PLACEMENT_3D('',#110355,#85001,#85002) ;
#71045=AXIS2_PLACEMENT_3D('',#110356,#85003,#85004) ;
#71046=AXIS2_PLACEMENT_3D('',#110357,#85005,#85006) ;
#71047=AXIS2_PLACEMENT_3D('',#110358,#85007,#85008) ;
#71048=AXIS2_PLACEMENT_3D('',#110359,#85009,#85010) ;
#71049=AXIS2_PLACEMENT_3D('',#110360,#85011,#85012) ;
#71050=AXIS2_PLACEMENT_3D('',#110361,#85013,#85014) ;
#71051=AXIS2_PLACEMENT_3D('',#110362,#85015,#85016) ;
#71052=AXIS2_PLACEMENT_3D('',#110363,#85017,#85018) ;
#71053=AXIS2_PLACEMENT_3D('',#110364,#85019,#85020) ;
#71054=AXIS2_PLACEMENT_3D('',#110365,#85021,#85022) ;
#71055=AXIS2_PLACEMENT_3D('',#110366,#85023,#85024) ;
#71056=AXIS2_PLACEMENT_3D('',#110367,#85025,#85026) ;
#71057=AXIS2_PLACEMENT_3D('',#110368,#85027,#85028) ;
#71058=AXIS2_PLACEMENT_3D('',#110369,#85029,#85030) ;
#71059=AXIS2_PLACEMENT_3D('',#110370,#85031,#85032) ;
#71060=AXIS2_PLACEMENT_3D('',#110371,#85033,#85034) ;
#71061=AXIS2_PLACEMENT_3D('',#110372,#85035,#85036) ;
#71062=AXIS2_PLACEMENT_3D('',#110373,#85037,#85038) ;
#71063=AXIS2_PLACEMENT_3D('',#110374,#85039,#85040) ;
#71064=AXIS2_PLACEMENT_3D('',#110381,#85041,#85042) ;
#71065=AXIS2_PLACEMENT_3D('',#110382,#85043,#85044) ;
#71066=AXIS2_PLACEMENT_3D('',#110383,#85045,#85046) ;
#71067=AXIS2_PLACEMENT_3D('',#110384,#85047,#85048) ;
#71068=AXIS2_PLACEMENT_3D('',#110385,#85049,#85050) ;
#71069=AXIS2_PLACEMENT_3D('',#110386,#85051,#85052) ;
#71070=AXIS2_PLACEMENT_3D('',#110387,#85053,#85054) ;
#71071=AXIS2_PLACEMENT_3D('',#110388,#85055,#85056) ;
#71072=AXIS2_PLACEMENT_3D('',#110389,#85057,#85058) ;
#71073=AXIS2_PLACEMENT_3D('',#110390,#85059,#85060) ;
#71074=AXIS2_PLACEMENT_3D('',#110391,#85061,#85062) ;
#71075=AXIS2_PLACEMENT_3D('',#110392,#85063,#85064) ;
#71076=AXIS2_PLACEMENT_3D('',#110393,#85065,#85066) ;
#71077=AXIS2_PLACEMENT_3D('',#110394,#85067,#85068) ;
#71078=AXIS2_PLACEMENT_3D('',#110395,#85069,#85070) ;
#71079=AXIS2_PLACEMENT_3D('',#110396,#85071,#85072) ;
#71080=AXIS2_PLACEMENT_3D('',#110397,#85073,#85074) ;
#71081=AXIS2_PLACEMENT_3D('',#110398,#85075,#85076) ;
#71082=AXIS2_PLACEMENT_3D('',#110399,#85077,#85078) ;
#71083=AXIS2_PLACEMENT_3D('',#110400,#85079,#85080) ;
#71084=AXIS2_PLACEMENT_3D('',#110401,#85081,#85082) ;
#71085=AXIS2_PLACEMENT_3D('',#110402,#85083,#85084) ;
#71086=AXIS2_PLACEMENT_3D('',#110403,#85085,#85086) ;
#71087=AXIS2_PLACEMENT_3D('',#110404,#85087,#85088) ;
#71088=AXIS2_PLACEMENT_3D('',#110405,#85089,#85090) ;
#71089=AXIS2_PLACEMENT_3D('',#110406,#85091,#85092) ;
#71090=AXIS2_PLACEMENT_3D('',#110407,#85093,#85094) ;
#71091=AXIS2_PLACEMENT_3D('',#110408,#85095,#85096) ;
#71092=AXIS2_PLACEMENT_3D('',#110409,#85097,#85098) ;
#71093=AXIS2_PLACEMENT_3D('',#110410,#85099,#85100) ;
#71094=AXIS2_PLACEMENT_3D('',#110411,#85101,#85102) ;
#71095=AXIS2_PLACEMENT_3D('',#110412,#85103,#85104) ;
#71096=AXIS2_PLACEMENT_3D('',#110413,#85105,#85106) ;
#71097=AXIS2_PLACEMENT_3D('',#110414,#85107,#85108) ;
#71098=AXIS2_PLACEMENT_3D('',#110415,#85109,#85110) ;
#71099=AXIS2_PLACEMENT_3D('',#110416,#85111,#85112) ;
#71100=AXIS2_PLACEMENT_3D('',#110417,#85113,#85114) ;
#71101=AXIS2_PLACEMENT_3D('',#110418,#85115,#85116) ;
#71102=AXIS2_PLACEMENT_3D('',#110419,#85117,#85118) ;
#71103=AXIS2_PLACEMENT_3D('',#110450,#85119,#85120) ;
#71104=AXIS2_PLACEMENT_3D('',#110451,#85121,#85122) ;
#71105=AXIS2_PLACEMENT_3D('',#110452,#85123,#85124) ;
#71106=AXIS2_PLACEMENT_3D('',#110453,#85125,#85126) ;
#71107=AXIS2_PLACEMENT_3D('',#110454,#85127,#85128) ;
#71108=AXIS2_PLACEMENT_3D('',#110455,#85129,#85130) ;
#71109=AXIS2_PLACEMENT_3D('',#110456,#85131,#85132) ;
#71110=AXIS2_PLACEMENT_3D('',#110457,#85133,#85134) ;
#71111=AXIS2_PLACEMENT_3D('',#110458,#85135,#85136) ;
#71112=AXIS2_PLACEMENT_3D('',#110459,#85137,#85138) ;
#71113=AXIS2_PLACEMENT_3D('',#110486,#85139,#85140) ;
#71114=AXIS2_PLACEMENT_3D('',#110487,#85141,#85142) ;
#71115=AXIS2_PLACEMENT_3D('',#110488,#85143,#85144) ;
#71116=AXIS2_PLACEMENT_3D('',#110489,#85145,#85146) ;
#71117=AXIS2_PLACEMENT_3D('',#110490,#85147,#85148) ;
#71118=AXIS2_PLACEMENT_3D('',#110491,#85149,#85150) ;
#71119=AXIS2_PLACEMENT_3D('',#110492,#85151,#85152) ;
#71120=AXIS2_PLACEMENT_3D('',#110493,#85153,#85154) ;
#71121=AXIS2_PLACEMENT_3D('',#110494,#85155,#85156) ;
#71122=AXIS2_PLACEMENT_3D('',#110495,#85157,#85158) ;
#71123=AXIS2_PLACEMENT_3D('',#110496,#85159,#85160) ;
#71124=AXIS2_PLACEMENT_3D('',#110497,#85161,#85162) ;
#71125=AXIS2_PLACEMENT_3D('',#110498,#85163,#85164) ;
#71126=AXIS2_PLACEMENT_3D('',#110499,#85165,#85166) ;
#71127=AXIS2_PLACEMENT_3D('',#110500,#85167,#85168) ;
#71128=AXIS2_PLACEMENT_3D('',#110501,#85169,#85170) ;
#71129=AXIS2_PLACEMENT_3D('',#110502,#85171,#85172) ;
#71130=AXIS2_PLACEMENT_3D('',#110503,#85173,#85174) ;
#71131=AXIS2_PLACEMENT_3D('',#110504,#85175,#85176) ;
#71132=AXIS2_PLACEMENT_3D('',#110505,#85177,#85178) ;
#71133=AXIS2_PLACEMENT_3D('',#110506,#85179,#85180) ;
#71134=AXIS2_PLACEMENT_3D('',#110507,#85181,#85182) ;
#71135=AXIS2_PLACEMENT_3D('',#110508,#85183,#85184) ;
#71136=AXIS2_PLACEMENT_3D('',#110509,#85185,#85186) ;
#71137=AXIS2_PLACEMENT_3D('',#110510,#85187,#85188) ;
#71138=AXIS2_PLACEMENT_3D('',#110511,#85189,#85190) ;
#71139=AXIS2_PLACEMENT_3D('',#110512,#85191,#85192) ;
#71140=AXIS2_PLACEMENT_3D('',#110513,#85193,#85194) ;
#71141=AXIS2_PLACEMENT_3D('',#110514,#85195,#85196) ;
#71142=AXIS2_PLACEMENT_3D('',#110539,#85197,#85198) ;
#71143=AXIS2_PLACEMENT_3D('',#110540,#85199,#85200) ;
#71144=AXIS2_PLACEMENT_3D('',#110541,#85201,#85202) ;
#71145=AXIS2_PLACEMENT_3D('',#110542,#85203,#85204) ;
#71146=AXIS2_PLACEMENT_3D('',#110543,#85205,#85206) ;
#71147=AXIS2_PLACEMENT_3D('',#110544,#85207,#85208) ;
#71148=AXIS2_PLACEMENT_3D('',#110545,#85209,#85210) ;
#71149=AXIS2_PLACEMENT_3D('',#110594,#85211,#85212) ;
#71150=AXIS2_PLACEMENT_3D('',#110595,#85213,#85214) ;
#71151=AXIS2_PLACEMENT_3D('',#110596,#85215,#85216) ;
#71152=AXIS2_PLACEMENT_3D('',#110597,#85217,#85218) ;
#71153=AXIS2_PLACEMENT_3D('',#110598,#85219,#85220) ;
#71154=AXIS2_PLACEMENT_3D('',#110599,#85221,#85222) ;
#71155=AXIS2_PLACEMENT_3D('',#110600,#85223,#85224) ;
#71156=AXIS2_PLACEMENT_3D('',#110662,#85225,#85226) ;
#71157=AXIS2_PLACEMENT_3D('',#110663,#85227,#85228) ;
#71158=AXIS2_PLACEMENT_3D('',#110664,#85229,#85230) ;
#71159=AXIS2_PLACEMENT_3D('',#110837,#85231,#85232) ;
#71160=AXIS2_PLACEMENT_3D('',#110838,#85233,#85234) ;
#71161=AXIS2_PLACEMENT_3D('',#110893,#85235,#85236) ;
#71162=AXIS2_PLACEMENT_3D('',#110940,#85237,#85238) ;
#71163=AXIS2_PLACEMENT_3D('',#110941,#85239,#85240) ;
#71164=AXIS2_PLACEMENT_3D('',#110942,#85241,#85242) ;
#71165=AXIS2_PLACEMENT_3D('',#110943,#85243,#85244) ;
#71166=AXIS2_PLACEMENT_3D('',#110944,#85245,#85246) ;
#71167=AXIS2_PLACEMENT_3D('',#110945,#85247,#85248) ;
#71168=AXIS2_PLACEMENT_3D('',#111050,#85249,#85250) ;
#71169=AXIS2_PLACEMENT_3D('',#111051,#85251,#85252) ;
#71170=AXIS2_PLACEMENT_3D('',#111052,#85253,#85254) ;
#71171=AXIS2_PLACEMENT_3D('',#111053,#85255,#85256) ;
#71172=AXIS2_PLACEMENT_3D('',#111066,#85257,#85258) ;
#71173=AXIS2_PLACEMENT_3D('',#111067,#85259,#85260) ;
#71174=AXIS2_PLACEMENT_3D('',#111068,#85261,#85262) ;
#71175=AXIS2_PLACEMENT_3D('',#111069,#85263,#85264) ;
#71176=AXIS2_PLACEMENT_3D('',#111070,#85265,#85266) ;
#71177=AXIS2_PLACEMENT_3D('',#111071,#85267,#85268) ;
#71178=AXIS2_PLACEMENT_3D('',#111072,#85269,#85270) ;
#71179=AXIS2_PLACEMENT_3D('',#111073,#85271,#85272) ;
#71180=AXIS2_PLACEMENT_3D('',#111074,#85273,#85274) ;
#71181=AXIS2_PLACEMENT_3D('',#111075,#85275,#85276) ;
#71182=AXIS2_PLACEMENT_3D('',#111076,#85277,#85278) ;
#71183=AXIS2_PLACEMENT_3D('',#111077,#85279,#85280) ;
#71184=AXIS2_PLACEMENT_3D('',#111078,#85281,#85282) ;
#71185=AXIS2_PLACEMENT_3D('',#111079,#85283,#85284) ;
#71186=AXIS2_PLACEMENT_3D('',#111080,#85285,#85286) ;
#71187=AXIS2_PLACEMENT_3D('',#111081,#85287,#85288) ;
#71188=AXIS2_PLACEMENT_3D('',#111082,#85289,#85290) ;
#71189=AXIS2_PLACEMENT_3D('',#111083,#85291,#85292) ;
#71190=AXIS2_PLACEMENT_3D('',#111084,#85293,#85294) ;
#71191=AXIS2_PLACEMENT_3D('',#111085,#85295,#85296) ;
#71192=AXIS2_PLACEMENT_3D('',#111086,#85297,#85298) ;
#71193=AXIS2_PLACEMENT_3D('',#111087,#85299,#85300) ;
#71194=AXIS2_PLACEMENT_3D('',#111088,#85301,#85302) ;
#71195=AXIS2_PLACEMENT_3D('',#111089,#85303,#85304) ;
#71196=AXIS2_PLACEMENT_3D('',#111090,#85305,#85306) ;
#71197=AXIS2_PLACEMENT_3D('',#111091,#85307,#85308) ;
#71198=AXIS2_PLACEMENT_3D('',#111092,#85309,#85310) ;
#71199=AXIS2_PLACEMENT_3D('',#111093,#85311,#85312) ;
#71200=AXIS2_PLACEMENT_3D('',#111094,#85313,#85314) ;
#71201=AXIS2_PLACEMENT_3D('',#111095,#85315,#85316) ;
#71202=AXIS2_PLACEMENT_3D('',#111096,#85317,#85318) ;
#71203=AXIS2_PLACEMENT_3D('',#111097,#85319,#85320) ;
#71204=AXIS2_PLACEMENT_3D('',#111098,#85321,#85322) ;
#71205=AXIS2_PLACEMENT_3D('',#111099,#85323,#85324) ;
#71206=AXIS2_PLACEMENT_3D('',#111100,#85325,#85326) ;
#71207=AXIS2_PLACEMENT_3D('',#111101,#85327,#85328) ;
#71208=AXIS2_PLACEMENT_3D('',#111102,#85329,#85330) ;
#71209=AXIS2_PLACEMENT_3D('',#111103,#85331,#85332) ;
#71210=AXIS2_PLACEMENT_3D('',#111116,#85333,#85334) ;
#71211=AXIS2_PLACEMENT_3D('',#111117,#85335,#85336) ;
#71212=AXIS2_PLACEMENT_3D('',#111118,#85337,#85338) ;
#71213=AXIS2_PLACEMENT_3D('',#111119,#85339,#85340) ;
#71214=AXIS2_PLACEMENT_3D('',#111174,#85341,#85342) ;
#71215=AXIS2_PLACEMENT_3D('',#111175,#85343,#85344) ;
#71216=AXIS2_PLACEMENT_3D('',#111176,#85345,#85346) ;
#71217=AXIS2_PLACEMENT_3D('',#111231,#85347,#85348) ;
#71218=AXIS2_PLACEMENT_3D('',#111232,#85349,#85350) ;
#71219=AXIS2_PLACEMENT_3D('',#111258,#85351,#85352) ;
#71220=AXIS2_PLACEMENT_3D('',#111260,#85353,#85354) ;
#71221=AXIS2_PLACEMENT_3D('',#111262,#85355,#85356) ;
#71222=AXIS2_PLACEMENT_3D('',#111301,#85357,#85358) ;
#71223=AXIS2_PLACEMENT_3D('',#111303,#85359,#85360) ;
#71224=AXIS2_PLACEMENT_3D('',#111305,#85361,#85362) ;
#71225=AXIS2_PLACEMENT_3D('',#111306,#85363,#85364) ;
#71226=AXIS2_PLACEMENT_3D('',#111307,#85365,#85366) ;
#71227=AXIS2_PLACEMENT_3D('',#111309,#85367,#85368) ;
#71228=AXIS2_PLACEMENT_3D('',#111311,#85369,#85370) ;
#71229=AXIS2_PLACEMENT_3D('',#111312,#85371,#85372) ;
#71230=AXIS2_PLACEMENT_3D('',#111313,#85373,#85374) ;
#71231=AXIS2_PLACEMENT_3D('',#111315,#85375,#85376) ;
#71232=AXIS2_PLACEMENT_3D('',#111317,#85377,#85378) ;
#71233=AXIS2_PLACEMENT_3D('',#111318,#85379,#85380) ;
#71234=AXIS2_PLACEMENT_3D('',#111319,#85381,#85382) ;
#71235=AXIS2_PLACEMENT_3D('',#111322,#85383,#85384) ;
#71236=AXIS2_PLACEMENT_3D('',#111326,#85386,#85387) ;
#71237=AXIS2_PLACEMENT_3D('',#111328,#85388,#85389) ;
#71238=AXIS2_PLACEMENT_3D('',#111330,#85391,#85392) ;
#71239=AXIS2_PLACEMENT_3D('',#111333,#85393,#85394) ;
#71240=AXIS2_PLACEMENT_3D('',#111337,#85396,#85397) ;
#71241=AXIS2_PLACEMENT_3D('',#111339,#85399,#85400) ;
#71242=AXIS2_PLACEMENT_3D('',#111342,#85401,#85402) ;
#71243=AXIS2_PLACEMENT_3D('',#111344,#85403,#85404) ;
#71244=AXIS2_PLACEMENT_3D('',#111346,#85405,#85406) ;
#71245=AXIS2_PLACEMENT_3D('',#111347,#85407,#85408) ;
#71246=AXIS2_PLACEMENT_3D('',#111348,#85409,#85410) ;
#71247=AXIS2_PLACEMENT_3D('',#111350,#85412,#85413) ;
#71248=AXIS2_PLACEMENT_3D('',#111353,#85415,#85416) ;
#71249=AXIS2_PLACEMENT_3D('',#111362,#85417,#85418) ;
#71250=AXIS2_PLACEMENT_3D('',#111370,#85419,#85420) ;
#71251=AXIS2_PLACEMENT_3D('',#111372,#85422,#85423) ;
#71252=AXIS2_PLACEMENT_3D('',#111388,#85427,#85428) ;
#71253=AXIS2_PLACEMENT_3D('',#111390,#85430,#85431) ;
#71254=AXIS2_PLACEMENT_3D('',#111439,#85436,#85437) ;
#71255=AXIS2_PLACEMENT_3D('',#111448,#85442,#85443) ;
#71256=AXIS2_PLACEMENT_3D('',#111478,#85448,#85449) ;
#71257=AXIS2_PLACEMENT_3D('',#111487,#85454,#85455) ;
#71258=AXIS2_PLACEMENT_3D('',#111496,#85460,#85461) ;
#71259=AXIS2_PLACEMENT_3D('',#111507,#85466,#85467) ;
#71260=AXIS2_PLACEMENT_3D('',#111509,#85469,#85470) ;
#71261=AXIS2_PLACEMENT_3D('',#111513,#85472,#85473) ;
#71262=AXIS2_PLACEMENT_3D('',#111514,#85474,#85475) ;
#71263=AXIS2_PLACEMENT_3D('',#111515,#85476,#85477) ;
#71264=AXIS2_PLACEMENT_3D('',#111517,#85478,#85479) ;
#71265=AXIS2_PLACEMENT_3D('',#111521,#85481,#85482) ;
#71266=AXIS2_PLACEMENT_3D('',#111525,#85484,#85485) ;
#71267=AXIS2_PLACEMENT_3D('',#111529,#85487,#85488) ;
#71268=AXIS2_PLACEMENT_3D('',#111533,#85490,#85491) ;
#71269=AXIS2_PLACEMENT_3D('',#111537,#85493,#85494) ;
#71270=AXIS2_PLACEMENT_3D('',#111540,#85496,#85497) ;
#71271=AXIS2_PLACEMENT_3D('',#111542,#85498,#85499) ;
#71272=AXIS2_PLACEMENT_3D('',#111545,#85501,#85502) ;
#71273=AXIS2_PLACEMENT_3D('',#111547,#85503,#85504) ;
#71274=AXIS2_PLACEMENT_3D('',#111553,#85507,#85508) ;
#71275=AXIS2_PLACEMENT_3D('',#111557,#85510,#85511) ;
#71276=AXIS2_PLACEMENT_3D('',#111560,#85513,#85514) ;
#71277=AXIS2_PLACEMENT_3D('',#111561,#85515,#85516) ;
#71278=AXIS2_PLACEMENT_3D('',#111566,#85518,#85519) ;
#71279=AXIS2_PLACEMENT_3D('',#111570,#85521,#85522) ;
#71280=AXIS2_PLACEMENT_3D('',#111574,#85524,#85525) ;
#71281=AXIS2_PLACEMENT_3D('',#111578,#85527,#85528) ;
#71282=AXIS2_PLACEMENT_3D('',#111583,#85531,#85532) ;
#71283=AXIS2_PLACEMENT_3D('',#111585,#85533,#85534) ;
#71284=AXIS2_PLACEMENT_3D('',#111588,#85536,#85537) ;
#71285=AXIS2_PLACEMENT_3D('',#111590,#85538,#85539) ;
#71286=AXIS2_PLACEMENT_3D('',#111594,#85541,#85542) ;
#71287=AXIS2_PLACEMENT_3D('',#111598,#85544,#85545) ;
#71288=AXIS2_PLACEMENT_3D('',#111602,#85547,#85548) ;
#71289=AXIS2_PLACEMENT_3D('',#111606,#85550,#85551) ;
#71290=AXIS2_PLACEMENT_3D('',#111610,#85553,#85554) ;
#71291=AXIS2_PLACEMENT_3D('',#111614,#85556,#85557) ;
#71292=AXIS2_PLACEMENT_3D('',#111618,#85559,#85560) ;
#71293=AXIS2_PLACEMENT_3D('',#111621,#85562,#85563) ;
#71294=AXIS2_PLACEMENT_3D('',#111622,#85564,#85565) ;
#71295=AXIS2_PLACEMENT_3D('',#111625,#85568,#85569) ;
#71296=AXIS2_PLACEMENT_3D('',#111628,#85572,#85573) ;
#71297=AXIS2_PLACEMENT_3D('',#111717,#85578,#85579) ;
#71298=AXIS2_PLACEMENT_3D('',#111728,#85580,#85581) ;
#71299=AXIS2_PLACEMENT_3D('',#111733,#85585,#85586) ;
#71300=AXIS2_PLACEMENT_3D('',#111739,#85590,#85591) ;
#71301=AXIS2_PLACEMENT_3D('',#111759,#85595,#85596) ;
#71302=AXIS2_PLACEMENT_3D('',#111858,#85602,#85603) ;
#71303=AXIS2_PLACEMENT_3D('',#111862,#85605,#85606) ;
#71304=AXIS2_PLACEMENT_3D('',#111866,#85609,#85610) ;
#71305=AXIS2_PLACEMENT_3D('',#111869,#85611,#85612) ;
#71306=AXIS2_PLACEMENT_3D('',#111874,#85615,#85616) ;
#71307=AXIS2_PLACEMENT_3D('',#111876,#85617,#85618) ;
#71308=AXIS2_PLACEMENT_3D('',#111878,#85619,#85620) ;
#71309=AXIS2_PLACEMENT_3D('',#111886,#85624,#85625) ;
#71310=AXIS2_PLACEMENT_3D('',#111888,#85626,#85627) ;
#71311=AXIS2_PLACEMENT_3D('',#111890,#85628,#85629) ;
#71312=AXIS2_PLACEMENT_3D('',#111895,#85632,#85633) ;
#71313=AXIS2_PLACEMENT_3D('',#111897,#85634,#85635) ;
#71314=AXIS2_PLACEMENT_3D('',#111899,#85636,#85637) ;
#71315=AXIS2_PLACEMENT_3D('',#111903,#85639,#85640) ;
#71316=AXIS2_PLACEMENT_3D('',#111907,#85642,#85643) ;
#71317=AXIS2_PLACEMENT_3D('',#111908,#85644,#85645) ;
#71318=AXIS2_PLACEMENT_3D('',#111909,#85646,#85647) ;
#71319=AXIS2_PLACEMENT_3D('',#111912,#85648,#85649) ;
#71320=AXIS2_PLACEMENT_3D('',#111922,#85655,#85656) ;
#71321=AXIS2_PLACEMENT_3D('',#111924,#85658,#85659) ;
#71322=AXIS2_PLACEMENT_3D('',#111927,#85660,#85661) ;
#71323=AXIS2_PLACEMENT_3D('',#111933,#85665,#85666) ;
#71324=AXIS2_PLACEMENT_3D('',#111935,#85668,#85669) ;
#71325=AXIS2_PLACEMENT_3D('',#111941,#85672,#85673) ;
#71326=AXIS2_PLACEMENT_3D('',#111942,#85674,#85675) ;
#71327=AXIS2_PLACEMENT_3D('',#111945,#85676,#85677) ;
#71328=AXIS2_PLACEMENT_3D('',#111949,#85680,#85681) ;
#71329=AXIS2_PLACEMENT_3D('',#111966,#85690,#85691) ;
#71330=AXIS2_PLACEMENT_3D('',#111975,#85696,#85697) ;
#71331=AXIS2_PLACEMENT_3D('',#111984,#85702,#85703) ;
#71332=AXIS2_PLACEMENT_3D('',#111993,#85708,#85709) ;
#71333=AXIS2_PLACEMENT_3D('',#112020,#85714,#85715) ;
#71334=AXIS2_PLACEMENT_3D('',#112037,#85724,#85725) ;
#71335=AXIS2_PLACEMENT_3D('',#112042,#85727,#85728) ;
#71336=AXIS2_PLACEMENT_3D('',#112046,#85730,#85731) ;
#71337=AXIS2_PLACEMENT_3D('',#112050,#85733,#85734) ;
#71338=AXIS2_PLACEMENT_3D('',#112053,#85736,#85737) ;
#71339=AXIS2_PLACEMENT_3D('',#112054,#85738,#85739) ;
#71340=AXIS2_PLACEMENT_3D('',#112057,#85740,#85741) ;
#71341=AXIS2_PLACEMENT_3D('',#112062,#85744,#85745) ;
#71342=AXIS2_PLACEMENT_3D('',#112065,#85747,#85748) ;
#71343=AXIS2_PLACEMENT_3D('',#112066,#85749,#85750) ;
#71344=AXIS2_PLACEMENT_3D('',#112072,#85754,#85755) ;
#71345=AXIS2_PLACEMENT_3D('',#112078,#85759,#85760) ;
#71346=AXIS2_PLACEMENT_3D('',#112081,#85761,#85762) ;
#71347=AXIS2_PLACEMENT_3D('',#112085,#85764,#85765) ;
#71348=AXIS2_PLACEMENT_3D('',#112087,#85767,#85768) ;
#71349=AXIS2_PLACEMENT_3D('',#112090,#85769,#85770) ;
#71350=AXIS2_PLACEMENT_3D('',#112094,#85772,#85773) ;
#71351=AXIS2_PLACEMENT_3D('',#112096,#85775,#85776) ;
#71352=AXIS2_PLACEMENT_3D('',#112102,#85780,#85781) ;
#71353=AXIS2_PLACEMENT_3D('',#112108,#85785,#85786) ;
#71354=AXIS2_PLACEMENT_3D('',#112111,#85787,#85788) ;
#71355=AXIS2_PLACEMENT_3D('',#112116,#85791,#85792) ;
#71356=AXIS2_PLACEMENT_3D('',#112118,#85793,#85794) ;
#71357=AXIS2_PLACEMENT_3D('',#112120,#85796,#85797) ;
#71358=AXIS2_PLACEMENT_3D('',#112123,#85798,#85799) ;
#71359=AXIS2_PLACEMENT_3D('',#112128,#85803,#85804) ;
#71360=AXIS2_PLACEMENT_3D('',#112134,#85808,#85809) ;
#71361=AXIS2_PLACEMENT_3D('',#112137,#85810,#85811) ;
#71362=AXIS2_PLACEMENT_3D('',#112141,#85813,#85814) ;
#71363=AXIS2_PLACEMENT_3D('',#112143,#85816,#85817) ;
#71364=AXIS2_PLACEMENT_3D('',#112152,#85822,#85823) ;
#71365=AXIS2_PLACEMENT_3D('',#112155,#85824,#85825) ;
#71366=AXIS2_PLACEMENT_3D('',#112159,#85827,#85828) ;
#71367=AXIS2_PLACEMENT_3D('',#112161,#85830,#85831) ;
#71368=AXIS2_PLACEMENT_3D('',#112167,#85835,#85836) ;
#71369=AXIS2_PLACEMENT_3D('',#112176,#85841,#85842) ;
#71370=AXIS2_PLACEMENT_3D('',#112183,#85846,#85847) ;
#71371=AXIS2_PLACEMENT_3D('',#112184,#85848,#85849) ;
#71372=AXIS2_PLACEMENT_3D('',#112193,#85854,#85855) ;
#71373=AXIS2_PLACEMENT_3D('',#112196,#85856,#85857) ;
#71374=AXIS2_PLACEMENT_3D('',#112201,#85860,#85861) ;
#71375=AXIS2_PLACEMENT_3D('',#112205,#85863,#85864) ;
#71376=AXIS2_PLACEMENT_3D('',#112207,#85866,#85867) ;
#71377=AXIS2_PLACEMENT_3D('',#112215,#85872,#85873) ;
#71378=AXIS2_PLACEMENT_3D('',#112224,#85878,#85879) ;
#71379=AXIS2_PLACEMENT_3D('',#112233,#85884,#85885) ;
#71380=AXIS2_PLACEMENT_3D('',#112242,#85890,#85891) ;
#71381=AXIS2_PLACEMENT_3D('',#112248,#85895,#85896) ;
#71382=AXIS2_PLACEMENT_3D('',#112254,#85900,#85901) ;
#71383=AXIS2_PLACEMENT_3D('',#112260,#85905,#85906) ;
#71384=AXIS2_PLACEMENT_3D('',#112266,#85910,#85911) ;
#71385=AXIS2_PLACEMENT_3D('',#112275,#85915,#85916) ;
#71386=AXIS2_PLACEMENT_3D('',#112278,#85918,#85919) ;
#71387=AXIS2_PLACEMENT_3D('',#112279,#85920,#85921) ;
#71388=AXIS2_PLACEMENT_3D('',#112288,#85925,#85926) ;
#71389=AXIS2_PLACEMENT_3D('',#112291,#85928,#85929) ;
#71390=AXIS2_PLACEMENT_3D('',#112292,#85930,#85931) ;
#71391=AXIS2_PLACEMENT_3D('',#112296,#85933,#85934) ;
#71392=AXIS2_PLACEMENT_3D('',#112297,#85935,#85936) ;
#71393=AXIS2_PLACEMENT_3D('',#112298,#85937,#85938) ;
#71394=AXIS2_PLACEMENT_3D('',#112304,#85942,#85943) ;
#71395=AXIS2_PLACEMENT_3D('',#112313,#85948,#85949) ;
#71396=AXIS2_PLACEMENT_3D('',#112322,#85954,#85955) ;
#71397=AXIS2_PLACEMENT_3D('',#112331,#85960,#85961) ;
#71398=AXIS2_PLACEMENT_3D('',#112340,#85966,#85967) ;
#71399=AXIS2_PLACEMENT_3D('',#112341,#85968,#85969) ;
#71400=AXIS2_PLACEMENT_3D('',#112342,#85970,#85971) ;
#71401=AXIS2_PLACEMENT_3D('',#112343,#85972,#85973) ;
#71402=AXIS2_PLACEMENT_3D('',#112352,#85978,#85979) ;
#71403=AXIS2_PLACEMENT_3D('',#112361,#85984,#85985) ;
#71404=AXIS2_PLACEMENT_3D('',#112370,#85990,#85991) ;
#71405=AXIS2_PLACEMENT_3D('',#112379,#85996,#85997) ;
#71406=AXIS2_PLACEMENT_3D('',#112383,#85999,#86000) ;
#71407=AXIS2_PLACEMENT_3D('',#112385,#86002,#86003) ;
#71408=AXIS2_PLACEMENT_3D('',#112388,#86004,#86005) ;
#71409=AXIS2_PLACEMENT_3D('',#112389,#86006,#86007) ;
#71410=AXIS2_PLACEMENT_3D('',#112390,#86008,#86009) ;
#71411=AXIS2_PLACEMENT_3D('',#112391,#86010,#86011) ;
#71412=AXIS2_PLACEMENT_3D('',#112395,#86013,#86014) ;
#71413=AXIS2_PLACEMENT_3D('',#112397,#86016,#86017) ;
#71414=AXIS2_PLACEMENT_3D('',#112398,#86018,#86019) ;
#71415=AXIS2_PLACEMENT_3D('',#112399,#86020,#86021) ;
#71416=AXIS2_PLACEMENT_3D('',#112400,#86022,#86023) ;
#71417=AXIS2_PLACEMENT_3D('',#112401,#86024,#86025) ;
#71418=AXIS2_PLACEMENT_3D('',#112402,#86026,#86027) ;
#71419=AXIS2_PLACEMENT_3D('',#112403,#86028,#86029) ;
#71420=AXIS2_PLACEMENT_3D('',#112404,#86030,#86031) ;
#71421=AXIS2_PLACEMENT_3D('',#112405,#86032,#86033) ;
#71422=AXIS2_PLACEMENT_3D('',#112406,#86034,#86035) ;
#71423=AXIS2_PLACEMENT_3D('',#112407,#86036,#86037) ;
#71424=AXIS2_PLACEMENT_3D('',#112408,#86038,#86039) ;
#71425=AXIS2_PLACEMENT_3D('',#112409,#86040,#86041) ;
#71426=AXIS2_PLACEMENT_3D('',#112410,#86042,#86043) ;
#71427=AXIS2_PLACEMENT_3D('',#112411,#86044,#86045) ;
#71428=AXIS2_PLACEMENT_3D('',#112412,#86046,#86047) ;
#71429=AXIS2_PLACEMENT_3D('',#112413,#86048,#86049) ;
#71430=AXIS2_PLACEMENT_3D('',#112414,#86050,#86051) ;
#71431=AXIS2_PLACEMENT_3D('',#112415,#86052,#86053) ;
#71432=AXIS2_PLACEMENT_3D('',#112416,#86054,#86055) ;
#71433=AXIS2_PLACEMENT_3D('',#112417,#86056,#86057) ;
#71434=AXIS2_PLACEMENT_3D('',#112418,#86058,#86059) ;
#71435=AXIS2_PLACEMENT_3D('',#112419,#86060,#86061) ;
#71436=AXIS2_PLACEMENT_3D('',#112420,#86062,#86063) ;
#71437=AXIS2_PLACEMENT_3D('',#112421,#86064,#86065) ;
#71438=AXIS2_PLACEMENT_3D('',#112422,#86066,#86067) ;
#71439=AXIS2_PLACEMENT_3D('',#112423,#86068,#86069) ;
#71440=AXIS2_PLACEMENT_3D('',#112424,#86070,#86071) ;
#71441=AXIS2_PLACEMENT_3D('',#112425,#86072,#86073) ;
#71442=AXIS2_PLACEMENT_3D('',#112426,#86074,#86075) ;
#71443=AXIS2_PLACEMENT_3D('',#112427,#86076,#86077) ;
#71444=AXIS2_PLACEMENT_3D('',#112428,#86078,#86079) ;
#71445=AXIS2_PLACEMENT_3D('',#112429,#86080,#86081) ;
#71446=AXIS2_PLACEMENT_3D('',#112430,#86082,#86083) ;
#71447=AXIS2_PLACEMENT_3D('',#112431,#86084,#86085) ;
#71448=AXIS2_PLACEMENT_3D('',#112432,#86086,#86087) ;
#71449=AXIS2_PLACEMENT_3D('',#112433,#86088,#86089) ;
#71450=AXIS2_PLACEMENT_3D('',#112434,#86090,#86091) ;
#71451=AXIS2_PLACEMENT_3D('',#112435,#86092,#86093) ;
#71452=AXIS2_PLACEMENT_3D('',#112436,#86094,#86095) ;
#71453=AXIS2_PLACEMENT_3D('',#112437,#86096,#86097) ;
#71454=AXIS2_PLACEMENT_3D('',#112438,#86098,#86099) ;
#71455=AXIS2_PLACEMENT_3D('',#112439,#86100,#86101) ;
#71456=AXIS2_PLACEMENT_3D('',#112440,#86102,#86103) ;
#71457=AXIS2_PLACEMENT_3D('',#112441,#86104,#86105) ;
#71458=AXIS2_PLACEMENT_3D('',#112442,#86106,#86107) ;
#71459=AXIS2_PLACEMENT_3D('',#112443,#86108,#86109) ;
#71460=AXIS2_PLACEMENT_3D('',#112444,#86110,#86111) ;
#71461=AXIS2_PLACEMENT_3D('',#112445,#86112,#86113) ;
#71462=AXIS2_PLACEMENT_3D('',#112446,#86114,#86115) ;
#71463=AXIS2_PLACEMENT_3D('',#112447,#86116,#86117) ;
#71464=AXIS2_PLACEMENT_3D('',#112448,#86118,#86119) ;
#71465=AXIS2_PLACEMENT_3D('',#112449,#86120,#86121) ;
#71466=AXIS2_PLACEMENT_3D('',#112450,#86122,#86123) ;
#71467=AXIS2_PLACEMENT_3D('',#112451,#86124,#86125) ;
#71468=AXIS2_PLACEMENT_3D('',#112452,#86126,#86127) ;
#71469=AXIS2_PLACEMENT_3D('',#112453,#86128,#86129) ;
#71470=AXIS2_PLACEMENT_3D('',#112454,#86130,#86131) ;
#71471=AXIS2_PLACEMENT_3D('',#112455,#86132,#86133) ;
#71472=AXIS2_PLACEMENT_3D('',#112456,#86134,#86135) ;
#71473=AXIS2_PLACEMENT_3D('',#112457,#86136,#86137) ;
#71474=AXIS2_PLACEMENT_3D('',#112458,#86138,#86139) ;
#71475=AXIS2_PLACEMENT_3D('',#112459,#86140,#86141) ;
#71476=AXIS2_PLACEMENT_3D('',#112460,#86142,#86143) ;
#71477=AXIS2_PLACEMENT_3D('',#112461,#86144,#86145) ;
#71478=AXIS2_PLACEMENT_3D('',#112462,#86146,#86147) ;
#71479=AXIS2_PLACEMENT_3D('',#112463,#86148,#86149) ;
#71480=AXIS2_PLACEMENT_3D('',#112464,#86150,#86151) ;
#71481=AXIS2_PLACEMENT_3D('',#112465,#86152,#86153) ;
#71482=AXIS2_PLACEMENT_3D('',#112466,#86154,#86155) ;
#71483=AXIS2_PLACEMENT_3D('',#112467,#86156,#86157) ;
#71484=AXIS2_PLACEMENT_3D('',#112468,#86158,#86159) ;
#71485=AXIS2_PLACEMENT_3D('',#112469,#86160,#86161) ;
#71486=AXIS2_PLACEMENT_3D('',#112470,#86162,#86163) ;
#71487=AXIS2_PLACEMENT_3D('',#112486,#86164,#86165) ;
#71488=AXIS2_PLACEMENT_3D('',#112487,#86166,#86167) ;
#71489=AXIS2_PLACEMENT_3D('',#112489,#86168,#86169) ;
#71490=AXIS2_PLACEMENT_3D('',#112504,#86170,#86171) ;
#71491=AXIS2_PLACEMENT_3D('',#112505,#86172,#86173) ;
#71492=AXIS2_PLACEMENT_3D('',#112506,#86174,#86175) ;
#71493=AXIS2_PLACEMENT_3D('',#112508,#86176,#86177) ;
#71494=AXIS2_PLACEMENT_3D('',#112538,#86178,#86179) ;
#71495=AXIS2_PLACEMENT_3D('',#112539,#86180,#86181) ;
#71496=AXIS2_PLACEMENT_3D('',#112555,#86182,#86183) ;
#71497=AXIS2_PLACEMENT_3D('',#112557,#86184,#86185) ;
#71498=AXIS2_PLACEMENT_3D('',#112572,#86186,#86187) ;
#71499=AXIS2_PLACEMENT_3D('',#112573,#86188,#86189) ;
#71500=AXIS2_PLACEMENT_3D('',#112574,#86190,#86191) ;
#71501=AXIS2_PLACEMENT_3D('',#112575,#86192,#86193) ;
#71502=AXIS2_PLACEMENT_3D('',#112578,#86195,#86196) ;
#71503=AXIS2_PLACEMENT_3D('',#112579,#86197,#86198) ;
#71504=AXIS2_PLACEMENT_3D('',#112581,#86199,#86200) ;
#71505=AXIS2_PLACEMENT_3D('',#112582,#86201,#86202) ;
#71506=AXIS2_PLACEMENT_3D('',#112583,#86203,#86204) ;
#71507=AXIS2_PLACEMENT_3D('',#112585,#86205,#86206) ;
#71508=AXIS2_PLACEMENT_3D('',#112600,#86207,#86208) ;
#71509=AXIS2_PLACEMENT_3D('',#112601,#86209,#86210) ;
#71510=AXIS2_PLACEMENT_3D('',#112617,#86211,#86212) ;
#71511=AXIS2_PLACEMENT_3D('',#112618,#86213,#86214) ;
#71512=AXIS2_PLACEMENT_3D('',#112619,#86215,#86216) ;
#71513=AXIS2_PLACEMENT_3D('',#112621,#86217,#86218) ;
#71514=AXIS2_PLACEMENT_3D('',#112623,#86220,#86221) ;
#71515=AXIS2_PLACEMENT_3D('',#112624,#86222,#86223) ;
#71516=AXIS2_PLACEMENT_3D('',#112625,#86224,#86225) ;
#71517=AXIS2_PLACEMENT_3D('',#112626,#86226,#86227) ;
#71518=AXIS2_PLACEMENT_3D('',#112627,#86228,#86229) ;
#71519=AXIS2_PLACEMENT_3D('',#112628,#86230,#86231) ;
#71520=AXIS2_PLACEMENT_3D('',#112631,#86233,#86234) ;
#71521=AXIS2_PLACEMENT_3D('',#112632,#86235,#86236) ;
#71522=AXIS2_PLACEMENT_3D('',#112633,#86237,#86238) ;
#71523=AXIS2_PLACEMENT_3D('',#112634,#86239,#86240) ;
#71524=AXIS2_PLACEMENT_3D('',#112636,#86241,#86242) ;
#71525=AXIS2_PLACEMENT_3D('',#112637,#86243,#86244) ;
#71526=AXIS2_PLACEMENT_3D('',#112638,#86245,#86246) ;
#71527=AXIS2_PLACEMENT_3D('',#112639,#86247,#86248) ;
#71528=AXIS2_PLACEMENT_3D('',#112640,#86249,#86250) ;
#71529=AXIS2_PLACEMENT_3D('',#112641,#86251,#86252) ;
#71530=AXIS2_PLACEMENT_3D('',#112642,#86253,#86254) ;
#71531=AXIS2_PLACEMENT_3D('',#112644,#86255,#86256) ;
#71532=AXIS2_PLACEMENT_3D('',#112645,#86257,#86258) ;
#71533=AXIS2_PLACEMENT_3D('',#112646,#86259,#86260) ;
#71534=AXIS2_PLACEMENT_3D('',#112647,#86261,#86262) ;
#71535=AXIS2_PLACEMENT_3D('',#112648,#86263,#86264) ;
#71536=AXIS2_PLACEMENT_3D('',#112650,#86265,#86266) ;
#71537=AXIS2_PLACEMENT_3D('',#112652,#86268,#86269) ;
#71538=AXIS2_PLACEMENT_3D('',#112653,#86270,#86271) ;
#71539=AXIS2_PLACEMENT_3D('',#112654,#86272,#86273) ;
#71540=AXIS2_PLACEMENT_3D('',#112655,#86274,#86275) ;
#71541=AXIS2_PLACEMENT_3D('',#112656,#86276,#86277) ;
#71542=AXIS2_PLACEMENT_3D('',#112658,#86279,#86280) ;
#71543=AXIS2_PLACEMENT_3D('',#112659,#86281,#86282) ;
#71544=AXIS2_PLACEMENT_3D('',#112660,#86283,#86284) ;
#71545=AXIS2_PLACEMENT_3D('',#112661,#86285,#86286) ;
#71546=AXIS2_PLACEMENT_3D('',#112663,#86287,#86288) ;
#71547=AXIS2_PLACEMENT_3D('',#112664,#86289,#86290) ;
#71548=AXIS2_PLACEMENT_3D('',#112665,#86291,#86292) ;
#71549=AXIS2_PLACEMENT_3D('',#112666,#86293,#86294) ;
#71550=AXIS2_PLACEMENT_3D('',#112667,#86295,#86296) ;
#71551=AXIS2_PLACEMENT_3D('',#112668,#86297,#86298) ;
#71552=AXIS2_PLACEMENT_3D('',#112669,#86299,#86300) ;
#71553=AXIS2_PLACEMENT_3D('',#112671,#86302,#86303) ;
#71554=AXIS2_PLACEMENT_3D('',#112672,#86304,#86305) ;
#71555=AXIS2_PLACEMENT_3D('',#112673,#86306,#86307) ;
#71556=AXIS2_PLACEMENT_3D('',#112674,#86308,#86309) ;
#71557=AXIS2_PLACEMENT_3D('',#112675,#86310,#86311) ;
#71558=AXIS2_PLACEMENT_3D('',#112676,#86312,#86313) ;
#71559=AXIS2_PLACEMENT_3D('',#112677,#86314,#86315) ;
#71560=AXIS2_PLACEMENT_3D('',#112678,#86316,#86317) ;
#71561=AXIS2_PLACEMENT_3D('',#112679,#86318,#86319) ;
#71562=AXIS2_PLACEMENT_3D('',#112680,#86320,#86321) ;
#71563=AXIS2_PLACEMENT_3D('',#112681,#86322,#86323) ;
#71564=AXIS2_PLACEMENT_3D('',#112682,#86324,#86325) ;
#71565=AXIS2_PLACEMENT_3D('',#112683,#86326,#86327) ;
#71566=AXIS2_PLACEMENT_3D('',#112684,#86328,#86329) ;
#71567=AXIS2_PLACEMENT_3D('',#112685,#86330,#86331) ;
#71568=AXIS2_PLACEMENT_3D('',#112686,#86332,#86333) ;
#71569=AXIS2_PLACEMENT_3D('',#112687,#86334,#86335) ;
#71570=AXIS2_PLACEMENT_3D('',#112688,#86336,#86337) ;
#71571=AXIS2_PLACEMENT_3D('',#112689,#86338,#86339) ;
#71572=AXIS2_PLACEMENT_3D('',#112690,#86340,#86341) ;
#71573=AXIS2_PLACEMENT_3D('',#112691,#86342,#86343) ;
#71574=AXIS2_PLACEMENT_3D('',#112692,#86344,#86345) ;
#71575=AXIS2_PLACEMENT_3D('',#112693,#86346,#86347) ;
#71576=AXIS2_PLACEMENT_3D('',#112694,#86348,#86349) ;
#71577=AXIS2_PLACEMENT_3D('',#112695,#86350,#86351) ;
#71578=AXIS2_PLACEMENT_3D('',#112696,#86352,#86353) ;
#71579=AXIS2_PLACEMENT_3D('',#112697,#86354,#86355) ;
#71580=AXIS2_PLACEMENT_3D('',#112698,#86356,#86357) ;
#71581=AXIS2_PLACEMENT_3D('',#112699,#86358,#86359) ;
#71582=AXIS2_PLACEMENT_3D('',#112700,#86360,#86361) ;
#71583=AXIS2_PLACEMENT_3D('',#112701,#86362,#86363) ;
#71584=AXIS2_PLACEMENT_3D('',#112702,#86364,#86365) ;
#71585=AXIS2_PLACEMENT_3D('',#112703,#86366,#86367) ;
#71586=AXIS2_PLACEMENT_3D('',#112704,#86368,#86369) ;
#71587=AXIS2_PLACEMENT_3D('',#112705,#86370,#86371) ;
#71588=AXIS2_PLACEMENT_3D('',#112706,#86372,#86373) ;
#71589=AXIS2_PLACEMENT_3D('',#112707,#86374,#86375) ;
#71590=AXIS2_PLACEMENT_3D('',#112708,#86376,#86377) ;
#71591=AXIS2_PLACEMENT_3D('',#112709,#86378,#86379) ;
#71592=AXIS2_PLACEMENT_3D('',#112710,#86380,#86381) ;
#71593=AXIS2_PLACEMENT_3D('',#112711,#86382,#86383) ;
#71594=AXIS2_PLACEMENT_3D('',#112712,#86384,#86385) ;
#71595=AXIS2_PLACEMENT_3D('',#112713,#86386,#86387) ;
#71596=AXIS2_PLACEMENT_3D('',#112714,#86388,#86389) ;
#71597=AXIS2_PLACEMENT_3D('',#112715,#86390,#86391) ;
#71598=AXIS2_PLACEMENT_3D('',#112716,#86392,#86393) ;
#71599=AXIS2_PLACEMENT_3D('',#112717,#86394,#86395) ;
#71600=AXIS2_PLACEMENT_3D('',#112718,#86396,#86397) ;
#71601=AXIS2_PLACEMENT_3D('',#112719,#86398,#86399) ;
#71602=AXIS2_PLACEMENT_3D('',#112720,#86400,#86401) ;
#71603=AXIS2_PLACEMENT_3D('',#112737,#86402,#86403) ;
#71604=AXIS2_PLACEMENT_3D('',#112738,#86404,#86405) ;
#71605=AXIS2_PLACEMENT_3D('',#112739,#86406,#86407) ;
#71606=AXIS2_PLACEMENT_3D('',#112740,#86408,#86409) ;
#71607=AXIS2_PLACEMENT_3D('',#112741,#86410,#86411) ;
#71608=AXIS2_PLACEMENT_3D('',#112742,#86412,#86413) ;
#71609=AXIS2_PLACEMENT_3D('',#112743,#86414,#86415) ;
#71610=AXIS2_PLACEMENT_3D('',#112744,#86416,#86417) ;
#71611=AXIS2_PLACEMENT_3D('',#112745,#86418,#86419) ;
#71612=AXIS2_PLACEMENT_3D('',#112746,#86420,#86421) ;
#71613=AXIS2_PLACEMENT_3D('',#112747,#86422,#86423) ;
#71614=AXIS2_PLACEMENT_3D('',#112766,#86424,#86425) ;
#71615=AXIS2_PLACEMENT_3D('',#112767,#86426,#86427) ;
#71616=AXIS2_PLACEMENT_3D('',#112769,#86428,#86429) ;
#71617=AXIS2_PLACEMENT_3D('',#112770,#86430,#86431) ;
#71618=AXIS2_PLACEMENT_3D('',#112771,#86432,#86433) ;
#71619=AXIS2_PLACEMENT_3D('',#112772,#86434,#86435) ;
#71620=AXIS2_PLACEMENT_3D('',#112773,#86436,#86437) ;
#71621=AXIS2_PLACEMENT_3D('',#112774,#86438,#86439) ;
#71622=AXIS2_PLACEMENT_3D('',#112775,#86440,#86441) ;
#71623=AXIS2_PLACEMENT_3D('',#112776,#86442,#86443) ;
#71624=AXIS2_PLACEMENT_3D('',#112777,#86444,#86445) ;
#71625=AXIS2_PLACEMENT_3D('',#112778,#86446,#86447) ;
#71626=AXIS2_PLACEMENT_3D('',#112779,#86448,#86449) ;
#71627=AXIS2_PLACEMENT_3D('',#112814,#86450,#86451) ;
#71628=AXIS2_PLACEMENT_3D('',#112815,#86452,#86453) ;
#71629=AXIS2_PLACEMENT_3D('',#112816,#86454,#86455) ;
#71630=AXIS2_PLACEMENT_3D('',#112817,#86456,#86457) ;
#71631=AXIS2_PLACEMENT_3D('',#112828,#86458,#86459) ;
#71632=AXIS2_PLACEMENT_3D('',#112829,#86460,#86461) ;
#71633=AXIS2_PLACEMENT_3D('',#112830,#86462,#86463) ;
#71634=AXIS2_PLACEMENT_3D('',#112831,#86464,#86465) ;
#71635=AXIS2_PLACEMENT_3D('',#112838,#86466,#86467) ;
#71636=AXIS2_PLACEMENT_3D('',#112839,#86468,#86469) ;
#71637=AXIS2_PLACEMENT_3D('',#112840,#86470,#86471) ;
#71638=AXIS2_PLACEMENT_3D('',#112841,#86472,#86473) ;
#71639=AXIS2_PLACEMENT_3D('',#112842,#86474,#86475) ;
#71640=AXIS2_PLACEMENT_3D('',#112853,#86476,#86477) ;
#71641=AXIS2_PLACEMENT_3D('',#112854,#86478,#86479) ;
#71642=AXIS2_PLACEMENT_3D('',#112855,#86480,#86481) ;
#71643=AXIS2_PLACEMENT_3D('',#112856,#86482,#86483) ;
#71644=AXIS2_PLACEMENT_3D('',#112857,#86484,#86485) ;
#71645=AXIS2_PLACEMENT_3D('',#112858,#86486,#86487) ;
#71646=AXIS2_PLACEMENT_3D('',#112859,#86488,#86489) ;
#71647=AXIS2_PLACEMENT_3D('',#112860,#86490,#86491) ;
#71648=AXIS2_PLACEMENT_3D('',#112861,#86492,#86493) ;
#71649=AXIS2_PLACEMENT_3D('',#112862,#86494,#86495) ;
#71650=AXIS2_PLACEMENT_3D('',#112863,#86496,#86497) ;
#71651=AXIS2_PLACEMENT_3D('',#112864,#86498,#86499) ;
#71652=AXIS2_PLACEMENT_3D('',#112865,#86500,#86501) ;
#71653=AXIS2_PLACEMENT_3D('',#112866,#86502,#86503) ;
#71654=AXIS2_PLACEMENT_3D('',#112867,#86504,#86505) ;
#71655=AXIS2_PLACEMENT_3D('',#112868,#86506,#86507) ;
#71656=AXIS2_PLACEMENT_3D('',#112869,#86508,#86509) ;
#71657=AXIS2_PLACEMENT_3D('',#112870,#86510,#86511) ;
#71658=AXIS2_PLACEMENT_3D('',#112871,#86512,#86513) ;
#71659=AXIS2_PLACEMENT_3D('',#112872,#86514,#86515) ;
#71660=AXIS2_PLACEMENT_3D('',#112873,#86516,#86517) ;
#71661=AXIS2_PLACEMENT_3D('',#112874,#86518,#86519) ;
#71662=AXIS2_PLACEMENT_3D('',#112875,#86520,#86521) ;
#71663=AXIS2_PLACEMENT_3D('',#112876,#86522,#86523) ;
#71664=AXIS2_PLACEMENT_3D('',#112877,#86524,#86525) ;
#71665=AXIS2_PLACEMENT_3D('',#112878,#86526,#86527) ;
#71666=AXIS2_PLACEMENT_3D('',#112879,#86528,#86529) ;
#71667=AXIS2_PLACEMENT_3D('',#112880,#86530,#86531) ;
#71668=AXIS2_PLACEMENT_3D('',#112881,#86532,#86533) ;
#71669=AXIS2_PLACEMENT_3D('',#112882,#86534,#86535) ;
#71670=AXIS2_PLACEMENT_3D('',#112883,#86536,#86537) ;
#71671=AXIS2_PLACEMENT_3D('',#112884,#86538,#86539) ;
#71672=AXIS2_PLACEMENT_3D('',#112885,#86540,#86541) ;
#71673=AXIS2_PLACEMENT_3D('',#112886,#86542,#86543) ;
#71674=AXIS2_PLACEMENT_3D('',#112893,#86544,#86545) ;
#71675=AXIS2_PLACEMENT_3D('',#112894,#86546,#86547) ;
#71676=AXIS2_PLACEMENT_3D('',#112895,#86548,#86549) ;
#71677=AXIS2_PLACEMENT_3D('',#112896,#86550,#86551) ;
#71678=AXIS2_PLACEMENT_3D('',#112897,#86552,#86553) ;
#71679=AXIS2_PLACEMENT_3D('',#112898,#86554,#86555) ;
#71680=AXIS2_PLACEMENT_3D('',#112899,#86556,#86557) ;
#71681=AXIS2_PLACEMENT_3D('',#112900,#86558,#86559) ;
#71682=AXIS2_PLACEMENT_3D('',#112901,#86560,#86561) ;
#71683=AXIS2_PLACEMENT_3D('',#112902,#86562,#86563) ;
#71684=AXIS2_PLACEMENT_3D('',#112903,#86564,#86565) ;
#71685=AXIS2_PLACEMENT_3D('',#112904,#86566,#86567) ;
#71686=AXIS2_PLACEMENT_3D('',#112905,#86568,#86569) ;
#71687=AXIS2_PLACEMENT_3D('',#112906,#86570,#86571) ;
#71688=AXIS2_PLACEMENT_3D('',#112907,#86572,#86573) ;
#71689=AXIS2_PLACEMENT_3D('',#112908,#86574,#86575) ;
#71690=AXIS2_PLACEMENT_3D('',#112909,#86576,#86577) ;
#71691=AXIS2_PLACEMENT_3D('',#112910,#86578,#86579) ;
#71692=AXIS2_PLACEMENT_3D('',#112911,#86580,#86581) ;
#71693=AXIS2_PLACEMENT_3D('',#112912,#86582,#86583) ;
#71694=AXIS2_PLACEMENT_3D('',#112913,#86584,#86585) ;
#71695=AXIS2_PLACEMENT_3D('',#112914,#86586,#86587) ;
#71696=AXIS2_PLACEMENT_3D('',#112915,#86588,#86589) ;
#71697=AXIS2_PLACEMENT_3D('',#112916,#86590,#86591) ;
#71698=AXIS2_PLACEMENT_3D('',#112917,#86592,#86593) ;
#71699=AXIS2_PLACEMENT_3D('',#112918,#86594,#86595) ;
#71700=AXIS2_PLACEMENT_3D('',#112919,#86596,#86597) ;
#71701=AXIS2_PLACEMENT_3D('',#112920,#86598,#86599) ;
#71702=AXIS2_PLACEMENT_3D('',#112921,#86600,#86601) ;
#71703=AXIS2_PLACEMENT_3D('',#112922,#86602,#86603) ;
#71704=AXIS2_PLACEMENT_3D('',#112923,#86604,#86605) ;
#71705=AXIS2_PLACEMENT_3D('',#112924,#86606,#86607) ;
#71706=AXIS2_PLACEMENT_3D('',#112925,#86608,#86609) ;
#71707=AXIS2_PLACEMENT_3D('',#112926,#86610,#86611) ;
#71708=AXIS2_PLACEMENT_3D('',#112927,#86612,#86613) ;
#71709=AXIS2_PLACEMENT_3D('',#112928,#86614,#86615) ;
#71710=AXIS2_PLACEMENT_3D('',#112929,#86616,#86617) ;
#71711=AXIS2_PLACEMENT_3D('',#112930,#86618,#86619) ;
#71712=AXIS2_PLACEMENT_3D('',#112931,#86620,#86621) ;
#71713=AXIS2_PLACEMENT_3D('',#112962,#86622,#86623) ;
#71714=AXIS2_PLACEMENT_3D('',#112963,#86624,#86625) ;
#71715=AXIS2_PLACEMENT_3D('',#112964,#86626,#86627) ;
#71716=AXIS2_PLACEMENT_3D('',#112965,#86628,#86629) ;
#71717=AXIS2_PLACEMENT_3D('',#112966,#86630,#86631) ;
#71718=AXIS2_PLACEMENT_3D('',#112967,#86632,#86633) ;
#71719=AXIS2_PLACEMENT_3D('',#112968,#86634,#86635) ;
#71720=AXIS2_PLACEMENT_3D('',#112969,#86636,#86637) ;
#71721=AXIS2_PLACEMENT_3D('',#112970,#86638,#86639) ;
#71722=AXIS2_PLACEMENT_3D('',#112971,#86640,#86641) ;
#71723=AXIS2_PLACEMENT_3D('',#112998,#86642,#86643) ;
#71724=AXIS2_PLACEMENT_3D('',#112999,#86644,#86645) ;
#71725=AXIS2_PLACEMENT_3D('',#113000,#86646,#86647) ;
#71726=AXIS2_PLACEMENT_3D('',#113001,#86648,#86649) ;
#71727=AXIS2_PLACEMENT_3D('',#113002,#86650,#86651) ;
#71728=AXIS2_PLACEMENT_3D('',#113003,#86652,#86653) ;
#71729=AXIS2_PLACEMENT_3D('',#113004,#86654,#86655) ;
#71730=AXIS2_PLACEMENT_3D('',#113005,#86656,#86657) ;
#71731=AXIS2_PLACEMENT_3D('',#113006,#86658,#86659) ;
#71732=AXIS2_PLACEMENT_3D('',#113007,#86660,#86661) ;
#71733=AXIS2_PLACEMENT_3D('',#113008,#86662,#86663) ;
#71734=AXIS2_PLACEMENT_3D('',#113009,#86664,#86665) ;
#71735=AXIS2_PLACEMENT_3D('',#113010,#86666,#86667) ;
#71736=AXIS2_PLACEMENT_3D('',#113011,#86668,#86669) ;
#71737=AXIS2_PLACEMENT_3D('',#113012,#86670,#86671) ;
#71738=AXIS2_PLACEMENT_3D('',#113013,#86672,#86673) ;
#71739=AXIS2_PLACEMENT_3D('',#113014,#86674,#86675) ;
#71740=AXIS2_PLACEMENT_3D('',#113015,#86676,#86677) ;
#71741=AXIS2_PLACEMENT_3D('',#113016,#86678,#86679) ;
#71742=AXIS2_PLACEMENT_3D('',#113017,#86680,#86681) ;
#71743=AXIS2_PLACEMENT_3D('',#113018,#86682,#86683) ;
#71744=AXIS2_PLACEMENT_3D('',#113019,#86684,#86685) ;
#71745=AXIS2_PLACEMENT_3D('',#113020,#86686,#86687) ;
#71746=AXIS2_PLACEMENT_3D('',#113021,#86688,#86689) ;
#71747=AXIS2_PLACEMENT_3D('',#113022,#86690,#86691) ;
#71748=AXIS2_PLACEMENT_3D('',#113023,#86692,#86693) ;
#71749=AXIS2_PLACEMENT_3D('',#113024,#86694,#86695) ;
#71750=AXIS2_PLACEMENT_3D('',#113025,#86696,#86697) ;
#71751=AXIS2_PLACEMENT_3D('',#113026,#86698,#86699) ;
#71752=AXIS2_PLACEMENT_3D('',#113051,#86700,#86701) ;
#71753=AXIS2_PLACEMENT_3D('',#113052,#86702,#86703) ;
#71754=AXIS2_PLACEMENT_3D('',#113053,#86704,#86705) ;
#71755=AXIS2_PLACEMENT_3D('',#113054,#86706,#86707) ;
#71756=AXIS2_PLACEMENT_3D('',#113055,#86708,#86709) ;
#71757=AXIS2_PLACEMENT_3D('',#113056,#86710,#86711) ;
#71758=AXIS2_PLACEMENT_3D('',#113057,#86712,#86713) ;
#71759=AXIS2_PLACEMENT_3D('',#113106,#86714,#86715) ;
#71760=AXIS2_PLACEMENT_3D('',#113107,#86716,#86717) ;
#71761=AXIS2_PLACEMENT_3D('',#113108,#86718,#86719) ;
#71762=AXIS2_PLACEMENT_3D('',#113109,#86720,#86721) ;
#71763=AXIS2_PLACEMENT_3D('',#113110,#86722,#86723) ;
#71764=AXIS2_PLACEMENT_3D('',#113111,#86724,#86725) ;
#71765=AXIS2_PLACEMENT_3D('',#113112,#86726,#86727) ;
#71766=AXIS2_PLACEMENT_3D('',#113174,#86728,#86729) ;
#71767=AXIS2_PLACEMENT_3D('',#113175,#86730,#86731) ;
#71768=AXIS2_PLACEMENT_3D('',#113176,#86732,#86733) ;
#71769=AXIS2_PLACEMENT_3D('',#113349,#86734,#86735) ;
#71770=AXIS2_PLACEMENT_3D('',#113350,#86736,#86737) ;
#71771=AXIS2_PLACEMENT_3D('',#113405,#86738,#86739) ;
#71772=AXIS2_PLACEMENT_3D('',#113452,#86740,#86741) ;
#71773=AXIS2_PLACEMENT_3D('',#113453,#86742,#86743) ;
#71774=AXIS2_PLACEMENT_3D('',#113454,#86744,#86745) ;
#71775=AXIS2_PLACEMENT_3D('',#113455,#86746,#86747) ;
#71776=AXIS2_PLACEMENT_3D('',#113456,#86748,#86749) ;
#71777=AXIS2_PLACEMENT_3D('',#113457,#86750,#86751) ;
#71778=AXIS2_PLACEMENT_3D('',#113562,#86752,#86753) ;
#71779=AXIS2_PLACEMENT_3D('',#113563,#86754,#86755) ;
#71780=AXIS2_PLACEMENT_3D('',#113564,#86756,#86757) ;
#71781=AXIS2_PLACEMENT_3D('',#113565,#86758,#86759) ;
#71782=AXIS2_PLACEMENT_3D('',#113578,#86760,#86761) ;
#71783=AXIS2_PLACEMENT_3D('',#113579,#86762,#86763) ;
#71784=AXIS2_PLACEMENT_3D('',#113580,#86764,#86765) ;
#71785=AXIS2_PLACEMENT_3D('',#113581,#86766,#86767) ;
#71786=AXIS2_PLACEMENT_3D('',#113582,#86768,#86769) ;
#71787=AXIS2_PLACEMENT_3D('',#113583,#86770,#86771) ;
#71788=AXIS2_PLACEMENT_3D('',#113584,#86772,#86773) ;
#71789=AXIS2_PLACEMENT_3D('',#113585,#86774,#86775) ;
#71790=AXIS2_PLACEMENT_3D('',#113586,#86776,#86777) ;
#71791=AXIS2_PLACEMENT_3D('',#113587,#86778,#86779) ;
#71792=AXIS2_PLACEMENT_3D('',#113588,#86780,#86781) ;
#71793=AXIS2_PLACEMENT_3D('',#113589,#86782,#86783) ;
#71794=AXIS2_PLACEMENT_3D('',#113590,#86784,#86785) ;
#71795=AXIS2_PLACEMENT_3D('',#113591,#86786,#86787) ;
#71796=AXIS2_PLACEMENT_3D('',#113592,#86788,#86789) ;
#71797=AXIS2_PLACEMENT_3D('',#113593,#86790,#86791) ;
#71798=AXIS2_PLACEMENT_3D('',#113594,#86792,#86793) ;
#71799=AXIS2_PLACEMENT_3D('',#113595,#86794,#86795) ;
#71800=AXIS2_PLACEMENT_3D('',#113596,#86796,#86797) ;
#71801=AXIS2_PLACEMENT_3D('',#113597,#86798,#86799) ;
#71802=AXIS2_PLACEMENT_3D('',#113598,#86800,#86801) ;
#71803=AXIS2_PLACEMENT_3D('',#113599,#86802,#86803) ;
#71804=AXIS2_PLACEMENT_3D('',#113600,#86804,#86805) ;
#71805=AXIS2_PLACEMENT_3D('',#113601,#86806,#86807) ;
#71806=AXIS2_PLACEMENT_3D('',#113602,#86808,#86809) ;
#71807=AXIS2_PLACEMENT_3D('',#113603,#86810,#86811) ;
#71808=AXIS2_PLACEMENT_3D('',#113604,#86812,#86813) ;
#71809=AXIS2_PLACEMENT_3D('',#113605,#86814,#86815) ;
#71810=AXIS2_PLACEMENT_3D('',#113606,#86816,#86817) ;
#71811=AXIS2_PLACEMENT_3D('',#113607,#86818,#86819) ;
#71812=AXIS2_PLACEMENT_3D('',#113608,#86820,#86821) ;
#71813=AXIS2_PLACEMENT_3D('',#113609,#86822,#86823) ;
#71814=AXIS2_PLACEMENT_3D('',#113610,#86824,#86825) ;
#71815=AXIS2_PLACEMENT_3D('',#113611,#86826,#86827) ;
#71816=AXIS2_PLACEMENT_3D('',#113612,#86828,#86829) ;
#71817=AXIS2_PLACEMENT_3D('',#113613,#86830,#86831) ;
#71818=AXIS2_PLACEMENT_3D('',#113614,#86832,#86833) ;
#71819=AXIS2_PLACEMENT_3D('',#113615,#86834,#86835) ;
#71820=AXIS2_PLACEMENT_3D('',#113628,#86836,#86837) ;
#71821=AXIS2_PLACEMENT_3D('',#113629,#86838,#86839) ;
#71822=AXIS2_PLACEMENT_3D('',#113630,#86840,#86841) ;
#71823=AXIS2_PLACEMENT_3D('',#113631,#86842,#86843) ;
#71824=AXIS2_PLACEMENT_3D('',#113686,#86844,#86845) ;
#71825=AXIS2_PLACEMENT_3D('',#113687,#86846,#86847) ;
#71826=AXIS2_PLACEMENT_3D('',#113688,#86848,#86849) ;
#71827=AXIS2_PLACEMENT_3D('',#113743,#86850,#86851) ;
#71828=AXIS2_PLACEMENT_3D('',#113744,#86852,#86853) ;
#79337=DIRECTION('axis',(0.,0.,1.)) ;
#79338=DIRECTION('refdir',(1.,0.,0.)) ;
#79339=DIRECTION('center_axis',(0.967224433265373,0.251696850907845,0.0335498276829)) ;
#79340=DIRECTION('ref_axis',(0.148186156389733,-0.666803895723232,0.730351578147647)) ;
#79341=DIRECTION('center_axis',(0.,0.707106781186549,-0.707106781186547)) ;
#79342=DIRECTION('ref_axis',(0.,0.707106781186546,0.707106781186549)) ;
#79343=DIRECTION('center_axis',(0.978007532938554,-0.147978541149823,-0.146981688909242)) ;
#79344=DIRECTION('ref_axis',(0.193734423938406,0.383507624685863,0.902988856403589)) ;
#79345=DIRECTION('center_axis',(0.,0.447213595499958,0.894427190999916)) ;
#79346=DIRECTION('ref_axis',(0.,-0.894427190999916,0.447213595499958)) ;
#79347=DIRECTION('center_axis',(0.960001452008132,0.250435160947733,-0.125217579849484)) ;
#79348=DIRECTION('ref_axis',(0.276742394167923,-0.916645079799563,0.288401534235619)) ;
#79349=DIRECTION('center_axis',(0.,1.,0.)) ;
#79350=DIRECTION('ref_axis',(0.,0.,1.)) ;
#79351=DIRECTION('center_axis',(-1.,0.,0.)) ;
#79352=DIRECTION('ref_axis',(0.,0.413905171642071,-0.910320003563553)) ;
#79353=DIRECTION('center_axis',(1.,1.44560289664734E-16,0.)) ;
#79354=DIRECTION('ref_axis',(0.,1.,0.)) ;
#79355=DIRECTION('center_axis',(1.,1.44560289664734E-16,0.)) ;
#79356=DIRECTION('ref_axis',(-1.44560289664734E-16,1.,0.)) ;
#79357=DIRECTION('center_axis',(-1.77035296021731E-32,1.22464679914735E-16,
-1.)) ;
#79358=DIRECTION('ref_axis',(0.,-1.,-1.22464679914735E-16)) ;
#79359=DIRECTION('center_axis',(-1.,-1.44560289664734E-16,0.)) ;
#79360=DIRECTION('ref_axis',(-1.44560289664734E-16,1.,0.)) ;
#79361=DIRECTION('center_axis',(1.,-3.46944695195361E-16,0.)) ;
#79362=DIRECTION('ref_axis',(2.61228946970625E-16,1.,0.)) ;
#79363=DIRECTION('center_axis',(1.,-3.46944695195361E-16,0.)) ;
#79364=DIRECTION('ref_axis',(3.46944695195361E-16,1.,0.)) ;
#79365=DIRECTION('center_axis',(-4.24884710452153E-32,-1.22464679914735E-16,
1.)) ;
#79366=DIRECTION('ref_axis',(-3.26536183713281E-16,-1.,-1.22464679914735E-16)) ;
#79367=DIRECTION('center_axis',(-1.,3.46944695195361E-16,0.)) ;
#79368=DIRECTION('ref_axis',(3.46944695195361E-16,1.,0.)) ;
#79369=DIRECTION('center_axis',(-1.,3.46944695195361E-16,0.)) ;
#79370=DIRECTION('ref_axis',(-3.46944695195361E-16,-1.,0.)) ;
#79371=DIRECTION('center_axis',(-1.,0.,0.)) ;
#79372=DIRECTION('ref_axis',(0.,0.,1.)) ;
#79373=DIRECTION('',(1.,-3.46944695195361E-16,0.)) ;
#79374=DIRECTION('center_axis',(-1.,8.01625584951926E-16,-1.08420217248551E-15)) ;
#79375=DIRECTION('ref_axis',(1.08420217248551E-15,-1.92678538844662E-45,
-1.)) ;
#79376=DIRECTION('center_axis',(-1.,8.01625584951926E-16,-1.08420217248551E-15)) ;
#79377=DIRECTION('ref_axis',(1.08420217248551E-15,-1.92678538844662E-45,
-1.)) ;
#79378=DIRECTION('',(-1.,3.46944695195361E-16,0.)) ;
#79379=DIRECTION('center_axis',(-1.,3.46944695195361E-16,0.)) ;
#79380=DIRECTION('ref_axis',(-3.46944695195361E-16,-1.,0.)) ;
#79381=DIRECTION('center_axis',(-1.,0.,0.)) ;
#79382=DIRECTION('ref_axis',(0.,0.,1.)) ;
#79383=DIRECTION('',(1.,-3.46944695195361E-16,0.)) ;
#79384=DIRECTION('center_axis',(-1.,2.2680138501079E-15,0.)) ;
#79385=DIRECTION('ref_axis',(2.2680138501079E-15,1.,0.)) ;
#79386=DIRECTION('',(-1.,3.46944695195361E-16,0.)) ;
#79387=DIRECTION('center_axis',(-1.,3.18032637262401E-16,0.)) ;
#79388=DIRECTION('ref_axis',(-5.55111512312578E-16,-1.,0.)) ;
#79389=DIRECTION('center_axis',(1.,-3.18032637262401E-16,0.)) ;
#79390=DIRECTION('ref_axis',(-3.18032637262401E-16,-1.,0.)) ;
#79391=DIRECTION('center_axis',(-2.01298417874256E-16,-0.632948931301568,
-0.774193548387096)) ;
#79392=DIRECTION('ref_axis',(1.73472347597681E-14,-0.774193548387096,0.632948931301568)) ;
#79393=DIRECTION('center_axis',(-1.,3.18032637262401E-16,0.)) ;
#79394=DIRECTION('ref_axis',(-3.18032637262401E-16,-1.,0.)) ;
#79395=DIRECTION('center_axis',(-2.01298417874256E-16,-0.632948931301568,
0.774193548387096)) ;
#79396=DIRECTION('ref_axis',(9.63584817660562E-32,-0.774193548387096,-0.632948931301568)) ;
#79397=DIRECTION('center_axis',(1.,1.44560289664734E-16,0.)) ;
#79398=DIRECTION('ref_axis',(-1.44560289664734E-16,1.,0.)) ;
#79399=DIRECTION('',(-1.,-1.44560289664734E-16,0.)) ;
#79400=DIRECTION('center_axis',(-1.,3.46944695195361E-16,0.)) ;
#79401=DIRECTION('ref_axis',(-3.46944695195361E-16,-1.,0.)) ;
#79402=DIRECTION('',(-1.,3.46944695195361E-16,0.)) ;
#79403=DIRECTION('center_axis',(-1.,3.46944695195361E-16,0.)) ;
#79404=DIRECTION('ref_axis',(3.46944695195361E-16,1.,3.5527136788005E-15)) ;
#79405=DIRECTION('center_axis',(-1.,3.46944695195361E-16,0.)) ;
#79406=DIRECTION('ref_axis',(3.46944695195361E-16,1.,0.)) ;
#79407=DIRECTION('center_axis',(-1.,3.46944695195361E-16,0.)) ;
#79408=DIRECTION('ref_axis',(-3.46944695195361E-16,-1.,0.)) ;
#79409=DIRECTION('',(1.,-3.46944695195361E-16,0.)) ;
#79410=DIRECTION('center_axis',(-1.,-1.44560289664734E-16,-2.65552944032596E-32)) ;
#79411=DIRECTION('ref_axis',(1.44560289664734E-16,-1.,-2.80018320648271E-64)) ;
#79412=DIRECTION('',(2.65552944032596E-32,3.29043518662928E-48,-1.)) ;
#79413=DIRECTION('',(1.44560289664734E-16,-1.,-2.4093381610789E-16)) ;
#79414=DIRECTION('',(0.,0.,1.)) ;
#79415=DIRECTION('center_axis',(0.999999956301289,0.000282786981229719,
8.61913163152323E-5)) ;
#79416=DIRECTION('ref_axis',(0.000288266391063448,-0.997396273403499,-0.0721151211834231)) ;
#79417=DIRECTION('',(-1.44560289664734E-16,1.,-7.2280144832367E-17)) ;
#79418=DIRECTION('center_axis',(0.316227766016838,0.948683298050514,0.)) ;
#79419=DIRECTION('ref_axis',(-0.948683298050514,0.316227766016838,0.)) ;
#79420=DIRECTION('',(-0.948683298050514,0.316227766016838,0.)) ;
#79421=DIRECTION('',(0.,0.,1.)) ;
#79422=DIRECTION('',(0.937042571331636,-0.312347523777212,-0.156173761888606)) ;
#79423=DIRECTION('',(0.,0.,-1.)) ;
#79424=DIRECTION('center_axis',(1.,1.73472347597681E-15,0.)) ;
#79425=DIRECTION('ref_axis',(-1.73472347597681E-15,1.,0.)) ;
#79426=DIRECTION('',(-1.73472347597681E-15,1.,0.)) ;
#79427=DIRECTION('',(0.,0.,1.)) ;
#79428=DIRECTION('',(1.73472347597681E-15,-1.,-2.89120579329468E-16)) ;
#79429=DIRECTION('',(0.,0.,-1.)) ;
#79430=DIRECTION('center_axis',(0.164398987305357,-0.986393923832144,0.)) ;
#79431=DIRECTION('ref_axis',(0.986393923832144,0.164398987305357,0.)) ;
#79432=DIRECTION('',(-0.973328526784575,-0.162221421130762,0.162221421130763)) ;
#79433=DIRECTION('',(0.,0.,-1.)) ;
#79434=DIRECTION('',(0.986393923832144,0.164398987305357,0.)) ;
#79435=DIRECTION('',(0.,0.,1.)) ;
#79436=DIRECTION('center_axis',(-9.91270557701033E-17,1.,0.)) ;
#79437=DIRECTION('ref_axis',(-1.,-9.91270557701033E-17,0.)) ;
#79438=DIRECTION('',(1.,9.91270557701033E-17,0.)) ;
#79439=DIRECTION('',(0.,0.,-1.)) ;
#79440=DIRECTION('',(-1.,-9.91270557701033E-17,0.)) ;
#79441=DIRECTION('',(0.,0.,1.)) ;
#79442=DIRECTION('center_axis',(-9.91270557701033E-17,1.,0.)) ;
#79443=DIRECTION('ref_axis',(-1.,-9.91270557701033E-17,0.)) ;
#79444=DIRECTION('',(-1.,-9.91270557701033E-17,0.)) ;
#79445=DIRECTION('',(0.,0.,-1.)) ;
#79446=DIRECTION('',(-1.,-9.91270557701033E-17,0.)) ;
#79447=DIRECTION('',(0.,0.,1.)) ;
#79448=DIRECTION('center_axis',(1.,1.15648231731787E-15,0.)) ;
#79449=DIRECTION('ref_axis',(-1.15648231731787E-15,1.,0.)) ;
#79450=DIRECTION('',(-1.15648231731787E-15,1.,0.)) ;
#79451=DIRECTION('',(0.,0.,-1.)) ;
#79452=DIRECTION('',(-1.15648231731787E-15,1.,0.)) ;
#79453=DIRECTION('',(0.,0.,1.)) ;
#79454=DIRECTION('center_axis',(-1.,-1.15648231731787E-15,0.)) ;
#79455=DIRECTION('ref_axis',(-1.15648231731787E-15,1.,1.77635683940025E-15)) ;
#79456=DIRECTION('',(0.,0.,1.)) ;
#79457=DIRECTION('center_axis',(0.,0.,1.)) ;
#79458=DIRECTION('ref_axis',(1.,0.,0.)) ;
#79459=DIRECTION('',(-1.,0.,0.)) ;
#79460=DIRECTION('center_axis',(0.,0.,-1.)) ;
#79461=DIRECTION('ref_axis',(1.,0.,0.)) ;
#79462=DIRECTION('center_axis',(0.,0.,-1.)) ;
#79463=DIRECTION('ref_axis',(1.,0.,0.)) ;
#79464=DIRECTION('center_axis',(0.,0.,-1.)) ;
#79465=DIRECTION('ref_axis',(1.,0.,0.)) ;
#79466=DIRECTION('center_axis',(0.,0.,-1.)) ;
#79467=DIRECTION('ref_axis',(1.,0.,0.)) ;
#79468=DIRECTION('',(1.,0.,0.)) ;
#79469=DIRECTION('center_axis',(0.,0.,1.)) ;
#79470=DIRECTION('ref_axis',(1.,0.,0.)) ;
#79471=DIRECTION('',(3.46944695195361E-16,1.,0.)) ;
#79472=DIRECTION('center_axis',(0.,0.,1.)) ;
#79473=DIRECTION('ref_axis',(1.,0.,0.)) ;
#79474=DIRECTION('',(1.,-3.46944695195361E-16,0.)) ;
#79475=DIRECTION('center_axis',(0.,0.,-1.)) ;
#79476=DIRECTION('ref_axis',(1.,0.,0.)) ;
#79477=DIRECTION('',(2.71050543121376E-16,1.,0.)) ;
#79478=DIRECTION('center_axis',(0.,0.,-1.)) ;
#79479=DIRECTION('ref_axis',(1.,0.,0.)) ;
#79480=DIRECTION('',(-1.,3.46944695195361E-16,0.)) ;
#79481=DIRECTION('center_axis',(0.,0.,1.)) ;
#79482=DIRECTION('ref_axis',(1.,0.,0.)) ;
#79483=DIRECTION('',(3.46944695195361E-16,1.,0.)) ;
#79484=DIRECTION('center_axis',(0.,0.,1.)) ;
#79485=DIRECTION('ref_axis',(1.,0.,0.)) ;
#79486=DIRECTION('center_axis',(0.,0.,-1.)) ;
#79487=DIRECTION('ref_axis',(1.,0.,0.)) ;
#79488=DIRECTION('',(0.986393923832144,-0.164398987305354,0.)) ;
#79489=DIRECTION('center_axis',(0.,0.,-1.)) ;
#79490=DIRECTION('ref_axis',(1.,-6.50521303491307E-15,0.)) ;
#79491=DIRECTION('center_axis',(0.,0.,-1.)) ;
#79492=DIRECTION('ref_axis',(1.,0.,0.)) ;
#79493=DIRECTION('',(1.,0.,0.)) ;
#79494=DIRECTION('',(1.13380619344889E-16,-1.,0.)) ;
#79495=DIRECTION('center_axis',(0.,0.,-1.)) ;
#79496=DIRECTION('ref_axis',(1.,0.,0.)) ;
#79497=DIRECTION('',(-1.,-1.92747052886312E-16,0.)) ;
#79498=DIRECTION('center_axis',(0.,0.,1.)) ;
#79499=DIRECTION('ref_axis',(1.,0.,0.)) ;
#79500=DIRECTION('',(0.,-1.,0.)) ;
#79501=DIRECTION('center_axis',(0.,0.,-1.)) ;
#79502=DIRECTION('ref_axis',(1.,0.,0.)) ;
#79503=DIRECTION('center_axis',(0.,0.,1.)) ;
#79504=DIRECTION('ref_axis',(1.,0.,0.)) ;
#79505=DIRECTION('',(-0.948683298050514,0.316227766016838,0.)) ;
#79506=DIRECTION('center_axis',(0.,0.,1.)) ;
#79507=DIRECTION('ref_axis',(1.,0.,0.)) ;
#79508=DIRECTION('',(-1.,0.,0.)) ;
#79509=DIRECTION('center_axis',(0.,0.,1.)) ;
#79510=DIRECTION('ref_axis',(1.,0.,0.)) ;
#79511=DIRECTION('',(0.,-1.,0.)) ;
#79512=DIRECTION('center_axis',(0.,0.,-1.)) ;
#79513=DIRECTION('ref_axis',(1.,0.,0.)) ;
#79514=DIRECTION('',(-1.,-1.92747052886312E-16,0.)) ;
#79515=DIRECTION('center_axis',(0.,0.,1.)) ;
#79516=DIRECTION('ref_axis',(1.,0.,0.)) ;
#79517=DIRECTION('',(1.13380619344889E-16,-1.,0.)) ;
#79518=DIRECTION('',(1.,0.,0.)) ;
#79519=DIRECTION('center_axis',(0.,0.,1.)) ;
#79520=DIRECTION('ref_axis',(1.,0.,0.)) ;
#79521=DIRECTION('center_axis',(0.,0.,1.)) ;
#79522=DIRECTION('ref_axis',(1.,0.,0.)) ;
#79523=DIRECTION('',(-0.986393923832144,0.164398987305354,0.)) ;
#79524=DIRECTION('center_axis',(0.,0.,1.)) ;
#79525=DIRECTION('ref_axis',(1.,0.,0.)) ;
#79526=DIRECTION('center_axis',(0.,0.,-1.)) ;
#79527=DIRECTION('ref_axis',(1.,0.,0.)) ;
#79528=DIRECTION('',(-3.46944695195361E-16,-1.,0.)) ;
#79529=DIRECTION('center_axis',(0.,0.,-1.)) ;
#79530=DIRECTION('ref_axis',(1.,0.,0.)) ;
#79531=DIRECTION('',(-1.,3.46944695195361E-16,0.)) ;
#79532=DIRECTION('center_axis',(0.,0.,1.)) ;
#79533=DIRECTION('ref_axis',(1.,0.,0.)) ;
#79534=DIRECTION('',(3.46944695195361E-16,1.,0.)) ;
#79535=DIRECTION('center_axis',(0.,0.,1.)) ;
#79536=DIRECTION('ref_axis',(1.,0.,0.)) ;
#79537=DIRECTION('',(1.,-3.46944695195361E-16,0.)) ;
#79538=DIRECTION('center_axis',(0.,0.,-1.)) ;
#79539=DIRECTION('ref_axis',(1.,0.,0.)) ;
#79540=DIRECTION('',(-3.46944695195361E-16,-1.,0.)) ;
#79541=DIRECTION('center_axis',(0.,0.,-1.)) ;
#79542=DIRECTION('ref_axis',(1.,0.,0.)) ;
#79543=DIRECTION('',(1.,0.,0.)) ;
#79544=DIRECTION('center_axis',(0.,0.,1.)) ;
#79545=DIRECTION('ref_axis',(1.,0.,0.)) ;
#79546=DIRECTION('',(0.986393923832144,0.164398987305357,0.)) ;
#79547=DIRECTION('center_axis',(0.,0.,1.)) ;
#79548=DIRECTION('ref_axis',(1.,0.,0.)) ;
#79549=DIRECTION('',(-1.73472347597681E-15,1.,0.)) ;
#79550=DIRECTION('center_axis',(0.,0.,1.)) ;
#79551=DIRECTION('ref_axis',(1.,0.,0.)) ;
#79552=DIRECTION('center_axis',(-1.92747052886312E-16,1.,0.)) ;
#79553=DIRECTION('ref_axis',(-1.,-1.92747052886312E-16,0.)) ;
#79554=DIRECTION('',(0.,0.,1.)) ;
#79555=DIRECTION('',(0.,0.,-1.)) ;
#79556=DIRECTION('center_axis',(-1.,0.,0.)) ;
#79557=DIRECTION('ref_axis',(0.,0.,1.)) ;
#79558=DIRECTION('',(0.,0.,1.)) ;
#79559=DIRECTION('',(0.,0.,-1.)) ;
#79560=DIRECTION('center_axis',(0.,1.,0.)) ;
#79561=DIRECTION('ref_axis',(0.,0.,1.)) ;
#79562=DIRECTION('',(0.,0.,-1.)) ;
#79563=DIRECTION('',(0.,0.,1.)) ;
#79564=DIRECTION('',(0.,0.,-1.)) ;
#79565=DIRECTION('',(0.,0.,-1.)) ;
#79566=DIRECTION('center_axis',(0.316227766016838,0.948683298050514,0.)) ;
#79567=DIRECTION('ref_axis',(-0.948683298050514,0.316227766016838,0.)) ;
#79568=DIRECTION('center_axis',(-0.316227766016857,-0.948683298050507,-2.6817125824357E-14)) ;
#79569=DIRECTION('ref_axis',(0.831595960762403,-0.277198653587473,-0.481257794215271)) ;
#79570=DIRECTION('',(0.,0.,1.)) ;
#79571=DIRECTION('',(0.,0.,-1.)) ;
#79572=DIRECTION('',(-0.937042571331636,0.312347523777212,-0.156173761888606)) ;
#79573=DIRECTION('center_axis',(1.,1.73472347597681E-15,0.)) ;
#79574=DIRECTION('ref_axis',(-1.73472347597681E-15,1.,0.)) ;
#79575=DIRECTION('',(-1.73472347597681E-15,1.,-2.89120579329468E-16)) ;
#79576=DIRECTION('',(0.,0.,1.)) ;
#79577=DIRECTION('',(0.,0.,-1.)) ;
#79578=DIRECTION('center_axis',(0.164398987305357,-0.986393923832144,0.)) ;
#79579=DIRECTION('ref_axis',(0.986393923832144,0.164398987305357,0.)) ;
#79580=DIRECTION('',(0.973328526784575,0.162221421130762,0.162221421130763)) ;
#79581=DIRECTION('',(0.,0.,1.)) ;
#79582=DIRECTION('',(0.,0.,-1.)) ;
#79583=DIRECTION('center_axis',(0.,-1.,0.)) ;
#79584=DIRECTION('ref_axis',(0.,0.,-1.)) ;
#79585=DIRECTION('',(0.,0.,1.)) ;
#79586=DIRECTION('',(0.,0.,1.)) ;
#79587=DIRECTION('',(0.,0.,1.)) ;
#79588=DIRECTION('',(0.,0.,-1.)) ;
#79589=DIRECTION('',(1.,0.,2.25271179641597E-31)) ;
#79590=DIRECTION('center_axis',(0.,-1.,0.)) ;
#79591=DIRECTION('ref_axis',(0.,0.,-1.)) ;
#79592=DIRECTION('',(0.,0.,-1.)) ;
#79593=DIRECTION('center_axis',(0.,-1.,0.)) ;
#79594=DIRECTION('ref_axis',(0.,0.,-1.)) ;
#79595=DIRECTION('',(-1.,0.,-3.21815970916568E-32)) ;
#79596=DIRECTION('',(0.,0.,-1.)) ;
#79597=DIRECTION('center_axis',(1.,-3.46944695195361E-16,0.)) ;
#79598=DIRECTION('ref_axis',(3.46944695195361E-16,1.,0.)) ;
#79599=DIRECTION('center_axis',(1.,-3.46944695195361E-16,0.)) ;
#79600=DIRECTION('ref_axis',(3.46944695195361E-16,1.,0.)) ;
#79601=DIRECTION('',(1.5529910948782E-31,4.47619207437002E-16,-1.)) ;
#79602=DIRECTION('',(0.,0.,1.)) ;
#79603=DIRECTION('center_axis',(1.,-3.46944695195361E-16,0.)) ;
#79604=DIRECTION('ref_axis',(3.46944695195361E-16,1.,0.)) ;
#79605=DIRECTION('center_axis',(1.,-3.46944695195361E-16,0.)) ;
#79606=DIRECTION('ref_axis',(3.46944695195361E-16,1.,0.)) ;
#79607=DIRECTION('center_axis',(1.,-3.46944695195361E-16,0.)) ;
#79608=DIRECTION('ref_axis',(3.46944695195361E-16,1.,0.)) ;
#79609=DIRECTION('',(3.46944695195361E-16,1.,9.27571383489107E-17)) ;
#79610=DIRECTION('',(0.,0.,1.)) ;
#79611=DIRECTION('',(-3.46944695195361E-16,-1.,-6.49299968442375E-16)) ;
#79612=DIRECTION('center_axis',(1.,-3.46944695195361E-16,0.)) ;
#79613=DIRECTION('ref_axis',(3.46944695195361E-16,1.,0.)) ;
#79614=DIRECTION('center_axis',(1.,-3.46944695195361E-16,0.)) ;
#79615=DIRECTION('ref_axis',(3.46944695195361E-16,1.,0.)) ;
#79616=DIRECTION('center_axis',(1.,-3.46944695195361E-16,0.)) ;
#79617=DIRECTION('ref_axis',(3.46944695195361E-16,1.,0.)) ;
#79618=DIRECTION('',(0.,0.,1.)) ;
#79619=DIRECTION('',(-1.5529910948782E-31,-4.47619207437002E-16,-1.)) ;
#79620=DIRECTION('center_axis',(1.,-3.46944695195361E-16,0.)) ;
#79621=DIRECTION('ref_axis',(3.46944695195361E-16,1.,0.)) ;
#79622=DIRECTION('center_axis',(1.,-3.46944695195361E-16,0.)) ;
#79623=DIRECTION('ref_axis',(3.46944695195361E-16,1.,0.)) ;
#79624=DIRECTION('center_axis',(1.,-3.46944695195361E-16,0.)) ;
#79625=DIRECTION('ref_axis',(3.46944695195361E-16,1.,0.)) ;
#79626=DIRECTION('',(-3.46944695195361E-16,-1.,-1.06487173641454E-15)) ;
#79627=DIRECTION('center_axis',(1.,-3.46944695195361E-16,0.)) ;
#79628=DIRECTION('ref_axis',(3.46944695195361E-16,1.,0.)) ;
#79629=DIRECTION('',(3.46944695195361E-16,1.,2.45739631480277E-16)) ;
#79630=DIRECTION('center_axis',(1.,-3.46944695195361E-16,0.)) ;
#79631=DIRECTION('ref_axis',(3.46944695195361E-16,1.,0.)) ;
#79632=DIRECTION('center_axis',(1.,-3.46944695195361E-16,0.)) ;
#79633=DIRECTION('ref_axis',(3.46944695195361E-16,1.,0.)) ;
#79634=DIRECTION('center_axis',(0.,-1.,0.)) ;
#79635=DIRECTION('ref_axis',(0.,0.,-1.)) ;
#79636=DIRECTION('center_axis',(0.,-1.,0.)) ;
#79637=DIRECTION('ref_axis',(0.,0.,-1.)) ;
#79638=DIRECTION('',(-1.,0.,-1.40488587213121E-32)) ;
#79639=DIRECTION('',(0.,0.,1.)) ;
#79640=DIRECTION('',(0.,0.,1.)) ;
#79641=DIRECTION('',(0.,0.,1.)) ;
#79642=DIRECTION('',(1.,0.,1.40488587213121E-32)) ;
#79643=DIRECTION('center_axis',(0.,-1.,0.)) ;
#79644=DIRECTION('ref_axis',(0.,0.,-1.)) ;
#79645=DIRECTION('',(7.2280144832367E-17,0.,-1.)) ;
#79646=DIRECTION('center_axis',(-1.,-1.13380619344889E-16,0.)) ;
#79647=DIRECTION('ref_axis',(1.13380619344889E-16,-1.,0.)) ;
#79648=DIRECTION('center_axis',(-1.,-1.13380619344889E-16,0.)) ;
#79649=DIRECTION('ref_axis',(1.13380619344889E-16,-1.,0.)) ;
#79650=DIRECTION('',(1.13380619344889E-16,-1.,1.23908819712629E-16)) ;
#79651=DIRECTION('',(0.,0.,-1.)) ;
#79652=DIRECTION('',(-1.13380619344889E-16,1.,-1.23908819712629E-16)) ;
#79653=DIRECTION('center_axis',(-1.,-1.13380619344889E-16,0.)) ;
#79654=DIRECTION('ref_axis',(1.13380619344889E-16,-1.,0.)) ;
#79655=DIRECTION('',(0.,0.,1.)) ;
#79656=DIRECTION('center_axis',(-1.40488587213121E-32,1.23908819712629E-16,
1.)) ;
#79657=DIRECTION('ref_axis',(0.,-1.,1.23908819712629E-16)) ;
#79658=DIRECTION('',(-1.,0.,-1.40488587213121E-32)) ;
#79659=DIRECTION('',(-1.13380619344889E-16,1.,-1.23908819712629E-16)) ;
#79660=DIRECTION('center_axis',(1.40488587213121E-32,-1.23908819712629E-16,
-1.)) ;
#79661=DIRECTION('ref_axis',(-1.74077750246726E-48,-1.,1.23908819712629E-16)) ;
#79662=DIRECTION('center_axis',(1.40488587213121E-32,-1.23908819712629E-16,
-1.)) ;
#79663=DIRECTION('ref_axis',(0.,1.,-1.23908819712629E-16)) ;
#79664=DIRECTION('center_axis',(-1.40488587213121E-32,1.23908819712629E-16,
1.)) ;
#79665=DIRECTION('ref_axis',(1.74077750246726E-48,1.,-1.23908819712629E-16)) ;
#79666=DIRECTION('',(1.13380619344889E-16,-1.,1.23908819712629E-16)) ;
#79667=DIRECTION('',(1.,0.,1.40488587213121E-32)) ;
#79668=DIRECTION('center_axis',(-1.,-1.23908819712629E-16,-8.95614743483648E-33)) ;
#79669=DIRECTION('ref_axis',(1.23908819712629E-16,-1.,5.38566640001825E-66)) ;
#79670=DIRECTION('',(-8.95614743483648E-33,-1.10974565782288E-48,1.)) ;
#79671=DIRECTION('',(1.23908819712629E-16,-1.,7.2280144832367E-17)) ;
#79672=DIRECTION('',(-8.95614743483648E-33,0.,1.)) ;
#79673=DIRECTION('',(-1.23908819712629E-16,1.,-1.23908819712629E-16)) ;
#79674=DIRECTION('',(8.95614743483648E-33,1.0154535431059E-48,-1.)) ;
#79675=DIRECTION('',(1.23908819712629E-16,-1.,1.23908819712629E-16)) ;
#79676=DIRECTION('',(-8.95614743483648E-33,0.,1.)) ;
#79677=DIRECTION('',(-1.23908819712629E-16,1.,2.4093381610789E-16)) ;
#79678=DIRECTION('center_axis',(-1.7912294869673E-32,7.2280144832367E-17,
1.)) ;
#79679=DIRECTION('ref_axis',(0.,-1.,7.2280144832367E-17)) ;
#79680=DIRECTION('',(-1.23908819712629E-16,1.,-7.2280144832367E-17)) ;
#79681=DIRECTION('',(1.,1.23908819712629E-16,8.95614743483648E-33)) ;
#79682=DIRECTION('',(1.44560289664734E-16,-1.,7.2280144832367E-17)) ;
#79683=DIRECTION('',(-1.,0.,-1.7912294869673E-32)) ;
#79684=DIRECTION('center_axis',(-2.08976773479518E-32,2.4093381610789E-16,
-1.)) ;
#79685=DIRECTION('ref_axis',(0.,1.,2.4093381610789E-16)) ;
#79686=DIRECTION('',(-1.44560289664734E-16,1.,2.4093381610789E-16)) ;
#79687=DIRECTION('',(-1.,-1.23908819712629E-16,-8.95614743483648E-33)) ;
#79688=DIRECTION('',(1.23908819712629E-16,-1.,-2.4093381610789E-16)) ;
#79689=DIRECTION('',(1.,0.,-2.08976773479518E-32)) ;
#79690=DIRECTION('center_axis',(-1.23908819712629E-16,1.,0.)) ;
#79691=DIRECTION('ref_axis',(-1.,-1.23908819712629E-16,0.)) ;
#79692=DIRECTION('',(8.95614743483648E-33,1.10974565782288E-48,-1.)) ;
#79693=DIRECTION('',(1.,1.23908819712629E-16,8.95614743483648E-33)) ;
#79694=DIRECTION('',(-2.65552944032596E-32,-3.29043518662928E-48,1.)) ;
#79695=DIRECTION('',(-1.,-1.23908819712629E-16,-8.95614743483648E-33)) ;
#79696=DIRECTION('center_axis',(-1.,-1.44560289664734E-16,-2.65552944032596E-32)) ;
#79697=DIRECTION('ref_axis',(1.44560289664734E-16,-1.,-2.80018320648271E-64)) ;
#79698=DIRECTION('',(1.44560289664734E-16,-1.,-2.4093381610789E-16)) ;
#79699=DIRECTION('',(-2.65552944032596E-32,0.,1.)) ;
#79700=DIRECTION('',(-1.44560289664734E-16,1.,-7.2280144832367E-17)) ;
#79701=DIRECTION('',(0.,0.,-1.)) ;
#79702=DIRECTION('center_axis',(0.,1.,0.)) ;
#79703=DIRECTION('ref_axis',(0.,0.,1.)) ;
#79704=DIRECTION('',(8.95614743483648E-33,0.,-1.)) ;
#79705=DIRECTION('',(1.,0.,1.40488587213121E-32)) ;
#79706=DIRECTION('',(-7.2280144832367E-17,0.,1.)) ;
#79707=DIRECTION('',(-1.,0.,-1.40488587213121E-32)) ;
#79708=DIRECTION('',(8.95614743483648E-33,0.,-1.)) ;
#79709=DIRECTION('',(1.,0.,1.7912294869673E-32)) ;
#79710=DIRECTION('',(2.65552944032596E-32,0.,-1.)) ;
#79711=DIRECTION('',(-1.,0.,2.08976773479518E-32)) ;
#79712=DIRECTION('center_axis',(1.,1.44560289664734E-16,0.)) ;
#79713=DIRECTION('ref_axis',(-1.44560289664734E-16,1.,0.)) ;
#79714=DIRECTION('',(1.44560289664734E-16,-1.,0.)) ;
#79715=DIRECTION('center_axis',(-1.,-1.44560289664734E-16,0.)) ;
#79716=DIRECTION('ref_axis',(-1.44560289664734E-16,1.,-4.33680868994201E-15)) ;
#79717=DIRECTION('',(0.,0.,-1.)) ;
#79718=DIRECTION('center_axis',(-1.,-1.44560289664734E-16,0.)) ;
#79719=DIRECTION('ref_axis',(-1.44560289664734E-16,1.,0.)) ;
#79720=DIRECTION('',(1.44560289664734E-16,-1.,0.)) ;
#79721=DIRECTION('center_axis',(-1.,-1.44560289664734E-16,0.)) ;
#79722=DIRECTION('ref_axis',(-1.44560289664734E-16,1.,0.)) ;
#79723=DIRECTION('',(0.,0.,1.)) ;
#79724=DIRECTION('center_axis',(-1.,-1.44560289664734E-16,0.)) ;
#79725=DIRECTION('ref_axis',(-1.44560289664734E-16,1.,0.)) ;
#79726=DIRECTION('center_axis',(1.,-3.46944695195361E-16,0.)) ;
#79727=DIRECTION('ref_axis',(3.46944695195361E-16,1.,0.)) ;
#79728=DIRECTION('center_axis',(1.,-3.46944695195361E-16,0.)) ;
#79729=DIRECTION('ref_axis',(3.46944695195361E-16,1.,0.)) ;
#79730=DIRECTION('',(0.,0.,-1.)) ;
#79731=DIRECTION('',(-1.5529910948782E-31,-4.47619207437002E-16,1.)) ;
#79732=DIRECTION('center_axis',(-1.,3.46944695195361E-16,0.)) ;
#79733=DIRECTION('ref_axis',(3.46944695195361E-16,1.,-1.77635683940025E-15)) ;
#79734=DIRECTION('',(-3.46944695195361E-16,-1.,-2.45739631480277E-16)) ;
#79735=DIRECTION('center_axis',(1.,-3.46944695195361E-16,0.)) ;
#79736=DIRECTION('ref_axis',(3.46944695195361E-16,1.,0.)) ;
#79737=DIRECTION('center_axis',(3.46944695195361E-16,1.,4.47619207437002E-16)) ;
#79738=DIRECTION('ref_axis',(-8.18685017503995E-48,-4.47619207437002E-16,
1.)) ;
#79739=DIRECTION('',(-1.5529910948782E-31,-4.47619207437002E-16,1.)) ;
#79740=DIRECTION('',(-1.,3.46944695195361E-16,0.)) ;
#79741=DIRECTION('',(1.5529910948782E-31,4.47619207437002E-16,-1.)) ;
#79742=DIRECTION('center_axis',(-8.52580615413453E-32,-2.45739631480277E-16,
1.)) ;
#79743=DIRECTION('ref_axis',(0.,-1.,-2.45739631480277E-16)) ;
#79744=DIRECTION('',(1.,-3.46944695195361E-16,0.)) ;
#79745=DIRECTION('',(-3.46944695195361E-16,-1.,-2.45739631480277E-16)) ;
#79746=DIRECTION('',(3.46944695195361E-16,1.,2.45739631480277E-16)) ;
#79747=DIRECTION('center_axis',(1.,-3.46944695195361E-16,0.)) ;
#79748=DIRECTION('ref_axis',(3.46944695195361E-16,1.,0.)) ;
#79749=DIRECTION('center_axis',(1.,-3.46944695195361E-16,0.)) ;
#79750=DIRECTION('ref_axis',(3.46944695195361E-16,1.,0.)) ;
#79751=DIRECTION('',(1.,-3.46944695195361E-16,0.)) ;
#79752=DIRECTION('center_axis',(-1.,3.46944695195361E-16,0.)) ;
#79753=DIRECTION('ref_axis',(3.46944695195361E-16,1.,0.)) ;
#79754=DIRECTION('',(-1.,3.46944695195361E-16,0.)) ;
#79755=DIRECTION('center_axis',(1.,-3.46944695195361E-16,0.)) ;
#79756=DIRECTION('ref_axis',(3.46944695195361E-16,1.,0.)) ;
#79757=DIRECTION('center_axis',(1.,-3.46944695195361E-16,0.)) ;
#79758=DIRECTION('ref_axis',(-3.46944695195361E-16,-1.,-1.77635683940025E-15)) ;
#79759=DIRECTION('',(1.,-3.46944695195361E-16,0.)) ;
#79760=DIRECTION('center_axis',(-1.,3.46944695195361E-16,0.)) ;
#79761=DIRECTION('ref_axis',(3.46944695195361E-16,1.,-1.77635683940025E-15)) ;
#79762=DIRECTION('',(-1.,3.46944695195361E-16,0.)) ;
#79763=DIRECTION('center_axis',(3.69451600012496E-31,1.06487173641454E-15,
-1.)) ;
#79764=DIRECTION('ref_axis',(0.,1.,1.06487173641454E-15)) ;
#79765=DIRECTION('',(3.46944695195361E-16,1.,1.06487173641454E-15)) ;
#79766=DIRECTION('',(-1.,3.46944695195361E-16,0.)) ;
#79767=DIRECTION('',(-3.46944695195361E-16,-1.,-1.06487173641454E-15)) ;
#79768=DIRECTION('center_axis',(3.46944695195361E-16,1.,-4.47619207437002E-16)) ;
#79769=DIRECTION('ref_axis',(8.18685017503995E-48,4.47619207437002E-16,
1.)) ;
#79770=DIRECTION('',(1.,-3.46944695195361E-16,0.)) ;
#79771=DIRECTION('',(1.5529910948782E-31,4.47619207437002E-16,1.)) ;
#79772=DIRECTION('',(-1.5529910948782E-31,-4.47619207437002E-16,-1.)) ;
#79773=DIRECTION('center_axis',(-1.,3.46944695195361E-16,0.)) ;
#79774=DIRECTION('ref_axis',(-3.46944695195361E-16,-1.,0.)) ;
#79775=DIRECTION('center_axis',(-1.,3.46944695195361E-16,0.)) ;
#79776=DIRECTION('ref_axis',(-3.46944695195361E-16,-1.,0.)) ;
#79777=DIRECTION('',(1.5529910948782E-31,4.47619207437002E-16,1.)) ;
#79778=DIRECTION('',(0.,0.,-1.)) ;
#79779=DIRECTION('center_axis',(1.,-3.46944695195361E-16,0.)) ;
#79780=DIRECTION('ref_axis',(-3.46944695195361E-16,-1.,2.16840434497101E-15)) ;
#79781=DIRECTION('center_axis',(1.,-3.46944695195361E-16,0.)) ;
#79782=DIRECTION('ref_axis',(-3.46944695195361E-16,-1.,-5.32907051820075E-15)) ;
#79783=DIRECTION('',(3.46944695195361E-16,1.,1.06487173641454E-15)) ;
#79784=DIRECTION('center_axis',(1.,-3.46944695195361E-16,0.)) ;
#79785=DIRECTION('ref_axis',(3.46944695195361E-16,1.,0.)) ;
#79786=DIRECTION('center_axis',(-1.,3.46944695195361E-16,0.)) ;
#79787=DIRECTION('ref_axis',(3.46944695195361E-16,1.,0.)) ;
#79788=DIRECTION('',(0.,0.,-1.)) ;
#79789=DIRECTION('',(0.,0.,1.)) ;
#79790=DIRECTION('',(-3.46944695195361E-16,-1.,-9.27571383489107E-17)) ;
#79791=DIRECTION('center_axis',(-3.46944695195361E-16,-1.,0.)) ;
#79792=DIRECTION('ref_axis',(1.,-3.46944695195361E-16,0.)) ;
#79793=DIRECTION('',(1.,-3.46944695195361E-16,0.)) ;
#79794=DIRECTION('',(0.,0.,-1.)) ;
#79795=DIRECTION('',(0.,0.,1.)) ;
#79796=DIRECTION('center_axis',(1.,-3.46944695195361E-16,0.)) ;
#79797=DIRECTION('ref_axis',(3.46944695195361E-16,1.,0.)) ;
#79798=DIRECTION('center_axis',(1.,-3.46944695195361E-16,0.)) ;
#79799=DIRECTION('ref_axis',(3.46944695195361E-16,1.,0.)) ;
#79800=DIRECTION('',(1.,-3.46944695195361E-16,0.)) ;
#79801=DIRECTION('center_axis',(-1.,3.46944695195361E-16,0.)) ;
#79802=DIRECTION('ref_axis',(3.46944695195361E-16,1.,0.)) ;
#79803=DIRECTION('',(-1.,3.46944695195361E-16,0.)) ;
#79804=DIRECTION('center_axis',(-3.21815970916568E-32,-9.27571383489107E-17,
1.)) ;
#79805=DIRECTION('ref_axis',(0.,-1.,-9.27571383489107E-17)) ;
#79806=DIRECTION('',(3.46944695195361E-16,1.,9.27571383489107E-17)) ;
#79807=DIRECTION('',(1.,0.,3.21815970916568E-32)) ;
#79808=DIRECTION('',(-3.46944695195361E-16,-1.,-9.27571383489107E-17)) ;
#79809=DIRECTION('',(-1.,3.46944695195361E-16,0.)) ;
#79810=DIRECTION('center_axis',(1.,-3.46944695195361E-16,0.)) ;
#79811=DIRECTION('ref_axis',(3.46944695195361E-16,1.,0.)) ;
#79812=DIRECTION('center_axis',(1.,-3.46944695195361E-16,0.)) ;
#79813=DIRECTION('ref_axis',(-3.46944695195361E-16,-1.,-2.66453525910038E-15)) ;
#79814=DIRECTION('',(1.,-3.46944695195361E-16,0.)) ;
#79815=DIRECTION('center_axis',(-1.,3.46944695195361E-16,0.)) ;
#79816=DIRECTION('ref_axis',(3.46944695195361E-16,1.,-3.5527136788005E-15)) ;
#79817=DIRECTION('',(-1.,3.46944695195361E-16,0.)) ;
#79818=DIRECTION('center_axis',(-3.46944695195361E-16,-1.,0.)) ;
#79819=DIRECTION('ref_axis',(1.,-3.46944695195361E-16,0.)) ;
#79820=DIRECTION('',(0.,0.,-1.)) ;
#79821=DIRECTION('',(-1.,3.46944695195361E-16,0.)) ;
#79822=DIRECTION('',(0.,0.,1.)) ;
#79823=DIRECTION('center_axis',(2.25271179641597E-31,6.49299968442375E-16,
-1.)) ;
#79824=DIRECTION('ref_axis',(0.,1.,6.49299968442375E-16)) ;
#79825=DIRECTION('',(3.46944695195361E-16,1.,6.49299968442375E-16)) ;
#79826=DIRECTION('',(-1.,0.,-2.25271179641597E-31)) ;
#79827=DIRECTION('',(-3.46944695195361E-16,-1.,-6.49299968442375E-16)) ;
#79828=DIRECTION('',(1.,-3.46944695195361E-16,0.)) ;
#79829=DIRECTION('center_axis',(-1.,3.46944695195361E-16,0.)) ;
#79830=DIRECTION('ref_axis',(-3.46944695195361E-16,-1.,0.)) ;
#79831=DIRECTION('',(3.46944695195361E-16,1.,6.49299968442375E-16)) ;
#79832=DIRECTION('',(0.,0.,1.)) ;
#79833=DIRECTION('',(0.,0.,-1.)) ;
#79834=DIRECTION('center_axis',(-1.,3.46944695195361E-16,0.)) ;
#79835=DIRECTION('ref_axis',(-3.46944695195361E-16,-1.,0.)) ;
#79836=DIRECTION('center_axis',(-0.164398987305357,0.,-0.986393923832144)) ;
#79837=DIRECTION('ref_axis',(-0.986393923832144,0.,0.164398987305357)) ;
#79838=DIRECTION('',(-0.937042571331636,0.312347523777212,0.156173761888606)) ;
#79839=DIRECTION('',(0.,-1.,0.)) ;
#79840=DIRECTION('',(0.973328526784575,0.162221421130762,-0.162221421130763)) ;
#79841=DIRECTION('',(-1.73472347597681E-15,1.,2.89120579329468E-16)) ;
#79842=DIRECTION('center_axis',(-1.,0.,0.)) ;
#79843=DIRECTION('ref_axis',(0.,0.,1.)) ;
#79844=DIRECTION('center_axis',(-1.,0.,0.)) ;
#79845=DIRECTION('ref_axis',(0.,0.958782004973288,-0.284142687640211)) ;
#79846=DIRECTION('',(0.,0.,1.)) ;
#79847=DIRECTION('',(0.,-1.,0.)) ;
#79848=DIRECTION('center_axis',(-1.,0.,0.)) ;
#79849=DIRECTION('ref_axis',(0.,0.758705435142026,-0.651433851350964)) ;
#79850=DIRECTION('',(0.,0.,-1.)) ;
#79851=DIRECTION('center_axis',(-1.,0.,0.)) ;
#79852=DIRECTION('ref_axis',(0.,-0.654778578355217,-0.755820754760757)) ;
#79853=DIRECTION('',(0.,1.,0.)) ;
#79854=DIRECTION('center_axis',(-0.164398987305357,0.,0.986393923832144)) ;
#79855=DIRECTION('ref_axis',(0.986393923832144,0.,0.164398987305357)) ;
#79856=DIRECTION('',(-0.973328526784575,-0.162221421130762,-0.162221421130763)) ;
#79857=DIRECTION('',(0.,1.,0.)) ;
#79858=DIRECTION('',(0.937042571331636,-0.312347523777212,0.156173761888606)) ;
#79859=DIRECTION('',(1.73472347597681E-15,-1.,2.89120579329468E-16)) ;
#79860=DIRECTION('center_axis',(-0.573462344363329,0.81923192051904,0.)) ;
#79861=DIRECTION('ref_axis',(-0.81923192051904,-0.573462344363329,0.)) ;
#79862=DIRECTION('',(-0.710669054518702,-0.497468338163091,0.49746833816309)) ;
#79863=DIRECTION('',(0.,0.,-1.)) ;
#79864=DIRECTION('',(0.710669054518702,0.497468338163091,0.49746833816309)) ;
#79865=DIRECTION('',(0.,0.,1.)) ;
#79866=DIRECTION('center_axis',(-1.,0.,0.)) ;
#79867=DIRECTION('ref_axis',(0.,0.,1.)) ;
#79868=DIRECTION('',(0.,0.,1.)) ;
#79869=DIRECTION('',(0.,-1.,-9.34081871679819E-17)) ;
#79870=DIRECTION('',(0.,0.,-1.)) ;
#79871=DIRECTION('',(0.,1.,-9.34081871679819E-17)) ;
#79872=DIRECTION('center_axis',(-0.573462344363329,-0.81923192051904,0.)) ;
#79873=DIRECTION('ref_axis',(0.81923192051904,-0.573462344363329,0.)) ;
#79874=DIRECTION('',(-0.710669054518701,0.497468338163091,-0.497468338163091)) ;
#79875=DIRECTION('',(0.,0.,1.)) ;
#79876=DIRECTION('',(0.710669054518701,-0.497468338163091,-0.497468338163091)) ;
#79877=DIRECTION('',(0.,0.,-1.)) ;
#79878=DIRECTION('center_axis',(0.,0.,1.)) ;
#79879=DIRECTION('ref_axis',(1.,0.,0.)) ;
#79880=DIRECTION('',(1.,6.67201336914158E-17,0.)) ;
#79881=DIRECTION('',(1.33440267382831E-16,1.,0.)) ;
#79882=DIRECTION('',(-1.,1.33440267382831E-16,0.)) ;
#79883=DIRECTION('center_axis',(0.,0.,1.)) ;
#79884=DIRECTION('ref_axis',(1.,0.,0.)) ;
#79885=DIRECTION('',(1.,-1.33440267382831E-16,0.)) ;
#79886=DIRECTION('',(-1.33440267382831E-16,-1.,0.)) ;
#79887=DIRECTION('',(-1.,-6.67201336914158E-17,0.)) ;
#79888=DIRECTION('center_axis',(-6.67201336914158E-17,1.,0.)) ;
#79889=DIRECTION('ref_axis',(-1.,-6.67201336914158E-17,0.)) ;
#79890=DIRECTION('',(1.,6.67201336914158E-17,0.)) ;
#79891=DIRECTION('',(0.,0.,1.)) ;
#79892=DIRECTION('',(-1.,-6.67201336914158E-17,0.)) ;
#79893=DIRECTION('center_axis',(-1.33440267382831E-16,-1.,0.)) ;
#79894=DIRECTION('ref_axis',(1.,-1.33440267382831E-16,0.)) ;
#79895=DIRECTION('',(1.,-1.33440267382831E-16,0.)) ;
#79896=DIRECTION('',(0.,0.,-1.)) ;
#79897=DIRECTION('',(-1.,1.33440267382831E-16,0.)) ;
#79898=DIRECTION('center_axis',(0.,0.,1.)) ;
#79899=DIRECTION('ref_axis',(1.,0.,0.)) ;
#79900=DIRECTION('',(0.,-1.,0.)) ;
#79901=DIRECTION('',(1.,0.,0.)) ;
#79902=DIRECTION('',(0.,1.,0.)) ;
#79903=DIRECTION('center_axis',(0.,0.,-1.)) ;
#79904=DIRECTION('ref_axis',(1.,0.,0.)) ;
#79905=DIRECTION('',(-1.44560289664734E-16,1.,-7.2280144832367E-17)) ;
#79906=DIRECTION('center_axis',(0.,0.,1.)) ;
#79907=DIRECTION('ref_axis',(1.,0.,0.)) ;
#79908=DIRECTION('center_axis',(0.,0.,1.)) ;
#79909=DIRECTION('ref_axis',(1.,0.,0.)) ;
#79910=DIRECTION('',(0.,-1.,0.)) ;
#79911=DIRECTION('',(-1.,0.,0.)) ;
#79912=DIRECTION('',(0.,1.,0.)) ;
#79913=DIRECTION('center_axis',(0.,0.,-1.)) ;
#79914=DIRECTION('ref_axis',(1.,-1.82602471155453E-15,0.)) ;
#79915=DIRECTION('',(1.44560289664734E-16,-1.,-2.4093381610789E-16)) ;
#79916=DIRECTION('center_axis',(0.,0.,1.)) ;
#79917=DIRECTION('ref_axis',(1.,0.,0.)) ;
#79918=DIRECTION('center_axis',(0.,0.,-1.)) ;
#79919=DIRECTION('ref_axis',(-1.,0.,0.)) ;
#79920=DIRECTION('',(0.,0.,-1.)) ;
#79921=DIRECTION('center_axis',(0.,0.,-1.)) ;
#79922=DIRECTION('ref_axis',(1.,0.,0.)) ;
#79923=DIRECTION('center_axis',(0.,0.,1.)) ;
#79924=DIRECTION('ref_axis',(1.,0.,0.)) ;
#79925=DIRECTION('center_axis',(1.,0.,0.)) ;
#79926=DIRECTION('ref_axis',(0.,0.,-1.)) ;
#79927=DIRECTION('',(0.,-1.,0.)) ;
#79928=DIRECTION('',(0.,0.,1.)) ;
#79929=DIRECTION('',(0.,1.,0.)) ;
#79930=DIRECTION('center_axis',(0.81923192051904,0.573462344363329,0.)) ;
#79931=DIRECTION('ref_axis',(-0.573462344363329,0.81923192051904,0.)) ;
#79932=DIRECTION('',(-0.497468338163091,0.710669054518701,0.497468338163091)) ;
#79933=DIRECTION('',(0.,0.,-1.)) ;
#79934=DIRECTION('',(0.497468338163091,-0.710669054518701,0.497468338163091)) ;
#79935=DIRECTION('',(0.,0.,1.)) ;
#79936=DIRECTION('center_axis',(0.,1.,0.)) ;
#79937=DIRECTION('ref_axis',(0.,0.,1.)) ;
#79938=DIRECTION('',(0.,0.,1.)) ;
#79939=DIRECTION('',(-1.,0.,0.)) ;
#79940=DIRECTION('',(0.,0.,-1.)) ;
#79941=DIRECTION('',(1.,0.,0.)) ;
#79942=DIRECTION('center_axis',(-0.81923192051904,0.573462344363329,0.)) ;
#79943=DIRECTION('ref_axis',(-0.573462344363329,-0.81923192051904,0.)) ;
#79944=DIRECTION('',(0.497468338163091,0.710669054518701,-0.497468338163091)) ;
#79945=DIRECTION('',(0.,0.,1.)) ;
#79946=DIRECTION('',(-0.497468338163091,-0.710669054518701,-0.497468338163091)) ;
#79947=DIRECTION('',(0.,0.,-1.)) ;
#79948=DIRECTION('center_axis',(-1.,0.,0.)) ;
#79949=DIRECTION('ref_axis',(0.,0.,1.)) ;
#79950=DIRECTION('',(0.,-1.,0.)) ;
#79951=DIRECTION('',(0.,0.,-1.)) ;
#79952=DIRECTION('',(0.,1.,0.)) ;
#79953=DIRECTION('',(0.,0.,-1.)) ;
#79954=DIRECTION('center_axis',(0.,0.,-1.)) ;
#79955=DIRECTION('ref_axis',(-1.,0.,0.)) ;
#79956=DIRECTION('center_axis',(0.,0.,1.)) ;
#79957=DIRECTION('ref_axis',(1.,0.,0.)) ;
#79958=DIRECTION('center_axis',(0.,0.,-1.)) ;
#79959=DIRECTION('ref_axis',(1.,5.20417042793042E-15,0.)) ;
#79960=DIRECTION('center_axis',(-0.573462344363328,7.65229685658278E-17,
0.819231920519041)) ;
#79961=DIRECTION('ref_axis',(0.819231920519041,1.22423955297878E-32,0.573462344363328)) ;
#79962=DIRECTION('',(-0.710669054518702,-0.497468338163091,-0.497468338163091)) ;
#79963=DIRECTION('',(1.33440267382831E-16,1.,-2.91413396387194E-34)) ;
#79964=DIRECTION('',(0.710669054518701,-0.497468338163091,0.497468338163091)) ;
#79965=DIRECTION('',(5.04890651880155E-33,-1.,9.34081871679819E-17)) ;
#79966=DIRECTION('center_axis',(-0.573462344363328,7.65229685658278E-17,
-0.819231920519041)) ;
#79967=DIRECTION('ref_axis',(-0.819231920519041,-1.22423955297878E-32,0.573462344363328)) ;
#79968=DIRECTION('',(-0.710669054518701,0.497468338163091,0.497468338163091)) ;
#79969=DIRECTION('',(-1.33440267382831E-16,-1.,7.77328292223541E-33)) ;
#79970=DIRECTION('',(0.710669054518702,0.497468338163091,-0.497468338163091)) ;
#79971=DIRECTION('',(-5.04890651880155E-33,1.,9.34081871679819E-17)) ;
#79972=DIRECTION('center_axis',(0.,0.573462344363328,-0.819231920519041)) ;
#79973=DIRECTION('ref_axis',(0.,0.819231920519041,0.573462344363328)) ;
#79974=DIRECTION('',(0.497468338163091,0.710669054518701,0.497468338163091)) ;
#79975=DIRECTION('',(-1.,0.,0.)) ;
#79976=DIRECTION('',(0.497468338163091,-0.710669054518701,-0.497468338163091)) ;
#79977=DIRECTION('',(1.,0.,0.)) ;
#79978=DIRECTION('center_axis',(0.,0.573462344363328,0.819231920519041)) ;
#79979=DIRECTION('ref_axis',(0.,-0.819231920519041,0.573462344363328)) ;
#79980=DIRECTION('',(-0.497468338163091,0.710669054518701,-0.497468338163091)) ;
#79981=DIRECTION('',(1.,0.,0.)) ;
#79982=DIRECTION('',(-0.497468338163091,-0.710669054518701,0.497468338163091)) ;
#79983=DIRECTION('',(-1.,0.,0.)) ;
#79984=DIRECTION('center_axis',(-0.164398987305354,-0.986393923832144,0.)) ;
#79985=DIRECTION('ref_axis',(0.,0.,1.)) ;
#79986=DIRECTION('',(0.,0.,-1.)) ;
#79987=DIRECTION('center_axis',(-0.164398987305423,-0.986393923832133,1.19343312735544E-12)) ;
#79988=DIRECTION('ref_axis',(-0.057729035739095,0.0096215059577276,0.998285923498744)) ;
#79989=DIRECTION('',(0.,0.,1.)) ;
#79990=DIRECTION('center_axis',(1.,-2.89120579329441E-16,0.)) ;
#79991=DIRECTION('ref_axis',(-2.89120579329441E-16,-1.,-3.43024899888577E-15)) ;
#79992=DIRECTION('center_axis',(1.,1.15648231731787E-15,0.)) ;
#79993=DIRECTION('ref_axis',(1.15648231731787E-15,-1.,0.)) ;
#79994=DIRECTION('center_axis',(0.166689823575762,0.983956802822934,0.0635886223687179)) ;
#79995=DIRECTION('ref_axis',(-0.0486480010045635,0.0726194157819113,-0.996172571620878)) ;
#79996=DIRECTION('center_axis',(0.166689823572632,0.983956802827715,-0.0635886223029427)) ;
#79997=DIRECTION('ref_axis',(-0.0462047034091838,0.072214919352298,0.996318287900915)) ;
#79998=DIRECTION('center_axis',(-0.164398987305354,-0.986393923832144,0.)) ;
#79999=DIRECTION('ref_axis',(0.,0.,1.)) ;
#80000=DIRECTION('',(0.,0.,1.)) ;
#80001=DIRECTION('center_axis',(-0.164398987305404,-0.986393923832136,-8.67951365333722E-13)) ;
#80002=DIRECTION('ref_axis',(-0.0554192327871164,0.00923653879873397,-0.99842045000506)) ;
#80003=DIRECTION('',(0.,0.,-1.)) ;
#80004=DIRECTION('center_axis',(0.,0.,1.)) ;
#80005=DIRECTION('ref_axis',(1.,0.,0.)) ;
#80006=DIRECTION('center_axis',(0.,0.,1.)) ;
#80007=DIRECTION('ref_axis',(1.,0.,0.)) ;
#80008=DIRECTION('center_axis',(0.,1.,0.)) ;
#80009=DIRECTION('ref_axis',(1.,0.,0.)) ;
#80010=DIRECTION('center_axis',(0.,-0.888198741900269,0.45945945945946)) ;
#80011=DIRECTION('ref_axis',(0.,0.45945945945946,0.888198741900269)) ;
#80012=DIRECTION('center_axis',(-1.,0.,1.22067519501986E-15)) ;
#80013=DIRECTION('ref_axis',(-1.22067519501986E-15,0.,-1.)) ;
#80014=DIRECTION('center_axis',(0.,0.,1.)) ;
#80015=DIRECTION('ref_axis',(1.,0.,0.)) ;
#80016=DIRECTION('center_axis',(0.,0.,-1.)) ;
#80017=DIRECTION('ref_axis',(-1.,0.,0.)) ;
#80018=DIRECTION('center_axis',(1.,-3.46944695195361E-16,0.)) ;
#80019=DIRECTION('ref_axis',(3.46944695195361E-16,1.,0.)) ;
#80020=DIRECTION('center_axis',(-1.,3.46944695195361E-16,0.)) ;
#80021=DIRECTION('ref_axis',(3.46944695195361E-16,1.,2.168404344971E-15)) ;
#80022=DIRECTION('center_axis',(-1.,3.46944695195361E-16,0.)) ;
#80023=DIRECTION('ref_axis',(-3.41607084500048E-16,-1.,0.)) ;
#80024=DIRECTION('center_axis',(0.,-0.459459459459457,0.888198741900271)) ;
#80025=DIRECTION('ref_axis',(0.,-0.888198741900271,-0.459459459459457)) ;
#80026=DIRECTION('center_axis',(1.,-3.46944695195361E-16,0.)) ;
#80027=DIRECTION('ref_axis',(0.,1.,0.)) ;
#80028=DIRECTION('center_axis',(0.,0.888198741900269,-0.45945945945946)) ;
#80029=DIRECTION('ref_axis',(0.,-0.45945945945946,-0.888198741900269)) ;
#80030=DIRECTION('center_axis',(0.,1.,0.)) ;
#80031=DIRECTION('ref_axis',(1.,0.,0.)) ;
#80032=DIRECTION('center_axis',(0.,-1.,0.)) ;
#80033=DIRECTION('ref_axis',(0.,0.,1.)) ;
#80034=DIRECTION('center_axis',(-1.,0.,0.)) ;
#80035=DIRECTION('ref_axis',(0.,0.,-1.)) ;
#80036=DIRECTION('center_axis',(0.,0.,-1.)) ;
#80037=DIRECTION('ref_axis',(-1.,0.,0.)) ;
#80038=DIRECTION('center_axis',(0.,0.,-1.)) ;
#80039=DIRECTION('ref_axis',(-1.,0.,0.)) ;
#80040=DIRECTION('center_axis',(1.,-3.46944695195361E-16,0.)) ;
#80041=DIRECTION('ref_axis',(3.46944695195361E-16,1.,0.)) ;
#80042=DIRECTION('center_axis',(-1.,3.46944695195361E-16,0.)) ;
#80043=DIRECTION('ref_axis',(3.46944695195361E-16,1.,0.)) ;
#80044=DIRECTION('center_axis',(1.,0.,0.)) ;
#80045=DIRECTION('ref_axis',(0.,0.,-1.)) ;
#80046=DIRECTION('center_axis',(0.,0.,1.)) ;
#80047=DIRECTION('ref_axis',(1.,0.,0.)) ;
#80048=DIRECTION('center_axis',(0.,0.,1.)) ;
#80049=DIRECTION('ref_axis',(1.,0.,0.)) ;
#80050=DIRECTION('center_axis',(1.,-3.46944695195361E-16,0.)) ;
#80051=DIRECTION('ref_axis',(3.80647894157197E-16,1.,0.)) ;
#80052=DIRECTION('center_axis',(0.,0.459459459459459,-0.888198741900269)) ;
#80053=DIRECTION('ref_axis',(0.,0.88819874190027,0.459459459459459)) ;
#80054=DIRECTION('center_axis',(1.,-3.46944695195361E-16,0.)) ;
#80055=DIRECTION('ref_axis',(3.46944695195361E-16,1.,0.)) ;
#80056=DIRECTION('center_axis',(-1.,3.46944695195361E-16,0.)) ;
#80057=DIRECTION('ref_axis',(3.46944695195361E-16,1.,-3.25260651745651E-15)) ;
#80058=DIRECTION('center_axis',(-3.46944695195361E-16,-1.,-6.49299968442375E-16)) ;
#80059=DIRECTION('ref_axis',(2.25271179641597E-31,6.49299968442375E-16,
-1.)) ;
#80060=DIRECTION('center_axis',(0.,-1.,0.)) ;
#80061=DIRECTION('ref_axis',(0.,0.,-1.)) ;
#80062=DIRECTION('center_axis',(0.,0.,1.)) ;
#80063=DIRECTION('ref_axis',(1.,0.,0.)) ;
#80064=DIRECTION('center_axis',(-3.25260651745651E-15,0.,1.)) ;
#80065=DIRECTION('ref_axis',(1.,0.,3.25260651745651E-15)) ;
#80066=DIRECTION('center_axis',(0.,1.,0.)) ;
#80067=DIRECTION('ref_axis',(1.,0.,0.)) ;
#80068=DIRECTION('center_axis',(0.,-0.888198741900269,-0.45945945945946)) ;
#80069=DIRECTION('ref_axis',(0.,-0.45945945945946,0.888198741900269)) ;
#80070=DIRECTION('center_axis',(1.,-3.46944695195361E-16,0.)) ;
#80071=DIRECTION('ref_axis',(0.,1.,0.)) ;
#80072=DIRECTION('center_axis',(0.,0.888198741900269,0.45945945945946)) ;
#80073=DIRECTION('ref_axis',(0.,0.45945945945946,-0.888198741900269)) ;
#80074=DIRECTION('center_axis',(1.,-3.46944695195361E-16,0.)) ;
#80075=DIRECTION('ref_axis',(0.,1.,0.)) ;
#80076=DIRECTION('center_axis',(0.,1.,0.)) ;
#80077=DIRECTION('ref_axis',(0.,0.,-1.)) ;
#80078=DIRECTION('center_axis',(0.,1.,0.)) ;
#80079=DIRECTION('ref_axis',(1.,0.,0.)) ;
#80080=DIRECTION('center_axis',(-1.,0.,0.)) ;
#80081=DIRECTION('ref_axis',(0.,0.,-1.)) ;
#80082=DIRECTION('center_axis',(1.,-3.46944695195361E-16,0.)) ;
#80083=DIRECTION('ref_axis',(3.41607084500048E-16,1.,0.)) ;
#80084=DIRECTION('center_axis',(-9.62987005567165E-16,-0.459459459459459,
-0.88819874190027)) ;
#80085=DIRECTION('ref_axis',(-9.03304156918849E-31,0.88819874190027,-0.459459459459459)) ;
#80086=DIRECTION('center_axis',(1.,-3.46944695195361E-16,0.)) ;
#80087=DIRECTION('ref_axis',(3.46944695195361E-16,1.,0.)) ;
#80088=DIRECTION('center_axis',(-1.,3.46944695195361E-16,0.)) ;
#80089=DIRECTION('ref_axis',(3.46944695195361E-16,1.,-5.42101086242751E-15)) ;
#80090=DIRECTION('center_axis',(1.,0.,0.)) ;
#80091=DIRECTION('ref_axis',(0.,0.,-1.)) ;
#80092=DIRECTION('center_axis',(1.,-3.46944695195361E-16,0.)) ;
#80093=DIRECTION('ref_axis',(3.80647894157197E-16,1.,0.)) ;
#80094=DIRECTION('center_axis',(0.,0.459459459459459,0.888198741900269)) ;
#80095=DIRECTION('ref_axis',(0.,-0.88819874190027,0.459459459459459)) ;
#80096=DIRECTION('center_axis',(-3.46944695195361E-16,-1.,-6.49299968442375E-16)) ;
#80097=DIRECTION('ref_axis',(2.25271179641597E-31,6.49299968442375E-16,
-1.)) ;
#80098=DIRECTION('center_axis',(0.,1.,0.)) ;
#80099=DIRECTION('ref_axis',(0.,0.,-1.)) ;
#80100=DIRECTION('center_axis',(1.,0.,2.25271179641597E-31)) ;
#80101=DIRECTION('ref_axis',(2.25271179641597E-31,0.,-1.)) ;
#80102=DIRECTION('center_axis',(-1.,0.,0.)) ;
#80103=DIRECTION('ref_axis',(0.,0.,1.)) ;
#80104=DIRECTION('center_axis',(0.,1.,0.)) ;
#80105=DIRECTION('ref_axis',(1.,0.,0.)) ;
#80106=DIRECTION('center_axis',(0.,-1.,0.)) ;
#80107=DIRECTION('ref_axis',(-1.0842021724855E-15,0.,1.)) ;
#80108=DIRECTION('center_axis',(1.,-3.46944695195361E-16,0.)) ;
#80109=DIRECTION('ref_axis',(0.,1.,0.)) ;
#80110=DIRECTION('center_axis',(0.,1.,0.)) ;
#80111=DIRECTION('ref_axis',(0.,0.,-1.)) ;
#80112=DIRECTION('center_axis',(0.,-1.,0.)) ;
#80113=DIRECTION('ref_axis',(0.,0.,-1.)) ;
#80114=DIRECTION('center_axis',(0.,0.,1.)) ;
#80115=DIRECTION('ref_axis',(-1.,0.,0.)) ;
#80116=DIRECTION('center_axis',(0.,0.,-1.)) ;
#80117=DIRECTION('ref_axis',(-1.,0.,0.)) ;
#80118=DIRECTION('center_axis',(0.,0.,-1.)) ;
#80119=DIRECTION('ref_axis',(-1.,0.,0.)) ;
#80120=DIRECTION('center_axis',(-3.46944695195361E-16,-1.,-9.27571383489107E-17)) ;
#80121=DIRECTION('ref_axis',(1.,-3.46944695195361E-16,-3.21815970916568E-32)) ;
#80122=DIRECTION('center_axis',(0.,-1.,0.)) ;
#80123=DIRECTION('ref_axis',(0.,0.,-1.)) ;
#80124=DIRECTION('center_axis',(3.46944695195361E-16,1.,9.27571383489107E-17)) ;
#80125=DIRECTION('ref_axis',(-1.,3.46944695195361E-16,3.21815970916568E-32)) ;
#80126=DIRECTION('center_axis',(0.,1.,0.)) ;
#80127=DIRECTION('ref_axis',(0.,0.,-1.)) ;
#80128=DIRECTION('center_axis',(0.,0.,-1.)) ;
#80129=DIRECTION('ref_axis',(-1.,0.,0.)) ;
#80130=DIRECTION('center_axis',(0.,0.,1.)) ;
#80131=DIRECTION('ref_axis',(1.,0.,0.)) ;
#80132=DIRECTION('center_axis',(0.,1.,0.)) ;
#80133=DIRECTION('ref_axis',(1.,0.,0.)) ;
#80134=DIRECTION('center_axis',(-1.,0.,1.0842021724855E-15)) ;
#80135=DIRECTION('ref_axis',(-1.0842021724855E-15,0.,-1.)) ;
#80136=DIRECTION('center_axis',(0.,-1.,0.)) ;
#80137=DIRECTION('ref_axis',(0.,0.,-1.)) ;
#80138=DIRECTION('center_axis',(1.,0.,0.)) ;
#80139=DIRECTION('ref_axis',(0.,0.,1.)) ;
#80140=DIRECTION('center_axis',(1.,0.,3.21815970916568E-32)) ;
#80141=DIRECTION('ref_axis',(3.21815970916568E-32,0.,-1.)) ;
#80142=DIRECTION('center_axis',(0.,1.,0.)) ;
#80143=DIRECTION('ref_axis',(1.,0.,0.)) ;
#80144=DIRECTION('center_axis',(0.,0.,-1.)) ;
#80145=DIRECTION('ref_axis',(1.,0.,0.)) ;
#80146=DIRECTION('center_axis',(1.,0.,0.)) ;
#80147=DIRECTION('ref_axis',(0.,-1.0842021724855E-15,1.)) ;
#80148=DIRECTION('center_axis',(1.0842021724855E-15,1.,0.)) ;
#80149=DIRECTION('ref_axis',(1.,-1.0842021724855E-15,0.)) ;
#80150=DIRECTION('center_axis',(1.,0.,-2.08976773479518E-32)) ;
#80151=DIRECTION('ref_axis',(-2.08976773479518E-32,0.,-1.)) ;
#80152=DIRECTION('center_axis',(-0.447220452189876,-7.10036016473618E-6,
-0.894423762593922)) ;
#80153=DIRECTION('ref_axis',(0.894325663269753,0.0148067719390998,-0.447171519130926)) ;
#80154=DIRECTION('center_axis',(-1.23908819712629E-16,1.,2.4093381610789E-16)) ;
#80155=DIRECTION('ref_axis',(2.98538247827883E-32,-2.4093381610789E-16,
1.)) ;
#80156=DIRECTION('center_axis',(-5.60223391439791E-6,-0.447219005480428,
-0.894424485971684)) ;
#80157=DIRECTION('ref_axis',(0.0146917039380788,0.894327914919915,-0.447170811245985)) ;
#80158=DIRECTION('center_axis',(-8.95614743483648E-33,0.,1.)) ;
#80159=DIRECTION('ref_axis',(1.,0.,8.95614743483648E-33)) ;
#80160=DIRECTION('center_axis',(1.40488587213121E-32,-1.23908819712629E-16,
-1.)) ;
#80161=DIRECTION('ref_axis',(1.74077750246726E-48,1.,-1.23908819712629E-16)) ;
#80162=DIRECTION('center_axis',(-2.65552944032596E-32,0.,1.)) ;
#80163=DIRECTION('ref_axis',(1.,0.,2.65552944032596E-32)) ;
#80164=DIRECTION('center_axis',(0.8944244859717,-5.60223399946766E-6,0.447219005480397)) ;
#80165=DIRECTION('ref_axis',(0.447170811245932,0.0146917039416789,-0.894327914919883)) ;
#80166=DIRECTION('center_axis',(0.894423762593955,-7.10036019092399E-6,
-0.447220452189809)) ;
#80167=DIRECTION('ref_axis',(0.44717151913086,0.0148067719390903,0.894325663269786)) ;
#80168=DIRECTION('center_axis',(-8.95614743483648E-33,-1.10974565782288E-48,
1.)) ;
#80169=DIRECTION('ref_axis',(1.,-9.9390457266313E-81,8.95614743483648E-33)) ;
#80170=DIRECTION('center_axis',(-7.10036022482307E-6,0.894423762593866,
0.447220452189987)) ;
#80171=DIRECTION('ref_axis',(-0.014806771937735,-0.447171519131047,0.894325663269715)) ;
#80172=DIRECTION('center_axis',(-5.60223398444571E-6,0.894424485971634,
-0.447219005480529)) ;
#80173=DIRECTION('ref_axis',(0.0146917039434335,0.447170811246052,0.894327914919794)) ;
#80174=DIRECTION('center_axis',(1.40488587213121E-32,-1.23908819712629E-16,
-1.)) ;
#80175=DIRECTION('ref_axis',(0.,1.,0.)) ;
#80176=DIRECTION('center_axis',(-1.,0.,0.)) ;
#80177=DIRECTION('ref_axis',(0.,0.,-1.)) ;
#80178=DIRECTION('center_axis',(0.,-1.,0.)) ;
#80179=DIRECTION('ref_axis',(0.,0.,1.)) ;
#80180=DIRECTION('center_axis',(-1.,0.,-1.40488587213121E-32)) ;
#80181=DIRECTION('ref_axis',(-1.40488587213121E-32,0.,1.)) ;
#80182=DIRECTION('',(-1.,0.,-1.40488587213121E-32)) ;
#80183=DIRECTION('center_axis',(-1.,0.,0.)) ;
#80184=DIRECTION('ref_axis',(0.,0.,1.)) ;
#80185=DIRECTION('center_axis',(0.,1.,0.)) ;
#80186=DIRECTION('ref_axis',(1.,0.,0.)) ;
#80187=DIRECTION('center_axis',(0.,1.,0.)) ;
#80188=DIRECTION('ref_axis',(0.,0.,-1.)) ;
#80189=DIRECTION('center_axis',(0.,0.,-1.)) ;
#80190=DIRECTION('ref_axis',(1.,0.,0.)) ;
#80191=DIRECTION('center_axis',(-1.,0.,-1.7912294869673E-32)) ;
#80192=DIRECTION('ref_axis',(-1.7912294869673E-32,0.,1.)) ;
#80193=DIRECTION('center_axis',(-0.447219005480468,-5.60223398368281E-6,
0.894424485971665)) ;
#80194=DIRECTION('ref_axis',(0.894327914919842,0.0146917039421028,0.447170811245999)) ;
#80195=DIRECTION('center_axis',(-1.,0.,0.)) ;
#80196=DIRECTION('ref_axis',(0.,0.,1.)) ;
#80197=DIRECTION('center_axis',(1.23908819712629E-16,-1.,7.2280144832367E-17)) ;
#80198=DIRECTION('ref_axis',(1.,1.23908819712629E-16,-8.95614743483648E-33)) ;
#80199=DIRECTION('center_axis',(-7.10036017276901E-6,-0.447220452189912,
0.894423762593904)) ;
#80200=DIRECTION('ref_axis',(-0.0148067719326949,-0.894325663269819,-0.447171519131005)) ;
#80201=DIRECTION('center_axis',(0.,-1.,1.0842021724855E-15)) ;
#80202=DIRECTION('ref_axis',(0.,-1.0842021724855E-15,-1.)) ;
#80203=DIRECTION('center_axis',(1.23908819712629E-16,-1.,1.23908819712629E-16)) ;
#80204=DIRECTION('ref_axis',(3.09997069395837E-48,-1.23908819712629E-16,
-1.)) ;
#80205=DIRECTION('center_axis',(0.,-1.,0.)) ;
#80206=DIRECTION('ref_axis',(0.,0.,-1.)) ;
#80207=DIRECTION('',(-1.23908819712629E-16,1.,-1.23908819712629E-16)) ;
#80208=DIRECTION('center_axis',(1.,0.,1.40488587213121E-32)) ;
#80209=DIRECTION('ref_axis',(1.40488587213121E-32,0.,-1.)) ;
#80210=DIRECTION('center_axis',(-0.707106781186547,0.707106781186548,-7.05268145719433E-16)) ;
#80211=DIRECTION('ref_axis',(0.707106781186548,0.707106781186547,-6.32735679406601E-14)) ;
#80212=DIRECTION('center_axis',(1.,0.,0.)) ;
#80213=DIRECTION('ref_axis',(0.,0.,-1.)) ;
#80214=DIRECTION('center_axis',(0.,-1.,0.)) ;
#80215=DIRECTION('ref_axis',(0.,0.,-1.)) ;
#80216=DIRECTION('center_axis',(0.,0.,1.)) ;
#80217=DIRECTION('ref_axis',(-1.,0.,0.)) ;
#80218=DIRECTION('center_axis',(7.2280144832367E-17,0.,-1.)) ;
#80219=DIRECTION('ref_axis',(-1.,0.,-7.2280144832367E-17)) ;
#80220=DIRECTION('',(7.2280144832367E-17,0.,-1.)) ;
#80221=DIRECTION('center_axis',(0.,0.,-1.)) ;
#80222=DIRECTION('ref_axis',(-1.,0.,0.)) ;
#80223=DIRECTION('center_axis',(0.,1.,0.)) ;
#80224=DIRECTION('ref_axis',(1.,0.,0.)) ;
#80225=DIRECTION('center_axis',(0.,0.,1.)) ;
#80226=DIRECTION('ref_axis',(-1.,0.,0.)) ;
#80227=DIRECTION('center_axis',(0.,1.,0.)) ;
#80228=DIRECTION('ref_axis',(1.,0.,0.)) ;
#80229=DIRECTION('center_axis',(1.,0.,0.)) ;
#80230=DIRECTION('ref_axis',(0.,0.,1.)) ;
#80231=DIRECTION('center_axis',(0.,0.,-1.)) ;
#80232=DIRECTION('ref_axis',(1.,0.,0.)) ;
#80233=DIRECTION('center_axis',(-1.13380619344889E-16,1.,-1.23908819712629E-16)) ;
#80234=DIRECTION('ref_axis',(-1.40488587213121E-32,1.23908819712629E-16,
1.)) ;
#80235=DIRECTION('center_axis',(0.,1.,0.)) ;
#80236=DIRECTION('ref_axis',(0.,0.,1.)) ;
#80237=DIRECTION('center_axis',(7.2280144832367E-17,0.,-1.)) ;
#80238=DIRECTION('ref_axis',(-1.,0.,-7.2280144832367E-17)) ;
#80239=DIRECTION('center_axis',(0.,0.,1.)) ;
#80240=DIRECTION('ref_axis',(1.,0.,0.)) ;
#80241=DIRECTION('center_axis',(0.,1.,0.)) ;
#80242=DIRECTION('ref_axis',(1.,0.,0.)) ;
#80243=DIRECTION('center_axis',(0.,1.,0.)) ;
#80244=DIRECTION('ref_axis',(0.,0.,-1.)) ;
#80245=DIRECTION('center_axis',(1.,2.16840434497101E-15,-2.93873587705572E-31)) ;
#80246=DIRECTION('ref_axis',(2.16840434497101E-15,-1.,-1.03035812136257E-62)) ;
#80247=DIRECTION('center_axis',(-8.95614743483648E-33,0.,1.)) ;
#80248=DIRECTION('ref_axis',(1.,0.,8.95614743483648E-33)) ;
#80249=DIRECTION('center_axis',(-1.40488587213121E-32,1.23908819712629E-16,
1.)) ;
#80250=DIRECTION('ref_axis',(-1.74077750246726E-48,-1.,1.23908819712629E-16)) ;
#80251=DIRECTION('center_axis',(8.95614743483648E-33,1.0154535431059E-48,
-1.)) ;
#80252=DIRECTION('ref_axis',(-1.,1.76545184268265E-95,-8.95614743483648E-33)) ;
#80253=DIRECTION('center_axis',(2.16840434497101E-15,0.,-1.)) ;
#80254=DIRECTION('ref_axis',(-1.,0.,-2.16840434497101E-15)) ;
#80255=DIRECTION('',(-8.95614743483648E-33,-1.0154535431059E-48,1.)) ;
#80256=DIRECTION('center_axis',(-1.,-1.13380619344889E-16,0.)) ;
#80257=DIRECTION('ref_axis',(0.,-1.,0.)) ;
#80258=DIRECTION('center_axis',(0.,0.,1.)) ;
#80259=DIRECTION('ref_axis',(-1.,0.,0.)) ;
#80260=DIRECTION('center_axis',(0.,-1.,0.)) ;
#80261=DIRECTION('ref_axis',(0.,0.,-1.)) ;
#80262=DIRECTION('center_axis',(-1.,0.,0.)) ;
#80263=DIRECTION('ref_axis',(0.,0.,-1.)) ;
#80264=DIRECTION('center_axis',(1.,0.,1.40488587213121E-32)) ;
#80265=DIRECTION('ref_axis',(1.40488587213121E-32,0.,-1.)) ;
#80266=DIRECTION('',(1.,0.,1.40488587213121E-32)) ;
#80267=DIRECTION('center_axis',(1.,0.,0.)) ;
#80268=DIRECTION('ref_axis',(0.,0.,-1.)) ;
#80269=DIRECTION('center_axis',(-1.40488587213121E-32,1.23908819712629E-16,
1.)) ;
#80270=DIRECTION('ref_axis',(0.,-1.,0.)) ;
#80271=DIRECTION('center_axis',(0.,-1.,0.)) ;
#80272=DIRECTION('ref_axis',(0.,0.,1.)) ;
#80273=DIRECTION('center_axis',(0.,1.,0.)) ;
#80274=DIRECTION('ref_axis',(1.,0.,0.)) ;
#80275=DIRECTION('center_axis',(1.,0.,0.)) ;
#80276=DIRECTION('ref_axis',(0.,0.,1.)) ;
#80277=DIRECTION('center_axis',(0.,1.,0.)) ;
#80278=DIRECTION('ref_axis',(0.,0.,-1.)) ;
#80279=DIRECTION('center_axis',(0.,0.,1.)) ;
#80280=DIRECTION('ref_axis',(1.,0.,0.)) ;
#80281=DIRECTION('center_axis',(0.,0.,1.)) ;
#80282=DIRECTION('ref_axis',(1.,0.,0.)) ;
#80283=DIRECTION('center_axis',(1.,0.,1.40488587213121E-32)) ;
#80284=DIRECTION('ref_axis',(1.40488587213121E-32,0.,-1.)) ;
#80285=DIRECTION('center_axis',(-0.707106781186543,0.707106781186552,9.74552346812296E-15)) ;
#80286=DIRECTION('ref_axis',(0.707106781186552,0.707106781186543,-2.44769167512091E-14)) ;
#80287=DIRECTION('center_axis',(-1.23908819712629E-16,1.,-1.23908819712629E-16)) ;
#80288=DIRECTION('ref_axis',(-3.09997069395837E-48,1.23908819712629E-16,
1.)) ;
#80289=DIRECTION('',(1.23908819712629E-16,-1.,1.23908819712629E-16)) ;
#80290=DIRECTION('center_axis',(-1.,-1.13380619344889E-16,0.)) ;
#80291=DIRECTION('ref_axis',(0.,-1.,0.)) ;
#80292=DIRECTION('center_axis',(0.,-1.,0.)) ;
#80293=DIRECTION('ref_axis',(0.,0.,1.)) ;
#80294=DIRECTION('center_axis',(1.13380619344889E-16,-1.,1.23908819712629E-16)) ;
#80295=DIRECTION('ref_axis',(1.40488587213121E-32,-1.23908819712629E-16,
-1.)) ;
#80296=DIRECTION('center_axis',(-1.5529910948782E-31,-4.47619207437002E-16,
1.)) ;
#80297=DIRECTION('ref_axis',(-1.26404997831554E-61,-1.,-4.47619207437002E-16)) ;
#80298=DIRECTION('center_axis',(0.,2.16840434497101E-15,-1.)) ;
#80299=DIRECTION('ref_axis',(0.,1.,2.16840434497101E-15)) ;
#80300=DIRECTION('center_axis',(0.,1.,0.)) ;
#80301=DIRECTION('ref_axis',(1.,0.,0.)) ;
#80302=DIRECTION('center_axis',(3.85194802226865E-15,0.888198741900269,
-0.45945945945946)) ;
#80303=DIRECTION('ref_axis',(1.56255765105114E-31,-0.45945945945946,-0.888198741900269)) ;
#80304=DIRECTION('center_axis',(-1.,0.,1.22067519501986E-15)) ;
#80305=DIRECTION('ref_axis',(-1.22067519501986E-15,-4.33680868994202E-15,
-1.)) ;
#80306=DIRECTION('center_axis',(1.5529910948782E-31,4.47619207437002E-16,
-1.)) ;
#80307=DIRECTION('ref_axis',(-6.951486430461E-47,1.,4.47619207437002E-16)) ;
#80308=DIRECTION('center_axis',(0.,0.,1.)) ;
#80309=DIRECTION('ref_axis',(1.,0.,0.)) ;
#80310=DIRECTION('center_axis',(1.,-3.46944695195361E-16,0.)) ;
#80311=DIRECTION('ref_axis',(3.46944695195361E-16,1.,0.)) ;
#80312=DIRECTION('center_axis',(-1.,3.46944695195361E-16,0.)) ;
#80313=DIRECTION('ref_axis',(3.46944695195361E-16,1.,0.)) ;
#80314=DIRECTION('center_axis',(1.,-3.46944695195361E-16,0.)) ;
#80315=DIRECTION('ref_axis',(3.41607084500048E-16,1.,0.)) ;
#80316=DIRECTION('center_axis',(0.,0.459459459459457,-0.888198741900271)) ;
#80317=DIRECTION('ref_axis',(0.,0.888198741900271,0.459459459459457)) ;
#80318=DIRECTION('center_axis',(0.,0.,1.)) ;
#80319=DIRECTION('ref_axis',(1.,0.,0.)) ;
#80320=DIRECTION('center_axis',(0.,0.,-1.)) ;
#80321=DIRECTION('ref_axis',(-1.,0.,0.)) ;
#80322=DIRECTION('center_axis',(-1.,3.46944695195361E-16,0.)) ;
#80323=DIRECTION('ref_axis',(-3.46944695195361E-16,-1.,0.)) ;
#80324=DIRECTION('center_axis',(-1.,3.46944695195361E-16,0.)) ;
#80325=DIRECTION('ref_axis',(-3.46944695195361E-16,-1.,0.)) ;
#80326=DIRECTION('center_axis',(-1.,3.46944695195361E-16,0.)) ;
#80327=DIRECTION('ref_axis',(3.46944695195361E-16,1.,0.)) ;
#80328=DIRECTION('center_axis',(1.,-3.46944695195361E-16,0.)) ;
#80329=DIRECTION('ref_axis',(0.,1.,0.)) ;
#80330=DIRECTION('center_axis',(0.,-0.888198741900269,0.459459459459461)) ;
#80331=DIRECTION('ref_axis',(0.,0.459459459459461,0.888198741900269)) ;
#80332=DIRECTION('center_axis',(0.,1.,0.)) ;
#80333=DIRECTION('ref_axis',(1.,0.,0.)) ;
#80334=DIRECTION('center_axis',(0.,1.,0.)) ;
#80335=DIRECTION('ref_axis',(1.0842021724855E-15,0.,-1.)) ;
#80336=DIRECTION('center_axis',(-1.,0.,0.)) ;
#80337=DIRECTION('ref_axis',(0.,0.,-1.)) ;
#80338=DIRECTION('center_axis',(1.,-3.46944695195361E-16,0.)) ;
#80339=DIRECTION('ref_axis',(3.70074341541719E-16,1.,0.)) ;
#80340=DIRECTION('center_axis',(0.,0.63294893130157,-0.774193548387094)) ;
#80341=DIRECTION('ref_axis',(-1.0842021724855E-15,-0.774193548387094,-0.63294893130157)) ;
#80342=DIRECTION('center_axis',(1.,-3.46944695195361E-16,0.)) ;
#80343=DIRECTION('ref_axis',(3.80647894157197E-16,1.,0.)) ;
#80344=DIRECTION('center_axis',(0.,-0.45945945945946,0.888198741900269)) ;
#80345=DIRECTION('ref_axis',(0.,-0.888198741900269,-0.45945945945946)) ;
#80346=DIRECTION('center_axis',(1.,-3.46944695195361E-16,0.)) ;
#80347=DIRECTION('ref_axis',(3.46944695195361E-16,1.,0.)) ;
#80348=DIRECTION('center_axis',(-1.,3.46944695195361E-16,0.)) ;
#80349=DIRECTION('ref_axis',(3.46944695195361E-16,1.,-7.58941520739854E-15)) ;
#80350=DIRECTION('center_axis',(-3.46944695195361E-16,-1.,-2.45739631480277E-16)) ;
#80351=DIRECTION('ref_axis',(1.,-3.46944695195361E-16,-8.52580615413453E-32)) ;
#80352=DIRECTION('center_axis',(0.,1.,0.)) ;
#80353=DIRECTION('ref_axis',(0.,0.,1.)) ;
#80354=DIRECTION('center_axis',(1.,-3.46944695195361E-16,0.)) ;
#80355=DIRECTION('ref_axis',(3.33066907387547E-16,1.,0.)) ;
#80356=DIRECTION('center_axis',(8.02036034720251E-16,0.293103448275862,
-0.956080733311157)) ;
#80357=DIRECTION('ref_axis',(-2.28610793645795E-31,0.956080733311157,0.293103448275862)) ;
#80358=DIRECTION('center_axis',(-1.,3.46944695195361E-16,0.)) ;
#80359=DIRECTION('ref_axis',(-3.46944695195361E-16,-1.,0.)) ;
#80360=DIRECTION('center_axis',(-1.,3.46944695195361E-16,0.)) ;
#80361=DIRECTION('ref_axis',(-3.46944695195361E-16,-1.,0.)) ;
#80362=DIRECTION('center_axis',(-1.,3.46944695195361E-16,0.)) ;
#80363=DIRECTION('ref_axis',(-3.46944695195361E-16,-1.,0.)) ;
#80364=DIRECTION('center_axis',(0.,0.,-1.)) ;
#80365=DIRECTION('ref_axis',(-1.,0.,0.)) ;
#80366=DIRECTION('center_axis',(0.,0.,1.)) ;
#80367=DIRECTION('ref_axis',(1.,0.,0.)) ;
#80368=DIRECTION('center_axis',(-1.5529910948782E-31,-4.47619207437002E-16,
-1.)) ;
#80369=DIRECTION('ref_axis',(1.06958075088238E-61,1.,-4.47619207437002E-16)) ;
#80370=DIRECTION('center_axis',(2.16840434497101E-15,0.,1.)) ;
#80371=DIRECTION('ref_axis',(1.,0.,-2.16840434497101E-15)) ;
#80372=DIRECTION('center_axis',(1.,-3.46944695195361E-16,0.)) ;
#80373=DIRECTION('ref_axis',(0.,1.,0.)) ;
#80374=DIRECTION('center_axis',(0.,-1.,0.)) ;
#80375=DIRECTION('ref_axis',(0.,0.,1.)) ;
#80376=DIRECTION('center_axis',(0.577350269189625,0.577350269189627,0.577350269189625)) ;
#80377=DIRECTION('ref_axis',(-0.707106781186548,0.,0.707106781186548)) ;
#80378=DIRECTION('center_axis',(-1.,3.46944695195361E-16,0.)) ;
#80379=DIRECTION('ref_axis',(-3.70074341541719E-16,-1.,0.)) ;
#80380=DIRECTION('center_axis',(0.,0.63294893130157,0.774193548387094)) ;
#80381=DIRECTION('ref_axis',(0.,0.774193548387094,-0.63294893130157)) ;
#80382=DIRECTION('center_axis',(0.,1.,0.)) ;
#80383=DIRECTION('ref_axis',(1.,0.,0.)) ;
#80384=DIRECTION('center_axis',(-1.,0.,0.)) ;
#80385=DIRECTION('ref_axis',(0.,-4.33680868994202E-15,-1.)) ;
#80386=DIRECTION('center_axis',(0.,0.888198741900271,0.459459459459457)) ;
#80387=DIRECTION('ref_axis',(-1.0842021724855E-15,0.459459459459457,-0.888198741900271)) ;
#80388=DIRECTION('center_axis',(3.46944695195361E-16,1.,2.45739631480277E-16)) ;
#80389=DIRECTION('ref_axis',(-1.,3.46944695195361E-16,8.52580615413453E-32)) ;
#80390=DIRECTION('center_axis',(-1.,3.46944695195361E-16,0.)) ;
#80391=DIRECTION('ref_axis',(-3.33066907387547E-16,-1.,0.)) ;
#80392=DIRECTION('center_axis',(0.,0.293103448275864,0.956080733311156)) ;
#80393=DIRECTION('ref_axis',(0.,-0.956080733311156,0.293103448275864)) ;
#80394=DIRECTION('center_axis',(-3.46944695195361E-16,-1.,-1.06487173641454E-15)) ;
#80395=DIRECTION('ref_axis',(3.69451600012496E-31,1.06487173641454E-15,
-1.)) ;
#80396=DIRECTION('center_axis',(0.,-1.,0.)) ;
#80397=DIRECTION('ref_axis',(0.,0.,-1.)) ;
#80398=DIRECTION('center_axis',(0.,1.,0.)) ;
#80399=DIRECTION('ref_axis',(0.,0.,1.)) ;
#80400=DIRECTION('center_axis',(-1.,3.46944695195361E-16,0.)) ;
#80401=DIRECTION('ref_axis',(-3.41607084500048E-16,-1.,0.)) ;
#80402=DIRECTION('center_axis',(-4.88154879316133E-15,0.45945945945946,
0.888198741900269)) ;
#80403=DIRECTION('ref_axis',(5.19745563204766E-30,-0.888198741900269,0.45945945945946)) ;
#80404=DIRECTION('center_axis',(1.,-3.46944695195361E-16,0.)) ;
#80405=DIRECTION('ref_axis',(3.46944695195361E-16,1.,0.)) ;
#80406=DIRECTION('center_axis',(-1.,3.46944695195361E-16,0.)) ;
#80407=DIRECTION('ref_axis',(3.46944695195361E-16,1.,0.)) ;
#80408=DIRECTION('center_axis',(-1.5529910948782E-31,-4.47619207437002E-16,
-1.)) ;
#80409=DIRECTION('ref_axis',(-6.95148643046101E-47,1.,-4.47619207437002E-16)) ;
#80410=DIRECTION('center_axis',(0.,0.,-1.)) ;
#80411=DIRECTION('ref_axis',(-1.,0.,0.)) ;
#80412=DIRECTION('center_axis',(0.,0.224137931034483,-0.974557431797419)) ;
#80413=DIRECTION('ref_axis',(0.,-0.974557431797419,-0.224137931034483)) ;
#80414=DIRECTION('center_axis',(0.577350269189626,0.577350269189625,0.577350269189626)) ;
#80415=DIRECTION('ref_axis',(-0.707106781186548,0.,0.707106781186548)) ;
#80416=DIRECTION('center_axis',(0.408248290463863,-0.816496580927726,0.408248290463863)) ;
#80417=DIRECTION('ref_axis',(0.707106781186548,0.,-0.707106781186548)) ;
#80418=DIRECTION('center_axis',(0.,1.,0.)) ;
#80419=DIRECTION('ref_axis',(1.,0.,0.)) ;
#80420=DIRECTION('center_axis',(-1.,0.,0.)) ;
#80421=DIRECTION('ref_axis',(0.,-8.67361737988403E-15,-1.)) ;
#80422=DIRECTION('center_axis',(1.,-3.46944695195361E-16,0.)) ;
#80423=DIRECTION('ref_axis',(0.,1.,0.)) ;
#80424=DIRECTION('center_axis',(9.96293888229924E-16,-0.888198741900269,
-0.45945945945946)) ;
#80425=DIRECTION('ref_axis',(-5.65334012505894E-32,-0.45945945945946,0.888198741900269)) ;
#80426=DIRECTION('center_axis',(1.,-3.46944695195361E-16,0.)) ;
#80427=DIRECTION('ref_axis',(-3.70074341541719E-16,-1.,-1.22464679914735E-16)) ;
#80428=DIRECTION('center_axis',(1.58436874053304E-16,-0.224137931034483,
-0.974557431797419)) ;
#80429=DIRECTION('ref_axis',(6.2575771930786E-32,0.974557431797419,-0.224137931034483)) ;
#80430=DIRECTION('center_axis',(1.,-3.46944695195361E-16,0.)) ;
#80431=DIRECTION('ref_axis',(3.46944695195361E-16,1.,0.)) ;
#80432=DIRECTION('center_axis',(-1.,3.46944695195361E-16,0.)) ;
#80433=DIRECTION('ref_axis',(3.46944695195361E-16,1.,3.25260651745652E-15)) ;
#80434=DIRECTION('center_axis',(1.,-3.46944695195361E-16,0.)) ;
#80435=DIRECTION('ref_axis',(3.80647894157197E-16,1.,0.)) ;
#80436=DIRECTION('center_axis',(0.,-0.45945945945946,-0.888198741900269)) ;
#80437=DIRECTION('ref_axis',(0.,0.888198741900269,-0.45945945945946)) ;
#80438=DIRECTION('center_axis',(1.,-3.46944695195361E-16,0.)) ;
#80439=DIRECTION('ref_axis',(0.,1.,0.)) ;
#80440=DIRECTION('center_axis',(0.,-1.,0.)) ;
#80441=DIRECTION('ref_axis',(0.,0.,1.)) ;
#80442=DIRECTION('center_axis',(-3.46944695195361E-16,-1.,-1.06487173641454E-15)) ;
#80443=DIRECTION('ref_axis',(3.69451600012496E-31,1.06487173641454E-15,
-1.)) ;
#80444=DIRECTION('center_axis',(0.,0.,1.)) ;
#80445=DIRECTION('ref_axis',(1.,0.,0.)) ;
#80446=DIRECTION('center_axis',(0.,-1.,0.)) ;
#80447=DIRECTION('ref_axis',(0.,0.,-1.)) ;
#80448=DIRECTION('center_axis',(0.,-1.,0.)) ;
#80449=DIRECTION('ref_axis',(0.,0.,-1.)) ;
#80450=DIRECTION('center_axis',(0.,1.,0.)) ;
#80451=DIRECTION('ref_axis',(0.,0.,-1.)) ;
#80452=DIRECTION('center_axis',(0.,0.,1.)) ;
#80453=DIRECTION('ref_axis',(1.,0.,0.)) ;
#80454=DIRECTION('center_axis',(8.67361737988404E-15,-1.,0.)) ;
#80455=DIRECTION('ref_axis',(1.,8.67361737988404E-15,0.)) ;
#80456=DIRECTION('center_axis',(0.497468338163091,-0.710669054518702,0.497468338163091)) ;
#80457=DIRECTION('ref_axis',(0.81923192051904,0.573462344363328,8.04804396179112E-16)) ;
#80458=DIRECTION('center_axis',(0.497468338163091,-0.710669054518702,0.497468338163091)) ;
#80459=DIRECTION('ref_axis',(0.81923192051904,0.573462344363328,7.6535433881835E-16)) ;
#80460=DIRECTION('center_axis',(0.497468338163092,-0.7106690545187,0.497468338163092)) ;
#80461=DIRECTION('ref_axis',(-2.51524304138174E-16,-0.57346234436333,-0.819231920519039)) ;
#80462=DIRECTION('center_axis',(0.,0.,1.)) ;
#80463=DIRECTION('ref_axis',(1.,0.,0.)) ;
#80464=DIRECTION('center_axis',(0.,-1.,0.)) ;
#80465=DIRECTION('ref_axis',(0.,0.,-1.)) ;
#80466=DIRECTION('center_axis',(0.,1.,0.)) ;
#80467=DIRECTION('ref_axis',(0.,0.,1.)) ;
#80468=DIRECTION('center_axis',(0.,1.,0.)) ;
#80469=DIRECTION('ref_axis',(0.,0.,1.)) ;
#80470=DIRECTION('center_axis',(0.,1.,0.)) ;
#80471=DIRECTION('ref_axis',(1.,0.,0.)) ;
#80472=DIRECTION('center_axis',(-1.98515611757154E-15,0.,1.)) ;
#80473=DIRECTION('ref_axis',(-1.,0.,-1.98515611757154E-15)) ;
#80474=DIRECTION('center_axis',(1.,-4.06575814682065E-16,2.84603070277446E-16)) ;
#80475=DIRECTION('ref_axis',(-4.06575814682065E-16,-1.,6.48893816316174E-47)) ;
#80476=DIRECTION('center_axis',(0.,1.,0.)) ;
#80477=DIRECTION('ref_axis',(0.,0.,1.)) ;
#80478=DIRECTION('center_axis',(0.,1.,0.)) ;
#80479=DIRECTION('ref_axis',(0.,0.,1.)) ;
#80480=DIRECTION('center_axis',(0.497468338163091,0.710669054518702,-0.497468338163091)) ;
#80481=DIRECTION('ref_axis',(-0.81923192051904,0.573462344363328,7.6535433881835E-16)) ;
#80482=DIRECTION('center_axis',(-0.497468338163091,-0.710669054518702,0.497468338163091)) ;
#80483=DIRECTION('ref_axis',(-0.81923192051904,0.57346234436333,3.73565257438817E-15)) ;
#80484=DIRECTION('center_axis',(-0.497468338163093,-0.7106690545187,0.497468338163091)) ;
#80485=DIRECTION('ref_axis',(0.819231920519039,-0.573462344363331,1.48853464230757E-16)) ;
#80486=DIRECTION('center_axis',(1.,0.,0.)) ;
#80487=DIRECTION('ref_axis',(0.,0.,-1.)) ;
#80488=DIRECTION('center_axis',(1.,0.,-9.9257805878577E-16)) ;
#80489=DIRECTION('ref_axis',(-9.9257805878577E-16,0.,-1.)) ;
#80490=DIRECTION('center_axis',(0.,0.,-1.)) ;
#80491=DIRECTION('ref_axis',(-1.,0.,0.)) ;
#80492=DIRECTION('center_axis',(-1.23327997120227E-15,1.76182853028895E-15,
1.)) ;
#80493=DIRECTION('ref_axis',(7.00649232162409E-46,-1.,1.76182853028895E-15)) ;
#80494=DIRECTION('center_axis',(-0.497468338163091,0.710669054518702,0.497468338163091)) ;
#80495=DIRECTION('ref_axis',(-0.81923192051904,-0.573462344363328,7.6535433881835E-16)) ;
#80496=DIRECTION('center_axis',(0.497468338163091,-0.710669054518702,-0.497468338163091)) ;
#80497=DIRECTION('ref_axis',(-0.819231920519043,-0.573462344363324,-7.46600562027492E-15)) ;
#80498=DIRECTION('center_axis',(0.497468338163093,-0.7106690545187,-0.497468338163091)) ;
#80499=DIRECTION('ref_axis',(0.819231920519039,0.573462344363331,2.16059097207149E-16)) ;
#80500=DIRECTION('center_axis',(0.,1.,0.)) ;
#80501=DIRECTION('ref_axis',(1.,0.,0.)) ;
#80502=DIRECTION('center_axis',(-1.13841228110978E-15,-1.62630325872826E-15,
1.)) ;
#80503=DIRECTION('ref_axis',(3.5236570605779E-15,1.,1.62630325872826E-15)) ;
#80504=DIRECTION('center_axis',(0.,1.,0.)) ;
#80505=DIRECTION('ref_axis',(1.,0.,0.)) ;
#80506=DIRECTION('center_axis',(1.,0.,-1.65429676464295E-16)) ;
#80507=DIRECTION('ref_axis',(1.65429676464295E-16,0.,1.)) ;
#80508=DIRECTION('center_axis',(0.,0.,-1.)) ;
#80509=DIRECTION('ref_axis',(-1.,0.,0.)) ;
#80510=DIRECTION('center_axis',(3.3085935292859E-16,0.,1.)) ;
#80511=DIRECTION('ref_axis',(1.,0.,-3.3085935292859E-16)) ;
#80512=DIRECTION('center_axis',(1.,0.,0.)) ;
#80513=DIRECTION('ref_axis',(0.,0.,-1.)) ;
#80514=DIRECTION('center_axis',(1.,1.21972744404619E-15,8.53809210832338E-16)) ;
#80515=DIRECTION('ref_axis',(-1.21972744404619E-15,1.,-2.84382165153726E-47)) ;
#80516=DIRECTION('center_axis',(0.,1.,0.)) ;
#80517=DIRECTION('ref_axis',(1.,0.,0.)) ;
#80518=DIRECTION('center_axis',(0.497468338163092,0.710669054518701,0.497468338163092)) ;
#80519=DIRECTION('ref_axis',(2.72143460710088E-15,0.573462344363328,-0.819231920519041)) ;
#80520=DIRECTION('center_axis',(-0.497468338163091,-0.710669054518702,-0.497468338163091)) ;
#80521=DIRECTION('ref_axis',(0.81923192051904,-0.573462344363328,7.6535433881835E-16)) ;
#80522=DIRECTION('center_axis',(-0.497468338163091,-0.710669054518702,-0.497468338163091)) ;
#80523=DIRECTION('ref_axis',(0.81923192051904,-0.573462344363328,7.6535433881835E-16)) ;
#80524=DIRECTION('center_axis',(0.,-1.,0.)) ;
#80525=DIRECTION('ref_axis',(0.,0.,-1.)) ;
#80526=DIRECTION('center_axis',(0.,1.,0.)) ;
#80527=DIRECTION('ref_axis',(0.,0.,-1.)) ;
#80528=DIRECTION('center_axis',(-8.67361737988403E-15,1.,0.)) ;
#80529=DIRECTION('ref_axis',(-1.,-8.67361737988403E-15,0.)) ;
#80530=DIRECTION('center_axis',(0.,0.,1.)) ;
#80531=DIRECTION('ref_axis',(1.,0.,0.)) ;
#80532=DIRECTION('center_axis',(1.,6.67201336914158E-17,0.)) ;
#80533=DIRECTION('ref_axis',(-6.67201336914158E-17,1.,0.)) ;
#80534=DIRECTION('center_axis',(-1.,-6.67201336914158E-17,0.)) ;
#80535=DIRECTION('ref_axis',(-6.67201336914158E-17,1.,0.)) ;
#80536=DIRECTION('center_axis',(-1.,1.33440267382831E-16,0.)) ;
#80537=DIRECTION('ref_axis',(-1.33440267382831E-16,-1.,0.)) ;
#80538=DIRECTION('center_axis',(-1.,1.33440267382831E-16,0.)) ;
#80539=DIRECTION('ref_axis',(-1.33440267382831E-16,-1.,0.)) ;
#80540=DIRECTION('center_axis',(0.710669054518702,0.497468338163091,0.497468338163091)) ;
#80541=DIRECTION('ref_axis',(-0.573462344363328,0.819231920519041,3.92980824865032E-16)) ;
#80542=DIRECTION('center_axis',(0.710669054518702,0.497468338163091,0.497468338163091)) ;
#80543=DIRECTION('ref_axis',(-0.573462344363328,0.819231920519041,3.92980824865032E-16)) ;
#80544=DIRECTION('center_axis',(0.710669054518701,0.497468338163091,0.497468338163092)) ;
#80545=DIRECTION('ref_axis',(0.573462344363329,2.49119655197717E-16,-0.81923192051904)) ;
#80546=DIRECTION('center_axis',(-0.710669054518702,0.497468338163091,-0.497468338163091)) ;
#80547=DIRECTION('ref_axis',(-0.573462344363328,-0.819231920519041,6.69271761853466E-16)) ;
#80548=DIRECTION('center_axis',(0.710669054518702,-0.497468338163091,0.497468338163091)) ;
#80549=DIRECTION('ref_axis',(-0.573462344363329,-0.81923192051904,1.7228593515426E-15)) ;
#80550=DIRECTION('center_axis',(0.7106690545187,-0.497468338163094,0.497468338163091)) ;
#80551=DIRECTION('ref_axis',(0.573462344363331,0.819231920519038,2.86772422505918E-16)) ;
#80552=DIRECTION('center_axis',(0.,1.,-9.34081871679819E-17)) ;
#80553=DIRECTION('ref_axis',(0.,9.34081871679819E-17,1.)) ;
#80554=DIRECTION('center_axis',(-4.33680868994205E-15,-1.,-3.03576608295944E-15)) ;
#80555=DIRECTION('ref_axis',(1.,-4.33680868994205E-15,-1.12103877145985E-44)) ;
#80556=DIRECTION('center_axis',(0.,1.,5.29374964685745E-15)) ;
#80557=DIRECTION('ref_axis',(0.,-5.29374964685745E-15,1.)) ;
#80558=DIRECTION('center_axis',(0.,1.,0.)) ;
#80559=DIRECTION('ref_axis',(1.,0.,0.)) ;
#80560=DIRECTION('center_axis',(0.,6.45175738210751E-15,1.)) ;
#80561=DIRECTION('ref_axis',(0.,1.,-6.45175738210751E-15)) ;
#80562=DIRECTION('center_axis',(-1.,-6.67201336914158E-17,0.)) ;
#80563=DIRECTION('ref_axis',(6.67201336914158E-17,-1.,0.)) ;
#80564=DIRECTION('center_axis',(-1.,-6.67201336914158E-17,0.)) ;
#80565=DIRECTION('ref_axis',(6.67201336914158E-17,-1.,0.)) ;
#80566=DIRECTION('center_axis',(1.,-1.33440267382831E-16,0.)) ;
#80567=DIRECTION('ref_axis',(1.33440267382831E-16,1.,0.)) ;
#80568=DIRECTION('center_axis',(-1.,1.33440267382831E-16,0.)) ;
#80569=DIRECTION('ref_axis',(1.33440267382831E-16,1.,0.)) ;
#80570=DIRECTION('center_axis',(0.,1.,0.)) ;
#80571=DIRECTION('ref_axis',(1.,0.,0.)) ;
#80572=DIRECTION('center_axis',(1.76182853028896E-15,-1.23327997120227E-15,
1.)) ;
#80573=DIRECTION('ref_axis',(-1.,7.2314321996121E-47,1.76182853028896E-15)) ;
#80574=DIRECTION('center_axis',(0.,0.,-1.)) ;
#80575=DIRECTION('ref_axis',(-1.,0.,0.)) ;
#80576=DIRECTION('center_axis',(-2.71050543121378E-16,-1.89735380184965E-16,
1.)) ;
#80577=DIRECTION('ref_axis',(1.,-2.13821176807699E-48,2.71050543121378E-16)) ;
#80578=DIRECTION('center_axis',(-0.710669054518702,-0.497468338163091,0.497468338163091)) ;
#80579=DIRECTION('ref_axis',(0.573462344363328,-0.819231920519041,3.92980824865032E-16)) ;
#80580=DIRECTION('center_axis',(0.710669054518702,0.497468338163091,-0.497468338163091)) ;
#80581=DIRECTION('ref_axis',(0.573462344363328,-0.819231920519041,3.92980824865032E-16)) ;
#80582=DIRECTION('center_axis',(0.710669054518701,0.497468338163091,-0.497468338163092)) ;
#80583=DIRECTION('ref_axis',(-0.573462344363329,-1.81914022221326E-16,-0.81923192051904)) ;
#80584=DIRECTION('center_axis',(0.710669054518702,-0.497468338163091,-0.497468338163091)) ;
#80585=DIRECTION('ref_axis',(0.573462344363328,0.819231920519041,6.69271761853466E-16)) ;
#80586=DIRECTION('center_axis',(0.710669054518702,-0.497468338163091,-0.497468338163091)) ;
#80587=DIRECTION('ref_axis',(0.573462344363328,0.819231920519041,6.69271761853466E-16)) ;
#80588=DIRECTION('center_axis',(0.7106690545187,-0.497468338163091,-0.497468338163093)) ;
#80589=DIRECTION('ref_axis',(-0.573462344363331,2.8326473018354E-16,-0.819231920519039)) ;
#80590=DIRECTION('center_axis',(0.,0.,-1.)) ;
#80591=DIRECTION('ref_axis',(-1.,0.,0.)) ;
#80592=DIRECTION('center_axis',(0.,1.15800773525007E-15,1.)) ;
#80593=DIRECTION('ref_axis',(0.,-1.,1.15800773525007E-15)) ;
#80594=DIRECTION('center_axis',(0.,1.,0.)) ;
#80595=DIRECTION('ref_axis',(1.,0.,0.)) ;
#80596=DIRECTION('center_axis',(0.,1.,0.)) ;
#80597=DIRECTION('ref_axis',(0.,0.,-1.)) ;
#80598=DIRECTION('center_axis',(0.,1.,0.)) ;
#80599=DIRECTION('ref_axis',(1.,0.,0.)) ;
#80600=DIRECTION('center_axis',(4.33680868994204E-15,-1.,-3.03576608295944E-15)) ;
#80601=DIRECTION('ref_axis',(-1.,-4.33680868994205E-15,4.47233396150273E-15)) ;
#80602=DIRECTION('center_axis',(0.,1.,9.34081871679819E-17)) ;
#80603=DIRECTION('ref_axis',(0.,-9.34081871679819E-17,1.)) ;
#80604=DIRECTION('center_axis',(0.,0.,1.)) ;
#80605=DIRECTION('ref_axis',(1.,0.,0.)) ;
#80606=DIRECTION('center_axis',(-2.16840434497102E-15,-3.61400724161847E-16,
1.)) ;
#80607=DIRECTION('ref_axis',(1.,1.51670488080685E-47,2.16840434497102E-15)) ;
#80608=DIRECTION('center_axis',(0.973328526784575,0.162221421130762,-0.162221421130763)) ;
#80609=DIRECTION('ref_axis',(-0.164398987305358,5.99282649549846E-16,-0.986393923832144)) ;
#80610=DIRECTION('center_axis',(0.973328526784574,0.162221421130765,-0.162221421130767)) ;
#80611=DIRECTION('ref_axis',(-0.164398987305362,8.41797083535674E-17,-0.986393923832143)) ;
#80612=DIRECTION('center_axis',(0.,1.,0.)) ;
#80613=DIRECTION('ref_axis',(1.,0.,0.)) ;
#80614=DIRECTION('center_axis',(0.,1.,-8.79325913341701E-15)) ;
#80615=DIRECTION('ref_axis',(0.,-8.79325913341701E-15,-1.)) ;
#80616=DIRECTION('center_axis',(0.,0.,1.)) ;
#80617=DIRECTION('ref_axis',(1.,0.,0.)) ;
#80618=DIRECTION('center_axis',(0.,-2.28569887277128E-15,1.)) ;
#80619=DIRECTION('ref_axis',(0.,-1.,-2.28569887277128E-15)) ;
#80620=DIRECTION('center_axis',(1.73472347597681E-15,-1.,-2.89120579329468E-16)) ;
#80621=DIRECTION('ref_axis',(1.,1.73472347597681E-15,5.01544256350843E-31)) ;
#80622=DIRECTION('center_axis',(8.67361737988409E-15,1.,-1.44560289664739E-15)) ;
#80623=DIRECTION('ref_axis',(-1.,8.67361737988409E-15,-1.40129846432482E-45)) ;
#80624=DIRECTION('center_axis',(0.,1.,0.)) ;
#80625=DIRECTION('ref_axis',(1.,0.,0.)) ;
#80626=DIRECTION('center_axis',(-0.937042571331634,0.312347523777217,0.156173761888611)) ;
#80627=DIRECTION('ref_axis',(0.316227766016843,0.948683298050512,6.71158276827649E-18)) ;
#80628=DIRECTION('center_axis',(0.937042571331636,-0.312347523777212,-0.156173761888606)) ;
#80629=DIRECTION('ref_axis',(0.316227766016838,0.948683298050514,8.61595672567599E-16)) ;
#80630=DIRECTION('center_axis',(-0.973328526784575,-0.162221421130762,-0.162221421130763)) ;
#80631=DIRECTION('ref_axis',(-0.164398987305358,5.99282649549846E-16,0.986393923832144)) ;
#80632=DIRECTION('center_axis',(0.978231976292118,-0.146734796047265,-0.146734795425574)) ;
#80633=DIRECTION('ref_axis',(0.182318633552554,0.945435290892317,0.270022270553542)) ;
#80634=DIRECTION('center_axis',(0.973328526784574,0.162221421130767,0.162221421130768)) ;
#80635=DIRECTION('ref_axis',(0.164398987305363,1.28476843531205E-16,-0.986393923832143)) ;
#80636=DIRECTION('center_axis',(0.,0.,1.)) ;
#80637=DIRECTION('ref_axis',(1.,0.,0.)) ;
#80638=DIRECTION('center_axis',(0.,2.19831478335425E-15,-1.)) ;
#80639=DIRECTION('ref_axis',(0.,1.,2.19831478335425E-15)) ;
#80640=DIRECTION('center_axis',(0.,1.,0.)) ;
#80641=DIRECTION('ref_axis',(1.,0.,0.)) ;
#80642=DIRECTION('center_axis',(8.67361737988408E-15,1.,1.44560289664739E-15)) ;
#80643=DIRECTION('ref_axis',(1.,-8.67361737988408E-15,5.60519385729927E-45)) ;
#80644=DIRECTION('center_axis',(1.73472347597681E-15,-1.,2.89120579329468E-16)) ;
#80645=DIRECTION('ref_axis',(1.,1.73472347597681E-15,-5.01544256350843E-31)) ;
#80646=DIRECTION('center_axis',(0.,1.,0.)) ;
#80647=DIRECTION('ref_axis',(0.,0.,1.)) ;
#80648=DIRECTION('center_axis',(0.,0.,1.)) ;
#80649=DIRECTION('ref_axis',(1.,0.,0.)) ;
#80650=DIRECTION('center_axis',(3.25260651745652E-15,-1.08420217248553E-15,
-1.)) ;
#80651=DIRECTION('ref_axis',(-1.,9.53266123289697E-45,-3.25260651745652E-15)) ;
#80652=DIRECTION('center_axis',(0.,1.,0.)) ;
#80653=DIRECTION('ref_axis',(1.,0.,0.)) ;
#80654=DIRECTION('center_axis',(-0.937042571331635,0.312347523777215,-0.15617376188861)) ;
#80655=DIRECTION('ref_axis',(0.316227766016841,0.948683298050513,6.5590042956861E-18)) ;
#80656=DIRECTION('center_axis',(-0.937042571331636,0.312347523777212,-0.156173761888606)) ;
#80657=DIRECTION('ref_axis',(0.331350514299571,0.654034959159569,-0.680033167478286)) ;
#80658=DIRECTION('center_axis',(0.961519724091138,0.245047216428683,-0.124224320904791)) ;
#80659=DIRECTION('ref_axis',(0.262092069891023,-0.682554728199521,0.682221950623634)) ;
#80660=DIRECTION('center_axis',(2.65552944032596E-32,3.29043518662928E-48,
-1.)) ;
#80661=DIRECTION('ref_axis',(-1.,1.31155984465371E-95,-2.65552944032596E-32)) ;
#80662=DIRECTION('center_axis',(2.65552944032596E-32,3.29043518662928E-48,
-1.)) ;
#80663=DIRECTION('ref_axis',(-1.,8.7378475095785E-80,-2.65552944032596E-32)) ;
#80664=DIRECTION('center_axis',(-2.65552944032596E-32,-3.29043518662928E-48,
1.)) ;
#80665=DIRECTION('ref_axis',(-1.,8.7378475095785E-80,-2.65552944032596E-32)) ;
#80666=DIRECTION('center_axis',(0.,0.,1.)) ;
#80667=DIRECTION('ref_axis',(1.,0.,0.)) ;
#80668=DIRECTION('center_axis',(0.,0.,-1.)) ;
#80669=DIRECTION('ref_axis',(-1.,0.,0.)) ;
#80670=DIRECTION('center_axis',(0.,0.,1.)) ;
#80671=DIRECTION('ref_axis',(1.,0.,0.)) ;
#80672=DIRECTION('center_axis',(0.,0.,1.)) ;
#80673=DIRECTION('ref_axis',(1.,0.,0.)) ;
#80674=DIRECTION('center_axis',(0.,0.,-1.)) ;
#80675=DIRECTION('ref_axis',(-1.,0.,0.)) ;
#80676=DIRECTION('center_axis',(0.,0.,-1.)) ;
#80677=DIRECTION('ref_axis',(-1.,0.,0.)) ;
#80678=DIRECTION('center_axis',(1.,1.15648231731787E-15,0.)) ;
#80679=DIRECTION('ref_axis',(1.03435541192675E-15,-1.,7.6571373978539E-16)) ;
#80680=DIRECTION('center_axis',(7.089177613099E-16,-0.612994899008946,-0.790086864711098)) ;
#80681=DIRECTION('ref_axis',(-4.46849810277083E-31,-0.790086864711098,0.612994899008946)) ;
#80682=DIRECTION('center_axis',(7.08917761309899E-16,-0.612994899008945,
0.790086864711098)) ;
#80683=DIRECTION('ref_axis',(-1.73472347597681E-14,0.790086864711098,0.612994899008945)) ;
#80684=DIRECTION('center_axis',(0.,0.,-1.)) ;
#80685=DIRECTION('ref_axis',(-1.,0.,0.)) ;
#80686=DIRECTION('center_axis',(0.,0.,1.)) ;
#80687=DIRECTION('ref_axis',(-1.,2.16840434497102E-15,0.)) ;
#80688=DIRECTION('center_axis',(1.08420217248551E-15,-1.,0.)) ;
#80689=DIRECTION('ref_axis',(1.,1.08420217248551E-15,0.)) ;
#80690=DIRECTION('center_axis',(1.44560289664734E-16,-1.,-2.4093381610789E-16)) ;
#80691=DIRECTION('ref_axis',(2.05395038580596E-47,2.4093381610789E-16,-1.)) ;
#80692=DIRECTION('center_axis',(0.,-1.,0.)) ;
#80693=DIRECTION('ref_axis',(0.,0.,-1.)) ;
#80694=DIRECTION('center_axis',(1.,0.,0.)) ;
#80695=DIRECTION('ref_axis',(0.,1.,0.)) ;
#80696=DIRECTION('center_axis',(1.,0.,0.)) ;
#80697=DIRECTION('ref_axis',(0.,0.,-1.)) ;
#80698=DIRECTION('center_axis',(1.,1.23908819712629E-16,8.95614743483648E-33)) ;
#80699=DIRECTION('ref_axis',(-1.23908819712629E-16,1.,-1.10974565782288E-48)) ;
#80700=DIRECTION('center_axis',(1.,0.,0.)) ;
#80701=DIRECTION('ref_axis',(0.,0.,-1.)) ;
#80702=DIRECTION('center_axis',(-1.,0.,0.)) ;
#80703=DIRECTION('ref_axis',(0.,0.,1.)) ;
#80704=DIRECTION('center_axis',(1.,1.23908819712629E-16,8.95614743483648E-33)) ;
#80705=DIRECTION('ref_axis',(-1.23908819712629E-16,1.,-1.10974565782288E-48)) ;
#80706=DIRECTION('center_axis',(-1.,0.,0.)) ;
#80707=DIRECTION('ref_axis',(0.,0.,1.)) ;
#80708=DIRECTION('center_axis',(1.,0.,0.)) ;
#80709=DIRECTION('ref_axis',(0.,-1.,0.)) ;
#80710=DIRECTION('center_axis',(0.,1.,0.)) ;
#80711=DIRECTION('ref_axis',(0.,0.,1.)) ;
#80712=DIRECTION('center_axis',(-1.44560289664734E-16,1.,-7.2280144832367E-17)) ;
#80713=DIRECTION('ref_axis',(0.707106781238322,1.5332934167208E-16,0.707106781134773)) ;
#80714=DIRECTION('center_axis',(-1.0842021724855E-15,1.,0.)) ;
#80715=DIRECTION('ref_axis',(-1.,-1.0842021724855E-15,0.)) ;
#80716=DIRECTION('center_axis',(0.,1.,0.)) ;
#80717=DIRECTION('ref_axis',(0.,0.,1.)) ;
#80718=DIRECTION('center_axis',(0.,-1.,0.)) ;
#80719=DIRECTION('ref_axis',(0.,0.,-1.)) ;
#80720=DIRECTION('center_axis',(0.,1.,0.)) ;
#80721=DIRECTION('ref_axis',(0.,0.,1.)) ;
#80722=DIRECTION('center_axis',(0.,0.,1.)) ;
#80723=DIRECTION('ref_axis',(1.,0.,0.)) ;
#80724=DIRECTION('center_axis',(0.431191646767813,0.0335421424156054,0.901636672080186)) ;
#80725=DIRECTION('ref_axis',(0.899826811311216,0.0573593277252533,-0.432459960190994)) ;
#80726=DIRECTION('center_axis',(0.,0.,1.)) ;
#80727=DIRECTION('ref_axis',(-1.,0.,0.)) ;
#80728=DIRECTION('center_axis',(0.,0.,-1.)) ;
#80729=DIRECTION('ref_axis',(0.707109343403322,-0.707104218960488,0.)) ;
#80730=DIRECTION('center_axis',(-3.25260651745653E-15,0.,1.)) ;
#80731=DIRECTION('ref_axis',(1.,0.,3.25260651745653E-15)) ;
#80732=DIRECTION('center_axis',(0.,0.,1.)) ;
#80733=DIRECTION('ref_axis',(1.,0.,0.)) ;
#80734=DIRECTION('center_axis',(0.431188264323706,0.0335835000991875,-0.901636750155293)) ;
#80735=DIRECTION('ref_axis',(0.899831768190665,0.0572892318879771,0.432458937778544)) ;
#80736=DIRECTION('center_axis',(0.,-1.,0.)) ;
#80737=DIRECTION('ref_axis',(0.,0.,-1.)) ;
#80738=DIRECTION('center_axis',(0.,1.,0.)) ;
#80739=DIRECTION('ref_axis',(0.,0.,1.)) ;
#80740=DIRECTION('center_axis',(0.,0.,1.)) ;
#80741=DIRECTION('ref_axis',(1.,0.,0.)) ;
#80742=DIRECTION('center_axis',(0.,0.,-1.)) ;
#80743=DIRECTION('ref_axis',(-1.,0.,0.)) ;
#80744=DIRECTION('center_axis',(0.,0.,1.)) ;
#80745=DIRECTION('ref_axis',(-0.986393923832144,0.164398987305354,0.)) ;
#80746=DIRECTION('center_axis',(0.98470178743927,-0.164116964573216,0.0585492250433781)) ;
#80747=DIRECTION('ref_axis',(0.164398987305362,0.986393923832143,-7.60669428566932E-17)) ;
#80748=DIRECTION('center_axis',(0.984834538781277,-0.164139089796902,0.0562075655416074)) ;
#80749=DIRECTION('ref_axis',(0.164398987305379,0.98639392383214,1.87706412796466E-17)) ;
#80750=DIRECTION('center_axis',(0.986393923832144,-0.129889480441767,0.100775740620418)) ;
#80751=DIRECTION('ref_axis',(0.,0.612994899008947,0.790086864711097)) ;
#80752=DIRECTION('center_axis',(0.,1.,0.)) ;
#80753=DIRECTION('ref_axis',(1.,0.,0.)) ;
#80754=DIRECTION('center_axis',(0.,0.,-1.)) ;
#80755=DIRECTION('ref_axis',(-1.,0.,0.)) ;
#80756=DIRECTION('center_axis',(1.,2.8359373108165E-15,0.)) ;
#80757=DIRECTION('ref_axis',(-2.8359373108165E-15,1.,0.)) ;
#80758=DIRECTION('center_axis',(0.,0.,-1.)) ;
#80759=DIRECTION('ref_axis',(-1.,0.,0.)) ;
#80760=DIRECTION('center_axis',(0.,0.,1.)) ;
#80761=DIRECTION('ref_axis',(1.,0.,0.)) ;
#80762=DIRECTION('center_axis',(1.,0.,0.)) ;
#80763=DIRECTION('ref_axis',(0.,0.,-1.)) ;
#80764=DIRECTION('center_axis',(1.,0.,0.)) ;
#80765=DIRECTION('ref_axis',(0.,0.,-1.)) ;
#80766=DIRECTION('center_axis',(0.,1.,0.)) ;
#80767=DIRECTION('ref_axis',(1.,0.,0.)) ;
#80768=DIRECTION('center_axis',(1.,-8.50781193244945E-15,0.)) ;
#80769=DIRECTION('ref_axis',(8.50781193244945E-15,1.,0.)) ;
#80770=DIRECTION('center_axis',(0.,1.,0.)) ;
#80771=DIRECTION('ref_axis',(1.,0.,0.)) ;
#80772=DIRECTION('center_axis',(-5.42101086242753E-16,1.70882313734897E-16,
1.)) ;
#80773=DIRECTION('ref_axis',(1.,9.53096053428495E-47,5.42101086242753E-16)) ;
#80774=DIRECTION('center_axis',(-1.,0.,0.)) ;
#80775=DIRECTION('ref_axis',(0.,0.,1.)) ;
#80776=DIRECTION('center_axis',(1.,0.,0.)) ;
#80777=DIRECTION('ref_axis',(0.,0.,-1.)) ;
#80778=DIRECTION('center_axis',(0.,0.,-1.)) ;
#80779=DIRECTION('ref_axis',(-1.,0.,0.)) ;
#80780=DIRECTION('center_axis',(0.,0.,1.)) ;
#80781=DIRECTION('ref_axis',(1.,0.,0.)) ;
#80782=DIRECTION('center_axis',(0.,1.,0.)) ;
#80783=DIRECTION('ref_axis',(1.,0.,0.)) ;
#80784=DIRECTION('center_axis',(0.,1.,0.)) ;
#80785=DIRECTION('ref_axis',(1.,0.,0.)) ;
#80786=DIRECTION('center_axis',(0.,0.,-1.)) ;
#80787=DIRECTION('ref_axis',(-1.,0.,0.)) ;
#80788=DIRECTION('center_axis',(0.,1.,0.)) ;
#80789=DIRECTION('ref_axis',(0.,0.,1.)) ;
#80790=DIRECTION('center_axis',(0.,0.,-1.)) ;
#80791=DIRECTION('ref_axis',(-1.,0.,0.)) ;
#80792=DIRECTION('center_axis',(0.,0.,1.)) ;
#80793=DIRECTION('ref_axis',(1.,0.,0.)) ;
#80794=DIRECTION('center_axis',(1.33440267382831E-16,1.,0.)) ;
#80795=DIRECTION('ref_axis',(-1.,1.33440267382831E-16,0.)) ;
#80796=DIRECTION('center_axis',(0.,1.,0.)) ;
#80797=DIRECTION('ref_axis',(0.,0.,1.)) ;
#80798=DIRECTION('center_axis',(0.,1.,0.)) ;
#80799=DIRECTION('ref_axis',(1.,0.,0.)) ;
#80800=DIRECTION('center_axis',(0.,1.,0.)) ;
#80801=DIRECTION('ref_axis',(0.,0.,1.)) ;
#80802=DIRECTION('center_axis',(0.,1.,0.)) ;
#80803=DIRECTION('ref_axis',(1.,0.,0.)) ;
#80804=DIRECTION('center_axis',(1.37797793267296E-15,-1.62630325872825E-15,
1.)) ;
#80805=DIRECTION('ref_axis',(0.,-1.,-1.62630325872825E-15)) ;
#80806=DIRECTION('center_axis',(-1.33440267382831E-16,-1.,0.)) ;
#80807=DIRECTION('ref_axis',(1.,-1.33440267382831E-16,0.)) ;
#80808=DIRECTION('center_axis',(0.,1.,0.)) ;
#80809=DIRECTION('ref_axis',(0.,0.,1.)) ;
#80810=DIRECTION('center_axis',(0.,0.,-1.)) ;
#80811=DIRECTION('ref_axis',(-1.,0.,0.)) ;
#80812=DIRECTION('center_axis',(0.,0.,1.)) ;
#80813=DIRECTION('ref_axis',(1.,0.,0.)) ;
#80814=DIRECTION('center_axis',(0.,1.,0.)) ;
#80815=DIRECTION('ref_axis',(1.,0.,0.)) ;
#80816=DIRECTION('center_axis',(0.,0.,1.)) ;
#80817=DIRECTION('ref_axis',(1.,0.,0.)) ;
#80818=DIRECTION('center_axis',(0.,0.,1.)) ;
#80819=DIRECTION('ref_axis',(1.,0.,0.)) ;
#80820=DIRECTION('center_axis',(0.,0.,1.)) ;
#80821=DIRECTION('ref_axis',(-0.986393923832144,0.164398987305354,0.)) ;
#80822=DIRECTION('center_axis',(0.984701787439272,-0.164116964573205,-0.0585492250433871)) ;
#80823=DIRECTION('ref_axis',(0.16439898730535,0.986393923832145,-3.2807868055655E-16)) ;
#80824=DIRECTION('center_axis',(0.984834538781259,-0.164139089796881,-0.0562075655419907)) ;
#80825=DIRECTION('ref_axis',(0.164398987305362,0.986393923832143,6.03508511856301E-17)) ;
#80826=DIRECTION('center_axis',(0.,0.,1.)) ;
#80827=DIRECTION('ref_axis',(-0.986393923832144,0.164398987305354,0.)) ;
#80828=DIRECTION('center_axis',(0.,0.,1.)) ;
#80829=DIRECTION('ref_axis',(1.,0.,0.)) ;
#80830=DIRECTION('center_axis',(0.342346838791424,0.100237737316009,-0.934211452502744)) ;
#80831=DIRECTION('ref_axis',(0.878411850255022,0.318727802445567,0.356097190777698)) ;
#80832=DIRECTION('center_axis',(0.,0.,-1.)) ;
#80833=DIRECTION('ref_axis',(-1.,0.,0.)) ;
#80834=DIRECTION('center_axis',(0.,0.,-1.)) ;
#80835=DIRECTION('ref_axis',(-1.,0.,0.)) ;
#80836=DIRECTION('center_axis',(0.,0.,-1.)) ;
#80837=DIRECTION('ref_axis',(-1.,0.,0.)) ;
#80838=DIRECTION('center_axis',(-0.342346838792776,-0.10023773732969,-0.93421145250078)) ;
#80839=DIRECTION('ref_axis',(0.87841177851845,0.318728005207571,-0.35609718625181)) ;
#80840=DIRECTION('center_axis',(0.,0.,1.)) ;
#80841=DIRECTION('ref_axis',(1.,0.,0.)) ;
#80842=DIRECTION('center_axis',(0.967224433277961,0.251696850864675,0.0335498276438615)) ;
#80843=DIRECTION('ref_axis',(0.148186136307302,-0.666803827414714,0.730351644587319)) ;
#80844=DIRECTION('center_axis',(0.,0.707106781186549,-0.707106781186547)) ;
#80845=DIRECTION('ref_axis',(0.,0.707106781186546,0.707106781186549)) ;
#80846=DIRECTION('center_axis',(0.978007532938632,-0.147978541149458,-0.146981688909092)) ;
#80847=DIRECTION('ref_axis',(0.193734423934244,0.383507624640146,0.902988856423898)) ;
#80848=DIRECTION('center_axis',(0.,0.447213595499958,0.894427190999916)) ;
#80849=DIRECTION('ref_axis',(0.,-0.894427190999916,0.447213595499958)) ;
#80850=DIRECTION('center_axis',(0.960001452008144,0.250435160947709,-0.125217579849438)) ;
#80851=DIRECTION('ref_axis',(0.276742394168032,-0.916645079798508,0.288401534238868)) ;
#80852=DIRECTION('center_axis',(0.,1.,0.)) ;
#80853=DIRECTION('ref_axis',(0.,0.,1.)) ;
#80854=DIRECTION('center_axis',(-1.,-1.19199144472199E-13,1.20231350744192E-12)) ;
#80855=DIRECTION('ref_axis',(-1.14382718901782E-12,0.413905147578545,-0.91032001450478)) ;
#80856=DIRECTION('center_axis',(1.,1.44560289664734E-16,0.)) ;
#80857=DIRECTION('ref_axis',(0.,1.,0.)) ;
#80858=DIRECTION('center_axis',(1.,1.44560289664734E-16,0.)) ;
#80859=DIRECTION('ref_axis',(-1.44560289664734E-16,1.,0.)) ;
#80860=DIRECTION('center_axis',(0.,0.,-1.)) ;
#80861=DIRECTION('ref_axis',(0.,-1.,0.)) ;
#80862=DIRECTION('center_axis',(-1.,-1.44560289664734E-16,0.)) ;
#80863=DIRECTION('ref_axis',(-1.44560289664734E-16,1.,0.)) ;
#80864=DIRECTION('center_axis',(1.,-3.46944695195361E-16,0.)) ;
#80865=DIRECTION('ref_axis',(2.61228946970625E-16,1.,0.)) ;
#80866=DIRECTION('center_axis',(1.,-3.46944695195361E-16,0.)) ;
#80867=DIRECTION('ref_axis',(3.46944695195361E-16,1.,0.)) ;
#80868=DIRECTION('center_axis',(0.,0.,1.)) ;
#80869=DIRECTION('ref_axis',(-3.26536183713281E-16,-1.,0.)) ;
#80870=DIRECTION('center_axis',(-1.,3.46944695195361E-16,0.)) ;
#80871=DIRECTION('ref_axis',(3.46944695195361E-16,1.,0.)) ;
#80872=DIRECTION('center_axis',(-1.,3.46944695195361E-16,0.)) ;
#80873=DIRECTION('ref_axis',(-3.46944695195361E-16,-1.,0.)) ;
#80874=DIRECTION('center_axis',(-1.,0.,0.)) ;
#80875=DIRECTION('ref_axis',(0.,0.,1.)) ;
#80876=DIRECTION('',(1.,-3.46944695195361E-16,0.)) ;
#80877=DIRECTION('center_axis',(-1.,8.01625584951926E-16,-1.08420217248551E-15)) ;
#80878=DIRECTION('ref_axis',(1.08420217248551E-15,2.168404344971E-15,-1.)) ;
#80879=DIRECTION('center_axis',(-1.,8.01625584951926E-16,-1.08420217248551E-15)) ;
#80880=DIRECTION('ref_axis',(1.08420217248551E-15,2.168404344971E-15,-1.)) ;
#80881=DIRECTION('',(-1.,3.46944695195361E-16,0.)) ;
#80882=DIRECTION('center_axis',(-1.,3.46944695195361E-16,0.)) ;
#80883=DIRECTION('ref_axis',(-3.46944695195361E-16,-1.,0.)) ;
#80884=DIRECTION('center_axis',(-1.,0.,0.)) ;
#80885=DIRECTION('ref_axis',(0.,0.,1.)) ;
#80886=DIRECTION('',(1.,-3.46944695195361E-16,0.)) ;
#80887=DIRECTION('center_axis',(-1.,2.2680138501079E-15,0.)) ;
#80888=DIRECTION('ref_axis',(2.2680138501079E-15,1.,0.)) ;
#80889=DIRECTION('',(-1.,3.46944695195361E-16,0.)) ;
#80890=DIRECTION('center_axis',(-1.,3.18032637262401E-16,0.)) ;
#80891=DIRECTION('ref_axis',(-5.55111512312578E-16,-1.,0.)) ;
#80892=DIRECTION('center_axis',(1.,-3.18032637262401E-16,0.)) ;
#80893=DIRECTION('ref_axis',(-3.18032637262401E-16,-1.,0.)) ;
#80894=DIRECTION('center_axis',(-2.01298417874256E-16,-0.632948931301568,
-0.774193548387096)) ;
#80895=DIRECTION('ref_axis',(1.73472347597681E-14,-0.774193548387096,0.632948931301568)) ;
#80896=DIRECTION('center_axis',(-1.,3.18032637262401E-16,0.)) ;
#80897=DIRECTION('ref_axis',(-3.18032637262401E-16,-1.,0.)) ;
#80898=DIRECTION('center_axis',(-2.01298417874256E-16,-0.632948931301568,
0.774193548387096)) ;
#80899=DIRECTION('ref_axis',(9.63584817660562E-32,-0.774193548387096,-0.632948931301568)) ;
#80900=DIRECTION('center_axis',(1.,1.44560289664734E-16,0.)) ;
#80901=DIRECTION('ref_axis',(-1.44560289664734E-16,1.,0.)) ;
#80902=DIRECTION('',(-1.,-1.44560289664734E-16,0.)) ;
#80903=DIRECTION('center_axis',(-1.,3.46944695195361E-16,0.)) ;
#80904=DIRECTION('ref_axis',(-3.46944695195361E-16,-1.,0.)) ;
#80905=DIRECTION('',(-1.,3.46944695195361E-16,0.)) ;
#80906=DIRECTION('center_axis',(-1.,3.46944695195361E-16,0.)) ;
#80907=DIRECTION('ref_axis',(3.46944695195361E-16,1.,3.46944695195361E-15)) ;
#80908=DIRECTION('center_axis',(-1.,3.46944695195361E-16,0.)) ;
#80909=DIRECTION('ref_axis',(3.46944695195361E-16,1.,0.)) ;
#80910=DIRECTION('center_axis',(-1.,3.46944695195361E-16,0.)) ;
#80911=DIRECTION('ref_axis',(-3.46944695195361E-16,-1.,0.)) ;
#80912=DIRECTION('',(1.,-3.46944695195361E-16,0.)) ;
#80913=DIRECTION('center_axis',(-1.,-1.44560289664734E-16,-2.65552944032596E-32)) ;
#80914=DIRECTION('ref_axis',(1.44560289664734E-16,-1.,-2.80018320648271E-64)) ;
#80915=DIRECTION('',(2.65552944032596E-32,3.29043518662928E-48,-1.)) ;
#80916=DIRECTION('',(1.44560289664734E-16,-1.,-2.4093381610789E-16)) ;
#80917=DIRECTION('',(0.,0.,1.)) ;
#80918=DIRECTION('center_axis',(0.999999956301289,0.000282786981237219,
8.61913163216796E-5)) ;
#80919=DIRECTION('ref_axis',(0.000288266391068138,-0.99739627340708,-0.0721151211339053)) ;
#80920=DIRECTION('',(-1.44560289664734E-16,1.,-7.2280144832367E-17)) ;
#80921=DIRECTION('center_axis',(0.316227766016838,0.948683298050514,0.)) ;
#80922=DIRECTION('ref_axis',(-0.948683298050514,0.316227766016838,0.)) ;
#80923=DIRECTION('',(-0.948683298050514,0.316227766016838,0.)) ;
#80924=DIRECTION('',(0.,0.,1.)) ;
#80925=DIRECTION('',(0.937042571331636,-0.312347523777212,-0.156173761888606)) ;
#80926=DIRECTION('',(0.,0.,-1.)) ;
#80927=DIRECTION('center_axis',(1.,1.73472347597681E-15,0.)) ;
#80928=DIRECTION('ref_axis',(-1.73472347597681E-15,1.,0.)) ;
#80929=DIRECTION('',(-1.73472347597681E-15,1.,0.)) ;
#80930=DIRECTION('',(0.,0.,1.)) ;
#80931=DIRECTION('',(1.73472347597681E-15,-1.,-2.89120579329468E-16)) ;
#80932=DIRECTION('',(0.,0.,-1.)) ;
#80933=DIRECTION('center_axis',(0.164398987305357,-0.986393923832144,0.)) ;
#80934=DIRECTION('ref_axis',(0.986393923832144,0.164398987305357,0.)) ;
#80935=DIRECTION('',(-0.973328526784575,-0.162221421130762,0.162221421130763)) ;
#80936=DIRECTION('',(0.,0.,-1.)) ;
#80937=DIRECTION('',(0.986393923832144,0.164398987305357,0.)) ;
#80938=DIRECTION('',(0.,0.,1.)) ;
#80939=DIRECTION('center_axis',(-9.91270557701033E-17,1.,0.)) ;
#80940=DIRECTION('ref_axis',(-1.,-9.91270557701033E-17,0.)) ;
#80941=DIRECTION('',(1.,9.91270557701033E-17,0.)) ;
#80942=DIRECTION('',(0.,0.,-1.)) ;
#80943=DIRECTION('',(-1.,-9.91270557701033E-17,0.)) ;
#80944=DIRECTION('',(0.,0.,1.)) ;
#80945=DIRECTION('center_axis',(-9.91270557701033E-17,1.,0.)) ;
#80946=DIRECTION('ref_axis',(-1.,-9.91270557701033E-17,0.)) ;
#80947=DIRECTION('',(-1.,-9.91270557701033E-17,0.)) ;
#80948=DIRECTION('',(0.,0.,-1.)) ;
#80949=DIRECTION('',(-1.,-9.91270557701033E-17,0.)) ;
#80950=DIRECTION('',(0.,0.,1.)) ;
#80951=DIRECTION('center_axis',(1.,1.15648231731787E-15,0.)) ;
#80952=DIRECTION('ref_axis',(-1.15648231731787E-15,1.,0.)) ;
#80953=DIRECTION('',(-1.15648231731787E-15,1.,0.)) ;
#80954=DIRECTION('',(0.,0.,-1.)) ;
#80955=DIRECTION('',(-1.15648231731787E-15,1.,0.)) ;
#80956=DIRECTION('',(0.,0.,1.)) ;
#80957=DIRECTION('center_axis',(-1.,-1.15648231731787E-15,0.)) ;
#80958=DIRECTION('ref_axis',(-1.15648231731787E-15,1.,1.82070621850777E-15)) ;
#80959=DIRECTION('',(0.,0.,1.)) ;
#80960=DIRECTION('center_axis',(0.,0.,1.)) ;
#80961=DIRECTION('ref_axis',(1.,0.,0.)) ;
#80962=DIRECTION('',(-1.,0.,0.)) ;
#80963=DIRECTION('center_axis',(0.,0.,-1.)) ;
#80964=DIRECTION('ref_axis',(1.,0.,0.)) ;
#80965=DIRECTION('center_axis',(0.,0.,-1.)) ;
#80966=DIRECTION('ref_axis',(1.,0.,0.)) ;
#80967=DIRECTION('center_axis',(0.,0.,-1.)) ;
#80968=DIRECTION('ref_axis',(1.,0.,0.)) ;
#80969=DIRECTION('center_axis',(0.,0.,-1.)) ;
#80970=DIRECTION('ref_axis',(1.,0.,0.)) ;
#80971=DIRECTION('',(1.,0.,0.)) ;
#80972=DIRECTION('center_axis',(0.,0.,1.)) ;
#80973=DIRECTION('ref_axis',(1.,0.,0.)) ;
#80974=DIRECTION('',(3.46944695195361E-16,1.,0.)) ;
#80975=DIRECTION('center_axis',(0.,0.,1.)) ;
#80976=DIRECTION('ref_axis',(1.,0.,0.)) ;
#80977=DIRECTION('',(1.,-3.46944695195361E-16,0.)) ;
#80978=DIRECTION('center_axis',(0.,0.,-1.)) ;
#80979=DIRECTION('ref_axis',(1.,0.,0.)) ;
#80980=DIRECTION('',(2.71050543121376E-16,1.,0.)) ;
#80981=DIRECTION('center_axis',(0.,0.,-1.)) ;
#80982=DIRECTION('ref_axis',(1.,0.,0.)) ;
#80983=DIRECTION('',(-1.,3.46944695195361E-16,0.)) ;
#80984=DIRECTION('center_axis',(0.,0.,1.)) ;
#80985=DIRECTION('ref_axis',(1.,0.,0.)) ;
#80986=DIRECTION('',(3.46944695195361E-16,1.,0.)) ;
#80987=DIRECTION('center_axis',(0.,0.,1.)) ;
#80988=DIRECTION('ref_axis',(1.,0.,0.)) ;
#80989=DIRECTION('center_axis',(0.,0.,-1.)) ;
#80990=DIRECTION('ref_axis',(1.,0.,0.)) ;
#80991=DIRECTION('',(0.986393923832144,-0.164398987305354,0.)) ;
#80992=DIRECTION('center_axis',(0.,0.,-1.)) ;
#80993=DIRECTION('ref_axis',(1.,-6.50521303491307E-15,0.)) ;
#80994=DIRECTION('center_axis',(0.,0.,-1.)) ;
#80995=DIRECTION('ref_axis',(1.,0.,0.)) ;
#80996=DIRECTION('',(1.,0.,0.)) ;
#80997=DIRECTION('',(1.13380619344889E-16,-1.,0.)) ;
#80998=DIRECTION('center_axis',(0.,0.,-1.)) ;
#80999=DIRECTION('ref_axis',(1.,0.,0.)) ;
#81000=DIRECTION('',(-1.,-1.92747052886312E-16,0.)) ;
#81001=DIRECTION('center_axis',(0.,0.,1.)) ;
#81002=DIRECTION('ref_axis',(1.,0.,0.)) ;
#81003=DIRECTION('',(0.,-1.,0.)) ;
#81004=DIRECTION('center_axis',(0.,0.,-1.)) ;
#81005=DIRECTION('ref_axis',(1.,0.,0.)) ;
#81006=DIRECTION('center_axis',(0.,0.,1.)) ;
#81007=DIRECTION('ref_axis',(1.,0.,0.)) ;
#81008=DIRECTION('',(-0.948683298050514,0.316227766016838,0.)) ;
#81009=DIRECTION('center_axis',(0.,0.,1.)) ;
#81010=DIRECTION('ref_axis',(1.,0.,0.)) ;
#81011=DIRECTION('',(-1.,0.,0.)) ;
#81012=DIRECTION('center_axis',(0.,0.,1.)) ;
#81013=DIRECTION('ref_axis',(1.,0.,0.)) ;
#81014=DIRECTION('',(0.,-1.,0.)) ;
#81015=DIRECTION('center_axis',(0.,0.,-1.)) ;
#81016=DIRECTION('ref_axis',(1.,0.,0.)) ;
#81017=DIRECTION('',(-1.,-1.92747052886312E-16,0.)) ;
#81018=DIRECTION('center_axis',(0.,0.,1.)) ;
#81019=DIRECTION('ref_axis',(1.,0.,0.)) ;
#81020=DIRECTION('',(1.13380619344889E-16,-1.,0.)) ;
#81021=DIRECTION('',(1.,0.,0.)) ;
#81022=DIRECTION('center_axis',(0.,0.,1.)) ;
#81023=DIRECTION('ref_axis',(1.,0.,0.)) ;
#81024=DIRECTION('center_axis',(0.,0.,1.)) ;
#81025=DIRECTION('ref_axis',(1.,0.,0.)) ;
#81026=DIRECTION('',(-0.986393923832144,0.164398987305354,0.)) ;
#81027=DIRECTION('center_axis',(0.,0.,1.)) ;
#81028=DIRECTION('ref_axis',(1.,0.,0.)) ;
#81029=DIRECTION('center_axis',(0.,0.,-1.)) ;
#81030=DIRECTION('ref_axis',(1.,0.,0.)) ;
#81031=DIRECTION('',(-3.46944695195361E-16,-1.,0.)) ;
#81032=DIRECTION('center_axis',(0.,0.,-1.)) ;
#81033=DIRECTION('ref_axis',(1.,0.,0.)) ;
#81034=DIRECTION('',(-1.,3.46944695195361E-16,0.)) ;
#81035=DIRECTION('center_axis',(0.,0.,1.)) ;
#81036=DIRECTION('ref_axis',(1.,0.,0.)) ;
#81037=DIRECTION('',(3.46944695195361E-16,1.,0.)) ;
#81038=DIRECTION('center_axis',(0.,0.,1.)) ;
#81039=DIRECTION('ref_axis',(1.,0.,0.)) ;
#81040=DIRECTION('',(1.,-3.46944695195361E-16,0.)) ;
#81041=DIRECTION('center_axis',(0.,0.,-1.)) ;
#81042=DIRECTION('ref_axis',(1.,0.,0.)) ;
#81043=DIRECTION('',(-3.46944695195361E-16,-1.,0.)) ;
#81044=DIRECTION('center_axis',(0.,0.,-1.)) ;
#81045=DIRECTION('ref_axis',(1.,0.,0.)) ;
#81046=DIRECTION('',(1.,0.,0.)) ;
#81047=DIRECTION('center_axis',(0.,0.,1.)) ;
#81048=DIRECTION('ref_axis',(1.,0.,0.)) ;
#81049=DIRECTION('',(0.986393923832144,0.164398987305357,0.)) ;
#81050=DIRECTION('center_axis',(0.,0.,1.)) ;
#81051=DIRECTION('ref_axis',(1.,0.,0.)) ;
#81052=DIRECTION('',(-1.73472347597681E-15,1.,0.)) ;
#81053=DIRECTION('center_axis',(0.,0.,1.)) ;
#81054=DIRECTION('ref_axis',(1.,0.,0.)) ;
#81055=DIRECTION('center_axis',(-1.92747052886312E-16,1.,0.)) ;
#81056=DIRECTION('ref_axis',(-1.,-1.92747052886312E-16,0.)) ;
#81057=DIRECTION('',(0.,0.,1.)) ;
#81058=DIRECTION('',(0.,0.,-1.)) ;
#81059=DIRECTION('center_axis',(-1.,0.,0.)) ;
#81060=DIRECTION('ref_axis',(0.,0.,1.)) ;
#81061=DIRECTION('',(0.,0.,1.)) ;
#81062=DIRECTION('',(0.,0.,-1.)) ;
#81063=DIRECTION('center_axis',(0.,1.,0.)) ;
#81064=DIRECTION('ref_axis',(0.,0.,1.)) ;
#81065=DIRECTION('',(0.,0.,-1.)) ;
#81066=DIRECTION('',(0.,0.,1.)) ;
#81067=DIRECTION('',(0.,0.,-1.)) ;
#81068=DIRECTION('',(0.,0.,-1.)) ;
#81069=DIRECTION('center_axis',(0.316227766016838,0.948683298050514,0.)) ;
#81070=DIRECTION('ref_axis',(-0.948683298050514,0.316227766016838,0.)) ;
#81071=DIRECTION('center_axis',(-0.316227766016878,-0.9486832980505,-8.70066748967434E-14)) ;
#81072=DIRECTION('ref_axis',(0.831595960760918,-0.277198653586968,-0.481257794218128)) ;
#81073=DIRECTION('',(0.,0.,1.)) ;
#81074=DIRECTION('',(0.,0.,-1.)) ;
#81075=DIRECTION('',(-0.937042571331636,0.312347523777212,-0.156173761888606)) ;
#81076=DIRECTION('center_axis',(1.,1.73472347597681E-15,0.)) ;
#81077=DIRECTION('ref_axis',(-1.73472347597681E-15,1.,0.)) ;
#81078=DIRECTION('',(-1.73472347597681E-15,1.,-2.89120579329468E-16)) ;
#81079=DIRECTION('',(0.,0.,1.)) ;
#81080=DIRECTION('',(0.,0.,-1.)) ;
#81081=DIRECTION('center_axis',(0.164398987305357,-0.986393923832144,0.)) ;
#81082=DIRECTION('ref_axis',(0.986393923832144,0.164398987305357,0.)) ;
#81083=DIRECTION('',(0.973328526784575,0.162221421130762,0.162221421130763)) ;
#81084=DIRECTION('',(0.,0.,1.)) ;
#81085=DIRECTION('',(0.,0.,-1.)) ;
#81086=DIRECTION('center_axis',(0.,-1.,0.)) ;
#81087=DIRECTION('ref_axis',(0.,0.,-1.)) ;
#81088=DIRECTION('',(0.,0.,1.)) ;
#81089=DIRECTION('',(0.,0.,1.)) ;
#81090=DIRECTION('',(0.,0.,1.)) ;
#81091=DIRECTION('',(0.,0.,-1.)) ;
#81092=DIRECTION('',(1.,0.,2.25271179641597E-31)) ;
#81093=DIRECTION('center_axis',(0.,-1.,0.)) ;
#81094=DIRECTION('ref_axis',(0.,0.,-1.)) ;
#81095=DIRECTION('',(0.,0.,-1.)) ;
#81096=DIRECTION('center_axis',(0.,-1.,0.)) ;
#81097=DIRECTION('ref_axis',(0.,0.,-1.)) ;
#81098=DIRECTION('',(-1.,0.,-3.21815970916568E-32)) ;
#81099=DIRECTION('',(0.,0.,-1.)) ;
#81100=DIRECTION('center_axis',(1.,-3.46944695195361E-16,0.)) ;
#81101=DIRECTION('ref_axis',(3.46944695195361E-16,1.,0.)) ;
#81102=DIRECTION('center_axis',(1.,-3.46944695195361E-16,0.)) ;
#81103=DIRECTION('ref_axis',(3.46944695195361E-16,1.,0.)) ;
#81104=DIRECTION('',(1.5529910948782E-31,4.47619207437002E-16,-1.)) ;
#81105=DIRECTION('',(0.,0.,1.)) ;
#81106=DIRECTION('center_axis',(1.,-3.46944695195361E-16,0.)) ;
#81107=DIRECTION('ref_axis',(3.46944695195361E-16,1.,0.)) ;
#81108=DIRECTION('center_axis',(1.,-3.46944695195361E-16,0.)) ;
#81109=DIRECTION('ref_axis',(3.46944695195361E-16,1.,0.)) ;
#81110=DIRECTION('center_axis',(1.,-3.46944695195361E-16,0.)) ;
#81111=DIRECTION('ref_axis',(3.46944695195361E-16,1.,0.)) ;
#81112=DIRECTION('',(3.46944695195361E-16,1.,9.27571383489107E-17)) ;
#81113=DIRECTION('',(0.,0.,1.)) ;
#81114=DIRECTION('',(-3.46944695195361E-16,-1.,-6.49299968442375E-16)) ;
#81115=DIRECTION('center_axis',(1.,-3.46944695195361E-16,0.)) ;
#81116=DIRECTION('ref_axis',(3.46944695195361E-16,1.,0.)) ;
#81117=DIRECTION('center_axis',(1.,-3.46944695195361E-16,0.)) ;
#81118=DIRECTION('ref_axis',(3.46944695195361E-16,1.,0.)) ;
#81119=DIRECTION('center_axis',(1.,-3.46944695195361E-16,0.)) ;
#81120=DIRECTION('ref_axis',(3.46944695195361E-16,1.,0.)) ;
#81121=DIRECTION('',(0.,0.,1.)) ;
#81122=DIRECTION('',(-1.5529910948782E-31,-4.47619207437002E-16,-1.)) ;
#81123=DIRECTION('center_axis',(1.,-3.46944695195361E-16,0.)) ;
#81124=DIRECTION('ref_axis',(3.46944695195361E-16,1.,0.)) ;
#81125=DIRECTION('center_axis',(1.,-3.46944695195361E-16,0.)) ;
#81126=DIRECTION('ref_axis',(3.46944695195361E-16,1.,0.)) ;
#81127=DIRECTION('center_axis',(1.,-3.46944695195361E-16,0.)) ;
#81128=DIRECTION('ref_axis',(3.46944695195361E-16,1.,0.)) ;
#81129=DIRECTION('',(-3.46944695195361E-16,-1.,-1.06487173641454E-15)) ;
#81130=DIRECTION('center_axis',(1.,-3.46944695195361E-16,0.)) ;
#81131=DIRECTION('ref_axis',(3.46944695195361E-16,1.,0.)) ;
#81132=DIRECTION('',(3.46944695195361E-16,1.,2.45739631480277E-16)) ;
#81133=DIRECTION('center_axis',(1.,-3.46944695195361E-16,0.)) ;
#81134=DIRECTION('ref_axis',(3.46944695195361E-16,1.,0.)) ;
#81135=DIRECTION('center_axis',(1.,-3.46944695195361E-16,0.)) ;
#81136=DIRECTION('ref_axis',(3.46944695195361E-16,1.,0.)) ;
#81137=DIRECTION('center_axis',(0.,-1.,0.)) ;
#81138=DIRECTION('ref_axis',(0.,0.,-1.)) ;
#81139=DIRECTION('center_axis',(0.,-1.,0.)) ;
#81140=DIRECTION('ref_axis',(0.,0.,-1.)) ;
#81141=DIRECTION('',(-1.,0.,-1.40488587213121E-32)) ;
#81142=DIRECTION('',(0.,0.,1.)) ;
#81143=DIRECTION('',(0.,0.,1.)) ;
#81144=DIRECTION('',(0.,0.,1.)) ;
#81145=DIRECTION('',(1.,0.,1.40488587213121E-32)) ;
#81146=DIRECTION('center_axis',(0.,-1.,0.)) ;
#81147=DIRECTION('ref_axis',(0.,0.,-1.)) ;
#81148=DIRECTION('',(7.2280144832367E-17,0.,-1.)) ;
#81149=DIRECTION('center_axis',(-1.,-1.13380619344889E-16,0.)) ;
#81150=DIRECTION('ref_axis',(1.13380619344889E-16,-1.,0.)) ;
#81151=DIRECTION('center_axis',(-1.,-1.13380619344889E-16,0.)) ;
#81152=DIRECTION('ref_axis',(1.13380619344889E-16,-1.,0.)) ;
#81153=DIRECTION('',(1.13380619344889E-16,-1.,1.23908819712629E-16)) ;
#81154=DIRECTION('',(0.,0.,-1.)) ;
#81155=DIRECTION('',(-1.13380619344889E-16,1.,-1.23908819712629E-16)) ;
#81156=DIRECTION('center_axis',(-1.,-1.13380619344889E-16,0.)) ;
#81157=DIRECTION('ref_axis',(1.13380619344889E-16,-1.,0.)) ;
#81158=DIRECTION('',(0.,0.,1.)) ;
#81159=DIRECTION('center_axis',(-1.40488587213121E-32,1.23908819712629E-16,
1.)) ;
#81160=DIRECTION('ref_axis',(0.,-1.,1.23908819712629E-16)) ;
#81161=DIRECTION('',(-1.,0.,-1.40488587213121E-32)) ;
#81162=DIRECTION('',(-1.13380619344889E-16,1.,-1.23908819712629E-16)) ;
#81163=DIRECTION('center_axis',(1.40488587213121E-32,-1.23908819712629E-16,
-1.)) ;
#81164=DIRECTION('ref_axis',(-1.74077750246726E-48,-1.,1.23908819712629E-16)) ;
#81165=DIRECTION('center_axis',(1.40488587213121E-32,-1.23908819712629E-16,
-1.)) ;
#81166=DIRECTION('ref_axis',(0.,1.,-1.23908819712629E-16)) ;
#81167=DIRECTION('center_axis',(-1.40488587213121E-32,1.23908819712629E-16,
1.)) ;
#81168=DIRECTION('ref_axis',(1.74077750246726E-48,1.,-1.23908819712629E-16)) ;
#81169=DIRECTION('',(1.13380619344889E-16,-1.,1.23908819712629E-16)) ;
#81170=DIRECTION('',(1.,0.,1.40488587213121E-32)) ;
#81171=DIRECTION('center_axis',(-1.,-1.23908819712629E-16,-8.95614743483648E-33)) ;
#81172=DIRECTION('ref_axis',(1.23908819712629E-16,-1.,5.38566640001825E-66)) ;
#81173=DIRECTION('',(-8.95614743483648E-33,-1.10974565782288E-48,1.)) ;
#81174=DIRECTION('',(1.23908819712629E-16,-1.,7.2280144832367E-17)) ;
#81175=DIRECTION('',(-8.95614743483648E-33,0.,1.)) ;
#81176=DIRECTION('',(-1.23908819712629E-16,1.,-1.23908819712629E-16)) ;
#81177=DIRECTION('',(8.95614743483648E-33,1.0154535431059E-48,-1.)) ;
#81178=DIRECTION('',(1.23908819712629E-16,-1.,1.23908819712629E-16)) ;
#81179=DIRECTION('',(-8.95614743483648E-33,0.,1.)) ;
#81180=DIRECTION('',(-1.23908819712629E-16,1.,2.4093381610789E-16)) ;
#81181=DIRECTION('center_axis',(-1.7912294869673E-32,7.2280144832367E-17,
1.)) ;
#81182=DIRECTION('ref_axis',(0.,-1.,7.2280144832367E-17)) ;
#81183=DIRECTION('',(-1.23908819712629E-16,1.,-7.2280144832367E-17)) ;
#81184=DIRECTION('',(1.,1.23908819712629E-16,8.95614743483648E-33)) ;
#81185=DIRECTION('',(1.44560289664734E-16,-1.,7.2280144832367E-17)) ;
#81186=DIRECTION('',(-1.,0.,-1.7912294869673E-32)) ;
#81187=DIRECTION('center_axis',(-2.08976773479518E-32,2.4093381610789E-16,
-1.)) ;
#81188=DIRECTION('ref_axis',(0.,1.,2.4093381610789E-16)) ;
#81189=DIRECTION('',(-1.44560289664734E-16,1.,2.4093381610789E-16)) ;
#81190=DIRECTION('',(-1.,-1.23908819712629E-16,-8.95614743483648E-33)) ;
#81191=DIRECTION('',(1.23908819712629E-16,-1.,-2.4093381610789E-16)) ;
#81192=DIRECTION('',(1.,0.,-2.08976773479518E-32)) ;
#81193=DIRECTION('center_axis',(-1.23908819712629E-16,1.,0.)) ;
#81194=DIRECTION('ref_axis',(-1.,-1.23908819712629E-16,0.)) ;
#81195=DIRECTION('',(8.95614743483648E-33,1.10974565782288E-48,-1.)) ;
#81196=DIRECTION('',(1.,1.23908819712629E-16,8.95614743483648E-33)) ;
#81197=DIRECTION('',(-2.65552944032596E-32,-3.29043518662928E-48,1.)) ;
#81198=DIRECTION('',(-1.,-1.23908819712629E-16,-8.95614743483648E-33)) ;
#81199=DIRECTION('center_axis',(-1.,-1.44560289664734E-16,-2.65552944032596E-32)) ;
#81200=DIRECTION('ref_axis',(1.44560289664734E-16,-1.,-2.80018320648271E-64)) ;
#81201=DIRECTION('',(1.44560289664734E-16,-1.,-2.4093381610789E-16)) ;
#81202=DIRECTION('',(-2.65552944032596E-32,0.,1.)) ;
#81203=DIRECTION('',(-1.44560289664734E-16,1.,-7.2280144832367E-17)) ;
#81204=DIRECTION('',(0.,0.,-1.)) ;
#81205=DIRECTION('center_axis',(0.,1.,0.)) ;
#81206=DIRECTION('ref_axis',(0.,0.,1.)) ;
#81207=DIRECTION('',(8.95614743483648E-33,0.,-1.)) ;
#81208=DIRECTION('',(1.,0.,1.40488587213121E-32)) ;
#81209=DIRECTION('',(-7.2280144832367E-17,0.,1.)) ;
#81210=DIRECTION('',(-1.,0.,-1.40488587213121E-32)) ;
#81211=DIRECTION('',(8.95614743483648E-33,0.,-1.)) ;
#81212=DIRECTION('',(1.,0.,1.7912294869673E-32)) ;
#81213=DIRECTION('',(2.65552944032596E-32,0.,-1.)) ;
#81214=DIRECTION('',(-1.,0.,2.08976773479518E-32)) ;
#81215=DIRECTION('center_axis',(1.,1.44560289664734E-16,0.)) ;
#81216=DIRECTION('ref_axis',(-1.44560289664734E-16,1.,0.)) ;
#81217=DIRECTION('',(1.44560289664734E-16,-1.,0.)) ;
#81218=DIRECTION('center_axis',(-1.,-1.44560289664734E-16,0.)) ;
#81219=DIRECTION('ref_axis',(-1.44560289664734E-16,1.,0.)) ;
#81220=DIRECTION('',(0.,0.,-1.)) ;
#81221=DIRECTION('center_axis',(-1.,-1.44560289664734E-16,0.)) ;
#81222=DIRECTION('ref_axis',(-1.44560289664734E-16,1.,0.)) ;
#81223=DIRECTION('',(1.44560289664734E-16,-1.,0.)) ;
#81224=DIRECTION('center_axis',(-1.,-1.44560289664734E-16,0.)) ;
#81225=DIRECTION('ref_axis',(-1.44560289664734E-16,1.,0.)) ;
#81226=DIRECTION('',(0.,0.,1.)) ;
#81227=DIRECTION('center_axis',(-1.,-1.44560289664734E-16,0.)) ;
#81228=DIRECTION('ref_axis',(-1.44560289664734E-16,1.,0.)) ;
#81229=DIRECTION('center_axis',(1.,-3.46944695195361E-16,0.)) ;
#81230=DIRECTION('ref_axis',(3.46944695195361E-16,1.,0.)) ;
#81231=DIRECTION('center_axis',(1.,-3.46944695195361E-16,0.)) ;
#81232=DIRECTION('ref_axis',(3.46944695195361E-16,1.,0.)) ;
#81233=DIRECTION('',(0.,0.,-1.)) ;
#81234=DIRECTION('',(-1.5529910948782E-31,-4.47619207437002E-16,1.)) ;
#81235=DIRECTION('center_axis',(-1.,3.46944695195361E-16,0.)) ;
#81236=DIRECTION('ref_axis',(3.46944695195361E-16,1.,1.87537673078574E-15)) ;
#81237=DIRECTION('',(-3.46944695195361E-16,-1.,-2.45739631480277E-16)) ;
#81238=DIRECTION('center_axis',(1.,-3.46944695195361E-16,0.)) ;
#81239=DIRECTION('ref_axis',(3.46944695195361E-16,1.,0.)) ;
#81240=DIRECTION('center_axis',(3.46944695195361E-16,1.,4.47619207437002E-16)) ;
#81241=DIRECTION('ref_axis',(-8.18685017503995E-48,-4.47619207437002E-16,
1.)) ;
#81242=DIRECTION('',(-1.5529910948782E-31,-4.47619207437002E-16,1.)) ;
#81243=DIRECTION('',(-1.,3.46944695195361E-16,0.)) ;
#81244=DIRECTION('',(1.5529910948782E-31,4.47619207437002E-16,-1.)) ;
#81245=DIRECTION('center_axis',(-8.52580615413453E-32,-2.45739631480277E-16,
1.)) ;
#81246=DIRECTION('ref_axis',(0.,-1.,-2.45739631480277E-16)) ;
#81247=DIRECTION('',(1.,-3.46944695195361E-16,0.)) ;
#81248=DIRECTION('',(-3.46944695195361E-16,-1.,-2.45739631480277E-16)) ;
#81249=DIRECTION('',(3.46944695195361E-16,1.,2.45739631480277E-16)) ;
#81250=DIRECTION('center_axis',(1.,-3.46944695195361E-16,0.)) ;
#81251=DIRECTION('ref_axis',(3.46944695195361E-16,1.,0.)) ;
#81252=DIRECTION('center_axis',(1.,-3.46944695195361E-16,0.)) ;
#81253=DIRECTION('ref_axis',(3.46944695195361E-16,1.,0.)) ;
#81254=DIRECTION('',(1.,-3.46944695195361E-16,0.)) ;
#81255=DIRECTION('center_axis',(-1.,3.46944695195361E-16,0.)) ;
#81256=DIRECTION('ref_axis',(3.46944695195361E-16,1.,0.)) ;
#81257=DIRECTION('',(-1.,3.46944695195361E-16,0.)) ;
#81258=DIRECTION('center_axis',(1.,-3.46944695195361E-16,0.)) ;
#81259=DIRECTION('ref_axis',(3.46944695195361E-16,1.,0.)) ;
#81260=DIRECTION('center_axis',(1.,-3.46944695195361E-16,0.)) ;
#81261=DIRECTION('ref_axis',(-3.46944695195361E-16,-1.,-5.45198806735568E-15)) ;
#81262=DIRECTION('',(1.,-3.46944695195361E-16,0.)) ;
#81263=DIRECTION('center_axis',(-1.,3.46944695195361E-16,0.)) ;
#81264=DIRECTION('ref_axis',(3.46944695195361E-16,1.,-2.47817639425258E-15)) ;
#81265=DIRECTION('',(-1.,3.46944695195361E-16,0.)) ;
#81266=DIRECTION('center_axis',(3.69451600012496E-31,1.06487173641454E-15,
-1.)) ;
#81267=DIRECTION('ref_axis',(0.,1.,1.06487173641454E-15)) ;
#81268=DIRECTION('',(3.46944695195361E-16,1.,1.06487173641454E-15)) ;
#81269=DIRECTION('',(-1.,3.46944695195361E-16,0.)) ;
#81270=DIRECTION('',(-3.46944695195361E-16,-1.,-1.06487173641454E-15)) ;
#81271=DIRECTION('center_axis',(3.46944695195361E-16,1.,-4.47619207437002E-16)) ;
#81272=DIRECTION('ref_axis',(8.18685017503995E-48,4.47619207437002E-16,
1.)) ;
#81273=DIRECTION('',(1.,-3.46944695195361E-16,0.)) ;
#81274=DIRECTION('',(1.5529910948782E-31,4.47619207437002E-16,1.)) ;
#81275=DIRECTION('',(-1.5529910948782E-31,-4.47619207437002E-16,-1.)) ;
#81276=DIRECTION('center_axis',(-1.,3.46944695195361E-16,0.)) ;
#81277=DIRECTION('ref_axis',(-3.46944695195361E-16,-1.,0.)) ;
#81278=DIRECTION('center_axis',(-1.,3.46944695195361E-16,0.)) ;
#81279=DIRECTION('ref_axis',(-3.46944695195361E-16,-1.,0.)) ;
#81280=DIRECTION('',(1.5529910948782E-31,4.47619207437002E-16,1.)) ;
#81281=DIRECTION('',(0.,0.,-1.)) ;
#81282=DIRECTION('center_axis',(1.,-3.46944695195361E-16,0.)) ;
#81283=DIRECTION('ref_axis',(-3.46944695195361E-16,-1.,2.16840434497101E-15)) ;
#81284=DIRECTION('center_axis',(1.,-3.46944695195361E-16,0.)) ;
#81285=DIRECTION('ref_axis',(-3.46944695195361E-16,-1.,-6.28089534405396E-15)) ;
#81286=DIRECTION('',(3.46944695195361E-16,1.,1.06487173641454E-15)) ;
#81287=DIRECTION('center_axis',(1.,-3.46944695195361E-16,0.)) ;
#81288=DIRECTION('ref_axis',(3.46944695195361E-16,1.,0.)) ;
#81289=DIRECTION('center_axis',(-1.,3.46944695195361E-16,0.)) ;
#81290=DIRECTION('ref_axis',(3.46944695195361E-16,1.,0.)) ;
#81291=DIRECTION('',(0.,0.,-1.)) ;
#81292=DIRECTION('',(0.,0.,1.)) ;
#81293=DIRECTION('',(-3.46944695195361E-16,-1.,-9.27571383489107E-17)) ;
#81294=DIRECTION('center_axis',(-3.46944695195361E-16,-1.,0.)) ;
#81295=DIRECTION('ref_axis',(1.,-3.46944695195361E-16,0.)) ;
#81296=DIRECTION('',(1.,-3.46944695195361E-16,0.)) ;
#81297=DIRECTION('',(0.,0.,-1.)) ;
#81298=DIRECTION('',(0.,0.,1.)) ;
#81299=DIRECTION('center_axis',(1.,-3.46944695195361E-16,0.)) ;
#81300=DIRECTION('ref_axis',(3.46944695195361E-16,1.,0.)) ;
#81301=DIRECTION('center_axis',(1.,-3.46944695195361E-16,0.)) ;
#81302=DIRECTION('ref_axis',(3.46944695195361E-16,1.,0.)) ;
#81303=DIRECTION('',(1.,-3.46944695195361E-16,0.)) ;
#81304=DIRECTION('center_axis',(-1.,3.46944695195361E-16,0.)) ;
#81305=DIRECTION('ref_axis',(3.46944695195361E-16,1.,0.)) ;
#81306=DIRECTION('',(-1.,3.46944695195361E-16,0.)) ;
#81307=DIRECTION('center_axis',(-3.21815970916568E-32,-9.27571383489107E-17,
1.)) ;
#81308=DIRECTION('ref_axis',(0.,-1.,-9.27571383489107E-17)) ;
#81309=DIRECTION('',(3.46944695195361E-16,1.,9.27571383489107E-17)) ;
#81310=DIRECTION('',(1.,0.,3.21815970916568E-32)) ;
#81311=DIRECTION('',(-3.46944695195361E-16,-1.,-9.27571383489107E-17)) ;
#81312=DIRECTION('',(-1.,3.46944695195361E-16,0.)) ;
#81313=DIRECTION('center_axis',(1.,-3.46944695195361E-16,0.)) ;
#81314=DIRECTION('ref_axis',(3.46944695195361E-16,1.,0.)) ;
#81315=DIRECTION('center_axis',(1.,-3.46944695195361E-16,0.)) ;
#81316=DIRECTION('ref_axis',(-3.46944695195361E-16,-1.,-2.47817639425258E-15)) ;
#81317=DIRECTION('',(1.,-3.46944695195361E-16,0.)) ;
#81318=DIRECTION('center_axis',(-1.,3.46944695195361E-16,0.)) ;
#81319=DIRECTION('ref_axis',(3.46944695195361E-16,1.,-3.46944695195361E-15)) ;
#81320=DIRECTION('',(-1.,3.46944695195361E-16,0.)) ;
#81321=DIRECTION('center_axis',(-3.46944695195361E-16,-1.,0.)) ;
#81322=DIRECTION('ref_axis',(1.,-3.46944695195361E-16,0.)) ;
#81323=DIRECTION('',(0.,0.,-1.)) ;
#81324=DIRECTION('',(-1.,3.46944695195361E-16,0.)) ;
#81325=DIRECTION('',(0.,0.,1.)) ;
#81326=DIRECTION('center_axis',(2.25271179641597E-31,6.49299968442375E-16,
-1.)) ;
#81327=DIRECTION('ref_axis',(0.,1.,6.49299968442375E-16)) ;
#81328=DIRECTION('',(3.46944695195361E-16,1.,6.49299968442375E-16)) ;
#81329=DIRECTION('',(-1.,0.,-2.25271179641597E-31)) ;
#81330=DIRECTION('',(-3.46944695195361E-16,-1.,-6.49299968442375E-16)) ;
#81331=DIRECTION('',(1.,-3.46944695195361E-16,0.)) ;
#81332=DIRECTION('center_axis',(-1.,3.46944695195361E-16,0.)) ;
#81333=DIRECTION('ref_axis',(-3.46944695195361E-16,-1.,0.)) ;
#81334=DIRECTION('',(3.46944695195361E-16,1.,6.49299968442375E-16)) ;
#81335=DIRECTION('',(0.,0.,1.)) ;
#81336=DIRECTION('',(0.,0.,-1.)) ;
#81337=DIRECTION('center_axis',(-1.,3.46944695195361E-16,0.)) ;
#81338=DIRECTION('ref_axis',(-3.46944695195361E-16,-1.,0.)) ;
#81339=DIRECTION('center_axis',(-0.164398987305357,0.,-0.986393923832144)) ;
#81340=DIRECTION('ref_axis',(-0.986393923832144,0.,0.164398987305357)) ;
#81341=DIRECTION('',(-0.937042571331636,0.312347523777212,0.156173761888606)) ;
#81342=DIRECTION('',(0.,-1.,0.)) ;
#81343=DIRECTION('',(0.973328526784575,0.162221421130762,-0.162221421130763)) ;
#81344=DIRECTION('',(-1.73472347597681E-15,1.,2.89120579329468E-16)) ;
#81345=DIRECTION('center_axis',(-1.,0.,0.)) ;
#81346=DIRECTION('ref_axis',(0.,0.,1.)) ;
#81347=DIRECTION('center_axis',(-1.,0.,0.)) ;
#81348=DIRECTION('ref_axis',(0.,0.958782004879663,-0.284142687956128)) ;
#81349=DIRECTION('',(0.,0.,1.)) ;
#81350=DIRECTION('',(0.,-1.,0.)) ;
#81351=DIRECTION('center_axis',(-1.,0.,0.)) ;
#81352=DIRECTION('ref_axis',(0.,0.758705346999943,-0.651433954007385)) ;
#81353=DIRECTION('',(0.,0.,-1.)) ;
#81354=DIRECTION('center_axis',(-1.,0.,0.)) ;
#81355=DIRECTION('ref_axis',(0.,-0.654778494946305,-0.75582082701911)) ;
#81356=DIRECTION('',(0.,1.,0.)) ;
#81357=DIRECTION('center_axis',(-0.164398987305357,0.,0.986393923832144)) ;
#81358=DIRECTION('ref_axis',(0.986393923832144,0.,0.164398987305357)) ;
#81359=DIRECTION('',(-0.973328526784575,-0.162221421130762,-0.162221421130763)) ;
#81360=DIRECTION('',(0.,1.,0.)) ;
#81361=DIRECTION('',(0.937042571331636,-0.312347523777212,0.156173761888606)) ;
#81362=DIRECTION('',(1.73472347597681E-15,-1.,2.89120579329468E-16)) ;
#81363=DIRECTION('center_axis',(-0.573462344363329,0.81923192051904,0.)) ;
#81364=DIRECTION('ref_axis',(-0.81923192051904,-0.573462344363329,0.)) ;
#81365=DIRECTION('',(-0.710669054518702,-0.497468338163091,0.49746833816309)) ;
#81366=DIRECTION('',(0.,0.,-1.)) ;
#81367=DIRECTION('',(0.710669054518702,0.497468338163091,0.49746833816309)) ;
#81368=DIRECTION('',(0.,0.,1.)) ;
#81369=DIRECTION('center_axis',(-1.,0.,0.)) ;
#81370=DIRECTION('ref_axis',(0.,0.,1.)) ;
#81371=DIRECTION('',(0.,0.,1.)) ;
#81372=DIRECTION('',(0.,-1.,-9.34081871679819E-17)) ;
#81373=DIRECTION('',(0.,0.,-1.)) ;
#81374=DIRECTION('',(0.,1.,-9.34081871679819E-17)) ;
#81375=DIRECTION('center_axis',(-0.573462344363329,-0.81923192051904,0.)) ;
#81376=DIRECTION('ref_axis',(0.81923192051904,-0.573462344363329,0.)) ;
#81377=DIRECTION('',(-0.710669054518701,0.497468338163091,-0.497468338163091)) ;
#81378=DIRECTION('',(0.,0.,1.)) ;
#81379=DIRECTION('',(0.710669054518701,-0.497468338163091,-0.497468338163091)) ;
#81380=DIRECTION('',(0.,0.,-1.)) ;
#81381=DIRECTION('center_axis',(0.,0.,1.)) ;
#81382=DIRECTION('ref_axis',(1.,0.,0.)) ;
#81383=DIRECTION('',(1.,6.67201336914158E-17,0.)) ;
#81384=DIRECTION('',(1.33440267382831E-16,1.,0.)) ;
#81385=DIRECTION('',(-1.,1.33440267382831E-16,0.)) ;
#81386=DIRECTION('center_axis',(0.,0.,1.)) ;
#81387=DIRECTION('ref_axis',(1.,0.,0.)) ;
#81388=DIRECTION('',(1.,-1.33440267382831E-16,0.)) ;
#81389=DIRECTION('',(-1.33440267382831E-16,-1.,0.)) ;
#81390=DIRECTION('',(-1.,-6.67201336914158E-17,0.)) ;
#81391=DIRECTION('center_axis',(-6.67201336914158E-17,1.,0.)) ;
#81392=DIRECTION('ref_axis',(-1.,-6.67201336914158E-17,0.)) ;
#81393=DIRECTION('',(1.,6.67201336914158E-17,0.)) ;
#81394=DIRECTION('',(0.,0.,1.)) ;
#81395=DIRECTION('',(-1.,-6.67201336914158E-17,0.)) ;
#81396=DIRECTION('center_axis',(-1.33440267382831E-16,-1.,0.)) ;
#81397=DIRECTION('ref_axis',(1.,-1.33440267382831E-16,0.)) ;
#81398=DIRECTION('',(1.,-1.33440267382831E-16,0.)) ;
#81399=DIRECTION('',(0.,0.,-1.)) ;
#81400=DIRECTION('',(-1.,1.33440267382831E-16,0.)) ;
#81401=DIRECTION('center_axis',(0.,0.,1.)) ;
#81402=DIRECTION('ref_axis',(1.,0.,0.)) ;
#81403=DIRECTION('',(0.,-1.,0.)) ;
#81404=DIRECTION('',(1.,0.,0.)) ;
#81405=DIRECTION('',(0.,1.,0.)) ;
#81406=DIRECTION('center_axis',(0.,0.,-1.)) ;
#81407=DIRECTION('ref_axis',(1.,0.,0.)) ;
#81408=DIRECTION('',(-1.44560289664734E-16,1.,-7.2280144832367E-17)) ;
#81409=DIRECTION('center_axis',(0.,0.,1.)) ;
#81410=DIRECTION('ref_axis',(1.,0.,0.)) ;
#81411=DIRECTION('center_axis',(0.,0.,1.)) ;
#81412=DIRECTION('ref_axis',(1.,0.,0.)) ;
#81413=DIRECTION('',(0.,-1.,0.)) ;
#81414=DIRECTION('',(-1.,0.,0.)) ;
#81415=DIRECTION('',(0.,1.,0.)) ;
#81416=DIRECTION('center_axis',(0.,0.,-1.)) ;
#81417=DIRECTION('ref_axis',(1.,-1.82602471155453E-15,0.)) ;
#81418=DIRECTION('',(1.44560289664734E-16,-1.,-2.4093381610789E-16)) ;
#81419=DIRECTION('center_axis',(0.,0.,1.)) ;
#81420=DIRECTION('ref_axis',(1.,0.,0.)) ;
#81421=DIRECTION('center_axis',(0.,0.,-1.)) ;
#81422=DIRECTION('ref_axis',(-1.,0.,0.)) ;
#81423=DIRECTION('',(0.,0.,-1.)) ;
#81424=DIRECTION('center_axis',(0.,0.,-1.)) ;
#81425=DIRECTION('ref_axis',(1.,0.,0.)) ;
#81426=DIRECTION('center_axis',(0.,0.,1.)) ;
#81427=DIRECTION('ref_axis',(1.,0.,0.)) ;
#81428=DIRECTION('center_axis',(1.,0.,0.)) ;
#81429=DIRECTION('ref_axis',(0.,0.,-1.)) ;
#81430=DIRECTION('',(0.,-1.,0.)) ;
#81431=DIRECTION('',(0.,0.,1.)) ;
#81432=DIRECTION('',(0.,1.,0.)) ;
#81433=DIRECTION('center_axis',(0.81923192051904,0.573462344363329,0.)) ;
#81434=DIRECTION('ref_axis',(-0.573462344363329,0.81923192051904,0.)) ;
#81435=DIRECTION('',(-0.497468338163091,0.710669054518701,0.497468338163091)) ;
#81436=DIRECTION('',(0.,0.,-1.)) ;
#81437=DIRECTION('',(0.497468338163091,-0.710669054518701,0.497468338163091)) ;
#81438=DIRECTION('',(0.,0.,1.)) ;
#81439=DIRECTION('center_axis',(0.,1.,0.)) ;
#81440=DIRECTION('ref_axis',(0.,0.,1.)) ;
#81441=DIRECTION('',(0.,0.,1.)) ;
#81442=DIRECTION('',(-1.,0.,0.)) ;
#81443=DIRECTION('',(0.,0.,-1.)) ;
#81444=DIRECTION('',(1.,0.,0.)) ;
#81445=DIRECTION('center_axis',(-0.81923192051904,0.573462344363329,0.)) ;
#81446=DIRECTION('ref_axis',(-0.573462344363329,-0.81923192051904,0.)) ;
#81447=DIRECTION('',(0.497468338163091,0.710669054518701,-0.497468338163091)) ;
#81448=DIRECTION('',(0.,0.,1.)) ;
#81449=DIRECTION('',(-0.497468338163091,-0.710669054518701,-0.497468338163091)) ;
#81450=DIRECTION('',(0.,0.,-1.)) ;
#81451=DIRECTION('center_axis',(-1.,0.,0.)) ;
#81452=DIRECTION('ref_axis',(0.,0.,1.)) ;
#81453=DIRECTION('',(0.,-1.,0.)) ;
#81454=DIRECTION('',(0.,0.,-1.)) ;
#81455=DIRECTION('',(0.,1.,0.)) ;
#81456=DIRECTION('',(0.,0.,-1.)) ;
#81457=DIRECTION('center_axis',(0.,0.,-1.)) ;
#81458=DIRECTION('ref_axis',(-1.,0.,0.)) ;
#81459=DIRECTION('center_axis',(0.,0.,1.)) ;
#81460=DIRECTION('ref_axis',(1.,0.,0.)) ;
#81461=DIRECTION('center_axis',(0.,0.,-1.)) ;
#81462=DIRECTION('ref_axis',(1.,5.20417042793042E-15,0.)) ;
#81463=DIRECTION('center_axis',(-0.573462344363328,7.65229685658278E-17,
0.819231920519041)) ;
#81464=DIRECTION('ref_axis',(0.819231920519041,1.22423955297878E-32,0.573462344363328)) ;
#81465=DIRECTION('',(-0.710669054518702,-0.497468338163091,-0.497468338163091)) ;
#81466=DIRECTION('',(1.33440267382831E-16,1.,-2.91413396387194E-34)) ;
#81467=DIRECTION('',(0.710669054518701,-0.497468338163091,0.497468338163091)) ;
#81468=DIRECTION('',(5.04890651880155E-33,-1.,9.34081871679819E-17)) ;
#81469=DIRECTION('center_axis',(-0.573462344363328,7.65229685658278E-17,
-0.819231920519041)) ;
#81470=DIRECTION('ref_axis',(-0.819231920519041,-1.22423955297878E-32,0.573462344363328)) ;
#81471=DIRECTION('',(-0.710669054518701,0.497468338163091,0.497468338163091)) ;
#81472=DIRECTION('',(-1.33440267382831E-16,-1.,7.77328292223541E-33)) ;
#81473=DIRECTION('',(0.710669054518702,0.497468338163091,-0.497468338163091)) ;
#81474=DIRECTION('',(-5.04890651880155E-33,1.,9.34081871679819E-17)) ;
#81475=DIRECTION('center_axis',(0.,0.573462344363328,-0.819231920519041)) ;
#81476=DIRECTION('ref_axis',(0.,0.819231920519041,0.573462344363328)) ;
#81477=DIRECTION('',(0.497468338163091,0.710669054518701,0.497468338163091)) ;
#81478=DIRECTION('',(-1.,0.,0.)) ;
#81479=DIRECTION('',(0.497468338163091,-0.710669054518701,-0.497468338163091)) ;
#81480=DIRECTION('',(1.,0.,0.)) ;
#81481=DIRECTION('center_axis',(0.,0.573462344363328,0.819231920519041)) ;
#81482=DIRECTION('ref_axis',(0.,-0.819231920519041,0.573462344363328)) ;
#81483=DIRECTION('',(-0.497468338163091,0.710669054518701,-0.497468338163091)) ;
#81484=DIRECTION('',(1.,0.,0.)) ;
#81485=DIRECTION('',(-0.497468338163091,-0.710669054518701,0.497468338163091)) ;
#81486=DIRECTION('',(-1.,0.,0.)) ;
#81487=DIRECTION('center_axis',(-0.164398987305354,-0.986393923832144,0.)) ;
#81488=DIRECTION('ref_axis',(0.,0.,1.)) ;
#81489=DIRECTION('',(0.,0.,-1.)) ;
#81490=DIRECTION('center_axis',(-0.164398987305441,-0.98639392383213,1.51891488936633E-12)) ;
#81491=DIRECTION('ref_axis',(-0.0577290357396497,0.00962150595815054,0.998285923498708)) ;
#81492=DIRECTION('',(0.,0.,1.)) ;
#81493=DIRECTION('center_axis',(1.,-2.89120579329441E-16,0.)) ;
#81494=DIRECTION('ref_axis',(-2.89120579329441E-16,-1.,4.23109396156707E-14)) ;
#81495=DIRECTION('center_axis',(1.,1.15648231731787E-15,0.)) ;
#81496=DIRECTION('ref_axis',(1.15648231731787E-15,-1.,0.)) ;
#81497=DIRECTION('center_axis',(0.166689823568342,0.983956802834268,0.0635886222127804)) ;
#81498=DIRECTION('ref_axis',(-0.0486480010311504,0.0726194156279799,-0.996172571630801)) ;
#81499=DIRECTION('center_axis',(0.166689823568934,0.983956802833365,-0.0635886222252155)) ;
#81500=DIRECTION('ref_axis',(-0.0462047034218524,0.0722149192754741,0.996318287905896)) ;
#81501=DIRECTION('center_axis',(-0.164398987305354,-0.986393923832144,0.)) ;
#81502=DIRECTION('ref_axis',(0.,0.,1.)) ;
#81503=DIRECTION('',(0.,0.,1.)) ;
#81504=DIRECTION('center_axis',(-0.164398987305435,-0.986393923832131,-1.41042096917786E-12)) ;
#81505=DIRECTION('ref_axis',(-0.055419232787587,0.00923653879936327,-0.998420450005028)) ;
#81506=DIRECTION('',(0.,0.,-1.)) ;
#81507=DIRECTION('center_axis',(0.,0.,1.)) ;
#81508=DIRECTION('ref_axis',(1.,0.,0.)) ;
#81509=DIRECTION('center_axis',(0.,0.,1.)) ;
#81510=DIRECTION('ref_axis',(1.,0.,0.)) ;
#81511=DIRECTION('center_axis',(0.,1.,0.)) ;
#81512=DIRECTION('ref_axis',(1.,0.,0.)) ;
#81513=DIRECTION('center_axis',(0.,-0.888198741900269,0.45945945945946)) ;
#81514=DIRECTION('ref_axis',(0.,0.45945945945946,0.888198741900269)) ;
#81515=DIRECTION('center_axis',(-1.,0.,1.22067519501986E-15)) ;
#81516=DIRECTION('ref_axis',(-1.22067519501986E-15,0.,-1.)) ;
#81517=DIRECTION('center_axis',(0.,0.,1.)) ;
#81518=DIRECTION('ref_axis',(1.,0.,0.)) ;
#81519=DIRECTION('center_axis',(0.,0.,-1.)) ;
#81520=DIRECTION('ref_axis',(-1.,0.,0.)) ;
#81521=DIRECTION('center_axis',(1.,-3.46944695195361E-16,0.)) ;
#81522=DIRECTION('ref_axis',(3.46944695195361E-16,1.,0.)) ;
#81523=DIRECTION('center_axis',(-1.,3.46944695195361E-16,0.)) ;
#81524=DIRECTION('ref_axis',(3.46944695195361E-16,1.,4.33680868994201E-15)) ;
#81525=DIRECTION('center_axis',(-1.,3.46944695195361E-16,0.)) ;
#81526=DIRECTION('ref_axis',(-3.41607084500048E-16,-1.,0.)) ;
#81527=DIRECTION('center_axis',(0.,-0.459459459459457,0.888198741900271)) ;
#81528=DIRECTION('ref_axis',(0.,-0.888198741900271,-0.459459459459457)) ;
#81529=DIRECTION('center_axis',(1.,-3.46944695195361E-16,0.)) ;
#81530=DIRECTION('ref_axis',(0.,1.,0.)) ;
#81531=DIRECTION('center_axis',(0.,0.888198741900269,-0.45945945945946)) ;
#81532=DIRECTION('ref_axis',(0.,-0.45945945945946,-0.888198741900269)) ;
#81533=DIRECTION('center_axis',(0.,1.,0.)) ;
#81534=DIRECTION('ref_axis',(1.,0.,0.)) ;
#81535=DIRECTION('center_axis',(0.,-1.,0.)) ;
#81536=DIRECTION('ref_axis',(0.,0.,1.)) ;
#81537=DIRECTION('center_axis',(-1.,0.,0.)) ;
#81538=DIRECTION('ref_axis',(0.,0.,-1.)) ;
#81539=DIRECTION('center_axis',(0.,0.,-1.)) ;
#81540=DIRECTION('ref_axis',(-1.,0.,0.)) ;
#81541=DIRECTION('center_axis',(0.,0.,-1.)) ;
#81542=DIRECTION('ref_axis',(-1.,0.,0.)) ;
#81543=DIRECTION('center_axis',(1.,-3.46944695195361E-16,0.)) ;
#81544=DIRECTION('ref_axis',(3.46944695195361E-16,1.,0.)) ;
#81545=DIRECTION('center_axis',(-1.,3.46944695195361E-16,0.)) ;
#81546=DIRECTION('ref_axis',(3.46944695195361E-16,1.,0.)) ;
#81547=DIRECTION('center_axis',(1.,0.,0.)) ;
#81548=DIRECTION('ref_axis',(0.,0.,-1.)) ;
#81549=DIRECTION('center_axis',(0.,0.,1.)) ;
#81550=DIRECTION('ref_axis',(1.,0.,0.)) ;
#81551=DIRECTION('center_axis',(0.,0.,1.)) ;
#81552=DIRECTION('ref_axis',(1.,0.,0.)) ;
#81553=DIRECTION('center_axis',(1.,-3.46944695195361E-16,0.)) ;
#81554=DIRECTION('ref_axis',(3.80647894157197E-16,1.,0.)) ;
#81555=DIRECTION('center_axis',(0.,0.459459459459459,-0.888198741900269)) ;
#81556=DIRECTION('ref_axis',(0.,0.88819874190027,0.459459459459459)) ;
#81557=DIRECTION('center_axis',(1.,-3.46944695195361E-16,0.)) ;
#81558=DIRECTION('ref_axis',(3.46944695195361E-16,1.,0.)) ;
#81559=DIRECTION('center_axis',(-1.,3.46944695195361E-16,0.)) ;
#81560=DIRECTION('ref_axis',(3.46944695195361E-16,1.,0.)) ;
#81561=DIRECTION('center_axis',(-3.46944695195361E-16,-1.,-6.49299968442375E-16)) ;
#81562=DIRECTION('ref_axis',(2.25271179641597E-31,6.49299968442375E-16,
-1.)) ;
#81563=DIRECTION('center_axis',(0.,-1.,0.)) ;
#81564=DIRECTION('ref_axis',(0.,0.,-1.)) ;
#81565=DIRECTION('center_axis',(0.,0.,1.)) ;
#81566=DIRECTION('ref_axis',(1.,0.,0.)) ;
#81567=DIRECTION('center_axis',(-3.25260651745651E-15,0.,1.)) ;
#81568=DIRECTION('ref_axis',(1.,0.,3.25260651745651E-15)) ;
#81569=DIRECTION('center_axis',(0.,1.,0.)) ;
#81570=DIRECTION('ref_axis',(1.,0.,0.)) ;
#81571=DIRECTION('center_axis',(0.,-0.888198741900269,-0.45945945945946)) ;
#81572=DIRECTION('ref_axis',(0.,-0.45945945945946,0.888198741900269)) ;
#81573=DIRECTION('center_axis',(1.,-3.46944695195361E-16,0.)) ;
#81574=DIRECTION('ref_axis',(0.,1.,0.)) ;
#81575=DIRECTION('center_axis',(0.,0.888198741900269,0.45945945945946)) ;
#81576=DIRECTION('ref_axis',(0.,0.45945945945946,-0.888198741900269)) ;
#81577=DIRECTION('center_axis',(1.,-3.46944695195361E-16,0.)) ;
#81578=DIRECTION('ref_axis',(0.,1.,0.)) ;
#81579=DIRECTION('center_axis',(0.,1.,0.)) ;
#81580=DIRECTION('ref_axis',(0.,0.,-1.)) ;
#81581=DIRECTION('center_axis',(0.,1.,0.)) ;
#81582=DIRECTION('ref_axis',(1.,0.,0.)) ;
#81583=DIRECTION('center_axis',(-1.,0.,0.)) ;
#81584=DIRECTION('ref_axis',(0.,0.,-1.)) ;
#81585=DIRECTION('center_axis',(1.,-3.46944695195361E-16,0.)) ;
#81586=DIRECTION('ref_axis',(3.41607084500048E-16,1.,0.)) ;
#81587=DIRECTION('center_axis',(-9.62987005567165E-16,-0.459459459459459,
-0.88819874190027)) ;
#81588=DIRECTION('ref_axis',(1.2595106985394E-31,0.88819874190027,-0.459459459459459)) ;
#81589=DIRECTION('center_axis',(1.,-3.46944695195361E-16,0.)) ;
#81590=DIRECTION('ref_axis',(3.46944695195361E-16,1.,0.)) ;
#81591=DIRECTION('center_axis',(-1.,3.46944695195361E-16,0.)) ;
#81592=DIRECTION('ref_axis',(3.46944695195361E-16,1.,0.)) ;
#81593=DIRECTION('center_axis',(1.,0.,0.)) ;
#81594=DIRECTION('ref_axis',(0.,0.,-1.)) ;
#81595=DIRECTION('center_axis',(1.,-3.46944695195361E-16,0.)) ;
#81596=DIRECTION('ref_axis',(3.80647894157197E-16,1.,0.)) ;
#81597=DIRECTION('center_axis',(0.,0.459459459459459,0.888198741900269)) ;
#81598=DIRECTION('ref_axis',(0.,-0.88819874190027,0.459459459459459)) ;
#81599=DIRECTION('center_axis',(-3.46944695195361E-16,-1.,-6.49299968442375E-16)) ;
#81600=DIRECTION('ref_axis',(2.25271179641597E-31,6.49299968442375E-16,
-1.)) ;
#81601=DIRECTION('center_axis',(0.,1.,0.)) ;
#81602=DIRECTION('ref_axis',(0.,0.,-1.)) ;
#81603=DIRECTION('center_axis',(1.,0.,2.25271179641597E-31)) ;
#81604=DIRECTION('ref_axis',(2.25271179641597E-31,0.,-1.)) ;
#81605=DIRECTION('center_axis',(-1.,0.,0.)) ;
#81606=DIRECTION('ref_axis',(0.,0.,1.)) ;
#81607=DIRECTION('center_axis',(0.,1.,0.)) ;
#81608=DIRECTION('ref_axis',(1.,0.,0.)) ;
#81609=DIRECTION('center_axis',(0.,-1.,0.)) ;
#81610=DIRECTION('ref_axis',(-1.0842021724855E-15,0.,1.)) ;
#81611=DIRECTION('center_axis',(1.,-3.46944695195361E-16,0.)) ;
#81612=DIRECTION('ref_axis',(0.,1.,0.)) ;
#81613=DIRECTION('center_axis',(0.,1.,0.)) ;
#81614=DIRECTION('ref_axis',(0.,0.,-1.)) ;
#81615=DIRECTION('center_axis',(0.,-1.,0.)) ;
#81616=DIRECTION('ref_axis',(0.,0.,-1.)) ;
#81617=DIRECTION('center_axis',(0.,0.,1.)) ;
#81618=DIRECTION('ref_axis',(-1.,0.,0.)) ;
#81619=DIRECTION('center_axis',(0.,0.,-1.)) ;
#81620=DIRECTION('ref_axis',(-1.,0.,0.)) ;
#81621=DIRECTION('center_axis',(0.,0.,-1.)) ;
#81622=DIRECTION('ref_axis',(-1.,0.,0.)) ;
#81623=DIRECTION('center_axis',(-3.46944695195361E-16,-1.,-9.27571383489107E-17)) ;
#81624=DIRECTION('ref_axis',(1.,-3.46944695195361E-16,-3.21815970916568E-32)) ;
#81625=DIRECTION('center_axis',(0.,-1.,0.)) ;
#81626=DIRECTION('ref_axis',(0.,0.,-1.)) ;
#81627=DIRECTION('center_axis',(3.46944695195361E-16,1.,9.27571383489107E-17)) ;
#81628=DIRECTION('ref_axis',(-1.,3.46944695195361E-16,3.21815970916568E-32)) ;
#81629=DIRECTION('center_axis',(0.,1.,0.)) ;
#81630=DIRECTION('ref_axis',(0.,0.,-1.)) ;
#81631=DIRECTION('center_axis',(0.,0.,-1.)) ;
#81632=DIRECTION('ref_axis',(-1.,0.,0.)) ;
#81633=DIRECTION('center_axis',(0.,0.,1.)) ;
#81634=DIRECTION('ref_axis',(1.,0.,0.)) ;
#81635=DIRECTION('center_axis',(0.,1.,0.)) ;
#81636=DIRECTION('ref_axis',(1.,0.,0.)) ;
#81637=DIRECTION('center_axis',(-1.,0.,1.0842021724855E-15)) ;
#81638=DIRECTION('ref_axis',(-1.0842021724855E-15,0.,-1.)) ;
#81639=DIRECTION('center_axis',(0.,-1.,0.)) ;
#81640=DIRECTION('ref_axis',(0.,0.,-1.)) ;
#81641=DIRECTION('center_axis',(1.,0.,0.)) ;
#81642=DIRECTION('ref_axis',(0.,0.,1.)) ;
#81643=DIRECTION('center_axis',(1.,0.,3.21815970916568E-32)) ;
#81644=DIRECTION('ref_axis',(3.21815970916568E-32,0.,-1.)) ;
#81645=DIRECTION('center_axis',(0.,1.,0.)) ;
#81646=DIRECTION('ref_axis',(1.,0.,0.)) ;
#81647=DIRECTION('center_axis',(0.,0.,-1.)) ;
#81648=DIRECTION('ref_axis',(1.,0.,0.)) ;
#81649=DIRECTION('center_axis',(1.,0.,0.)) ;
#81650=DIRECTION('ref_axis',(0.,-1.0842021724855E-15,1.)) ;
#81651=DIRECTION('center_axis',(1.0842021724855E-15,1.,0.)) ;
#81652=DIRECTION('ref_axis',(1.,-1.0842021724855E-15,0.)) ;
#81653=DIRECTION('center_axis',(1.,0.,-2.08976773479518E-32)) ;
#81654=DIRECTION('ref_axis',(-2.08976773479518E-32,0.,-1.)) ;
#81655=DIRECTION('center_axis',(-0.447220452189904,-7.10036017517955E-6,
-0.894423762593907)) ;
#81656=DIRECTION('ref_axis',(0.894325663269773,0.0148067719364733,-0.447171519130972)) ;
#81657=DIRECTION('center_axis',(-1.23908819712629E-16,1.,2.4093381610789E-16)) ;
#81658=DIRECTION('ref_axis',(2.98538247827883E-32,-2.4093381610789E-16,
1.)) ;
#81659=DIRECTION('center_axis',(-5.60223420161783E-6,-0.447219005480058,
-0.89442448597187)) ;
#81660=DIRECTION('ref_axis',(0.0146917039338177,0.894327914920155,-0.447170811245647)) ;
#81661=DIRECTION('center_axis',(-8.95614743483648E-33,0.,1.)) ;
#81662=DIRECTION('ref_axis',(1.,0.,8.95614743483648E-33)) ;
#81663=DIRECTION('center_axis',(1.40488587213121E-32,-1.23908819712629E-16,
-1.)) ;
#81664=DIRECTION('ref_axis',(1.74077750246726E-48,1.,-1.23908819712629E-16)) ;
#81665=DIRECTION('center_axis',(-2.65552944032596E-32,0.,1.)) ;
#81666=DIRECTION('ref_axis',(1.,0.,2.65552944032596E-32)) ;
#81667=DIRECTION('center_axis',(0.894424485971804,-5.60223417044988E-6,
0.44721900548019)) ;
#81668=DIRECTION('ref_axis',(0.447170811245807,0.0146917039294042,-0.894327914920147)) ;
#81669=DIRECTION('center_axis',(0.894423762594036,-7.10036034885401E-6,
-0.447220452189647)) ;
#81670=DIRECTION('ref_axis',(0.447171519130767,0.0148067719290092,0.89432566327)) ;
#81671=DIRECTION('center_axis',(-8.95614743483648E-33,-1.10974565782288E-48,
1.)) ;
#81672=DIRECTION('ref_axis',(1.,-9.9390457266313E-81,8.95614743483648E-33)) ;
#81673=DIRECTION('center_axis',(-7.10036015927338E-6,0.894423762593895,
0.447220452189929)) ;
#81674=DIRECTION('ref_axis',(-0.014806771929487,-0.447171519131043,0.894325663269853)) ;
#81675=DIRECTION('center_axis',(-5.60223394757394E-6,0.89442448597165,-0.447219005480498)) ;
#81676=DIRECTION('ref_axis',(0.0146917039348304,0.447170811246077,0.894327914919923)) ;
#81677=DIRECTION('center_axis',(1.40488587213121E-32,-1.23908819712629E-16,
-1.)) ;
#81678=DIRECTION('ref_axis',(0.,1.,0.)) ;
#81679=DIRECTION('center_axis',(-1.,0.,0.)) ;
#81680=DIRECTION('ref_axis',(0.,0.,-1.)) ;
#81681=DIRECTION('center_axis',(0.,-1.,0.)) ;
#81682=DIRECTION('ref_axis',(0.,0.,1.)) ;
#81683=DIRECTION('center_axis',(-1.,0.,-1.40488587213121E-32)) ;
#81684=DIRECTION('ref_axis',(-1.40488587213121E-32,0.,1.)) ;
#81685=DIRECTION('',(-1.,0.,-1.40488587213121E-32)) ;
#81686=DIRECTION('center_axis',(-1.,0.,0.)) ;
#81687=DIRECTION('ref_axis',(0.,0.,1.)) ;
#81688=DIRECTION('center_axis',(0.,1.,0.)) ;
#81689=DIRECTION('ref_axis',(1.,0.,0.)) ;
#81690=DIRECTION('center_axis',(0.,1.,0.)) ;
#81691=DIRECTION('ref_axis',(0.,0.,-1.)) ;
#81692=DIRECTION('center_axis',(0.,0.,-1.)) ;
#81693=DIRECTION('ref_axis',(1.,0.,0.)) ;
#81694=DIRECTION('center_axis',(-1.,0.,-1.7912294869673E-32)) ;
#81695=DIRECTION('ref_axis',(-1.7912294869673E-32,0.,1.)) ;
#81696=DIRECTION('center_axis',(-0.447219005480384,-5.6022339276529E-6,
0.894424485971707)) ;
#81697=DIRECTION('ref_axis',(0.8943279149199,0.014691703940891,0.447170811245923)) ;
#81698=DIRECTION('center_axis',(-1.,0.,0.)) ;
#81699=DIRECTION('ref_axis',(0.,0.,1.)) ;
#81700=DIRECTION('center_axis',(1.23908819712629E-16,-1.,7.2280144832367E-17)) ;
#81701=DIRECTION('ref_axis',(1.,1.23908819712629E-16,-8.95614743483648E-33)) ;
#81702=DIRECTION('center_axis',(-7.10036038195002E-6,-0.447220452189466,
0.894423762594126)) ;
#81703=DIRECTION('ref_axis',(-0.0148067719344191,-0.894325663270018,-0.447171519130551)) ;
#81704=DIRECTION('center_axis',(0.,-1.,1.0842021724855E-15)) ;
#81705=DIRECTION('ref_axis',(0.,-1.0842021724855E-15,-1.)) ;
#81706=DIRECTION('center_axis',(1.23908819712629E-16,-1.,1.23908819712629E-16)) ;
#81707=DIRECTION('ref_axis',(3.32059923884369E-47,-1.23908819712629E-16,
-1.)) ;
#81708=DIRECTION('center_axis',(0.,-1.,0.)) ;
#81709=DIRECTION('ref_axis',(0.,0.,-1.)) ;
#81710=DIRECTION('',(-1.23908819712629E-16,1.,-1.23908819712629E-16)) ;
#81711=DIRECTION('center_axis',(1.,0.,1.40488587213121E-32)) ;
#81712=DIRECTION('ref_axis',(1.40488587213121E-32,0.,-1.)) ;
#81713=DIRECTION('center_axis',(-0.707106781186547,0.707106781186548,-7.05268145719399E-16)) ;
#81714=DIRECTION('ref_axis',(0.707106781186548,0.707106781186547,-6.41252558311899E-13)) ;
#81715=DIRECTION('center_axis',(1.,0.,0.)) ;
#81716=DIRECTION('ref_axis',(0.,0.,-1.)) ;
#81717=DIRECTION('center_axis',(0.,-1.,0.)) ;
#81718=DIRECTION('ref_axis',(0.,0.,-1.)) ;
#81719=DIRECTION('center_axis',(0.,0.,1.)) ;
#81720=DIRECTION('ref_axis',(-1.,0.,0.)) ;
#81721=DIRECTION('center_axis',(7.2280144832367E-17,0.,-1.)) ;
#81722=DIRECTION('ref_axis',(-1.,0.,-7.2280144832367E-17)) ;
#81723=DIRECTION('',(7.2280144832367E-17,0.,-1.)) ;
#81724=DIRECTION('center_axis',(0.,0.,-1.)) ;
#81725=DIRECTION('ref_axis',(-1.,0.,0.)) ;
#81726=DIRECTION('center_axis',(0.,1.,0.)) ;
#81727=DIRECTION('ref_axis',(1.,0.,0.)) ;
#81728=DIRECTION('center_axis',(0.,0.,1.)) ;
#81729=DIRECTION('ref_axis',(-1.,0.,0.)) ;
#81730=DIRECTION('center_axis',(0.,1.,0.)) ;
#81731=DIRECTION('ref_axis',(1.,0.,0.)) ;
#81732=DIRECTION('center_axis',(1.,0.,0.)) ;
#81733=DIRECTION('ref_axis',(0.,0.,1.)) ;
#81734=DIRECTION('center_axis',(0.,0.,-1.)) ;
#81735=DIRECTION('ref_axis',(1.,0.,0.)) ;
#81736=DIRECTION('center_axis',(-1.13380619344889E-16,1.,-1.23908819712629E-16)) ;
#81737=DIRECTION('ref_axis',(-1.40488587213121E-32,1.23908819712629E-16,
1.)) ;
#81738=DIRECTION('center_axis',(0.,1.,0.)) ;
#81739=DIRECTION('ref_axis',(0.,0.,1.)) ;
#81740=DIRECTION('center_axis',(7.2280144832367E-17,0.,-1.)) ;
#81741=DIRECTION('ref_axis',(-1.,0.,-7.2280144832367E-17)) ;
#81742=DIRECTION('center_axis',(0.,0.,1.)) ;
#81743=DIRECTION('ref_axis',(1.,0.,0.)) ;
#81744=DIRECTION('center_axis',(0.,1.,0.)) ;
#81745=DIRECTION('ref_axis',(1.,0.,0.)) ;
#81746=DIRECTION('center_axis',(0.,1.,0.)) ;
#81747=DIRECTION('ref_axis',(0.,0.,-1.)) ;
#81748=DIRECTION('center_axis',(1.,2.16840434497101E-15,-2.93873587705572E-31)) ;
#81749=DIRECTION('ref_axis',(2.16840434497101E-15,-1.,-1.03035812136257E-62)) ;
#81750=DIRECTION('center_axis',(-8.95614743483648E-33,0.,1.)) ;
#81751=DIRECTION('ref_axis',(1.,0.,8.95614743483648E-33)) ;
#81752=DIRECTION('center_axis',(-1.40488587213121E-32,1.23908819712629E-16,
1.)) ;
#81753=DIRECTION('ref_axis',(-1.74077750246726E-48,-1.,1.23908819712629E-16)) ;
#81754=DIRECTION('center_axis',(8.95614743483648E-33,1.0154535431059E-48,
-1.)) ;
#81755=DIRECTION('ref_axis',(-1.,9.09455164528354E-81,-8.95614743483648E-33)) ;
#81756=DIRECTION('center_axis',(2.16840434497101E-15,0.,-1.)) ;
#81757=DIRECTION('ref_axis',(-1.,0.,-2.16840434497101E-15)) ;
#81758=DIRECTION('',(-8.95614743483648E-33,-1.0154535431059E-48,1.)) ;
#81759=DIRECTION('center_axis',(-1.,-1.13380619344889E-16,0.)) ;
#81760=DIRECTION('ref_axis',(0.,-1.,0.)) ;
#81761=DIRECTION('center_axis',(0.,0.,1.)) ;
#81762=DIRECTION('ref_axis',(-1.,0.,0.)) ;
#81763=DIRECTION('center_axis',(0.,-1.,0.)) ;
#81764=DIRECTION('ref_axis',(0.,0.,-1.)) ;
#81765=DIRECTION('center_axis',(-1.,0.,0.)) ;
#81766=DIRECTION('ref_axis',(0.,0.,-1.)) ;
#81767=DIRECTION('center_axis',(1.,0.,1.40488587213121E-32)) ;
#81768=DIRECTION('ref_axis',(1.40488587213121E-32,0.,-1.)) ;
#81769=DIRECTION('',(1.,0.,1.40488587213121E-32)) ;
#81770=DIRECTION('center_axis',(1.,0.,0.)) ;
#81771=DIRECTION('ref_axis',(0.,0.,-1.)) ;
#81772=DIRECTION('center_axis',(-1.40488587213121E-32,1.23908819712629E-16,
1.)) ;
#81773=DIRECTION('ref_axis',(0.,-1.,0.)) ;
#81774=DIRECTION('center_axis',(0.,-1.,0.)) ;
#81775=DIRECTION('ref_axis',(0.,0.,1.)) ;
#81776=DIRECTION('center_axis',(0.,1.,0.)) ;
#81777=DIRECTION('ref_axis',(1.,0.,0.)) ;
#81778=DIRECTION('center_axis',(1.,0.,0.)) ;
#81779=DIRECTION('ref_axis',(0.,0.,1.)) ;
#81780=DIRECTION('center_axis',(0.,1.,0.)) ;
#81781=DIRECTION('ref_axis',(0.,0.,-1.)) ;
#81782=DIRECTION('center_axis',(0.,0.,1.)) ;
#81783=DIRECTION('ref_axis',(1.,0.,0.)) ;
#81784=DIRECTION('center_axis',(0.,0.,1.)) ;
#81785=DIRECTION('ref_axis',(1.,0.,0.)) ;
#81786=DIRECTION('center_axis',(1.,0.,1.40488587213121E-32)) ;
#81787=DIRECTION('ref_axis',(1.40488587213121E-32,0.,-1.)) ;
#81788=DIRECTION('center_axis',(-0.707106781186546,0.707106781186549,4.10337830236758E-15)) ;
#81789=DIRECTION('ref_axis',(0.707106781186549,0.707106781186546,2.73734725485009E-13)) ;
#81790=DIRECTION('center_axis',(-1.23908819712629E-16,1.,-1.23908819712629E-16)) ;
#81791=DIRECTION('ref_axis',(2.97429620636545E-47,1.23908819712629E-16,
1.)) ;
#81792=DIRECTION('',(1.23908819712629E-16,-1.,1.23908819712629E-16)) ;
#81793=DIRECTION('center_axis',(-1.,-1.13380619344889E-16,0.)) ;
#81794=DIRECTION('ref_axis',(0.,-1.,0.)) ;
#81795=DIRECTION('center_axis',(0.,-1.,0.)) ;
#81796=DIRECTION('ref_axis',(0.,0.,1.)) ;
#81797=DIRECTION('center_axis',(1.13380619344889E-16,-1.,1.23908819712629E-16)) ;
#81798=DIRECTION('ref_axis',(1.40488587213121E-32,-1.23908819712629E-16,
-1.)) ;
#81799=DIRECTION('center_axis',(-1.5529910948782E-31,-4.47619207437002E-16,
1.)) ;
#81800=DIRECTION('ref_axis',(6.951486430461E-47,-1.,-4.47619207437002E-16)) ;
#81801=DIRECTION('center_axis',(0.,2.16840434497101E-15,-1.)) ;
#81802=DIRECTION('ref_axis',(0.,1.,2.16840434497101E-15)) ;
#81803=DIRECTION('center_axis',(0.,1.,0.)) ;
#81804=DIRECTION('ref_axis',(1.,0.,0.)) ;
#81805=DIRECTION('center_axis',(3.85194802226865E-15,0.888198741900269,
-0.45945945945946)) ;
#81806=DIRECTION('ref_axis',(3.2526065174565E-15,-0.45945945945946,-0.888198741900269)) ;
#81807=DIRECTION('center_axis',(-1.,0.,1.22067519501986E-15)) ;
#81808=DIRECTION('ref_axis',(-1.22067519501986E-15,-1.7347234759768E-14,
-1.)) ;
#81809=DIRECTION('center_axis',(1.5529910948782E-31,4.47619207437002E-16,
-1.)) ;
#81810=DIRECTION('ref_axis',(-6.951486430461E-47,1.,4.47619207437002E-16)) ;
#81811=DIRECTION('center_axis',(0.,0.,1.)) ;
#81812=DIRECTION('ref_axis',(1.,0.,0.)) ;
#81813=DIRECTION('center_axis',(1.,-3.46944695195361E-16,0.)) ;
#81814=DIRECTION('ref_axis',(3.46944695195361E-16,1.,0.)) ;
#81815=DIRECTION('center_axis',(-1.,3.46944695195361E-16,0.)) ;
#81816=DIRECTION('ref_axis',(3.46944695195361E-16,1.,0.)) ;
#81817=DIRECTION('center_axis',(1.,-3.46944695195361E-16,0.)) ;
#81818=DIRECTION('ref_axis',(3.41607084500048E-16,1.,0.)) ;
#81819=DIRECTION('center_axis',(0.,0.459459459459457,-0.888198741900271)) ;
#81820=DIRECTION('ref_axis',(0.,0.888198741900271,0.459459459459457)) ;
#81821=DIRECTION('center_axis',(0.,0.,1.)) ;
#81822=DIRECTION('ref_axis',(1.,0.,0.)) ;
#81823=DIRECTION('center_axis',(0.,0.,-1.)) ;
#81824=DIRECTION('ref_axis',(-1.,0.,0.)) ;
#81825=DIRECTION('center_axis',(-1.,3.46944695195361E-16,0.)) ;
#81826=DIRECTION('ref_axis',(-3.46944695195361E-16,-1.,0.)) ;
#81827=DIRECTION('center_axis',(-1.,3.46944695195361E-16,0.)) ;
#81828=DIRECTION('ref_axis',(-3.46944695195361E-16,-1.,0.)) ;
#81829=DIRECTION('center_axis',(-1.,3.46944695195361E-16,0.)) ;
#81830=DIRECTION('ref_axis',(3.46944695195361E-16,1.,-5.20417042793042E-14)) ;
#81831=DIRECTION('center_axis',(1.,-3.46944695195361E-16,0.)) ;
#81832=DIRECTION('ref_axis',(0.,1.,0.)) ;
#81833=DIRECTION('center_axis',(0.,-0.888198741900269,0.459459459459461)) ;
#81834=DIRECTION('ref_axis',(0.,0.459459459459461,0.888198741900269)) ;
#81835=DIRECTION('center_axis',(0.,1.,0.)) ;
#81836=DIRECTION('ref_axis',(1.,0.,0.)) ;
#81837=DIRECTION('center_axis',(0.,1.,0.)) ;
#81838=DIRECTION('ref_axis',(0.,0.,-1.)) ;
#81839=DIRECTION('center_axis',(-1.,0.,0.)) ;
#81840=DIRECTION('ref_axis',(0.,0.,-1.)) ;
#81841=DIRECTION('center_axis',(1.,-3.46944695195361E-16,0.)) ;
#81842=DIRECTION('ref_axis',(3.70074341541719E-16,1.,0.)) ;
#81843=DIRECTION('center_axis',(0.,0.63294893130157,-0.774193548387094)) ;
#81844=DIRECTION('ref_axis',(-1.08420217248551E-15,-0.774193548387094,-0.63294893130157)) ;
#81845=DIRECTION('center_axis',(1.,-3.46944695195361E-16,0.)) ;
#81846=DIRECTION('ref_axis',(3.80647894157197E-16,1.,0.)) ;
#81847=DIRECTION('center_axis',(0.,-0.45945945945946,0.888198741900269)) ;
#81848=DIRECTION('ref_axis',(0.,-0.888198741900269,-0.45945945945946)) ;
#81849=DIRECTION('center_axis',(1.,-3.46944695195361E-16,0.)) ;
#81850=DIRECTION('ref_axis',(3.46944695195361E-16,1.,0.)) ;
#81851=DIRECTION('center_axis',(-1.,3.46944695195361E-16,0.)) ;
#81852=DIRECTION('ref_axis',(3.46944695195361E-16,1.,8.67361737988405E-15)) ;
#81853=DIRECTION('center_axis',(-3.46944695195361E-16,-1.,-2.45739631480277E-16)) ;
#81854=DIRECTION('ref_axis',(1.,-3.46944695195361E-16,-8.52580615413453E-32)) ;
#81855=DIRECTION('center_axis',(0.,1.,0.)) ;
#81856=DIRECTION('ref_axis',(0.,0.,1.)) ;
#81857=DIRECTION('center_axis',(1.,-3.46944695195361E-16,0.)) ;
#81858=DIRECTION('ref_axis',(3.33066907387547E-16,1.,0.)) ;
#81859=DIRECTION('center_axis',(8.02036034720251E-16,0.293103448275862,
-0.956080733311157)) ;
#81860=DIRECTION('ref_axis',(-1.93209005840966E-30,0.956080733311157,0.293103448275862)) ;
#81861=DIRECTION('center_axis',(-1.,3.46944695195361E-16,0.)) ;
#81862=DIRECTION('ref_axis',(-3.46944695195361E-16,-1.,0.)) ;
#81863=DIRECTION('center_axis',(-1.,3.46944695195361E-16,0.)) ;
#81864=DIRECTION('ref_axis',(-3.46944695195361E-16,-1.,0.)) ;
#81865=DIRECTION('center_axis',(-1.,3.46944695195361E-16,0.)) ;
#81866=DIRECTION('ref_axis',(-3.46944695195361E-16,-1.,0.)) ;
#81867=DIRECTION('center_axis',(0.,0.,-1.)) ;
#81868=DIRECTION('ref_axis',(-1.,0.,0.)) ;
#81869=DIRECTION('center_axis',(0.,0.,1.)) ;
#81870=DIRECTION('ref_axis',(1.,0.,0.)) ;
#81871=DIRECTION('center_axis',(-1.5529910948782E-31,-4.47619207437002E-16,
-1.)) ;
#81872=DIRECTION('ref_axis',(-6.95148643046101E-47,1.,-4.47619207437002E-16)) ;
#81873=DIRECTION('center_axis',(2.16840434497101E-15,0.,1.)) ;
#81874=DIRECTION('ref_axis',(1.,0.,-2.16840434497101E-15)) ;
#81875=DIRECTION('center_axis',(1.,-3.46944695195361E-16,0.)) ;
#81876=DIRECTION('ref_axis',(0.,1.,0.)) ;
#81877=DIRECTION('center_axis',(0.,-1.,0.)) ;
#81878=DIRECTION('ref_axis',(0.,0.,1.)) ;
#81879=DIRECTION('center_axis',(0.577350269189627,0.577350269189627,0.577350269189623)) ;
#81880=DIRECTION('ref_axis',(-0.707106781186548,2.22044604925032E-15,0.707106781186547)) ;
#81881=DIRECTION('center_axis',(-1.,3.46944695195361E-16,0.)) ;
#81882=DIRECTION('ref_axis',(-3.70074341541719E-16,-1.,0.)) ;
#81883=DIRECTION('center_axis',(0.,0.63294893130157,0.774193548387094)) ;
#81884=DIRECTION('ref_axis',(0.,0.774193548387094,-0.63294893130157)) ;
#81885=DIRECTION('center_axis',(0.,1.,0.)) ;
#81886=DIRECTION('ref_axis',(1.,0.,0.)) ;
#81887=DIRECTION('center_axis',(-1.,0.,0.)) ;
#81888=DIRECTION('ref_axis',(0.,8.67361737988405E-15,-1.)) ;
#81889=DIRECTION('center_axis',(0.,0.888198741900271,0.459459459459457)) ;
#81890=DIRECTION('ref_axis',(-1.0842021724855E-15,0.459459459459457,-0.888198741900271)) ;
#81891=DIRECTION('center_axis',(3.46944695195361E-16,1.,2.45739631480277E-16)) ;
#81892=DIRECTION('ref_axis',(-1.,3.46944695195361E-16,8.52580615413453E-32)) ;
#81893=DIRECTION('center_axis',(-1.,3.46944695195361E-16,0.)) ;
#81894=DIRECTION('ref_axis',(-3.33066907387547E-16,-1.,0.)) ;
#81895=DIRECTION('center_axis',(0.,0.293103448275864,0.956080733311156)) ;
#81896=DIRECTION('ref_axis',(0.,-0.956080733311156,0.293103448275864)) ;
#81897=DIRECTION('center_axis',(-3.46944695195361E-16,-1.,-1.06487173641454E-15)) ;
#81898=DIRECTION('ref_axis',(3.69451600012496E-31,1.06487173641454E-15,
-1.)) ;
#81899=DIRECTION('center_axis',(0.,-1.,0.)) ;
#81900=DIRECTION('ref_axis',(0.,0.,-1.)) ;
#81901=DIRECTION('center_axis',(0.,1.,0.)) ;
#81902=DIRECTION('ref_axis',(0.,0.,1.)) ;
#81903=DIRECTION('center_axis',(-1.,3.46944695195361E-16,0.)) ;
#81904=DIRECTION('ref_axis',(-3.41607084500048E-16,-1.,0.)) ;
#81905=DIRECTION('center_axis',(-4.88154879316133E-15,0.45945945945946,
0.888198741900269)) ;
#81906=DIRECTION('ref_axis',(5.19745563204766E-30,-0.888198741900269,0.45945945945946)) ;
#81907=DIRECTION('center_axis',(1.,-3.46944695195361E-16,0.)) ;
#81908=DIRECTION('ref_axis',(3.46944695195361E-16,1.,0.)) ;
#81909=DIRECTION('center_axis',(-1.,3.46944695195361E-16,0.)) ;
#81910=DIRECTION('ref_axis',(3.46944695195361E-16,1.,0.)) ;
#81911=DIRECTION('center_axis',(-1.5529910948782E-31,-4.47619207437002E-16,
-1.)) ;
#81912=DIRECTION('ref_axis',(-6.95148643046101E-47,1.,-4.47619207437002E-16)) ;
#81913=DIRECTION('center_axis',(0.,0.,-1.)) ;
#81914=DIRECTION('ref_axis',(-1.,0.,0.)) ;
#81915=DIRECTION('center_axis',(0.,0.224137931034483,-0.974557431797419)) ;
#81916=DIRECTION('ref_axis',(0.,-0.974557431797419,-0.224137931034483)) ;
#81917=DIRECTION('center_axis',(0.577350269189627,0.577350269189627,0.577350269189623)) ;
#81918=DIRECTION('ref_axis',(-0.707106781186548,2.22044604925032E-15,0.707106781186547)) ;
#81919=DIRECTION('center_axis',(0.408248290463864,-0.816496580927725,0.408248290463864)) ;
#81920=DIRECTION('ref_axis',(0.707106781186545,-2.77555756156289E-15,-0.70710678118655)) ;
#81921=DIRECTION('center_axis',(0.,1.,0.)) ;
#81922=DIRECTION('ref_axis',(1.,0.,0.)) ;
#81923=DIRECTION('center_axis',(-1.,0.,0.)) ;
#81924=DIRECTION('ref_axis',(0.,8.67361737988401E-15,-1.)) ;
#81925=DIRECTION('center_axis',(1.,-3.46944695195361E-16,0.)) ;
#81926=DIRECTION('ref_axis',(0.,1.,0.)) ;
#81927=DIRECTION('center_axis',(9.96293888229924E-16,-0.888198741900269,
-0.45945945945946)) ;
#81928=DIRECTION('ref_axis',(-1.07192530966007E-30,-0.45945945945946,0.888198741900269)) ;
#81929=DIRECTION('center_axis',(1.,-3.46944695195361E-16,0.)) ;
#81930=DIRECTION('ref_axis',(-3.70074341541719E-16,-1.,0.)) ;
#81931=DIRECTION('center_axis',(1.58436874053304E-16,-0.224137931034483,
-0.974557431797419)) ;
#81932=DIRECTION('ref_axis',(2.18893094986727E-31,0.974557431797419,-0.224137931034483)) ;
#81933=DIRECTION('center_axis',(1.,-3.46944695195361E-16,0.)) ;
#81934=DIRECTION('ref_axis',(3.46944695195361E-16,1.,0.)) ;
#81935=DIRECTION('center_axis',(-1.,3.46944695195361E-16,0.)) ;
#81936=DIRECTION('ref_axis',(3.46944695195361E-16,1.,0.)) ;
#81937=DIRECTION('center_axis',(1.,-3.46944695195361E-16,0.)) ;
#81938=DIRECTION('ref_axis',(3.80647894157197E-16,1.,0.)) ;
#81939=DIRECTION('center_axis',(0.,-0.45945945945946,-0.888198741900269)) ;
#81940=DIRECTION('ref_axis',(0.,0.888198741900269,-0.45945945945946)) ;
#81941=DIRECTION('center_axis',(1.,-3.46944695195361E-16,0.)) ;
#81942=DIRECTION('ref_axis',(0.,1.,0.)) ;
#81943=DIRECTION('center_axis',(0.,-1.,0.)) ;
#81944=DIRECTION('ref_axis',(0.,0.,1.)) ;
#81945=DIRECTION('center_axis',(-3.46944695195361E-16,-1.,-1.06487173641454E-15)) ;
#81946=DIRECTION('ref_axis',(3.69451600012496E-31,1.06487173641454E-15,
-1.)) ;
#81947=DIRECTION('center_axis',(0.,0.,1.)) ;
#81948=DIRECTION('ref_axis',(1.,0.,0.)) ;
#81949=DIRECTION('center_axis',(0.,-1.,0.)) ;
#81950=DIRECTION('ref_axis',(0.,0.,-1.)) ;
#81951=DIRECTION('center_axis',(0.,-1.,0.)) ;
#81952=DIRECTION('ref_axis',(0.,0.,-1.)) ;
#81953=DIRECTION('center_axis',(0.,1.,0.)) ;
#81954=DIRECTION('ref_axis',(0.,0.,-1.)) ;
#81955=DIRECTION('center_axis',(0.,0.,1.)) ;
#81956=DIRECTION('ref_axis',(1.,0.,0.)) ;
#81957=DIRECTION('center_axis',(8.67361737988404E-15,-1.,0.)) ;
#81958=DIRECTION('ref_axis',(1.,8.67361737988404E-15,0.)) ;
#81959=DIRECTION('center_axis',(0.497468338163091,-0.710669054518702,0.497468338163091)) ;
#81960=DIRECTION('ref_axis',(0.81923192051904,0.573462344363328,8.04804396179112E-16)) ;
#81961=DIRECTION('center_axis',(0.497468338163091,-0.710669054518702,0.497468338163091)) ;
#81962=DIRECTION('ref_axis',(0.81923192051904,0.573462344363328,7.6535433881835E-16)) ;
#81963=DIRECTION('center_axis',(0.497468338163092,-0.7106690545187,0.497468338163092)) ;
#81964=DIRECTION('ref_axis',(3.85026974001056E-16,-0.57346234436333,-0.81923192051904)) ;
#81965=DIRECTION('center_axis',(0.,0.,1.)) ;
#81966=DIRECTION('ref_axis',(1.,0.,0.)) ;
#81967=DIRECTION('center_axis',(0.,-1.,0.)) ;
#81968=DIRECTION('ref_axis',(0.,0.,-1.)) ;
#81969=DIRECTION('center_axis',(0.,1.,0.)) ;
#81970=DIRECTION('ref_axis',(0.,0.,1.)) ;
#81971=DIRECTION('center_axis',(0.,1.,0.)) ;
#81972=DIRECTION('ref_axis',(0.,0.,1.)) ;
#81973=DIRECTION('center_axis',(0.,1.,0.)) ;
#81974=DIRECTION('ref_axis',(1.,0.,0.)) ;
#81975=DIRECTION('center_axis',(-1.98515611757154E-15,0.,1.)) ;
#81976=DIRECTION('ref_axis',(-1.,0.,-1.98515611757154E-15)) ;
#81977=DIRECTION('center_axis',(1.,-4.06575814682065E-16,2.84603070277446E-16)) ;
#81978=DIRECTION('ref_axis',(-4.06575814682065E-16,-1.,6.48893816316174E-47)) ;
#81979=DIRECTION('center_axis',(0.,1.,0.)) ;
#81980=DIRECTION('ref_axis',(0.,0.,1.)) ;
#81981=DIRECTION('center_axis',(0.,1.,0.)) ;
#81982=DIRECTION('ref_axis',(0.,0.,1.)) ;
#81983=DIRECTION('center_axis',(0.497468338163091,0.710669054518702,-0.497468338163091)) ;
#81984=DIRECTION('ref_axis',(-0.81923192051904,0.573462344363328,7.6535433881835E-16)) ;
#81985=DIRECTION('center_axis',(-0.497468338163091,-0.710669054518702,0.497468338163091)) ;
#81986=DIRECTION('ref_axis',(-0.819231920519043,0.573462344363324,-7.81372826690202E-15)) ;
#81987=DIRECTION('center_axis',(-0.497468338163093,-0.7106690545187,0.497468338163091)) ;
#81988=DIRECTION('ref_axis',(0.819231920519039,-0.573462344363331,1.48853464230757E-16)) ;
#81989=DIRECTION('center_axis',(1.,0.,0.)) ;
#81990=DIRECTION('ref_axis',(0.,0.,-1.)) ;
#81991=DIRECTION('center_axis',(1.,0.,-9.9257805878577E-16)) ;
#81992=DIRECTION('ref_axis',(-9.9257805878577E-16,0.,-1.)) ;
#81993=DIRECTION('center_axis',(0.,0.,-1.)) ;
#81994=DIRECTION('ref_axis',(-1.,0.,0.)) ;
#81995=DIRECTION('center_axis',(-1.23327997120227E-15,1.76182853028895E-15,
1.)) ;
#81996=DIRECTION('ref_axis',(-2.17282783909808E-30,-1.,1.76182853028895E-15)) ;
#81997=DIRECTION('center_axis',(-0.497468338163091,0.710669054518702,0.497468338163091)) ;
#81998=DIRECTION('ref_axis',(-0.81923192051904,-0.573462344363328,7.6535433881835E-16)) ;
#81999=DIRECTION('center_axis',(0.497468338163091,-0.710669054518702,-0.497468338163091)) ;
#82000=DIRECTION('ref_axis',(-0.819231920519046,-0.57346234436332,-1.68077391522259E-14)) ;
#82001=DIRECTION('center_axis',(0.497468338163093,-0.7106690545187,-0.497468338163091)) ;
#82002=DIRECTION('ref_axis',(0.819231920519039,0.573462344363331,2.16059097207149E-16)) ;
#82003=DIRECTION('center_axis',(0.,1.,0.)) ;
#82004=DIRECTION('ref_axis',(1.,0.,0.)) ;
#82005=DIRECTION('center_axis',(-1.13841228110978E-15,-1.62630325872826E-15,
1.)) ;
#82006=DIRECTION('ref_axis',(3.52365706057789E-15,1.,1.62630325872826E-15)) ;
#82007=DIRECTION('center_axis',(0.,1.,0.)) ;
#82008=DIRECTION('ref_axis',(1.,0.,0.)) ;
#82009=DIRECTION('center_axis',(1.,0.,-1.65429676464295E-16)) ;
#82010=DIRECTION('ref_axis',(1.65429676464295E-16,0.,1.)) ;
#82011=DIRECTION('center_axis',(0.,0.,-1.)) ;
#82012=DIRECTION('ref_axis',(-1.,0.,0.)) ;
#82013=DIRECTION('center_axis',(3.3085935292859E-16,0.,1.)) ;
#82014=DIRECTION('ref_axis',(1.,0.,-3.3085935292859E-16)) ;
#82015=DIRECTION('center_axis',(1.,0.,0.)) ;
#82016=DIRECTION('ref_axis',(0.,0.,-1.)) ;
#82017=DIRECTION('center_axis',(1.,1.21972744404619E-15,8.53809210832338E-16)) ;
#82018=DIRECTION('ref_axis',(-1.21972744404619E-15,1.,-2.84382165153726E-47)) ;
#82019=DIRECTION('center_axis',(0.,1.,0.)) ;
#82020=DIRECTION('ref_axis',(1.,0.,0.)) ;
#82021=DIRECTION('center_axis',(0.497468338163092,0.710669054518701,0.497468338163092)) ;
#82022=DIRECTION('ref_axis',(7.543021249686E-16,0.573462344363329,-0.81923192051904)) ;
#82023=DIRECTION('center_axis',(-0.497468338163091,-0.710669054518702,-0.497468338163091)) ;
#82024=DIRECTION('ref_axis',(0.81923192051904,-0.573462344363328,7.6535433881835E-16)) ;
#82025=DIRECTION('center_axis',(-0.497468338163091,-0.710669054518702,-0.497468338163091)) ;
#82026=DIRECTION('ref_axis',(0.81923192051904,-0.573462344363328,7.6535433881835E-16)) ;
#82027=DIRECTION('center_axis',(0.,-1.,0.)) ;
#82028=DIRECTION('ref_axis',(0.,0.,-1.)) ;
#82029=DIRECTION('center_axis',(0.,1.,0.)) ;
#82030=DIRECTION('ref_axis',(0.,0.,-1.)) ;
#82031=DIRECTION('center_axis',(-8.67361737988403E-15,1.,0.)) ;
#82032=DIRECTION('ref_axis',(-1.,-8.67361737988403E-15,0.)) ;
#82033=DIRECTION('center_axis',(0.,0.,1.)) ;
#82034=DIRECTION('ref_axis',(1.,0.,0.)) ;
#82035=DIRECTION('center_axis',(1.,6.67201336914158E-17,0.)) ;
#82036=DIRECTION('ref_axis',(-6.67201336914158E-17,1.,0.)) ;
#82037=DIRECTION('center_axis',(-1.,-6.67201336914158E-17,0.)) ;
#82038=DIRECTION('ref_axis',(-6.67201336914158E-17,1.,0.)) ;
#82039=DIRECTION('center_axis',(-1.,1.33440267382831E-16,0.)) ;
#82040=DIRECTION('ref_axis',(-1.33440267382831E-16,-1.,0.)) ;
#82041=DIRECTION('center_axis',(-1.,1.33440267382831E-16,0.)) ;
#82042=DIRECTION('ref_axis',(-1.33440267382831E-16,-1.,0.)) ;
#82043=DIRECTION('center_axis',(0.710669054518702,0.497468338163091,0.497468338163091)) ;
#82044=DIRECTION('ref_axis',(-0.573462344363328,0.819231920519041,3.92980824865032E-16)) ;
#82045=DIRECTION('center_axis',(0.710669054518702,0.497468338163091,0.497468338163091)) ;
#82046=DIRECTION('ref_axis',(-0.573462344363328,0.819231920519041,3.92980824865032E-16)) ;
#82047=DIRECTION('center_axis',(0.710669054518701,0.497468338163091,0.497468338163092)) ;
#82048=DIRECTION('ref_axis',(0.573462344363329,4.22980978511263E-16,-0.81923192051904)) ;
#82049=DIRECTION('center_axis',(-0.710669054518702,0.497468338163091,-0.497468338163091)) ;
#82050=DIRECTION('ref_axis',(-0.573462344363328,-0.819231920519041,6.69271761853466E-16)) ;
#82051=DIRECTION('center_axis',(0.710669054518702,-0.497468338163091,0.497468338163091)) ;
#82052=DIRECTION('ref_axis',(-0.573462344363328,-0.819231920519041,6.69271761853466E-16)) ;
#82053=DIRECTION('center_axis',(0.7106690545187,-0.497468338163094,0.497468338163091)) ;
#82054=DIRECTION('ref_axis',(0.573462344363331,0.819231920519038,2.86772422505918E-16)) ;
#82055=DIRECTION('center_axis',(0.,1.,-9.34081871679819E-17)) ;
#82056=DIRECTION('ref_axis',(0.,9.34081871679819E-17,1.)) ;
#82057=DIRECTION('center_axis',(-4.33680868994205E-15,-1.,-3.03576608295944E-15)) ;
#82058=DIRECTION('ref_axis',(1.,-4.33680868994205E-15,-1.12103877145985E-44)) ;
#82059=DIRECTION('center_axis',(0.,1.,5.29374964685745E-15)) ;
#82060=DIRECTION('ref_axis',(0.,-5.29374964685745E-15,1.)) ;
#82061=DIRECTION('center_axis',(0.,1.,0.)) ;
#82062=DIRECTION('ref_axis',(1.,0.,0.)) ;
#82063=DIRECTION('center_axis',(0.,6.45175738210751E-15,1.)) ;
#82064=DIRECTION('ref_axis',(0.,1.,-6.45175738210751E-15)) ;
#82065=DIRECTION('center_axis',(-1.,-6.67201336914158E-17,0.)) ;
#82066=DIRECTION('ref_axis',(6.67201336914158E-17,-1.,0.)) ;
#82067=DIRECTION('center_axis',(-1.,-6.67201336914158E-17,0.)) ;
#82068=DIRECTION('ref_axis',(6.67201336914158E-17,-1.,0.)) ;
#82069=DIRECTION('center_axis',(1.,-1.33440267382831E-16,0.)) ;
#82070=DIRECTION('ref_axis',(1.33440267382831E-16,1.,0.)) ;
#82071=DIRECTION('center_axis',(-1.,1.33440267382831E-16,0.)) ;
#82072=DIRECTION('ref_axis',(1.33440267382831E-16,1.,0.)) ;
#82073=DIRECTION('center_axis',(0.,1.,0.)) ;
#82074=DIRECTION('ref_axis',(1.,0.,0.)) ;
#82075=DIRECTION('center_axis',(1.76182853028896E-15,-1.23327997120227E-15,
1.)) ;
#82076=DIRECTION('ref_axis',(-1.,-2.1728278390981E-30,1.76182853028896E-15)) ;
#82077=DIRECTION('center_axis',(0.,0.,-1.)) ;
#82078=DIRECTION('ref_axis',(-1.,0.,0.)) ;
#82079=DIRECTION('center_axis',(-2.71050543121378E-16,-1.89735380184965E-16,
1.)) ;
#82080=DIRECTION('ref_axis',(1.,-5.14278778484758E-32,2.71050543121378E-16)) ;
#82081=DIRECTION('center_axis',(-0.710669054518702,-0.497468338163091,0.497468338163091)) ;
#82082=DIRECTION('ref_axis',(0.573462344363328,-0.819231920519041,3.92980824865032E-16)) ;
#82083=DIRECTION('center_axis',(0.710669054518702,0.497468338163091,-0.497468338163091)) ;
#82084=DIRECTION('ref_axis',(0.573462344363328,-0.819231920519041,3.92980824865032E-16)) ;
#82085=DIRECTION('center_axis',(0.710669054518701,0.497468338163091,-0.497468338163092)) ;
#82086=DIRECTION('ref_axis',(-0.573462344363329,-3.835309211505E-16,-0.81923192051904)) ;
#82087=DIRECTION('center_axis',(0.710669054518702,-0.497468338163091,-0.497468338163091)) ;
#82088=DIRECTION('ref_axis',(0.573462344363328,0.819231920519041,6.69271761853466E-16)) ;
#82089=DIRECTION('center_axis',(0.710669054518702,-0.497468338163091,-0.497468338163091)) ;
#82090=DIRECTION('ref_axis',(0.573462344363328,0.819231920519041,6.69271761853466E-16)) ;
#82091=DIRECTION('center_axis',(0.7106690545187,-0.497468338163091,-0.497468338163093)) ;
#82092=DIRECTION('ref_axis',(-0.57346234436333,9.18832260081103E-16,-0.819231920519039)) ;
#82093=DIRECTION('center_axis',(0.,0.,-1.)) ;
#82094=DIRECTION('ref_axis',(-1.,0.,0.)) ;
#82095=DIRECTION('center_axis',(0.,1.15800773525007E-15,1.)) ;
#82096=DIRECTION('ref_axis',(0.,-1.,1.15800773525007E-15)) ;
#82097=DIRECTION('center_axis',(0.,1.,0.)) ;
#82098=DIRECTION('ref_axis',(1.,0.,0.)) ;
#82099=DIRECTION('center_axis',(0.,1.,0.)) ;
#82100=DIRECTION('ref_axis',(0.,0.,-1.)) ;
#82101=DIRECTION('center_axis',(0.,1.,0.)) ;
#82102=DIRECTION('ref_axis',(1.,0.,0.)) ;
#82103=DIRECTION('center_axis',(4.33680868994204E-15,-1.,-3.03576608295944E-15)) ;
#82104=DIRECTION('ref_axis',(-1.,-4.33680868994204E-15,5.60519385729927E-45)) ;
#82105=DIRECTION('center_axis',(0.,1.,9.34081871679819E-17)) ;
#82106=DIRECTION('ref_axis',(0.,-9.34081871679819E-17,1.)) ;
#82107=DIRECTION('center_axis',(0.,0.,1.)) ;
#82108=DIRECTION('ref_axis',(1.,0.,0.)) ;
#82109=DIRECTION('center_axis',(-2.16840434497102E-15,-3.61400724161847E-16,
1.)) ;
#82110=DIRECTION('ref_axis',(1.,-7.83662900548222E-31,2.16840434497102E-15)) ;
#82111=DIRECTION('center_axis',(0.973328526784575,0.162221421130762,-0.162221421130763)) ;
#82112=DIRECTION('ref_axis',(-0.164398987305358,5.55382797573317E-16,-0.986393923832144)) ;
#82113=DIRECTION('center_axis',(0.973328526784574,0.162221421130765,-0.162221421130767)) ;
#82114=DIRECTION('ref_axis',(-0.164398987305362,-2.05045540520021E-17,-0.986393923832143)) ;
#82115=DIRECTION('center_axis',(0.,1.,0.)) ;
#82116=DIRECTION('ref_axis',(1.,0.,0.)) ;
#82117=DIRECTION('center_axis',(0.,1.,-8.79325913341701E-15)) ;
#82118=DIRECTION('ref_axis',(0.,-8.79325913341701E-15,-1.)) ;
#82119=DIRECTION('center_axis',(0.,0.,1.)) ;
#82120=DIRECTION('ref_axis',(1.,0.,0.)) ;
#82121=DIRECTION('center_axis',(0.,-2.28569887277128E-15,1.)) ;
#82122=DIRECTION('ref_axis',(0.,-1.,-2.28569887277128E-15)) ;
#82123=DIRECTION('center_axis',(1.73472347597681E-15,-1.,-2.89120579329468E-16)) ;
#82124=DIRECTION('ref_axis',(1.,1.73472347597681E-15,5.01544256350843E-31)) ;
#82125=DIRECTION('center_axis',(8.67361737988409E-15,1.,-1.44560289664739E-15)) ;
#82126=DIRECTION('ref_axis',(-1.,8.67361737988409E-15,-1.40129846432482E-45)) ;
#82127=DIRECTION('center_axis',(0.,1.,0.)) ;
#82128=DIRECTION('ref_axis',(1.,0.,0.)) ;
#82129=DIRECTION('center_axis',(-0.937042571331634,0.312347523777217,0.156173761888611)) ;
#82130=DIRECTION('ref_axis',(0.316227766016843,0.948683298050512,6.71158276827649E-18)) ;
#82131=DIRECTION('center_axis',(0.937042571331636,-0.312347523777212,-0.156173761888606)) ;
#82132=DIRECTION('ref_axis',(0.316227766016838,0.948683298050514,8.61595672567599E-16)) ;
#82133=DIRECTION('center_axis',(-0.973328526784575,-0.162221421130762,-0.162221421130763)) ;
#82134=DIRECTION('ref_axis',(-0.164398987305358,5.55382797573317E-16,0.986393923832144)) ;
#82135=DIRECTION('center_axis',(0.97823197629215,-0.146734796047206,-0.146734795425419)) ;
#82136=DIRECTION('ref_axis',(0.182318633555366,0.945435290883781,0.270022270581529)) ;
#82137=DIRECTION('center_axis',(0.973328526784574,0.162221421130767,0.162221421130768)) ;
#82138=DIRECTION('ref_axis',(0.164398987305363,2.02768900722254E-16,-0.986393923832143)) ;
#82139=DIRECTION('center_axis',(0.,0.,1.)) ;
#82140=DIRECTION('ref_axis',(1.,0.,0.)) ;
#82141=DIRECTION('center_axis',(0.,2.19831478335425E-15,-1.)) ;
#82142=DIRECTION('ref_axis',(0.,1.,2.19831478335425E-15)) ;
#82143=DIRECTION('center_axis',(0.,1.,0.)) ;
#82144=DIRECTION('ref_axis',(1.,0.,0.)) ;
#82145=DIRECTION('center_axis',(8.67361737988408E-15,1.,1.44560289664739E-15)) ;
#82146=DIRECTION('ref_axis',(1.,-8.67361737988408E-15,5.60519385729927E-45)) ;
#82147=DIRECTION('center_axis',(1.73472347597681E-15,-1.,2.89120579329468E-16)) ;
#82148=DIRECTION('ref_axis',(1.,1.73472347597681E-15,-5.01544256350843E-31)) ;
#82149=DIRECTION('center_axis',(0.,1.,0.)) ;
#82150=DIRECTION('ref_axis',(0.,0.,1.)) ;
#82151=DIRECTION('center_axis',(0.,0.,1.)) ;
#82152=DIRECTION('ref_axis',(1.,0.,0.)) ;
#82153=DIRECTION('center_axis',(3.25260651745652E-15,-1.08420217248553E-15,
-1.)) ;
#82154=DIRECTION('ref_axis',(-1.,-3.52648305246695E-30,-3.25260651745652E-15)) ;
#82155=DIRECTION('center_axis',(0.,1.,0.)) ;
#82156=DIRECTION('ref_axis',(1.,0.,0.)) ;
#82157=DIRECTION('center_axis',(-0.937042571331635,0.312347523777215,-0.15617376188861)) ;
#82158=DIRECTION('ref_axis',(0.316227766016841,0.948683298050513,6.5590042956861E-18)) ;
#82159=DIRECTION('center_axis',(-0.937042571331636,0.312347523777212,-0.156173761888606)) ;
#82160=DIRECTION('ref_axis',(0.331350514299575,0.654034959159593,-0.680033167478261)) ;
#82161=DIRECTION('center_axis',(0.961519724091326,0.245047216427987,-0.124224320904711)) ;
#82162=DIRECTION('ref_axis',(0.262092069890881,-0.682554728203127,0.682221950620082)) ;
#82163=DIRECTION('center_axis',(2.65552944032596E-32,3.29043518662928E-48,
-1.)) ;
#82164=DIRECTION('ref_axis',(-1.,8.7378475095785E-80,-2.65552944032596E-32)) ;
#82165=DIRECTION('center_axis',(2.65552944032596E-32,3.29043518662928E-48,
-1.)) ;
#82166=DIRECTION('ref_axis',(-1.,8.7378475095785E-80,-2.65552944032596E-32)) ;
#82167=DIRECTION('center_axis',(-2.65552944032596E-32,-3.29043518662928E-48,
1.)) ;
#82168=DIRECTION('ref_axis',(-1.,8.7378475095785E-80,-2.65552944032596E-32)) ;
#82169=DIRECTION('center_axis',(0.,0.,1.)) ;
#82170=DIRECTION('ref_axis',(1.,0.,0.)) ;
#82171=DIRECTION('center_axis',(0.,0.,-1.)) ;
#82172=DIRECTION('ref_axis',(-1.,0.,0.)) ;
#82173=DIRECTION('center_axis',(0.,0.,1.)) ;
#82174=DIRECTION('ref_axis',(1.,0.,0.)) ;
#82175=DIRECTION('center_axis',(0.,0.,1.)) ;
#82176=DIRECTION('ref_axis',(1.,0.,0.)) ;
#82177=DIRECTION('center_axis',(0.,0.,-1.)) ;
#82178=DIRECTION('ref_axis',(-1.,0.,0.)) ;
#82179=DIRECTION('center_axis',(0.,0.,-1.)) ;
#82180=DIRECTION('ref_axis',(-1.,0.,0.)) ;
#82181=DIRECTION('center_axis',(1.,1.15648231731787E-15,0.)) ;
#82182=DIRECTION('ref_axis',(1.03435541192675E-15,-1.,7.75766558945062E-16)) ;
#82183=DIRECTION('center_axis',(7.089177613099E-16,-0.612994899008946,-0.790086864711098)) ;
#82184=DIRECTION('ref_axis',(-4.46849810277083E-31,-0.790086864711098,0.612994899008946)) ;
#82185=DIRECTION('center_axis',(7.08917761309899E-16,-0.612994899008945,
0.790086864711098)) ;
#82186=DIRECTION('ref_axis',(-1.73472347597681E-14,0.790086864711098,0.612994899008945)) ;
#82187=DIRECTION('center_axis',(0.,0.,-1.)) ;
#82188=DIRECTION('ref_axis',(-1.,0.,0.)) ;
#82189=DIRECTION('center_axis',(0.,0.,1.)) ;
#82190=DIRECTION('ref_axis',(-1.,2.16840434497102E-15,0.)) ;
#82191=DIRECTION('center_axis',(1.08420217248551E-15,-1.,0.)) ;
#82192=DIRECTION('ref_axis',(1.,1.08420217248551E-15,0.)) ;
#82193=DIRECTION('center_axis',(1.44560289664734E-16,-1.,-2.4093381610789E-16)) ;
#82194=DIRECTION('ref_axis',(-7.25154722885103E-47,2.4093381610789E-16,
-1.)) ;
#82195=DIRECTION('center_axis',(0.,-1.,0.)) ;
#82196=DIRECTION('ref_axis',(0.,0.,-1.)) ;
#82197=DIRECTION('center_axis',(1.,0.,0.)) ;
#82198=DIRECTION('ref_axis',(0.,1.,0.)) ;
#82199=DIRECTION('center_axis',(1.,0.,0.)) ;
#82200=DIRECTION('ref_axis',(0.,0.,-1.)) ;
#82201=DIRECTION('center_axis',(1.,1.23908819712629E-16,8.95614743483648E-33)) ;
#82202=DIRECTION('ref_axis',(-1.23908819712629E-16,1.,-1.10974565782288E-48)) ;
#82203=DIRECTION('center_axis',(1.,0.,0.)) ;
#82204=DIRECTION('ref_axis',(0.,0.,-1.)) ;
#82205=DIRECTION('center_axis',(-1.,0.,0.)) ;
#82206=DIRECTION('ref_axis',(0.,0.,1.)) ;
#82207=DIRECTION('center_axis',(1.,1.23908819712629E-16,8.95614743483648E-33)) ;
#82208=DIRECTION('ref_axis',(-1.23908819712629E-16,1.,-1.10974565782288E-48)) ;
#82209=DIRECTION('center_axis',(-1.,0.,0.)) ;
#82210=DIRECTION('ref_axis',(0.,0.,1.)) ;
#82211=DIRECTION('center_axis',(1.,0.,0.)) ;
#82212=DIRECTION('ref_axis',(0.,-1.,0.)) ;
#82213=DIRECTION('center_axis',(0.,1.,0.)) ;
#82214=DIRECTION('ref_axis',(0.,0.,1.)) ;
#82215=DIRECTION('center_axis',(-1.44560289664734E-16,1.,-7.2280144832367E-17)) ;
#82216=DIRECTION('ref_axis',(0.707106781238324,1.5332934167208E-16,0.707106781134771)) ;
#82217=DIRECTION('center_axis',(-1.0842021724855E-15,1.,0.)) ;
#82218=DIRECTION('ref_axis',(-1.,-1.0842021724855E-15,0.)) ;
#82219=DIRECTION('center_axis',(0.,1.,0.)) ;
#82220=DIRECTION('ref_axis',(0.,0.,1.)) ;
#82221=DIRECTION('center_axis',(0.,-1.,0.)) ;
#82222=DIRECTION('ref_axis',(0.,0.,-1.)) ;
#82223=DIRECTION('center_axis',(0.,1.,0.)) ;
#82224=DIRECTION('ref_axis',(0.,0.,1.)) ;
#82225=DIRECTION('center_axis',(0.,0.,1.)) ;
#82226=DIRECTION('ref_axis',(1.,0.,0.)) ;
#82227=DIRECTION('center_axis',(0.431191646767808,0.0335421424157979,0.901636672080181)) ;
#82228=DIRECTION('ref_axis',(0.899826811333414,0.057359327390736,-0.432459960189175)) ;
#82229=DIRECTION('center_axis',(0.,0.,1.)) ;
#82230=DIRECTION('ref_axis',(-1.,0.,0.)) ;
#82231=DIRECTION('center_axis',(0.,0.,-1.)) ;
#82232=DIRECTION('ref_axis',(0.707109343403326,-0.707104218960485,0.)) ;
#82233=DIRECTION('center_axis',(-3.25260651745653E-15,0.,1.)) ;
#82234=DIRECTION('ref_axis',(1.,0.,3.25260651745653E-15)) ;
#82235=DIRECTION('center_axis',(0.,0.,1.)) ;
#82236=DIRECTION('ref_axis',(1.,0.,0.)) ;
#82237=DIRECTION('center_axis',(0.431188264323626,0.0335835000995436,-0.901636750155318)) ;
#82238=DIRECTION('ref_axis',(0.899831768136793,0.0572892327006458,0.432458937782981)) ;
#82239=DIRECTION('center_axis',(0.,-1.,0.)) ;
#82240=DIRECTION('ref_axis',(0.,0.,-1.)) ;
#82241=DIRECTION('center_axis',(0.,1.,0.)) ;
#82242=DIRECTION('ref_axis',(0.,0.,1.)) ;
#82243=DIRECTION('center_axis',(0.,0.,1.)) ;
#82244=DIRECTION('ref_axis',(1.,0.,0.)) ;
#82245=DIRECTION('center_axis',(0.,0.,-1.)) ;
#82246=DIRECTION('ref_axis',(-1.,0.,0.)) ;
#82247=DIRECTION('center_axis',(0.,0.,1.)) ;
#82248=DIRECTION('ref_axis',(-0.986393923832144,0.164398987305354,0.)) ;
#82249=DIRECTION('center_axis',(0.98470178743927,-0.164116964573216,0.0585492250433781)) ;
#82250=DIRECTION('ref_axis',(0.164398987305362,0.986393923832143,-7.60669428566932E-17)) ;
#82251=DIRECTION('center_axis',(0.984834538781277,-0.164139089796902,0.0562075655416074)) ;
#82252=DIRECTION('ref_axis',(0.164398987305379,0.98639392383214,1.87706412796466E-17)) ;
#82253=DIRECTION('center_axis',(0.986393923832144,-0.129889480441767,0.100775740620418)) ;
#82254=DIRECTION('ref_axis',(0.,0.612994899008947,0.790086864711097)) ;
#82255=DIRECTION('center_axis',(0.,1.,0.)) ;
#82256=DIRECTION('ref_axis',(1.,0.,0.)) ;
#82257=DIRECTION('center_axis',(0.,0.,-1.)) ;
#82258=DIRECTION('ref_axis',(-1.,0.,0.)) ;
#82259=DIRECTION('center_axis',(1.,2.8359373108165E-15,0.)) ;
#82260=DIRECTION('ref_axis',(-2.8359373108165E-15,1.,0.)) ;
#82261=DIRECTION('center_axis',(0.,0.,-1.)) ;
#82262=DIRECTION('ref_axis',(-1.,0.,0.)) ;
#82263=DIRECTION('center_axis',(0.,0.,1.)) ;
#82264=DIRECTION('ref_axis',(1.,0.,0.)) ;
#82265=DIRECTION('center_axis',(1.,0.,0.)) ;
#82266=DIRECTION('ref_axis',(0.,0.,-1.)) ;
#82267=DIRECTION('center_axis',(1.,0.,0.)) ;
#82268=DIRECTION('ref_axis',(0.,0.,-1.)) ;
#82269=DIRECTION('center_axis',(0.,1.,0.)) ;
#82270=DIRECTION('ref_axis',(1.,0.,0.)) ;
#82271=DIRECTION('center_axis',(1.,-8.50781193244945E-15,0.)) ;
#82272=DIRECTION('ref_axis',(8.50781193244945E-15,1.,0.)) ;
#82273=DIRECTION('center_axis',(0.,1.,0.)) ;
#82274=DIRECTION('ref_axis',(1.,0.,0.)) ;
#82275=DIRECTION('center_axis',(-5.42101086242753E-16,1.70882313734897E-16,
1.)) ;
#82276=DIRECTION('ref_axis',(1.,9.26354878953623E-32,5.42101086242753E-16)) ;
#82277=DIRECTION('center_axis',(-1.,0.,0.)) ;
#82278=DIRECTION('ref_axis',(0.,0.,1.)) ;
#82279=DIRECTION('center_axis',(1.,0.,0.)) ;
#82280=DIRECTION('ref_axis',(0.,0.,-1.)) ;
#82281=DIRECTION('center_axis',(0.,0.,-1.)) ;
#82282=DIRECTION('ref_axis',(-1.,0.,0.)) ;
#82283=DIRECTION('center_axis',(0.,0.,1.)) ;
#82284=DIRECTION('ref_axis',(1.,0.,0.)) ;
#82285=DIRECTION('center_axis',(0.,1.,0.)) ;
#82286=DIRECTION('ref_axis',(1.,0.,0.)) ;
#82287=DIRECTION('center_axis',(0.,1.,0.)) ;
#82288=DIRECTION('ref_axis',(1.,0.,0.)) ;
#82289=DIRECTION('center_axis',(0.,0.,-1.)) ;
#82290=DIRECTION('ref_axis',(-1.,0.,0.)) ;
#82291=DIRECTION('center_axis',(0.,1.,0.)) ;
#82292=DIRECTION('ref_axis',(0.,0.,1.)) ;
#82293=DIRECTION('center_axis',(0.,0.,-1.)) ;
#82294=DIRECTION('ref_axis',(-1.,0.,0.)) ;
#82295=DIRECTION('center_axis',(0.,0.,1.)) ;
#82296=DIRECTION('ref_axis',(1.,0.,0.)) ;
#82297=DIRECTION('center_axis',(1.33440267382831E-16,1.,0.)) ;
#82298=DIRECTION('ref_axis',(-1.,1.33440267382831E-16,0.)) ;
#82299=DIRECTION('center_axis',(0.,1.,0.)) ;
#82300=DIRECTION('ref_axis',(0.,0.,1.)) ;
#82301=DIRECTION('center_axis',(0.,1.,0.)) ;
#82302=DIRECTION('ref_axis',(1.,0.,0.)) ;
#82303=DIRECTION('center_axis',(0.,1.,0.)) ;
#82304=DIRECTION('ref_axis',(0.,0.,1.)) ;
#82305=DIRECTION('center_axis',(0.,1.,0.)) ;
#82306=DIRECTION('ref_axis',(1.,0.,0.)) ;
#82307=DIRECTION('center_axis',(1.37797793267296E-15,-1.62630325872825E-15,
1.)) ;
#82308=DIRECTION('ref_axis',(-2.24101000236165E-30,-1.,-1.62630325872825E-15)) ;
#82309=DIRECTION('center_axis',(-1.33440267382831E-16,-1.,0.)) ;
#82310=DIRECTION('ref_axis',(1.,-1.33440267382831E-16,0.)) ;
#82311=DIRECTION('center_axis',(0.,1.,0.)) ;
#82312=DIRECTION('ref_axis',(0.,0.,1.)) ;
#82313=DIRECTION('center_axis',(0.,0.,-1.)) ;
#82314=DIRECTION('ref_axis',(-1.,0.,0.)) ;
#82315=DIRECTION('center_axis',(0.,0.,1.)) ;
#82316=DIRECTION('ref_axis',(1.,0.,0.)) ;
#82317=DIRECTION('center_axis',(0.,1.,0.)) ;
#82318=DIRECTION('ref_axis',(1.,0.,0.)) ;
#82319=DIRECTION('center_axis',(0.,0.,1.)) ;
#82320=DIRECTION('ref_axis',(1.,0.,0.)) ;
#82321=DIRECTION('center_axis',(0.,0.,1.)) ;
#82322=DIRECTION('ref_axis',(1.,0.,0.)) ;
#82323=DIRECTION('center_axis',(0.,0.,1.)) ;
#82324=DIRECTION('ref_axis',(-0.986393923832144,0.164398987305354,0.)) ;
#82325=DIRECTION('center_axis',(0.984701787439272,-0.164116964573205,-0.0585492250433871)) ;
#82326=DIRECTION('ref_axis',(0.16439898730535,0.986393923832145,-3.2807868055655E-16)) ;
#82327=DIRECTION('center_axis',(0.984834538781259,-0.164139089796881,-0.0562075655419907)) ;
#82328=DIRECTION('ref_axis',(0.164398987305362,0.986393923832143,6.03508511856301E-17)) ;
#82329=DIRECTION('center_axis',(0.,0.,1.)) ;
#82330=DIRECTION('ref_axis',(-0.986393923832144,0.164398987305354,0.)) ;
#82331=DIRECTION('center_axis',(0.,0.,1.)) ;
#82332=DIRECTION('ref_axis',(1.,0.,0.)) ;
#82333=DIRECTION('center_axis',(0.342346838791228,0.100237737313318,-0.934211452503104)) ;
#82334=DIRECTION('ref_axis',(0.878411849450466,0.318727804720941,0.356097190725765)) ;
#82335=DIRECTION('center_axis',(0.,0.,-1.)) ;
#82336=DIRECTION('ref_axis',(-1.,0.,0.)) ;
#82337=DIRECTION('center_axis',(0.,0.,-1.)) ;
#82338=DIRECTION('ref_axis',(-1.,0.,0.)) ;
#82339=DIRECTION('center_axis',(0.,0.,-1.)) ;
#82340=DIRECTION('ref_axis',(-1.,0.,0.)) ;
#82341=DIRECTION('center_axis',(-0.34234683879479,-0.100237737344036,-0.934211452498503)) ;
#82342=DIRECTION('ref_axis',(0.878411778138233,0.318728006274644,-0.356097186234627)) ;
#82343=DIRECTION('center_axis',(0.,0.,1.)) ;
#82344=DIRECTION('ref_axis',(1.,0.,0.)) ;
#82345=DIRECTION('center_axis',(0.967224433243486,0.251696850982797,0.0335498277515765)) ;
#82346=DIRECTION('ref_axis',(0.148186128295972,-0.666803800143469,0.73035167111117)) ;
#82347=DIRECTION('center_axis',(0.,0.707106781186549,-0.707106781186547)) ;
#82348=DIRECTION('ref_axis',(0.,0.707106781186546,0.707106781186549)) ;
#82349=DIRECTION('center_axis',(0.978007532938557,-0.147978541149799,-0.146981688909249)) ;
#82350=DIRECTION('ref_axis',(0.193734423935374,0.383507624650126,0.902988856419417)) ;
#82351=DIRECTION('center_axis',(0.,0.447213595499958,0.894427190999916)) ;
#82352=DIRECTION('ref_axis',(0.,-0.894427190999916,0.447213595499958)) ;
#82353=DIRECTION('center_axis',(0.960001452008117,0.250435160947751,-0.125217579849561)) ;
#82354=DIRECTION('ref_axis',(0.276742394168104,-0.916645079798534,0.288401534238716)) ;
#82355=DIRECTION('center_axis',(0.,1.,0.)) ;
#82356=DIRECTION('ref_axis',(0.,0.,1.)) ;
#82357=DIRECTION('center_axis',(-1.,0.,0.)) ;
#82358=DIRECTION('ref_axis',(0.,0.413905208611621,-0.910319986754202)) ;
#82359=DIRECTION('center_axis',(1.,1.44560289664734E-16,0.)) ;
#82360=DIRECTION('ref_axis',(0.,1.,0.)) ;
#82361=DIRECTION('center_axis',(1.,1.44560289664734E-16,0.)) ;
#82362=DIRECTION('ref_axis',(-1.44560289664734E-16,1.,0.)) ;
#82363=DIRECTION('center_axis',(0.,0.,-1.)) ;
#82364=DIRECTION('ref_axis',(0.,-1.,0.)) ;
#82365=DIRECTION('center_axis',(-1.,-1.44560289664734E-16,0.)) ;
#82366=DIRECTION('ref_axis',(-1.44560289664734E-16,1.,0.)) ;
#82367=DIRECTION('center_axis',(1.,-3.46944695195361E-16,0.)) ;
#82368=DIRECTION('ref_axis',(2.61228946970625E-16,1.,0.)) ;
#82369=DIRECTION('center_axis',(1.,-3.46944695195361E-16,0.)) ;
#82370=DIRECTION('ref_axis',(3.46944695195361E-16,1.,0.)) ;
#82371=DIRECTION('center_axis',(0.,0.,1.)) ;
#82372=DIRECTION('ref_axis',(-3.26536183713281E-16,-1.,0.)) ;
#82373=DIRECTION('center_axis',(-1.,3.46944695195361E-16,0.)) ;
#82374=DIRECTION('ref_axis',(3.46944695195361E-16,1.,0.)) ;
#82375=DIRECTION('center_axis',(-1.,3.46944695195361E-16,0.)) ;
#82376=DIRECTION('ref_axis',(-3.46944695195361E-16,-1.,0.)) ;
#82377=DIRECTION('center_axis',(-1.,0.,0.)) ;
#82378=DIRECTION('ref_axis',(0.,0.,1.)) ;
#82379=DIRECTION('',(1.,-3.46944695195361E-16,0.)) ;
#82380=DIRECTION('center_axis',(-1.,8.01625584951926E-16,-1.08420217248551E-15)) ;
#82381=DIRECTION('ref_axis',(1.08420217248551E-15,-4.33680868994204E-15,
-1.)) ;
#82382=DIRECTION('center_axis',(-1.,8.01625584951926E-16,-1.08420217248551E-15)) ;
#82383=DIRECTION('ref_axis',(1.08420217248551E-15,-4.33680868994204E-15,
-1.)) ;
#82384=DIRECTION('',(-1.,3.46944695195361E-16,0.)) ;
#82385=DIRECTION('center_axis',(-1.,3.46944695195361E-16,0.)) ;
#82386=DIRECTION('ref_axis',(-3.46944695195361E-16,-1.,0.)) ;
#82387=DIRECTION('center_axis',(-1.,0.,0.)) ;
#82388=DIRECTION('ref_axis',(0.,0.,1.)) ;
#82389=DIRECTION('',(1.,-3.46944695195361E-16,0.)) ;
#82390=DIRECTION('center_axis',(-1.,2.2680138501079E-15,0.)) ;
#82391=DIRECTION('ref_axis',(2.2680138501079E-15,1.,0.)) ;
#82392=DIRECTION('',(-1.,3.46944695195361E-16,0.)) ;
#82393=DIRECTION('center_axis',(-1.,3.18032637262401E-16,0.)) ;
#82394=DIRECTION('ref_axis',(-5.55111512312578E-16,-1.,0.)) ;
#82395=DIRECTION('center_axis',(1.,-3.18032637262401E-16,0.)) ;
#82396=DIRECTION('ref_axis',(-3.18032637262401E-16,-1.,0.)) ;
#82397=DIRECTION('center_axis',(-2.01298417874256E-16,-0.632948931301568,
-0.774193548387096)) ;
#82398=DIRECTION('ref_axis',(1.73472347597681E-14,-0.774193548387096,0.632948931301568)) ;
#82399=DIRECTION('center_axis',(-1.,3.18032637262401E-16,0.)) ;
#82400=DIRECTION('ref_axis',(-3.18032637262401E-16,-1.,0.)) ;
#82401=DIRECTION('center_axis',(-2.01298417874256E-16,-0.632948931301568,
0.774193548387096)) ;
#82402=DIRECTION('ref_axis',(9.63584817660562E-32,-0.774193548387096,-0.632948931301568)) ;
#82403=DIRECTION('center_axis',(1.,1.44560289664734E-16,0.)) ;
#82404=DIRECTION('ref_axis',(-1.44560289664734E-16,1.,0.)) ;
#82405=DIRECTION('',(-1.,-1.44560289664734E-16,0.)) ;
#82406=DIRECTION('center_axis',(-1.,3.46944695195361E-16,0.)) ;
#82407=DIRECTION('ref_axis',(-3.46944695195361E-16,-1.,0.)) ;
#82408=DIRECTION('',(-1.,3.46944695195361E-16,0.)) ;
#82409=DIRECTION('center_axis',(-1.,3.46944695195361E-16,0.)) ;
#82410=DIRECTION('ref_axis',(3.46944695195361E-16,1.,-3.46944695195361E-15)) ;
#82411=DIRECTION('center_axis',(-1.,3.46944695195361E-16,0.)) ;
#82412=DIRECTION('ref_axis',(3.46944695195361E-16,1.,0.)) ;
#82413=DIRECTION('center_axis',(-1.,3.46944695195361E-16,0.)) ;
#82414=DIRECTION('ref_axis',(-3.46944695195361E-16,-1.,0.)) ;
#82415=DIRECTION('',(1.,-3.46944695195361E-16,0.)) ;
#82416=DIRECTION('center_axis',(-1.,-1.44560289664734E-16,-2.65552944032596E-32)) ;
#82417=DIRECTION('ref_axis',(1.44560289664734E-16,-1.,-2.80018320648271E-64)) ;
#82418=DIRECTION('',(2.65552944032596E-32,3.29043518662928E-48,-1.)) ;
#82419=DIRECTION('',(1.44560289664734E-16,-1.,-2.4093381610789E-16)) ;
#82420=DIRECTION('',(0.,0.,1.)) ;
#82421=DIRECTION('center_axis',(0.999999956301289,0.000282786981403369,
8.61913163653833E-5)) ;
#82422=DIRECTION('ref_axis',(0.000288266391240805,-0.997396273402903,-0.0721151211916738)) ;
#82423=DIRECTION('',(-1.44560289664734E-16,1.,-7.2280144832367E-17)) ;
#82424=DIRECTION('center_axis',(0.316227766016838,0.948683298050514,0.)) ;
#82425=DIRECTION('ref_axis',(-0.948683298050514,0.316227766016838,0.)) ;
#82426=DIRECTION('',(-0.948683298050514,0.316227766016838,0.)) ;
#82427=DIRECTION('',(0.,0.,1.)) ;
#82428=DIRECTION('',(0.937042571331636,-0.312347523777212,-0.156173761888606)) ;
#82429=DIRECTION('',(0.,0.,-1.)) ;
#82430=DIRECTION('center_axis',(1.,1.73472347597681E-15,0.)) ;
#82431=DIRECTION('ref_axis',(-1.73472347597681E-15,1.,0.)) ;
#82432=DIRECTION('',(-1.73472347597681E-15,1.,0.)) ;
#82433=DIRECTION('',(0.,0.,1.)) ;
#82434=DIRECTION('',(1.73472347597681E-15,-1.,-2.89120579329468E-16)) ;
#82435=DIRECTION('',(0.,0.,-1.)) ;
#82436=DIRECTION('center_axis',(0.164398987305357,-0.986393923832144,0.)) ;
#82437=DIRECTION('ref_axis',(0.986393923832144,0.164398987305357,0.)) ;
#82438=DIRECTION('',(-0.973328526784575,-0.162221421130762,0.162221421130763)) ;
#82439=DIRECTION('',(0.,0.,-1.)) ;
#82440=DIRECTION('',(0.986393923832144,0.164398987305357,0.)) ;
#82441=DIRECTION('',(0.,0.,1.)) ;
#82442=DIRECTION('center_axis',(-9.91270557701033E-17,1.,0.)) ;
#82443=DIRECTION('ref_axis',(-1.,-9.91270557701033E-17,0.)) ;
#82444=DIRECTION('',(1.,9.91270557701033E-17,0.)) ;
#82445=DIRECTION('',(0.,0.,-1.)) ;
#82446=DIRECTION('',(-1.,-9.91270557701033E-17,0.)) ;
#82447=DIRECTION('',(0.,0.,1.)) ;
#82448=DIRECTION('center_axis',(-9.91270557701033E-17,1.,0.)) ;
#82449=DIRECTION('ref_axis',(-1.,-9.91270557701033E-17,0.)) ;
#82450=DIRECTION('',(-1.,-9.91270557701033E-17,0.)) ;
#82451=DIRECTION('',(0.,0.,-1.)) ;
#82452=DIRECTION('',(-1.,-9.91270557701033E-17,0.)) ;
#82453=DIRECTION('',(0.,0.,1.)) ;
#82454=DIRECTION('center_axis',(1.,1.15648231731787E-15,0.)) ;
#82455=DIRECTION('ref_axis',(-1.15648231731787E-15,1.,0.)) ;
#82456=DIRECTION('',(-1.15648231731787E-15,1.,0.)) ;
#82457=DIRECTION('',(0.,0.,-1.)) ;
#82458=DIRECTION('',(-1.15648231731787E-15,1.,0.)) ;
#82459=DIRECTION('',(0.,0.,1.)) ;
#82460=DIRECTION('center_axis',(-1.,-1.15648231731787E-15,0.)) ;
#82461=DIRECTION('ref_axis',(-1.15648231731787E-15,1.,1.56060533014952E-15)) ;
#82462=DIRECTION('',(0.,0.,1.)) ;
#82463=DIRECTION('center_axis',(0.,0.,1.)) ;
#82464=DIRECTION('ref_axis',(1.,0.,0.)) ;
#82465=DIRECTION('',(-1.,0.,0.)) ;
#82466=DIRECTION('center_axis',(0.,0.,-1.)) ;
#82467=DIRECTION('ref_axis',(1.,0.,0.)) ;
#82468=DIRECTION('center_axis',(0.,0.,-1.)) ;
#82469=DIRECTION('ref_axis',(1.,0.,0.)) ;
#82470=DIRECTION('center_axis',(0.,0.,-1.)) ;
#82471=DIRECTION('ref_axis',(1.,0.,0.)) ;
#82472=DIRECTION('center_axis',(0.,0.,-1.)) ;
#82473=DIRECTION('ref_axis',(1.,0.,0.)) ;
#82474=DIRECTION('',(1.,0.,0.)) ;
#82475=DIRECTION('center_axis',(0.,0.,1.)) ;
#82476=DIRECTION('ref_axis',(1.,0.,0.)) ;
#82477=DIRECTION('',(3.46944695195361E-16,1.,0.)) ;
#82478=DIRECTION('center_axis',(0.,0.,1.)) ;
#82479=DIRECTION('ref_axis',(1.,0.,0.)) ;
#82480=DIRECTION('',(1.,-3.46944695195361E-16,0.)) ;
#82481=DIRECTION('center_axis',(0.,0.,-1.)) ;
#82482=DIRECTION('ref_axis',(1.,0.,0.)) ;
#82483=DIRECTION('',(2.71050543121376E-16,1.,0.)) ;
#82484=DIRECTION('center_axis',(0.,0.,-1.)) ;
#82485=DIRECTION('ref_axis',(1.,0.,0.)) ;
#82486=DIRECTION('',(-1.,3.46944695195361E-16,0.)) ;
#82487=DIRECTION('center_axis',(0.,0.,1.)) ;
#82488=DIRECTION('ref_axis',(1.,0.,0.)) ;
#82489=DIRECTION('',(3.46944695195361E-16,1.,0.)) ;
#82490=DIRECTION('center_axis',(0.,0.,1.)) ;
#82491=DIRECTION('ref_axis',(1.,0.,0.)) ;
#82492=DIRECTION('center_axis',(0.,0.,-1.)) ;
#82493=DIRECTION('ref_axis',(1.,0.,0.)) ;
#82494=DIRECTION('',(0.986393923832144,-0.164398987305354,0.)) ;
#82495=DIRECTION('center_axis',(0.,0.,-1.)) ;
#82496=DIRECTION('ref_axis',(1.,-6.50521303491307E-15,0.)) ;
#82497=DIRECTION('center_axis',(0.,0.,-1.)) ;
#82498=DIRECTION('ref_axis',(1.,0.,0.)) ;
#82499=DIRECTION('',(1.,0.,0.)) ;
#82500=DIRECTION('',(1.13380619344889E-16,-1.,0.)) ;
#82501=DIRECTION('center_axis',(0.,0.,-1.)) ;
#82502=DIRECTION('ref_axis',(1.,0.,0.)) ;
#82503=DIRECTION('',(-1.,-1.92747052886312E-16,0.)) ;
#82504=DIRECTION('center_axis',(0.,0.,1.)) ;
#82505=DIRECTION('ref_axis',(1.,0.,0.)) ;
#82506=DIRECTION('',(0.,-1.,0.)) ;
#82507=DIRECTION('center_axis',(0.,0.,-1.)) ;
#82508=DIRECTION('ref_axis',(1.,0.,0.)) ;
#82509=DIRECTION('center_axis',(0.,0.,1.)) ;
#82510=DIRECTION('ref_axis',(1.,0.,0.)) ;
#82511=DIRECTION('',(-0.948683298050514,0.316227766016838,0.)) ;
#82512=DIRECTION('center_axis',(0.,0.,1.)) ;
#82513=DIRECTION('ref_axis',(1.,0.,0.)) ;
#82514=DIRECTION('',(-1.,0.,0.)) ;
#82515=DIRECTION('center_axis',(0.,0.,1.)) ;
#82516=DIRECTION('ref_axis',(1.,0.,0.)) ;
#82517=DIRECTION('',(0.,-1.,0.)) ;
#82518=DIRECTION('center_axis',(0.,0.,-1.)) ;
#82519=DIRECTION('ref_axis',(1.,0.,0.)) ;
#82520=DIRECTION('',(-1.,-1.92747052886312E-16,0.)) ;
#82521=DIRECTION('center_axis',(0.,0.,1.)) ;
#82522=DIRECTION('ref_axis',(1.,0.,0.)) ;
#82523=DIRECTION('',(1.13380619344889E-16,-1.,0.)) ;
#82524=DIRECTION('',(1.,0.,0.)) ;
#82525=DIRECTION('center_axis',(0.,0.,1.)) ;
#82526=DIRECTION('ref_axis',(1.,0.,0.)) ;
#82527=DIRECTION('center_axis',(0.,0.,1.)) ;
#82528=DIRECTION('ref_axis',(1.,0.,0.)) ;
#82529=DIRECTION('',(-0.986393923832144,0.164398987305354,0.)) ;
#82530=DIRECTION('center_axis',(0.,0.,1.)) ;
#82531=DIRECTION('ref_axis',(1.,0.,0.)) ;
#82532=DIRECTION('center_axis',(0.,0.,-1.)) ;
#82533=DIRECTION('ref_axis',(1.,0.,0.)) ;
#82534=DIRECTION('',(-3.46944695195361E-16,-1.,0.)) ;
#82535=DIRECTION('center_axis',(0.,0.,-1.)) ;
#82536=DIRECTION('ref_axis',(1.,0.,0.)) ;
#82537=DIRECTION('',(-1.,3.46944695195361E-16,0.)) ;
#82538=DIRECTION('center_axis',(0.,0.,1.)) ;
#82539=DIRECTION('ref_axis',(1.,0.,0.)) ;
#82540=DIRECTION('',(3.46944695195361E-16,1.,0.)) ;
#82541=DIRECTION('center_axis',(0.,0.,1.)) ;
#82542=DIRECTION('ref_axis',(1.,0.,0.)) ;
#82543=DIRECTION('',(1.,-3.46944695195361E-16,0.)) ;
#82544=DIRECTION('center_axis',(0.,0.,-1.)) ;
#82545=DIRECTION('ref_axis',(1.,0.,0.)) ;
#82546=DIRECTION('',(-3.46944695195361E-16,-1.,0.)) ;
#82547=DIRECTION('center_axis',(0.,0.,-1.)) ;
#82548=DIRECTION('ref_axis',(1.,0.,0.)) ;
#82549=DIRECTION('',(1.,0.,0.)) ;
#82550=DIRECTION('center_axis',(0.,0.,1.)) ;
#82551=DIRECTION('ref_axis',(1.,0.,0.)) ;
#82552=DIRECTION('',(0.986393923832144,0.164398987305357,0.)) ;
#82553=DIRECTION('center_axis',(0.,0.,1.)) ;
#82554=DIRECTION('ref_axis',(1.,0.,0.)) ;
#82555=DIRECTION('',(-1.73472347597681E-15,1.,0.)) ;
#82556=DIRECTION('center_axis',(0.,0.,1.)) ;
#82557=DIRECTION('ref_axis',(1.,0.,0.)) ;
#82558=DIRECTION('center_axis',(-1.92747052886312E-16,1.,0.)) ;
#82559=DIRECTION('ref_axis',(-1.,-1.92747052886312E-16,0.)) ;
#82560=DIRECTION('',(0.,0.,1.)) ;
#82561=DIRECTION('',(0.,0.,-1.)) ;
#82562=DIRECTION('center_axis',(-1.,0.,0.)) ;
#82563=DIRECTION('ref_axis',(0.,0.,1.)) ;
#82564=DIRECTION('',(0.,0.,1.)) ;
#82565=DIRECTION('',(0.,0.,-1.)) ;
#82566=DIRECTION('center_axis',(0.,1.,0.)) ;
#82567=DIRECTION('ref_axis',(0.,0.,1.)) ;
#82568=DIRECTION('',(0.,0.,-1.)) ;
#82569=DIRECTION('',(0.,0.,1.)) ;
#82570=DIRECTION('',(0.,0.,-1.)) ;
#82571=DIRECTION('',(0.,0.,-1.)) ;
#82572=DIRECTION('center_axis',(0.316227766016838,0.948683298050514,0.)) ;
#82573=DIRECTION('ref_axis',(-0.948683298050514,0.316227766016838,0.)) ;
#82574=DIRECTION('center_axis',(-0.316227766016835,-0.948683298050515,3.34717459363351E-14)) ;
#82575=DIRECTION('ref_axis',(0.831595960764329,-0.277198653588124,-0.481257794211568)) ;
#82576=DIRECTION('',(0.,0.,1.)) ;
#82577=DIRECTION('',(0.,0.,-1.)) ;
#82578=DIRECTION('',(-0.937042571331636,0.312347523777212,-0.156173761888606)) ;
#82579=DIRECTION('center_axis',(1.,1.73472347597681E-15,0.)) ;
#82580=DIRECTION('ref_axis',(-1.73472347597681E-15,1.,0.)) ;
#82581=DIRECTION('',(-1.73472347597681E-15,1.,-2.89120579329468E-16)) ;
#82582=DIRECTION('',(0.,0.,1.)) ;
#82583=DIRECTION('',(0.,0.,-1.)) ;
#82584=DIRECTION('center_axis',(0.164398987305357,-0.986393923832144,0.)) ;
#82585=DIRECTION('ref_axis',(0.986393923832144,0.164398987305357,0.)) ;
#82586=DIRECTION('',(0.973328526784575,0.162221421130762,0.162221421130763)) ;
#82587=DIRECTION('',(0.,0.,1.)) ;
#82588=DIRECTION('',(0.,0.,-1.)) ;
#82589=DIRECTION('center_axis',(0.,-1.,0.)) ;
#82590=DIRECTION('ref_axis',(0.,0.,-1.)) ;
#82591=DIRECTION('',(0.,0.,1.)) ;
#82592=DIRECTION('',(0.,0.,1.)) ;
#82593=DIRECTION('',(0.,0.,1.)) ;
#82594=DIRECTION('',(0.,0.,-1.)) ;
#82595=DIRECTION('',(1.,0.,2.25271179641597E-31)) ;
#82596=DIRECTION('center_axis',(0.,-1.,0.)) ;
#82597=DIRECTION('ref_axis',(0.,0.,-1.)) ;
#82598=DIRECTION('',(0.,0.,-1.)) ;
#82599=DIRECTION('center_axis',(0.,-1.,0.)) ;
#82600=DIRECTION('ref_axis',(0.,0.,-1.)) ;
#82601=DIRECTION('',(-1.,0.,-3.21815970916568E-32)) ;
#82602=DIRECTION('',(0.,0.,-1.)) ;
#82603=DIRECTION('center_axis',(1.,-3.46944695195361E-16,0.)) ;
#82604=DIRECTION('ref_axis',(3.46944695195361E-16,1.,0.)) ;
#82605=DIRECTION('center_axis',(1.,-3.46944695195361E-16,0.)) ;
#82606=DIRECTION('ref_axis',(3.46944695195361E-16,1.,0.)) ;
#82607=DIRECTION('',(1.5529910948782E-31,4.47619207437002E-16,-1.)) ;
#82608=DIRECTION('',(0.,0.,1.)) ;
#82609=DIRECTION('center_axis',(1.,-3.46944695195361E-16,0.)) ;
#82610=DIRECTION('ref_axis',(3.46944695195361E-16,1.,0.)) ;
#82611=DIRECTION('center_axis',(1.,-3.46944695195361E-16,0.)) ;
#82612=DIRECTION('ref_axis',(3.46944695195361E-16,1.,0.)) ;
#82613=DIRECTION('center_axis',(1.,-3.46944695195361E-16,0.)) ;
#82614=DIRECTION('ref_axis',(3.46944695195361E-16,1.,0.)) ;
#82615=DIRECTION('',(3.46944695195361E-16,1.,9.27571383489107E-17)) ;
#82616=DIRECTION('',(0.,0.,1.)) ;
#82617=DIRECTION('',(-3.46944695195361E-16,-1.,-6.49299968442375E-16)) ;
#82618=DIRECTION('center_axis',(1.,-3.46944695195361E-16,0.)) ;
#82619=DIRECTION('ref_axis',(3.46944695195361E-16,1.,0.)) ;
#82620=DIRECTION('center_axis',(1.,-3.46944695195361E-16,0.)) ;
#82621=DIRECTION('ref_axis',(3.46944695195361E-16,1.,0.)) ;
#82622=DIRECTION('center_axis',(1.,-3.46944695195361E-16,0.)) ;
#82623=DIRECTION('ref_axis',(3.46944695195361E-16,1.,0.)) ;
#82624=DIRECTION('',(0.,0.,1.)) ;
#82625=DIRECTION('',(-1.5529910948782E-31,-4.47619207437002E-16,-1.)) ;
#82626=DIRECTION('center_axis',(1.,-3.46944695195361E-16,0.)) ;
#82627=DIRECTION('ref_axis',(3.46944695195361E-16,1.,0.)) ;
#82628=DIRECTION('center_axis',(1.,-3.46944695195361E-16,0.)) ;
#82629=DIRECTION('ref_axis',(3.46944695195361E-16,1.,0.)) ;
#82630=DIRECTION('center_axis',(1.,-3.46944695195361E-16,0.)) ;
#82631=DIRECTION('ref_axis',(3.46944695195361E-16,1.,0.)) ;
#82632=DIRECTION('',(-3.46944695195361E-16,-1.,-1.06487173641454E-15)) ;
#82633=DIRECTION('center_axis',(1.,-3.46944695195361E-16,0.)) ;
#82634=DIRECTION('ref_axis',(3.46944695195361E-16,1.,0.)) ;
#82635=DIRECTION('',(3.46944695195361E-16,1.,2.45739631480277E-16)) ;
#82636=DIRECTION('center_axis',(1.,-3.46944695195361E-16,0.)) ;
#82637=DIRECTION('ref_axis',(3.46944695195361E-16,1.,0.)) ;
#82638=DIRECTION('center_axis',(1.,-3.46944695195361E-16,0.)) ;
#82639=DIRECTION('ref_axis',(3.46944695195361E-16,1.,0.)) ;
#82640=DIRECTION('center_axis',(0.,-1.,0.)) ;
#82641=DIRECTION('ref_axis',(0.,0.,-1.)) ;
#82642=DIRECTION('center_axis',(0.,-1.,0.)) ;
#82643=DIRECTION('ref_axis',(0.,0.,-1.)) ;
#82644=DIRECTION('',(-1.,0.,-1.40488587213121E-32)) ;
#82645=DIRECTION('',(0.,0.,1.)) ;
#82646=DIRECTION('',(0.,0.,1.)) ;
#82647=DIRECTION('',(0.,0.,1.)) ;
#82648=DIRECTION('',(1.,0.,1.40488587213121E-32)) ;
#82649=DIRECTION('center_axis',(0.,-1.,0.)) ;
#82650=DIRECTION('ref_axis',(0.,0.,-1.)) ;
#82651=DIRECTION('',(7.2280144832367E-17,0.,-1.)) ;
#82652=DIRECTION('center_axis',(-1.,-1.13380619344889E-16,0.)) ;
#82653=DIRECTION('ref_axis',(1.13380619344889E-16,-1.,0.)) ;
#82654=DIRECTION('center_axis',(-1.,-1.13380619344889E-16,0.)) ;
#82655=DIRECTION('ref_axis',(1.13380619344889E-16,-1.,0.)) ;
#82656=DIRECTION('',(1.13380619344889E-16,-1.,1.23908819712629E-16)) ;
#82657=DIRECTION('',(0.,0.,-1.)) ;
#82658=DIRECTION('',(-1.13380619344889E-16,1.,-1.23908819712629E-16)) ;
#82659=DIRECTION('center_axis',(-1.,-1.13380619344889E-16,0.)) ;
#82660=DIRECTION('ref_axis',(1.13380619344889E-16,-1.,0.)) ;
#82661=DIRECTION('',(0.,0.,1.)) ;
#82662=DIRECTION('center_axis',(-1.40488587213121E-32,1.23908819712629E-16,
1.)) ;
#82663=DIRECTION('ref_axis',(0.,-1.,1.23908819712629E-16)) ;
#82664=DIRECTION('',(-1.,0.,-1.40488587213121E-32)) ;
#82665=DIRECTION('',(-1.13380619344889E-16,1.,-1.23908819712629E-16)) ;
#82666=DIRECTION('center_axis',(1.40488587213121E-32,-1.23908819712629E-16,
-1.)) ;
#82667=DIRECTION('ref_axis',(-1.74077750246726E-48,-1.,1.23908819712629E-16)) ;
#82668=DIRECTION('center_axis',(1.40488587213121E-32,-1.23908819712629E-16,
-1.)) ;
#82669=DIRECTION('ref_axis',(0.,1.,-1.23908819712629E-16)) ;
#82670=DIRECTION('center_axis',(-1.40488587213121E-32,1.23908819712629E-16,
1.)) ;
#82671=DIRECTION('ref_axis',(1.74077750246726E-48,1.,-1.23908819712629E-16)) ;
#82672=DIRECTION('',(1.13380619344889E-16,-1.,1.23908819712629E-16)) ;
#82673=DIRECTION('',(1.,0.,1.40488587213121E-32)) ;
#82674=DIRECTION('center_axis',(-1.,-1.23908819712629E-16,-8.95614743483648E-33)) ;
#82675=DIRECTION('ref_axis',(1.23908819712629E-16,-1.,5.38566640001825E-66)) ;
#82676=DIRECTION('',(-8.95614743483648E-33,-1.10974565782288E-48,1.)) ;
#82677=DIRECTION('',(1.23908819712629E-16,-1.,7.2280144832367E-17)) ;
#82678=DIRECTION('',(-8.95614743483648E-33,0.,1.)) ;
#82679=DIRECTION('',(-1.23908819712629E-16,1.,-1.23908819712629E-16)) ;
#82680=DIRECTION('',(8.95614743483648E-33,1.0154535431059E-48,-1.)) ;
#82681=DIRECTION('',(1.23908819712629E-16,-1.,1.23908819712629E-16)) ;
#82682=DIRECTION('',(-8.95614743483648E-33,0.,1.)) ;
#82683=DIRECTION('',(-1.23908819712629E-16,1.,2.4093381610789E-16)) ;
#82684=DIRECTION('center_axis',(-1.7912294869673E-32,7.2280144832367E-17,
1.)) ;
#82685=DIRECTION('ref_axis',(0.,-1.,7.2280144832367E-17)) ;
#82686=DIRECTION('',(-1.23908819712629E-16,1.,-7.2280144832367E-17)) ;
#82687=DIRECTION('',(1.,1.23908819712629E-16,8.95614743483648E-33)) ;
#82688=DIRECTION('',(1.44560289664734E-16,-1.,7.2280144832367E-17)) ;
#82689=DIRECTION('',(-1.,0.,-1.7912294869673E-32)) ;
#82690=DIRECTION('center_axis',(-2.08976773479518E-32,2.4093381610789E-16,
-1.)) ;
#82691=DIRECTION('ref_axis',(0.,1.,2.4093381610789E-16)) ;
#82692=DIRECTION('',(-1.44560289664734E-16,1.,2.4093381610789E-16)) ;
#82693=DIRECTION('',(-1.,-1.23908819712629E-16,-8.95614743483648E-33)) ;
#82694=DIRECTION('',(1.23908819712629E-16,-1.,-2.4093381610789E-16)) ;
#82695=DIRECTION('',(1.,0.,-2.08976773479518E-32)) ;
#82696=DIRECTION('center_axis',(-1.23908819712629E-16,1.,0.)) ;
#82697=DIRECTION('ref_axis',(-1.,-1.23908819712629E-16,0.)) ;
#82698=DIRECTION('',(8.95614743483648E-33,1.10974565782288E-48,-1.)) ;
#82699=DIRECTION('',(1.,1.23908819712629E-16,8.95614743483648E-33)) ;
#82700=DIRECTION('',(-2.65552944032596E-32,-3.29043518662928E-48,1.)) ;
#82701=DIRECTION('',(-1.,-1.23908819712629E-16,-8.95614743483648E-33)) ;
#82702=DIRECTION('center_axis',(-1.,-1.44560289664734E-16,-2.65552944032596E-32)) ;
#82703=DIRECTION('ref_axis',(1.44560289664734E-16,-1.,-2.80018320648271E-64)) ;
#82704=DIRECTION('',(1.44560289664734E-16,-1.,-2.4093381610789E-16)) ;
#82705=DIRECTION('',(-2.65552944032596E-32,0.,1.)) ;
#82706=DIRECTION('',(-1.44560289664734E-16,1.,-7.2280144832367E-17)) ;
#82707=DIRECTION('',(0.,0.,-1.)) ;
#82708=DIRECTION('center_axis',(0.,1.,0.)) ;
#82709=DIRECTION('ref_axis',(0.,0.,1.)) ;
#82710=DIRECTION('',(8.95614743483648E-33,0.,-1.)) ;
#82711=DIRECTION('',(1.,0.,1.40488587213121E-32)) ;
#82712=DIRECTION('',(-7.2280144832367E-17,0.,1.)) ;
#82713=DIRECTION('',(-1.,0.,-1.40488587213121E-32)) ;
#82714=DIRECTION('',(8.95614743483648E-33,0.,-1.)) ;
#82715=DIRECTION('',(1.,0.,1.7912294869673E-32)) ;
#82716=DIRECTION('',(2.65552944032596E-32,0.,-1.)) ;
#82717=DIRECTION('',(-1.,0.,2.08976773479518E-32)) ;
#82718=DIRECTION('center_axis',(1.,1.44560289664734E-16,0.)) ;
#82719=DIRECTION('ref_axis',(-1.44560289664734E-16,1.,0.)) ;
#82720=DIRECTION('',(1.44560289664734E-16,-1.,0.)) ;
#82721=DIRECTION('center_axis',(-1.,-1.44560289664734E-16,0.)) ;
#82722=DIRECTION('ref_axis',(-1.44560289664734E-16,1.,0.)) ;
#82723=DIRECTION('',(0.,0.,-1.)) ;
#82724=DIRECTION('center_axis',(-1.,-1.44560289664734E-16,0.)) ;
#82725=DIRECTION('ref_axis',(-1.44560289664734E-16,1.,0.)) ;
#82726=DIRECTION('',(1.44560289664734E-16,-1.,0.)) ;
#82727=DIRECTION('center_axis',(-1.,-1.44560289664734E-16,0.)) ;
#82728=DIRECTION('ref_axis',(-1.44560289664734E-16,1.,0.)) ;
#82729=DIRECTION('',(0.,0.,1.)) ;
#82730=DIRECTION('center_axis',(-1.,-1.44560289664734E-16,0.)) ;
#82731=DIRECTION('ref_axis',(-1.44560289664734E-16,1.,0.)) ;
#82732=DIRECTION('center_axis',(1.,-3.46944695195361E-16,0.)) ;
#82733=DIRECTION('ref_axis',(3.46944695195361E-16,1.,0.)) ;
#82734=DIRECTION('center_axis',(1.,-3.46944695195361E-16,0.)) ;
#82735=DIRECTION('ref_axis',(3.46944695195361E-16,1.,0.)) ;
#82736=DIRECTION('',(0.,0.,-1.)) ;
#82737=DIRECTION('',(-1.5529910948782E-31,-4.47619207437002E-16,1.)) ;
#82738=DIRECTION('center_axis',(-1.,3.46944695195361E-16,0.)) ;
#82739=DIRECTION('ref_axis',(3.46944695195361E-16,1.,0.)) ;
#82740=DIRECTION('',(-3.46944695195361E-16,-1.,-2.45739631480277E-16)) ;
#82741=DIRECTION('center_axis',(1.,-3.46944695195361E-16,0.)) ;
#82742=DIRECTION('ref_axis',(3.46944695195361E-16,1.,0.)) ;
#82743=DIRECTION('center_axis',(3.46944695195361E-16,1.,4.47619207437002E-16)) ;
#82744=DIRECTION('ref_axis',(-8.18685017503995E-48,-4.47619207437002E-16,
1.)) ;
#82745=DIRECTION('',(-1.5529910948782E-31,-4.47619207437002E-16,1.)) ;
#82746=DIRECTION('',(-1.,3.46944695195361E-16,0.)) ;
#82747=DIRECTION('',(1.5529910948782E-31,4.47619207437002E-16,-1.)) ;
#82748=DIRECTION('center_axis',(-8.52580615413453E-32,-2.45739631480277E-16,
1.)) ;
#82749=DIRECTION('ref_axis',(0.,-1.,-2.45739631480277E-16)) ;
#82750=DIRECTION('',(1.,-3.46944695195361E-16,0.)) ;
#82751=DIRECTION('',(-3.46944695195361E-16,-1.,-2.45739631480277E-16)) ;
#82752=DIRECTION('',(3.46944695195361E-16,1.,2.45739631480277E-16)) ;
#82753=DIRECTION('center_axis',(1.,-3.46944695195361E-16,0.)) ;
#82754=DIRECTION('ref_axis',(3.46944695195361E-16,1.,0.)) ;
#82755=DIRECTION('center_axis',(1.,-3.46944695195361E-16,0.)) ;
#82756=DIRECTION('ref_axis',(3.46944695195361E-16,1.,0.)) ;
#82757=DIRECTION('',(1.,-3.46944695195361E-16,0.)) ;
#82758=DIRECTION('center_axis',(-1.,3.46944695195361E-16,0.)) ;
#82759=DIRECTION('ref_axis',(3.46944695195361E-16,1.,0.)) ;
#82760=DIRECTION('',(-1.,3.46944695195361E-16,0.)) ;
#82761=DIRECTION('center_axis',(1.,-3.46944695195361E-16,0.)) ;
#82762=DIRECTION('ref_axis',(3.46944695195361E-16,1.,0.)) ;
#82763=DIRECTION('center_axis',(1.,-3.46944695195361E-16,0.)) ;
#82764=DIRECTION('ref_axis',(-3.46944695195361E-16,-1.,-9.91270557701033E-16)) ;
#82765=DIRECTION('',(1.,-3.46944695195361E-16,0.)) ;
#82766=DIRECTION('center_axis',(-1.,3.46944695195361E-16,0.)) ;
#82767=DIRECTION('ref_axis',(3.46944695195361E-16,1.,-1.98254111540207E-15)) ;
#82768=DIRECTION('',(-1.,3.46944695195361E-16,0.)) ;
#82769=DIRECTION('center_axis',(3.69451600012496E-31,1.06487173641454E-15,
-1.)) ;
#82770=DIRECTION('ref_axis',(0.,1.,1.06487173641454E-15)) ;
#82771=DIRECTION('',(3.46944695195361E-16,1.,1.06487173641454E-15)) ;
#82772=DIRECTION('',(-1.,3.46944695195361E-16,0.)) ;
#82773=DIRECTION('',(-3.46944695195361E-16,-1.,-1.06487173641454E-15)) ;
#82774=DIRECTION('center_axis',(3.46944695195361E-16,1.,-4.47619207437002E-16)) ;
#82775=DIRECTION('ref_axis',(8.18685017503995E-48,4.47619207437002E-16,
1.)) ;
#82776=DIRECTION('',(1.,-3.46944695195361E-16,0.)) ;
#82777=DIRECTION('',(1.5529910948782E-31,4.47619207437002E-16,1.)) ;
#82778=DIRECTION('',(-1.5529910948782E-31,-4.47619207437002E-16,-1.)) ;
#82779=DIRECTION('center_axis',(-1.,3.46944695195361E-16,0.)) ;
#82780=DIRECTION('ref_axis',(-3.46944695195361E-16,-1.,0.)) ;
#82781=DIRECTION('center_axis',(-1.,3.46944695195361E-16,0.)) ;
#82782=DIRECTION('ref_axis',(-3.46944695195361E-16,-1.,0.)) ;
#82783=DIRECTION('',(1.5529910948782E-31,4.47619207437002E-16,1.)) ;
#82784=DIRECTION('',(0.,0.,-1.)) ;
#82785=DIRECTION('center_axis',(1.,-3.46944695195361E-16,0.)) ;
#82786=DIRECTION('ref_axis',(-3.46944695195361E-16,-1.,0.)) ;
#82787=DIRECTION('center_axis',(1.,-3.46944695195361E-16,0.)) ;
#82788=DIRECTION('ref_axis',(-3.46944695195361E-16,-1.,0.)) ;
#82789=DIRECTION('',(3.46944695195361E-16,1.,1.06487173641454E-15)) ;
#82790=DIRECTION('center_axis',(1.,-3.46944695195361E-16,0.)) ;
#82791=DIRECTION('ref_axis',(3.46944695195361E-16,1.,0.)) ;
#82792=DIRECTION('center_axis',(-1.,3.46944695195361E-16,0.)) ;
#82793=DIRECTION('ref_axis',(3.46944695195361E-16,1.,0.)) ;
#82794=DIRECTION('',(0.,0.,-1.)) ;
#82795=DIRECTION('',(0.,0.,1.)) ;
#82796=DIRECTION('',(-3.46944695195361E-16,-1.,-9.27571383489107E-17)) ;
#82797=DIRECTION('center_axis',(-3.46944695195361E-16,-1.,0.)) ;
#82798=DIRECTION('ref_axis',(1.,-3.46944695195361E-16,0.)) ;
#82799=DIRECTION('',(1.,-3.46944695195361E-16,0.)) ;
#82800=DIRECTION('',(0.,0.,-1.)) ;
#82801=DIRECTION('',(0.,0.,1.)) ;
#82802=DIRECTION('center_axis',(1.,-3.46944695195361E-16,0.)) ;
#82803=DIRECTION('ref_axis',(3.46944695195361E-16,1.,0.)) ;
#82804=DIRECTION('center_axis',(1.,-3.46944695195361E-16,0.)) ;
#82805=DIRECTION('ref_axis',(3.46944695195361E-16,1.,0.)) ;
#82806=DIRECTION('',(1.,-3.46944695195361E-16,0.)) ;
#82807=DIRECTION('center_axis',(-1.,3.46944695195361E-16,0.)) ;
#82808=DIRECTION('ref_axis',(3.46944695195361E-16,1.,-9.91270557701033E-16)) ;
#82809=DIRECTION('',(-1.,3.46944695195361E-16,0.)) ;
#82810=DIRECTION('center_axis',(-3.21815970916568E-32,-9.27571383489107E-17,
1.)) ;
#82811=DIRECTION('ref_axis',(0.,-1.,-9.27571383489107E-17)) ;
#82812=DIRECTION('',(3.46944695195361E-16,1.,9.27571383489107E-17)) ;
#82813=DIRECTION('',(1.,0.,3.21815970916568E-32)) ;
#82814=DIRECTION('',(-3.46944695195361E-16,-1.,-9.27571383489107E-17)) ;
#82815=DIRECTION('',(-1.,3.46944695195361E-16,0.)) ;
#82816=DIRECTION('center_axis',(1.,-3.46944695195361E-16,0.)) ;
#82817=DIRECTION('ref_axis',(3.46944695195361E-16,1.,0.)) ;
#82818=DIRECTION('center_axis',(1.,-3.46944695195361E-16,0.)) ;
#82819=DIRECTION('ref_axis',(-3.46944695195361E-16,-1.,4.95635278850516E-15)) ;
#82820=DIRECTION('',(1.,-3.46944695195361E-16,0.)) ;
#82821=DIRECTION('center_axis',(-1.,3.46944695195361E-16,0.)) ;
#82822=DIRECTION('ref_axis',(3.46944695195361E-16,1.,2.9738116731031E-15)) ;
#82823=DIRECTION('',(-1.,3.46944695195361E-16,0.)) ;
#82824=DIRECTION('center_axis',(-3.46944695195361E-16,-1.,0.)) ;
#82825=DIRECTION('ref_axis',(1.,-3.46944695195361E-16,0.)) ;
#82826=DIRECTION('',(0.,0.,-1.)) ;
#82827=DIRECTION('',(-1.,3.46944695195361E-16,0.)) ;
#82828=DIRECTION('',(0.,0.,1.)) ;
#82829=DIRECTION('center_axis',(2.25271179641597E-31,6.49299968442375E-16,
-1.)) ;
#82830=DIRECTION('ref_axis',(0.,1.,6.49299968442375E-16)) ;
#82831=DIRECTION('',(3.46944695195361E-16,1.,6.49299968442375E-16)) ;
#82832=DIRECTION('',(-1.,0.,-2.25271179641597E-31)) ;
#82833=DIRECTION('',(-3.46944695195361E-16,-1.,-6.49299968442375E-16)) ;
#82834=DIRECTION('',(1.,-3.46944695195361E-16,0.)) ;
#82835=DIRECTION('center_axis',(-1.,3.46944695195361E-16,0.)) ;
#82836=DIRECTION('ref_axis',(-3.46944695195361E-16,-1.,0.)) ;
#82837=DIRECTION('',(3.46944695195361E-16,1.,6.49299968442375E-16)) ;
#82838=DIRECTION('',(0.,0.,1.)) ;
#82839=DIRECTION('',(0.,0.,-1.)) ;
#82840=DIRECTION('center_axis',(-1.,3.46944695195361E-16,0.)) ;
#82841=DIRECTION('ref_axis',(-3.46944695195361E-16,-1.,0.)) ;
#82842=DIRECTION('center_axis',(-0.164398987305357,0.,-0.986393923832144)) ;
#82843=DIRECTION('ref_axis',(-0.986393923832144,0.,0.164398987305357)) ;
#82844=DIRECTION('',(-0.937042571331636,0.312347523777212,0.156173761888606)) ;
#82845=DIRECTION('',(0.,-1.,0.)) ;
#82846=DIRECTION('',(0.973328526784575,0.162221421130762,-0.162221421130763)) ;
#82847=DIRECTION('',(-1.73472347597681E-15,1.,2.89120579329468E-16)) ;
#82848=DIRECTION('center_axis',(-1.,0.,0.)) ;
#82849=DIRECTION('ref_axis',(0.,0.,1.)) ;
#82850=DIRECTION('center_axis',(-1.,0.,0.)) ;
#82851=DIRECTION('ref_axis',(0.,0.958782008217047,-0.284142676694803)) ;
#82852=DIRECTION('',(0.,0.,1.)) ;
#82853=DIRECTION('',(0.,-1.,0.)) ;
#82854=DIRECTION('center_axis',(-1.,0.,0.)) ;
#82855=DIRECTION('ref_axis',(0.,0.75870512941688,-0.651434207419687)) ;
#82856=DIRECTION('',(0.,0.,-1.)) ;
#82857=DIRECTION('center_axis',(-1.,0.,0.)) ;
#82858=DIRECTION('ref_axis',(0.,-0.65477883641065,-0.755820531203483)) ;
#82859=DIRECTION('',(0.,1.,0.)) ;
#82860=DIRECTION('center_axis',(-0.164398987305357,0.,0.986393923832144)) ;
#82861=DIRECTION('ref_axis',(0.986393923832144,0.,0.164398987305357)) ;
#82862=DIRECTION('',(-0.973328526784575,-0.162221421130762,-0.162221421130763)) ;
#82863=DIRECTION('',(0.,1.,0.)) ;
#82864=DIRECTION('',(0.937042571331636,-0.312347523777212,0.156173761888606)) ;
#82865=DIRECTION('',(1.73472347597681E-15,-1.,2.89120579329468E-16)) ;
#82866=DIRECTION('center_axis',(-0.573462344363329,0.81923192051904,0.)) ;
#82867=DIRECTION('ref_axis',(-0.81923192051904,-0.573462344363329,0.)) ;
#82868=DIRECTION('',(-0.710669054518702,-0.497468338163091,0.49746833816309)) ;
#82869=DIRECTION('',(0.,0.,-1.)) ;
#82870=DIRECTION('',(0.710669054518702,0.497468338163091,0.49746833816309)) ;
#82871=DIRECTION('',(0.,0.,1.)) ;
#82872=DIRECTION('center_axis',(-1.,0.,0.)) ;
#82873=DIRECTION('ref_axis',(0.,0.,1.)) ;
#82874=DIRECTION('',(0.,0.,1.)) ;
#82875=DIRECTION('',(0.,-1.,-9.34081871679819E-17)) ;
#82876=DIRECTION('',(0.,0.,-1.)) ;
#82877=DIRECTION('',(0.,1.,-9.34081871679819E-17)) ;
#82878=DIRECTION('center_axis',(-0.573462344363329,-0.81923192051904,0.)) ;
#82879=DIRECTION('ref_axis',(0.81923192051904,-0.573462344363329,0.)) ;
#82880=DIRECTION('',(-0.710669054518701,0.497468338163091,-0.497468338163091)) ;
#82881=DIRECTION('',(0.,0.,1.)) ;
#82882=DIRECTION('',(0.710669054518701,-0.497468338163091,-0.497468338163091)) ;
#82883=DIRECTION('',(0.,0.,-1.)) ;
#82884=DIRECTION('center_axis',(0.,0.,1.)) ;
#82885=DIRECTION('ref_axis',(1.,0.,0.)) ;
#82886=DIRECTION('',(1.,6.67201336914158E-17,0.)) ;
#82887=DIRECTION('',(1.33440267382831E-16,1.,0.)) ;
#82888=DIRECTION('',(-1.,1.33440267382831E-16,0.)) ;
#82889=DIRECTION('center_axis',(0.,0.,1.)) ;
#82890=DIRECTION('ref_axis',(1.,0.,0.)) ;
#82891=DIRECTION('',(1.,-1.33440267382831E-16,0.)) ;
#82892=DIRECTION('',(-1.33440267382831E-16,-1.,0.)) ;
#82893=DIRECTION('',(-1.,-6.67201336914158E-17,0.)) ;
#82894=DIRECTION('center_axis',(-6.67201336914158E-17,1.,0.)) ;
#82895=DIRECTION('ref_axis',(-1.,-6.67201336914158E-17,0.)) ;
#82896=DIRECTION('',(1.,6.67201336914158E-17,0.)) ;
#82897=DIRECTION('',(0.,0.,1.)) ;
#82898=DIRECTION('',(-1.,-6.67201336914158E-17,0.)) ;
#82899=DIRECTION('center_axis',(-1.33440267382831E-16,-1.,0.)) ;
#82900=DIRECTION('ref_axis',(1.,-1.33440267382831E-16,0.)) ;
#82901=DIRECTION('',(1.,-1.33440267382831E-16,0.)) ;
#82902=DIRECTION('',(0.,0.,-1.)) ;
#82903=DIRECTION('',(-1.,1.33440267382831E-16,0.)) ;
#82904=DIRECTION('center_axis',(0.,0.,1.)) ;
#82905=DIRECTION('ref_axis',(1.,0.,0.)) ;
#82906=DIRECTION('',(0.,-1.,0.)) ;
#82907=DIRECTION('',(1.,0.,0.)) ;
#82908=DIRECTION('',(0.,1.,0.)) ;
#82909=DIRECTION('center_axis',(0.,0.,-1.)) ;
#82910=DIRECTION('ref_axis',(1.,0.,0.)) ;
#82911=DIRECTION('',(-1.44560289664734E-16,1.,-7.2280144832367E-17)) ;
#82912=DIRECTION('center_axis',(0.,0.,1.)) ;
#82913=DIRECTION('ref_axis',(1.,0.,0.)) ;
#82914=DIRECTION('center_axis',(0.,0.,1.)) ;
#82915=DIRECTION('ref_axis',(1.,0.,0.)) ;
#82916=DIRECTION('',(0.,-1.,0.)) ;
#82917=DIRECTION('',(-1.,0.,0.)) ;
#82918=DIRECTION('',(0.,1.,0.)) ;
#82919=DIRECTION('center_axis',(0.,0.,-1.)) ;
#82920=DIRECTION('ref_axis',(1.,-1.82602471155453E-15,0.)) ;
#82921=DIRECTION('',(1.44560289664734E-16,-1.,-2.4093381610789E-16)) ;
#82922=DIRECTION('center_axis',(0.,0.,1.)) ;
#82923=DIRECTION('ref_axis',(1.,0.,0.)) ;
#82924=DIRECTION('center_axis',(0.,0.,-1.)) ;
#82925=DIRECTION('ref_axis',(-1.,0.,0.)) ;
#82926=DIRECTION('',(0.,0.,-1.)) ;
#82927=DIRECTION('center_axis',(0.,0.,-1.)) ;
#82928=DIRECTION('ref_axis',(1.,0.,0.)) ;
#82929=DIRECTION('center_axis',(0.,0.,1.)) ;
#82930=DIRECTION('ref_axis',(1.,0.,0.)) ;
#82931=DIRECTION('center_axis',(1.,0.,0.)) ;
#82932=DIRECTION('ref_axis',(0.,0.,-1.)) ;
#82933=DIRECTION('',(0.,-1.,0.)) ;
#82934=DIRECTION('',(0.,0.,1.)) ;
#82935=DIRECTION('',(0.,1.,0.)) ;
#82936=DIRECTION('center_axis',(0.81923192051904,0.573462344363329,0.)) ;
#82937=DIRECTION('ref_axis',(-0.573462344363329,0.81923192051904,0.)) ;
#82938=DIRECTION('',(-0.497468338163091,0.710669054518701,0.497468338163091)) ;
#82939=DIRECTION('',(0.,0.,-1.)) ;
#82940=DIRECTION('',(0.497468338163091,-0.710669054518701,0.497468338163091)) ;
#82941=DIRECTION('',(0.,0.,1.)) ;
#82942=DIRECTION('center_axis',(0.,1.,0.)) ;
#82943=DIRECTION('ref_axis',(0.,0.,1.)) ;
#82944=DIRECTION('',(0.,0.,1.)) ;
#82945=DIRECTION('',(-1.,0.,0.)) ;
#82946=DIRECTION('',(0.,0.,-1.)) ;
#82947=DIRECTION('',(1.,0.,0.)) ;
#82948=DIRECTION('center_axis',(-0.81923192051904,0.573462344363329,0.)) ;
#82949=DIRECTION('ref_axis',(-0.573462344363329,-0.81923192051904,0.)) ;
#82950=DIRECTION('',(0.497468338163091,0.710669054518701,-0.497468338163091)) ;
#82951=DIRECTION('',(0.,0.,1.)) ;
#82952=DIRECTION('',(-0.497468338163091,-0.710669054518701,-0.497468338163091)) ;
#82953=DIRECTION('',(0.,0.,-1.)) ;
#82954=DIRECTION('center_axis',(-1.,0.,0.)) ;
#82955=DIRECTION('ref_axis',(0.,0.,1.)) ;
#82956=DIRECTION('',(0.,-1.,0.)) ;
#82957=DIRECTION('',(0.,0.,-1.)) ;
#82958=DIRECTION('',(0.,1.,0.)) ;
#82959=DIRECTION('',(0.,0.,-1.)) ;
#82960=DIRECTION('center_axis',(0.,0.,-1.)) ;
#82961=DIRECTION('ref_axis',(-1.,0.,0.)) ;
#82962=DIRECTION('center_axis',(0.,0.,1.)) ;
#82963=DIRECTION('ref_axis',(1.,0.,0.)) ;
#82964=DIRECTION('center_axis',(0.,0.,-1.)) ;
#82965=DIRECTION('ref_axis',(1.,5.20417042793042E-15,0.)) ;
#82966=DIRECTION('center_axis',(-0.573462344363328,7.65229685658278E-17,
0.819231920519041)) ;
#82967=DIRECTION('ref_axis',(0.819231920519041,1.22423955297878E-32,0.573462344363328)) ;
#82968=DIRECTION('',(-0.710669054518702,-0.497468338163091,-0.497468338163091)) ;
#82969=DIRECTION('',(1.33440267382831E-16,1.,-2.91413396387194E-34)) ;
#82970=DIRECTION('',(0.710669054518701,-0.497468338163091,0.497468338163091)) ;
#82971=DIRECTION('',(5.04890651880155E-33,-1.,9.34081871679819E-17)) ;
#82972=DIRECTION('center_axis',(-0.573462344363328,7.65229685658278E-17,
-0.819231920519041)) ;
#82973=DIRECTION('ref_axis',(-0.819231920519041,-1.22423955297878E-32,0.573462344363328)) ;
#82974=DIRECTION('',(-0.710669054518701,0.497468338163091,0.497468338163091)) ;
#82975=DIRECTION('',(-1.33440267382831E-16,-1.,7.77328292223541E-33)) ;
#82976=DIRECTION('',(0.710669054518702,0.497468338163091,-0.497468338163091)) ;
#82977=DIRECTION('',(-5.04890651880155E-33,1.,9.34081871679819E-17)) ;
#82978=DIRECTION('center_axis',(0.,0.573462344363328,-0.819231920519041)) ;
#82979=DIRECTION('ref_axis',(0.,0.819231920519041,0.573462344363328)) ;
#82980=DIRECTION('',(0.497468338163091,0.710669054518701,0.497468338163091)) ;
#82981=DIRECTION('',(-1.,0.,0.)) ;
#82982=DIRECTION('',(0.497468338163091,-0.710669054518701,-0.497468338163091)) ;
#82983=DIRECTION('',(1.,0.,0.)) ;
#82984=DIRECTION('center_axis',(0.,0.573462344363328,0.819231920519041)) ;
#82985=DIRECTION('ref_axis',(0.,-0.819231920519041,0.573462344363328)) ;
#82986=DIRECTION('',(-0.497468338163091,0.710669054518701,-0.497468338163091)) ;
#82987=DIRECTION('',(1.,0.,0.)) ;
#82988=DIRECTION('',(-0.497468338163091,-0.710669054518701,0.497468338163091)) ;
#82989=DIRECTION('',(-1.,0.,0.)) ;
#82990=DIRECTION('center_axis',(-0.164398987305354,-0.986393923832144,0.)) ;
#82991=DIRECTION('ref_axis',(0.,0.,1.)) ;
#82992=DIRECTION('',(0.,0.,-1.)) ;
#82993=DIRECTION('center_axis',(-0.164398987305377,-0.98639392383214,4.33975683157178E-13)) ;
#82994=DIRECTION('ref_axis',(-0.0577290357386321,0.00962150595687908,0.998285923498779)) ;
#82995=DIRECTION('',(0.,0.,1.)) ;
#82996=DIRECTION('center_axis',(1.,-2.89120579329441E-16,0.)) ;
#82997=DIRECTION('ref_axis',(-2.89120579329441E-16,-1.,-1.20980294963545E-15)) ;
#82998=DIRECTION('center_axis',(1.,1.15648231731787E-15,0.)) ;
#82999=DIRECTION('ref_axis',(1.15648231731787E-15,-1.,0.)) ;
#83000=DIRECTION('center_axis',(0.166689823582857,0.983956802812107,0.0635886225176511)) ;
#83001=DIRECTION('ref_axis',(-0.0486480009802627,0.0726194159291099,-0.996172571611334)) ;
#83002=DIRECTION('center_axis',(0.166689823544614,0.983956802870497,-0.0635886217143894)) ;
#83003=DIRECTION('ref_axis',(-0.0462047035092779,0.0722149187712735,0.996318287938387)) ;
#83004=DIRECTION('center_axis',(-0.164398987305354,-0.986393923832144,0.)) ;
#83005=DIRECTION('ref_axis',(0.,0.,1.)) ;
#83006=DIRECTION('',(0.,0.,1.)) ;
#83007=DIRECTION('center_axis',(-0.164398987305428,-0.986393923832132,-1.30192704752217E-12)) ;
#83008=DIRECTION('ref_axis',(-0.0554192327865001,0.0092365387990719,-0.998420450005091)) ;
#83009=DIRECTION('',(0.,0.,-1.)) ;
#83010=DIRECTION('center_axis',(0.,0.,1.)) ;
#83011=DIRECTION('ref_axis',(1.,0.,0.)) ;
#83012=DIRECTION('center_axis',(0.,0.,1.)) ;
#83013=DIRECTION('ref_axis',(1.,0.,0.)) ;
#83014=DIRECTION('center_axis',(0.,1.,0.)) ;
#83015=DIRECTION('ref_axis',(1.,0.,0.)) ;
#83016=DIRECTION('center_axis',(0.,-0.888198741900269,0.45945945945946)) ;
#83017=DIRECTION('ref_axis',(0.,0.45945945945946,0.888198741900269)) ;
#83018=DIRECTION('center_axis',(-1.,0.,1.22067519501986E-15)) ;
#83019=DIRECTION('ref_axis',(-1.22067519501986E-15,0.,-1.)) ;
#83020=DIRECTION('center_axis',(0.,0.,1.)) ;
#83021=DIRECTION('ref_axis',(1.,0.,0.)) ;
#83022=DIRECTION('center_axis',(0.,0.,-1.)) ;
#83023=DIRECTION('ref_axis',(-1.,0.,0.)) ;
#83024=DIRECTION('center_axis',(1.,-3.46944695195361E-16,0.)) ;
#83025=DIRECTION('ref_axis',(3.46944695195361E-16,1.,0.)) ;
#83026=DIRECTION('center_axis',(-1.,3.46944695195361E-16,0.)) ;
#83027=DIRECTION('ref_axis',(3.46944695195361E-16,1.,0.)) ;
#83028=DIRECTION('center_axis',(-1.,3.46944695195361E-16,0.)) ;
#83029=DIRECTION('ref_axis',(-3.41607084500048E-16,-1.,0.)) ;
#83030=DIRECTION('center_axis',(0.,-0.459459459459457,0.888198741900271)) ;
#83031=DIRECTION('ref_axis',(0.,-0.888198741900271,-0.459459459459457)) ;
#83032=DIRECTION('center_axis',(1.,-3.46944695195361E-16,0.)) ;
#83033=DIRECTION('ref_axis',(0.,1.,0.)) ;
#83034=DIRECTION('center_axis',(0.,0.888198741900269,-0.45945945945946)) ;
#83035=DIRECTION('ref_axis',(0.,-0.45945945945946,-0.888198741900269)) ;
#83036=DIRECTION('center_axis',(0.,1.,0.)) ;
#83037=DIRECTION('ref_axis',(1.,0.,0.)) ;
#83038=DIRECTION('center_axis',(0.,-1.,0.)) ;
#83039=DIRECTION('ref_axis',(0.,0.,1.)) ;
#83040=DIRECTION('center_axis',(-1.,0.,0.)) ;
#83041=DIRECTION('ref_axis',(0.,0.,-1.)) ;
#83042=DIRECTION('center_axis',(0.,0.,-1.)) ;
#83043=DIRECTION('ref_axis',(-1.,0.,0.)) ;
#83044=DIRECTION('center_axis',(0.,0.,-1.)) ;
#83045=DIRECTION('ref_axis',(-1.,0.,0.)) ;
#83046=DIRECTION('center_axis',(1.,-3.46944695195361E-16,0.)) ;
#83047=DIRECTION('ref_axis',(3.46944695195361E-16,1.,0.)) ;
#83048=DIRECTION('center_axis',(-1.,3.46944695195361E-16,0.)) ;
#83049=DIRECTION('ref_axis',(3.46944695195361E-16,1.,0.)) ;
#83050=DIRECTION('center_axis',(1.,0.,0.)) ;
#83051=DIRECTION('ref_axis',(0.,0.,-1.)) ;
#83052=DIRECTION('center_axis',(0.,0.,1.)) ;
#83053=DIRECTION('ref_axis',(1.,0.,0.)) ;
#83054=DIRECTION('center_axis',(0.,0.,1.)) ;
#83055=DIRECTION('ref_axis',(1.,0.,0.)) ;
#83056=DIRECTION('center_axis',(1.,-3.46944695195361E-16,0.)) ;
#83057=DIRECTION('ref_axis',(3.80647894157197E-16,1.,0.)) ;
#83058=DIRECTION('center_axis',(0.,0.459459459459459,-0.888198741900269)) ;
#83059=DIRECTION('ref_axis',(0.,0.888198741900269,0.459459459459459)) ;
#83060=DIRECTION('center_axis',(1.,-3.46944695195361E-16,0.)) ;
#83061=DIRECTION('ref_axis',(3.46944695195361E-16,1.,0.)) ;
#83062=DIRECTION('center_axis',(-1.,3.46944695195361E-16,0.)) ;
#83063=DIRECTION('ref_axis',(3.46944695195361E-16,1.,0.)) ;
#83064=DIRECTION('center_axis',(-3.46944695195361E-16,-1.,-6.49299968442375E-16)) ;
#83065=DIRECTION('ref_axis',(2.25271179641597E-31,6.49299968442375E-16,
-1.)) ;
#83066=DIRECTION('center_axis',(0.,-1.,0.)) ;
#83067=DIRECTION('ref_axis',(0.,0.,-1.)) ;
#83068=DIRECTION('center_axis',(0.,0.,1.)) ;
#83069=DIRECTION('ref_axis',(1.,0.,0.)) ;
#83070=DIRECTION('center_axis',(-3.25260651745651E-15,0.,1.)) ;
#83071=DIRECTION('ref_axis',(1.,0.,3.25260651745651E-15)) ;
#83072=DIRECTION('center_axis',(0.,1.,0.)) ;
#83073=DIRECTION('ref_axis',(1.,0.,0.)) ;
#83074=DIRECTION('center_axis',(0.,-0.888198741900269,-0.45945945945946)) ;
#83075=DIRECTION('ref_axis',(0.,-0.45945945945946,0.888198741900269)) ;
#83076=DIRECTION('center_axis',(1.,-3.46944695195361E-16,0.)) ;
#83077=DIRECTION('ref_axis',(0.,1.,0.)) ;
#83078=DIRECTION('center_axis',(0.,0.888198741900269,0.45945945945946)) ;
#83079=DIRECTION('ref_axis',(0.,0.45945945945946,-0.888198741900269)) ;
#83080=DIRECTION('center_axis',(1.,-3.46944695195361E-16,0.)) ;
#83081=DIRECTION('ref_axis',(0.,1.,0.)) ;
#83082=DIRECTION('center_axis',(0.,1.,0.)) ;
#83083=DIRECTION('ref_axis',(0.,0.,-1.)) ;
#83084=DIRECTION('center_axis',(0.,1.,0.)) ;
#83085=DIRECTION('ref_axis',(1.,0.,0.)) ;
#83086=DIRECTION('center_axis',(-1.,0.,0.)) ;
#83087=DIRECTION('ref_axis',(0.,0.,-1.)) ;
#83088=DIRECTION('center_axis',(1.,-3.46944695195361E-16,0.)) ;
#83089=DIRECTION('ref_axis',(3.41607084500048E-16,1.,0.)) ;
#83090=DIRECTION('center_axis',(-9.62987005567165E-16,-0.459459459459459,
-0.88819874190027)) ;
#83091=DIRECTION('ref_axis',(-7.31984232283282E-30,0.88819874190027,-0.459459459459459)) ;
#83092=DIRECTION('center_axis',(1.,-3.46944695195361E-16,0.)) ;
#83093=DIRECTION('ref_axis',(3.46944695195361E-16,1.,0.)) ;
#83094=DIRECTION('center_axis',(-1.,3.46944695195361E-16,0.)) ;
#83095=DIRECTION('ref_axis',(3.46944695195361E-16,1.,0.)) ;
#83096=DIRECTION('center_axis',(1.,0.,0.)) ;
#83097=DIRECTION('ref_axis',(0.,0.,-1.)) ;
#83098=DIRECTION('center_axis',(1.,-3.46944695195361E-16,0.)) ;
#83099=DIRECTION('ref_axis',(3.80647894157197E-16,1.,0.)) ;
#83100=DIRECTION('center_axis',(0.,0.459459459459459,0.888198741900269)) ;
#83101=DIRECTION('ref_axis',(0.,-0.888198741900269,0.459459459459459)) ;
#83102=DIRECTION('center_axis',(-3.46944695195361E-16,-1.,-6.49299968442375E-16)) ;
#83103=DIRECTION('ref_axis',(2.25271179641597E-31,6.49299968442375E-16,
-1.)) ;
#83104=DIRECTION('center_axis',(0.,1.,0.)) ;
#83105=DIRECTION('ref_axis',(0.,0.,-1.)) ;
#83106=DIRECTION('center_axis',(1.,0.,2.25271179641597E-31)) ;
#83107=DIRECTION('ref_axis',(2.25271179641597E-31,0.,-1.)) ;
#83108=DIRECTION('center_axis',(-1.,0.,0.)) ;
#83109=DIRECTION('ref_axis',(0.,0.,1.)) ;
#83110=DIRECTION('center_axis',(0.,1.,0.)) ;
#83111=DIRECTION('ref_axis',(1.,0.,0.)) ;
#83112=DIRECTION('center_axis',(0.,-1.,0.)) ;
#83113=DIRECTION('ref_axis',(-1.08420217248551E-15,0.,1.)) ;
#83114=DIRECTION('center_axis',(1.,-3.46944695195361E-16,0.)) ;
#83115=DIRECTION('ref_axis',(0.,1.,0.)) ;
#83116=DIRECTION('center_axis',(0.,1.,0.)) ;
#83117=DIRECTION('ref_axis',(0.,0.,-1.)) ;
#83118=DIRECTION('center_axis',(0.,-1.,0.)) ;
#83119=DIRECTION('ref_axis',(0.,0.,-1.)) ;
#83120=DIRECTION('center_axis',(0.,0.,1.)) ;
#83121=DIRECTION('ref_axis',(-1.,0.,0.)) ;
#83122=DIRECTION('center_axis',(0.,0.,-1.)) ;
#83123=DIRECTION('ref_axis',(-1.,0.,0.)) ;
#83124=DIRECTION('center_axis',(0.,0.,-1.)) ;
#83125=DIRECTION('ref_axis',(-1.,0.,0.)) ;
#83126=DIRECTION('center_axis',(-3.46944695195361E-16,-1.,-9.27571383489107E-17)) ;
#83127=DIRECTION('ref_axis',(1.,-3.46944695195361E-16,-3.21815970916568E-32)) ;
#83128=DIRECTION('center_axis',(0.,-1.,0.)) ;
#83129=DIRECTION('ref_axis',(0.,0.,-1.)) ;
#83130=DIRECTION('center_axis',(3.46944695195361E-16,1.,9.27571383489107E-17)) ;
#83131=DIRECTION('ref_axis',(-1.,3.46944695195361E-16,3.21815970916568E-32)) ;
#83132=DIRECTION('center_axis',(0.,1.,0.)) ;
#83133=DIRECTION('ref_axis',(0.,0.,-1.)) ;
#83134=DIRECTION('center_axis',(0.,0.,-1.)) ;
#83135=DIRECTION('ref_axis',(-1.,0.,0.)) ;
#83136=DIRECTION('center_axis',(0.,0.,1.)) ;
#83137=DIRECTION('ref_axis',(1.,0.,0.)) ;
#83138=DIRECTION('center_axis',(0.,1.,0.)) ;
#83139=DIRECTION('ref_axis',(1.,0.,0.)) ;
#83140=DIRECTION('center_axis',(-1.,0.,1.0842021724855E-15)) ;
#83141=DIRECTION('ref_axis',(-1.0842021724855E-15,0.,-1.)) ;
#83142=DIRECTION('center_axis',(0.,-1.,0.)) ;
#83143=DIRECTION('ref_axis',(0.,0.,-1.)) ;
#83144=DIRECTION('center_axis',(1.,0.,0.)) ;
#83145=DIRECTION('ref_axis',(0.,0.,1.)) ;
#83146=DIRECTION('center_axis',(1.,0.,3.21815970916568E-32)) ;
#83147=DIRECTION('ref_axis',(3.21815970916568E-32,0.,-1.)) ;
#83148=DIRECTION('center_axis',(0.,1.,0.)) ;
#83149=DIRECTION('ref_axis',(1.,0.,0.)) ;
#83150=DIRECTION('center_axis',(0.,0.,-1.)) ;
#83151=DIRECTION('ref_axis',(1.,0.,0.)) ;
#83152=DIRECTION('center_axis',(1.,0.,0.)) ;
#83153=DIRECTION('ref_axis',(0.,-1.08420217248551E-15,1.)) ;
#83154=DIRECTION('center_axis',(1.0842021724855E-15,1.,0.)) ;
#83155=DIRECTION('ref_axis',(1.,-1.0842021724855E-15,0.)) ;
#83156=DIRECTION('center_axis',(1.,0.,-2.08976773479518E-32)) ;
#83157=DIRECTION('ref_axis',(-2.08976773479518E-32,0.,-1.)) ;
#83158=DIRECTION('center_axis',(-0.447220452189278,-7.10035983522275E-6,
-0.894423762594221)) ;
#83159=DIRECTION('ref_axis',(0.894325663270205,0.0148067719276498,-0.4471715191304)) ;
#83160=DIRECTION('center_axis',(-1.23908819712629E-16,1.,2.4093381610789E-16)) ;
#83161=DIRECTION('ref_axis',(2.98538247827883E-32,-2.4093381610789E-16,
1.)) ;
#83162=DIRECTION('center_axis',(-5.60223412787738E-6,-0.447219005480045,
-0.894424485971876)) ;
#83163=DIRECTION('ref_axis',(0.0146917039260204,0.894327914920264,-0.447170811245684)) ;
#83164=DIRECTION('center_axis',(-8.95614743483648E-33,0.,1.)) ;
#83165=DIRECTION('ref_axis',(1.,0.,8.95614743483648E-33)) ;
#83166=DIRECTION('center_axis',(1.40488587213121E-32,-1.23908819712629E-16,
-1.)) ;
#83167=DIRECTION('ref_axis',(1.74077750246726E-48,1.,-1.23908819712629E-16)) ;
#83168=DIRECTION('center_axis',(-2.65552944032596E-32,0.,1.)) ;
#83169=DIRECTION('ref_axis',(1.,0.,2.65552944032596E-32)) ;
#83170=DIRECTION('center_axis',(0.894424485971418,-5.60223478642178E-6,
0.447219005480961)) ;
#83171=DIRECTION('ref_axis',(0.447170811246659,0.0146917039183822,-0.894327914919902)) ;
#83172=DIRECTION('center_axis',(0.89442376259406,-7.10036036684763E-6,-0.4472204521896)) ;
#83173=DIRECTION('ref_axis',(0.447171519130562,0.0148067719529079,0.894325663269706)) ;
#83174=DIRECTION('center_axis',(-8.95614743483648E-33,-1.10974565782288E-48,
1.)) ;
#83175=DIRECTION('ref_axis',(1.,-9.9390457266313E-81,8.95614743483648E-33)) ;
#83176=DIRECTION('center_axis',(-7.10035964917347E-6,0.894423762594175,
0.447220452189369)) ;
#83177=DIRECTION('ref_axis',(-0.0148067720024296,-0.447171519129994,0.89432566326917)) ;
#83178=DIRECTION('center_axis',(-5.60223406011642E-6,0.894424485971595,
-0.447219005480606)) ;
#83179=DIRECTION('ref_axis',(0.0146917039587169,0.44717081124603,0.894327914919554)) ;
#83180=DIRECTION('center_axis',(1.40488587213121E-32,-1.23908819712629E-16,
-1.)) ;
#83181=DIRECTION('ref_axis',(0.,1.,0.)) ;
#83182=DIRECTION('center_axis',(-1.,0.,0.)) ;
#83183=DIRECTION('ref_axis',(0.,0.,-1.)) ;
#83184=DIRECTION('center_axis',(0.,-1.,0.)) ;
#83185=DIRECTION('ref_axis',(0.,0.,1.)) ;
#83186=DIRECTION('center_axis',(-1.,0.,-1.40488587213121E-32)) ;
#83187=DIRECTION('ref_axis',(-1.40488587213121E-32,0.,1.)) ;
#83188=DIRECTION('',(-1.,0.,-1.40488587213121E-32)) ;
#83189=DIRECTION('center_axis',(-1.,0.,0.)) ;
#83190=DIRECTION('ref_axis',(0.,0.,1.)) ;
#83191=DIRECTION('center_axis',(0.,1.,0.)) ;
#83192=DIRECTION('ref_axis',(1.,0.,0.)) ;
#83193=DIRECTION('center_axis',(0.,1.,0.)) ;
#83194=DIRECTION('ref_axis',(0.,0.,-1.)) ;
#83195=DIRECTION('center_axis',(0.,0.,-1.)) ;
#83196=DIRECTION('ref_axis',(1.,0.,0.)) ;
#83197=DIRECTION('center_axis',(-1.,0.,-1.7912294869673E-32)) ;
#83198=DIRECTION('ref_axis',(-1.7912294869673E-32,0.,1.)) ;
#83199=DIRECTION('center_axis',(-0.447219005480393,-5.60223393701113E-6,
0.894424485971702)) ;
#83200=DIRECTION('ref_axis',(0.894327914919925,0.0146917039386571,0.447170811245947)) ;
#83201=DIRECTION('center_axis',(-1.,0.,0.)) ;
#83202=DIRECTION('ref_axis',(0.,0.,1.)) ;
#83203=DIRECTION('center_axis',(1.23908819712629E-16,-1.,7.2280144832367E-17)) ;
#83204=DIRECTION('ref_axis',(1.,1.23908819712629E-16,-8.95614743483648E-33)) ;
#83205=DIRECTION('center_axis',(-7.10036022080745E-6,-0.447220452189551,
0.894423762594084)) ;
#83206=DIRECTION('ref_axis',(-0.0148067719367088,-0.894325663269946,-0.447171519130618)) ;
#83207=DIRECTION('center_axis',(0.,-1.,1.0842021724855E-15)) ;
#83208=DIRECTION('ref_axis',(0.,-1.0842021724855E-15,-1.)) ;
#83209=DIRECTION('center_axis',(1.23908819712629E-16,-1.,1.23908819712629E-16)) ;
#83210=DIRECTION('ref_axis',(-9.81657386420148E-47,-1.23908819712629E-16,
-1.)) ;
#83211=DIRECTION('center_axis',(0.,-1.,0.)) ;
#83212=DIRECTION('ref_axis',(0.,0.,-1.)) ;
#83213=DIRECTION('',(-1.23908819712629E-16,1.,-1.23908819712629E-16)) ;
#83214=DIRECTION('center_axis',(1.,0.,1.40488587213121E-32)) ;
#83215=DIRECTION('ref_axis',(1.40488587213121E-32,0.,-1.)) ;
#83216=DIRECTION('center_axis',(-0.707106781186547,0.707106781186548,-6.4115285974492E-16)) ;
#83217=DIRECTION('ref_axis',(0.707106781186548,0.707106781186547,-1.7981834674121E-12)) ;
#83218=DIRECTION('center_axis',(1.,0.,0.)) ;
#83219=DIRECTION('ref_axis',(0.,0.,-1.)) ;
#83220=DIRECTION('center_axis',(0.,-1.,0.)) ;
#83221=DIRECTION('ref_axis',(0.,0.,-1.)) ;
#83222=DIRECTION('center_axis',(0.,0.,1.)) ;
#83223=DIRECTION('ref_axis',(-1.,0.,0.)) ;
#83224=DIRECTION('center_axis',(7.2280144832367E-17,0.,-1.)) ;
#83225=DIRECTION('ref_axis',(-1.,0.,-7.2280144832367E-17)) ;
#83226=DIRECTION('',(7.2280144832367E-17,0.,-1.)) ;
#83227=DIRECTION('center_axis',(0.,0.,-1.)) ;
#83228=DIRECTION('ref_axis',(-1.,0.,0.)) ;
#83229=DIRECTION('center_axis',(0.,1.,0.)) ;
#83230=DIRECTION('ref_axis',(1.,0.,0.)) ;
#83231=DIRECTION('center_axis',(0.,0.,1.)) ;
#83232=DIRECTION('ref_axis',(-1.,0.,0.)) ;
#83233=DIRECTION('center_axis',(0.,1.,0.)) ;
#83234=DIRECTION('ref_axis',(1.,0.,0.)) ;
#83235=DIRECTION('center_axis',(1.,0.,0.)) ;
#83236=DIRECTION('ref_axis',(0.,0.,1.)) ;
#83237=DIRECTION('center_axis',(0.,0.,-1.)) ;
#83238=DIRECTION('ref_axis',(1.,0.,0.)) ;
#83239=DIRECTION('center_axis',(-1.13380619344889E-16,1.,-1.23908819712629E-16)) ;
#83240=DIRECTION('ref_axis',(-1.40488587213121E-32,1.23908819712629E-16,
1.)) ;
#83241=DIRECTION('center_axis',(0.,1.,0.)) ;
#83242=DIRECTION('ref_axis',(0.,0.,1.)) ;
#83243=DIRECTION('center_axis',(7.2280144832367E-17,0.,-1.)) ;
#83244=DIRECTION('ref_axis',(-1.,0.,-7.2280144832367E-17)) ;
#83245=DIRECTION('center_axis',(0.,0.,1.)) ;
#83246=DIRECTION('ref_axis',(1.,0.,0.)) ;
#83247=DIRECTION('center_axis',(0.,1.,0.)) ;
#83248=DIRECTION('ref_axis',(1.,0.,0.)) ;
#83249=DIRECTION('center_axis',(0.,1.,0.)) ;
#83250=DIRECTION('ref_axis',(0.,0.,-1.)) ;
#83251=DIRECTION('center_axis',(1.,2.16840434497101E-15,-2.93873587705572E-31)) ;
#83252=DIRECTION('ref_axis',(2.16840434497101E-15,-1.,-1.03035812136257E-62)) ;
#83253=DIRECTION('center_axis',(-8.95614743483648E-33,0.,1.)) ;
#83254=DIRECTION('ref_axis',(1.,0.,8.95614743483648E-33)) ;
#83255=DIRECTION('center_axis',(-1.40488587213121E-32,1.23908819712629E-16,
1.)) ;
#83256=DIRECTION('ref_axis',(-1.74077750246726E-48,-1.,1.23908819712629E-16)) ;
#83257=DIRECTION('center_axis',(8.95614743483648E-33,1.0154535431059E-48,
-1.)) ;
#83258=DIRECTION('ref_axis',(-1.,9.09455164528354E-81,-8.95614743483648E-33)) ;
#83259=DIRECTION('center_axis',(2.16840434497101E-15,0.,-1.)) ;
#83260=DIRECTION('ref_axis',(-1.,0.,-2.16840434497101E-15)) ;
#83261=DIRECTION('',(-8.95614743483648E-33,-1.0154535431059E-48,1.)) ;
#83262=DIRECTION('center_axis',(-1.,-1.13380619344889E-16,0.)) ;
#83263=DIRECTION('ref_axis',(0.,-1.,0.)) ;
#83264=DIRECTION('center_axis',(0.,0.,1.)) ;
#83265=DIRECTION('ref_axis',(-1.,0.,0.)) ;
#83266=DIRECTION('center_axis',(0.,-1.,0.)) ;
#83267=DIRECTION('ref_axis',(0.,0.,-1.)) ;
#83268=DIRECTION('center_axis',(-1.,0.,0.)) ;
#83269=DIRECTION('ref_axis',(0.,0.,-1.)) ;
#83270=DIRECTION('center_axis',(1.,0.,1.40488587213121E-32)) ;
#83271=DIRECTION('ref_axis',(1.40488587213121E-32,0.,-1.)) ;
#83272=DIRECTION('',(1.,0.,1.40488587213121E-32)) ;
#83273=DIRECTION('center_axis',(1.,0.,0.)) ;
#83274=DIRECTION('ref_axis',(0.,0.,-1.)) ;
#83275=DIRECTION('center_axis',(-1.40488587213121E-32,1.23908819712629E-16,
1.)) ;
#83276=DIRECTION('ref_axis',(0.,-1.,0.)) ;
#83277=DIRECTION('center_axis',(0.,-1.,0.)) ;
#83278=DIRECTION('ref_axis',(0.,0.,1.)) ;
#83279=DIRECTION('center_axis',(0.,1.,0.)) ;
#83280=DIRECTION('ref_axis',(1.,0.,0.)) ;
#83281=DIRECTION('center_axis',(1.,0.,0.)) ;
#83282=DIRECTION('ref_axis',(0.,0.,1.)) ;
#83283=DIRECTION('center_axis',(0.,1.,0.)) ;
#83284=DIRECTION('ref_axis',(0.,0.,-1.)) ;
#83285=DIRECTION('center_axis',(0.,0.,1.)) ;
#83286=DIRECTION('ref_axis',(1.,0.,0.)) ;
#83287=DIRECTION('center_axis',(0.,0.,1.)) ;
#83288=DIRECTION('ref_axis',(1.,0.,0.)) ;
#83289=DIRECTION('center_axis',(1.,0.,1.40488587213121E-32)) ;
#83290=DIRECTION('ref_axis',(1.40488587213121E-32,0.,-1.)) ;
#83291=DIRECTION('center_axis',(-0.707106781186552,0.707106781186543,-7.95029546083767E-15)) ;
#83292=DIRECTION('ref_axis',(0.707106781186543,0.707106781186552,-2.58223494640614E-13)) ;
#83293=DIRECTION('center_axis',(-1.23908819712629E-16,1.,-1.23908819712629E-16)) ;
#83294=DIRECTION('ref_axis',(9.81657386420148E-47,1.23908819712629E-16,
1.)) ;
#83295=DIRECTION('',(1.23908819712629E-16,-1.,1.23908819712629E-16)) ;
#83296=DIRECTION('center_axis',(-1.,-1.13380619344889E-16,0.)) ;
#83297=DIRECTION('ref_axis',(0.,-1.,0.)) ;
#83298=DIRECTION('center_axis',(0.,-1.,0.)) ;
#83299=DIRECTION('ref_axis',(0.,0.,1.)) ;
#83300=DIRECTION('center_axis',(1.13380619344889E-16,-1.,1.23908819712629E-16)) ;
#83301=DIRECTION('ref_axis',(1.40488587213121E-32,-1.23908819712629E-16,
-1.)) ;
#83302=DIRECTION('center_axis',(-1.5529910948782E-31,-4.47619207437002E-16,
1.)) ;
#83303=DIRECTION('ref_axis',(6.951486430461E-47,-1.,-4.47619207437002E-16)) ;
#83304=DIRECTION('center_axis',(0.,2.16840434497101E-15,-1.)) ;
#83305=DIRECTION('ref_axis',(0.,1.,2.16840434497101E-15)) ;
#83306=DIRECTION('center_axis',(0.,1.,0.)) ;
#83307=DIRECTION('ref_axis',(1.,0.,0.)) ;
#83308=DIRECTION('center_axis',(3.85194802226865E-15,0.888198741900269,
-0.45945945945946)) ;
#83309=DIRECTION('ref_axis',(3.25260651745654E-15,-0.45945945945946,-0.888198741900269)) ;
#83310=DIRECTION('center_axis',(-1.,0.,1.22067519501986E-15)) ;
#83311=DIRECTION('ref_axis',(-1.22067519501986E-15,1.73472347597682E-14,
-1.)) ;
#83312=DIRECTION('center_axis',(1.5529910948782E-31,4.47619207437002E-16,
-1.)) ;
#83313=DIRECTION('ref_axis',(-6.951486430461E-47,1.,4.47619207437002E-16)) ;
#83314=DIRECTION('center_axis',(0.,0.,1.)) ;
#83315=DIRECTION('ref_axis',(1.,0.,0.)) ;
#83316=DIRECTION('center_axis',(1.,-3.46944695195361E-16,0.)) ;
#83317=DIRECTION('ref_axis',(3.46944695195361E-16,1.,0.)) ;
#83318=DIRECTION('center_axis',(-1.,3.46944695195361E-16,0.)) ;
#83319=DIRECTION('ref_axis',(3.46944695195361E-16,1.,1.73472347597681E-14)) ;
#83320=DIRECTION('center_axis',(1.,-3.46944695195361E-16,0.)) ;
#83321=DIRECTION('ref_axis',(3.41607084500048E-16,1.,0.)) ;
#83322=DIRECTION('center_axis',(0.,0.459459459459457,-0.888198741900271)) ;
#83323=DIRECTION('ref_axis',(0.,0.888198741900271,0.459459459459457)) ;
#83324=DIRECTION('center_axis',(0.,0.,1.)) ;
#83325=DIRECTION('ref_axis',(1.,0.,0.)) ;
#83326=DIRECTION('center_axis',(0.,0.,-1.)) ;
#83327=DIRECTION('ref_axis',(-1.,0.,0.)) ;
#83328=DIRECTION('center_axis',(-1.,3.46944695195361E-16,0.)) ;
#83329=DIRECTION('ref_axis',(-3.46944695195361E-16,-1.,0.)) ;
#83330=DIRECTION('center_axis',(-1.,3.46944695195361E-16,0.)) ;
#83331=DIRECTION('ref_axis',(-3.46944695195361E-16,-1.,0.)) ;
#83332=DIRECTION('center_axis',(-1.,3.46944695195361E-16,0.)) ;
#83333=DIRECTION('ref_axis',(3.46944695195361E-16,1.,0.)) ;
#83334=DIRECTION('center_axis',(1.,-3.46944695195361E-16,0.)) ;
#83335=DIRECTION('ref_axis',(0.,1.,0.)) ;
#83336=DIRECTION('center_axis',(0.,-0.888198741900269,0.459459459459461)) ;
#83337=DIRECTION('ref_axis',(0.,0.459459459459461,0.888198741900269)) ;
#83338=DIRECTION('center_axis',(0.,1.,0.)) ;
#83339=DIRECTION('ref_axis',(1.,0.,0.)) ;
#83340=DIRECTION('center_axis',(0.,1.,0.)) ;
#83341=DIRECTION('ref_axis',(0.,0.,-1.)) ;
#83342=DIRECTION('center_axis',(-1.,0.,0.)) ;
#83343=DIRECTION('ref_axis',(0.,-8.67361737988409E-15,-1.)) ;
#83344=DIRECTION('center_axis',(1.,-3.46944695195361E-16,0.)) ;
#83345=DIRECTION('ref_axis',(3.70074341541719E-16,1.,0.)) ;
#83346=DIRECTION('center_axis',(0.,0.63294893130157,-0.774193548387094)) ;
#83347=DIRECTION('ref_axis',(-1.08420217248551E-15,-0.774193548387094,-0.63294893130157)) ;
#83348=DIRECTION('center_axis',(1.,-3.46944695195361E-16,0.)) ;
#83349=DIRECTION('ref_axis',(3.80647894157197E-16,1.,0.)) ;
#83350=DIRECTION('center_axis',(0.,-0.45945945945946,0.888198741900269)) ;
#83351=DIRECTION('ref_axis',(0.,-0.888198741900269,-0.45945945945946)) ;
#83352=DIRECTION('center_axis',(1.,-3.46944695195361E-16,0.)) ;
#83353=DIRECTION('ref_axis',(3.46944695195361E-16,1.,0.)) ;
#83354=DIRECTION('center_axis',(-1.,3.46944695195361E-16,0.)) ;
#83355=DIRECTION('ref_axis',(3.46944695195361E-16,1.,0.)) ;
#83356=DIRECTION('center_axis',(-3.46944695195361E-16,-1.,-2.45739631480277E-16)) ;
#83357=DIRECTION('ref_axis',(1.,-3.46944695195361E-16,-8.52580615413453E-32)) ;
#83358=DIRECTION('center_axis',(0.,1.,0.)) ;
#83359=DIRECTION('ref_axis',(0.,0.,1.)) ;
#83360=DIRECTION('center_axis',(1.,-3.46944695195361E-16,0.)) ;
#83361=DIRECTION('ref_axis',(3.33066907387547E-16,1.,0.)) ;
#83362=DIRECTION('center_axis',(8.02036034720251E-16,0.293103448275862,
-0.956080733311157)) ;
#83363=DIRECTION('ref_axis',(-1.93209005840966E-30,0.956080733311157,0.293103448275862)) ;
#83364=DIRECTION('center_axis',(-1.,3.46944695195361E-16,0.)) ;
#83365=DIRECTION('ref_axis',(-3.46944695195361E-16,-1.,0.)) ;
#83366=DIRECTION('center_axis',(-1.,3.46944695195361E-16,0.)) ;
#83367=DIRECTION('ref_axis',(-3.46944695195361E-16,-1.,0.)) ;
#83368=DIRECTION('center_axis',(-1.,3.46944695195361E-16,0.)) ;
#83369=DIRECTION('ref_axis',(-3.46944695195361E-16,-1.,0.)) ;
#83370=DIRECTION('center_axis',(0.,0.,-1.)) ;
#83371=DIRECTION('ref_axis',(-1.,0.,0.)) ;
#83372=DIRECTION('center_axis',(0.,0.,1.)) ;
#83373=DIRECTION('ref_axis',(1.,0.,0.)) ;
#83374=DIRECTION('center_axis',(-1.5529910948782E-31,-4.47619207437002E-16,
-1.)) ;
#83375=DIRECTION('ref_axis',(-6.95148643046101E-47,1.,-4.47619207437002E-16)) ;
#83376=DIRECTION('center_axis',(2.16840434497101E-15,0.,1.)) ;
#83377=DIRECTION('ref_axis',(1.,0.,-2.16840434497101E-15)) ;
#83378=DIRECTION('center_axis',(1.,-3.46944695195361E-16,0.)) ;
#83379=DIRECTION('ref_axis',(0.,1.,0.)) ;
#83380=DIRECTION('center_axis',(0.,-1.,0.)) ;
#83381=DIRECTION('ref_axis',(0.,0.,1.)) ;
#83382=DIRECTION('center_axis',(0.577350269189627,0.577350269189627,0.577350269189623)) ;
#83383=DIRECTION('ref_axis',(-0.707106781186548,2.22044604925032E-15,0.707106781186547)) ;
#83384=DIRECTION('center_axis',(-1.,3.46944695195361E-16,0.)) ;
#83385=DIRECTION('ref_axis',(-3.70074341541719E-16,-1.,0.)) ;
#83386=DIRECTION('center_axis',(0.,0.63294893130157,0.774193548387094)) ;
#83387=DIRECTION('ref_axis',(0.,0.774193548387094,-0.63294893130157)) ;
#83388=DIRECTION('center_axis',(0.,1.,0.)) ;
#83389=DIRECTION('ref_axis',(1.,0.,0.)) ;
#83390=DIRECTION('center_axis',(-1.,0.,0.)) ;
#83391=DIRECTION('ref_axis',(0.,1.73472347597682E-14,-1.)) ;
#83392=DIRECTION('center_axis',(0.,0.888198741900271,0.459459459459457)) ;
#83393=DIRECTION('ref_axis',(-1.08420217248551E-15,0.459459459459457,-0.888198741900271)) ;
#83394=DIRECTION('center_axis',(3.46944695195361E-16,1.,2.45739631480277E-16)) ;
#83395=DIRECTION('ref_axis',(-1.,3.46944695195361E-16,8.52580615413453E-32)) ;
#83396=DIRECTION('center_axis',(-1.,3.46944695195361E-16,0.)) ;
#83397=DIRECTION('ref_axis',(-3.33066907387547E-16,-1.,0.)) ;
#83398=DIRECTION('center_axis',(0.,0.293103448275864,0.956080733311156)) ;
#83399=DIRECTION('ref_axis',(0.,-0.956080733311156,0.293103448275864)) ;
#83400=DIRECTION('center_axis',(-3.46944695195361E-16,-1.,-1.06487173641454E-15)) ;
#83401=DIRECTION('ref_axis',(3.69451600012496E-31,1.06487173641454E-15,
-1.)) ;
#83402=DIRECTION('center_axis',(0.,-1.,0.)) ;
#83403=DIRECTION('ref_axis',(0.,0.,-1.)) ;
#83404=DIRECTION('center_axis',(0.,1.,0.)) ;
#83405=DIRECTION('ref_axis',(0.,0.,1.)) ;
#83406=DIRECTION('center_axis',(-1.,3.46944695195361E-16,0.)) ;
#83407=DIRECTION('ref_axis',(-3.41607084500048E-16,-1.,0.)) ;
#83408=DIRECTION('center_axis',(-4.88154879316133E-15,0.45945945945946,
0.888198741900269)) ;
#83409=DIRECTION('ref_axis',(-3.39148554690438E-29,-0.888198741900269,0.45945945945946)) ;
#83410=DIRECTION('center_axis',(1.,-3.46944695195361E-16,0.)) ;
#83411=DIRECTION('ref_axis',(3.46944695195361E-16,1.,0.)) ;
#83412=DIRECTION('center_axis',(-1.,3.46944695195361E-16,0.)) ;
#83413=DIRECTION('ref_axis',(3.46944695195361E-16,1.,0.)) ;
#83414=DIRECTION('center_axis',(-1.5529910948782E-31,-4.47619207437002E-16,
-1.)) ;
#83415=DIRECTION('ref_axis',(-6.95148643046101E-47,1.,-4.47619207437002E-16)) ;
#83416=DIRECTION('center_axis',(0.,0.,-1.)) ;
#83417=DIRECTION('ref_axis',(-1.,0.,0.)) ;
#83418=DIRECTION('center_axis',(0.,0.224137931034483,-0.974557431797419)) ;
#83419=DIRECTION('ref_axis',(0.,-0.974557431797419,-0.224137931034483)) ;
#83420=DIRECTION('center_axis',(0.577350269189627,0.577350269189627,0.577350269189623)) ;
#83421=DIRECTION('ref_axis',(-0.707106781186548,2.22044604925032E-15,0.707106781186547)) ;
#83422=DIRECTION('center_axis',(0.408248290463864,-0.816496580927725,0.408248290463864)) ;
#83423=DIRECTION('ref_axis',(0.707106781186545,-2.77555756156289E-15,-0.70710678118655)) ;
#83424=DIRECTION('center_axis',(0.,1.,0.)) ;
#83425=DIRECTION('ref_axis',(1.,0.,0.)) ;
#83426=DIRECTION('center_axis',(-1.,0.,0.)) ;
#83427=DIRECTION('ref_axis',(0.,0.,-1.)) ;
#83428=DIRECTION('center_axis',(1.,-3.46944695195361E-16,0.)) ;
#83429=DIRECTION('ref_axis',(0.,1.,0.)) ;
#83430=DIRECTION('center_axis',(9.96293888229924E-16,-0.888198741900269,
-0.45945945945946)) ;
#83431=DIRECTION('ref_axis',(-3.00809911926502E-30,-0.45945945945946,0.888198741900269)) ;
#83432=DIRECTION('center_axis',(1.,-3.46944695195361E-16,0.)) ;
#83433=DIRECTION('ref_axis',(-3.70074341541719E-16,-1.,0.)) ;
#83434=DIRECTION('center_axis',(1.58436874053304E-16,-0.224137931034483,
-0.974557431797419)) ;
#83435=DIRECTION('ref_axis',(2.18893094986727E-31,0.974557431797419,-0.224137931034483)) ;
#83436=DIRECTION('center_axis',(1.,-3.46944695195361E-16,0.)) ;
#83437=DIRECTION('ref_axis',(3.46944695195361E-16,1.,0.)) ;
#83438=DIRECTION('center_axis',(-1.,3.46944695195361E-16,0.)) ;
#83439=DIRECTION('ref_axis',(3.46944695195361E-16,1.,0.)) ;
#83440=DIRECTION('center_axis',(1.,-3.46944695195361E-16,0.)) ;
#83441=DIRECTION('ref_axis',(3.80647894157197E-16,1.,0.)) ;
#83442=DIRECTION('center_axis',(0.,-0.45945945945946,-0.888198741900269)) ;
#83443=DIRECTION('ref_axis',(0.,0.888198741900269,-0.45945945945946)) ;
#83444=DIRECTION('center_axis',(1.,-3.46944695195361E-16,0.)) ;
#83445=DIRECTION('ref_axis',(0.,1.,0.)) ;
#83446=DIRECTION('center_axis',(0.,-1.,0.)) ;
#83447=DIRECTION('ref_axis',(0.,0.,1.)) ;
#83448=DIRECTION('center_axis',(-3.46944695195361E-16,-1.,-1.06487173641454E-15)) ;
#83449=DIRECTION('ref_axis',(3.69451600012496E-31,1.06487173641454E-15,
-1.)) ;
#83450=DIRECTION('center_axis',(0.,0.,1.)) ;
#83451=DIRECTION('ref_axis',(1.,0.,0.)) ;
#83452=DIRECTION('center_axis',(0.,-1.,0.)) ;
#83453=DIRECTION('ref_axis',(0.,0.,-1.)) ;
#83454=DIRECTION('center_axis',(0.,-1.,0.)) ;
#83455=DIRECTION('ref_axis',(0.,0.,-1.)) ;
#83456=DIRECTION('center_axis',(0.,1.,0.)) ;
#83457=DIRECTION('ref_axis',(0.,0.,-1.)) ;
#83458=DIRECTION('center_axis',(0.,0.,1.)) ;
#83459=DIRECTION('ref_axis',(1.,0.,0.)) ;
#83460=DIRECTION('center_axis',(8.67361737988404E-15,-1.,0.)) ;
#83461=DIRECTION('ref_axis',(1.,8.67361737988404E-15,0.)) ;
#83462=DIRECTION('center_axis',(0.497468338163091,-0.710669054518702,0.497468338163091)) ;
#83463=DIRECTION('ref_axis',(0.81923192051904,0.573462344363328,8.04804396179112E-16)) ;
#83464=DIRECTION('center_axis',(0.497468338163091,-0.710669054518702,0.497468338163091)) ;
#83465=DIRECTION('ref_axis',(0.81923192051904,0.573462344363328,7.6535433881835E-16)) ;
#83466=DIRECTION('center_axis',(0.497468338163092,-0.7106690545187,0.497468338163092)) ;
#83467=DIRECTION('ref_axis',(-1.24903860074368E-15,-0.57346234436333,-0.819231920519039)) ;
#83468=DIRECTION('center_axis',(0.,0.,1.)) ;
#83469=DIRECTION('ref_axis',(1.,0.,0.)) ;
#83470=DIRECTION('center_axis',(0.,-1.,0.)) ;
#83471=DIRECTION('ref_axis',(0.,0.,-1.)) ;
#83472=DIRECTION('center_axis',(0.,1.,0.)) ;
#83473=DIRECTION('ref_axis',(0.,0.,1.)) ;
#83474=DIRECTION('center_axis',(0.,1.,0.)) ;
#83475=DIRECTION('ref_axis',(0.,0.,1.)) ;
#83476=DIRECTION('center_axis',(0.,1.,0.)) ;
#83477=DIRECTION('ref_axis',(1.,0.,0.)) ;
#83478=DIRECTION('center_axis',(-1.98515611757154E-15,0.,1.)) ;
#83479=DIRECTION('ref_axis',(-1.,0.,-1.98515611757154E-15)) ;
#83480=DIRECTION('center_axis',(1.,-4.06575814682065E-16,2.84603070277446E-16)) ;
#83481=DIRECTION('ref_axis',(-4.06575814682065E-16,-1.,6.48893816316174E-47)) ;
#83482=DIRECTION('center_axis',(0.,1.,0.)) ;
#83483=DIRECTION('ref_axis',(0.,0.,1.)) ;
#83484=DIRECTION('center_axis',(0.,1.,0.)) ;
#83485=DIRECTION('ref_axis',(0.,0.,1.)) ;
#83486=DIRECTION('center_axis',(0.497468338163091,0.710669054518702,-0.497468338163091)) ;
#83487=DIRECTION('ref_axis',(-0.81923192051904,0.573462344363328,7.6535433881835E-16)) ;
#83488=DIRECTION('center_axis',(-0.497468338163091,-0.710669054518702,0.497468338163091)) ;
#83489=DIRECTION('ref_axis',(-0.819231920519035,0.573462344363336,1.64011789552923E-14)) ;
#83490=DIRECTION('center_axis',(-0.497468338163093,-0.7106690545187,0.497468338163091)) ;
#83491=DIRECTION('ref_axis',(0.819231920519039,-0.573462344363331,1.48853464230757E-16)) ;
#83492=DIRECTION('center_axis',(1.,0.,0.)) ;
#83493=DIRECTION('ref_axis',(0.,0.,-1.)) ;
#83494=DIRECTION('center_axis',(1.,0.,-9.9257805878577E-16)) ;
#83495=DIRECTION('ref_axis',(-9.9257805878577E-16,0.,-1.)) ;
#83496=DIRECTION('center_axis',(0.,0.,-1.)) ;
#83497=DIRECTION('ref_axis',(-1.,0.,0.)) ;
#83498=DIRECTION('center_axis',(-1.23327997120227E-15,1.76182853028895E-15,
1.)) ;
#83499=DIRECTION('ref_axis',(-2.17282783909808E-30,-1.,1.76182853028895E-15)) ;
#83500=DIRECTION('center_axis',(-0.497468338163091,0.710669054518702,0.497468338163091)) ;
#83501=DIRECTION('ref_axis',(-0.81923192051904,-0.573462344363328,7.6535433881835E-16)) ;
#83502=DIRECTION('center_axis',(0.497468338163091,-0.710669054518702,-0.497468338163091)) ;
#83503=DIRECTION('ref_axis',(-0.819231920519018,-0.57346234436336,6.87084924063159E-14)) ;
#83504=DIRECTION('center_axis',(0.497468338163093,-0.7106690545187,-0.497468338163091)) ;
#83505=DIRECTION('ref_axis',(0.819231920519039,0.573462344363331,2.16059097207149E-16)) ;
#83506=DIRECTION('center_axis',(0.,1.,0.)) ;
#83507=DIRECTION('ref_axis',(1.,0.,0.)) ;
#83508=DIRECTION('center_axis',(-1.13841228110978E-15,-1.62630325872826E-15,
1.)) ;
#83509=DIRECTION('ref_axis',(3.52365706057789E-15,1.,1.62630325872826E-15)) ;
#83510=DIRECTION('center_axis',(0.,1.,0.)) ;
#83511=DIRECTION('ref_axis',(1.,0.,0.)) ;
#83512=DIRECTION('center_axis',(1.,0.,-1.65429676464295E-16)) ;
#83513=DIRECTION('ref_axis',(1.65429676464295E-16,4.33680868994204E-15,
1.)) ;
#83514=DIRECTION('center_axis',(0.,0.,-1.)) ;
#83515=DIRECTION('ref_axis',(-1.,0.,0.)) ;
#83516=DIRECTION('center_axis',(3.3085935292859E-16,0.,1.)) ;
#83517=DIRECTION('ref_axis',(1.,0.,-3.3085935292859E-16)) ;
#83518=DIRECTION('center_axis',(1.,0.,0.)) ;
#83519=DIRECTION('ref_axis',(0.,0.,-1.)) ;
#83520=DIRECTION('center_axis',(1.,1.21972744404619E-15,8.53809210832338E-16)) ;
#83521=DIRECTION('ref_axis',(-1.21972744404619E-15,1.,-2.84382165153726E-47)) ;
#83522=DIRECTION('center_axis',(0.,1.,0.)) ;
#83523=DIRECTION('ref_axis',(1.,0.,0.)) ;
#83524=DIRECTION('center_axis',(0.497468338163092,0.710669054518701,0.497468338163092)) ;
#83525=DIRECTION('ref_axis',(1.11733937654106E-14,0.573462344363324,-0.819231920519043)) ;
#83526=DIRECTION('center_axis',(-0.497468338163091,-0.710669054518702,-0.497468338163091)) ;
#83527=DIRECTION('ref_axis',(0.81923192051904,-0.573462344363328,7.6535433881835E-16)) ;
#83528=DIRECTION('center_axis',(-0.497468338163091,-0.710669054518702,-0.497468338163091)) ;
#83529=DIRECTION('ref_axis',(0.81923192051904,-0.573462344363328,7.6535433881835E-16)) ;
#83530=DIRECTION('center_axis',(0.,-1.,0.)) ;
#83531=DIRECTION('ref_axis',(0.,0.,-1.)) ;
#83532=DIRECTION('center_axis',(0.,1.,0.)) ;
#83533=DIRECTION('ref_axis',(0.,0.,-1.)) ;
#83534=DIRECTION('center_axis',(-8.67361737988403E-15,1.,0.)) ;
#83535=DIRECTION('ref_axis',(-1.,-8.67361737988403E-15,0.)) ;
#83536=DIRECTION('center_axis',(0.,0.,1.)) ;
#83537=DIRECTION('ref_axis',(1.,0.,0.)) ;
#83538=DIRECTION('center_axis',(1.,6.67201336914158E-17,0.)) ;
#83539=DIRECTION('ref_axis',(-6.67201336914158E-17,1.,0.)) ;
#83540=DIRECTION('center_axis',(-1.,-6.67201336914158E-17,0.)) ;
#83541=DIRECTION('ref_axis',(-6.67201336914158E-17,1.,0.)) ;
#83542=DIRECTION('center_axis',(-1.,1.33440267382831E-16,0.)) ;
#83543=DIRECTION('ref_axis',(-1.33440267382831E-16,-1.,0.)) ;
#83544=DIRECTION('center_axis',(-1.,1.33440267382831E-16,0.)) ;
#83545=DIRECTION('ref_axis',(-1.33440267382831E-16,-1.,0.)) ;
#83546=DIRECTION('center_axis',(0.710669054518702,0.497468338163091,0.497468338163091)) ;
#83547=DIRECTION('ref_axis',(-0.573462344363328,0.819231920519041,3.92980824865032E-16)) ;
#83548=DIRECTION('center_axis',(0.710669054518702,0.497468338163091,0.497468338163091)) ;
#83549=DIRECTION('ref_axis',(-0.573462344363328,0.819231920519041,3.92980824865032E-16)) ;
#83550=DIRECTION('center_axis',(0.710669054518701,0.497468338163091,0.497468338163092)) ;
#83551=DIRECTION('ref_axis',(0.57346234436333,-1.81382726107456E-15,-0.819231920519039)) ;
#83552=DIRECTION('center_axis',(-0.710669054518702,0.497468338163091,-0.497468338163091)) ;
#83553=DIRECTION('ref_axis',(-0.573462344363328,-0.819231920519041,6.69271761853466E-16)) ;
#83554=DIRECTION('center_axis',(0.710669054518702,-0.497468338163091,0.497468338163091)) ;
#83555=DIRECTION('ref_axis',(-0.573462344363335,-0.819231920519036,1.5770623553551E-14)) ;
#83556=DIRECTION('center_axis',(0.7106690545187,-0.497468338163094,0.497468338163091)) ;
#83557=DIRECTION('ref_axis',(0.573462344363331,0.819231920519038,2.86772422505918E-16)) ;
#83558=DIRECTION('center_axis',(0.,1.,-9.34081871679819E-17)) ;
#83559=DIRECTION('ref_axis',(0.,9.34081871679819E-17,1.)) ;
#83560=DIRECTION('center_axis',(-4.33680868994205E-15,-1.,-3.03576608295944E-15)) ;
#83561=DIRECTION('ref_axis',(1.,-4.33680868994205E-15,-1.12103877145985E-44)) ;
#83562=DIRECTION('center_axis',(0.,1.,5.29374964685745E-15)) ;
#83563=DIRECTION('ref_axis',(0.,-5.29374964685745E-15,1.)) ;
#83564=DIRECTION('center_axis',(0.,1.,0.)) ;
#83565=DIRECTION('ref_axis',(1.,0.,0.)) ;
#83566=DIRECTION('center_axis',(0.,6.45175738210751E-15,1.)) ;
#83567=DIRECTION('ref_axis',(0.,1.,-6.45175738210751E-15)) ;
#83568=DIRECTION('center_axis',(-1.,-6.67201336914158E-17,0.)) ;
#83569=DIRECTION('ref_axis',(6.67201336914158E-17,-1.,0.)) ;
#83570=DIRECTION('center_axis',(-1.,-6.67201336914158E-17,0.)) ;
#83571=DIRECTION('ref_axis',(6.67201336914158E-17,-1.,0.)) ;
#83572=DIRECTION('center_axis',(1.,-1.33440267382831E-16,0.)) ;
#83573=DIRECTION('ref_axis',(1.33440267382831E-16,1.,0.)) ;
#83574=DIRECTION('center_axis',(-1.,1.33440267382831E-16,0.)) ;
#83575=DIRECTION('ref_axis',(1.33440267382831E-16,1.,0.)) ;
#83576=DIRECTION('center_axis',(0.,1.,0.)) ;
#83577=DIRECTION('ref_axis',(1.,0.,0.)) ;
#83578=DIRECTION('center_axis',(1.76182853028896E-15,-1.23327997120227E-15,
1.)) ;
#83579=DIRECTION('ref_axis',(-1.,-2.1728278390981E-30,1.76182853028896E-15)) ;
#83580=DIRECTION('center_axis',(0.,0.,-1.)) ;
#83581=DIRECTION('ref_axis',(-1.,0.,0.)) ;
#83582=DIRECTION('center_axis',(-2.71050543121378E-16,-1.89735380184965E-16,
1.)) ;
#83583=DIRECTION('ref_axis',(1.,-5.14278778484758E-32,2.71050543121378E-16)) ;
#83584=DIRECTION('center_axis',(-0.710669054518702,-0.497468338163091,0.497468338163091)) ;
#83585=DIRECTION('ref_axis',(0.573462344363328,-0.819231920519041,3.92980824865032E-16)) ;
#83586=DIRECTION('center_axis',(0.710669054518702,0.497468338163091,-0.497468338163091)) ;
#83587=DIRECTION('ref_axis',(0.573462344363328,-0.819231920519041,3.92980824865032E-16)) ;
#83588=DIRECTION('center_axis',(0.710669054518701,0.497468338163091,-0.497468338163092)) ;
#83589=DIRECTION('ref_axis',(-0.57346234436333,1.88103289405095E-15,-0.819231920519039)) ;
#83590=DIRECTION('center_axis',(0.710669054518702,-0.497468338163091,-0.497468338163091)) ;
#83591=DIRECTION('ref_axis',(0.573462344363328,0.819231920519041,6.69271761853466E-16)) ;
#83592=DIRECTION('center_axis',(0.710669054518702,-0.497468338163091,-0.497468338163091)) ;
#83593=DIRECTION('ref_axis',(0.573462344363328,0.819231920519041,6.69271761853466E-16)) ;
#83594=DIRECTION('center_axis',(0.7106690545187,-0.497468338163091,-0.497468338163093)) ;
#83595=DIRECTION('ref_axis',(-0.573462344363331,-1.17187023180681E-15,-0.819231920519038)) ;
#83596=DIRECTION('center_axis',(0.,0.,-1.)) ;
#83597=DIRECTION('ref_axis',(-1.,0.,0.)) ;
#83598=DIRECTION('center_axis',(0.,1.15800773525007E-15,1.)) ;
#83599=DIRECTION('ref_axis',(0.,-1.,1.15800773525007E-15)) ;
#83600=DIRECTION('center_axis',(0.,1.,0.)) ;
#83601=DIRECTION('ref_axis',(1.,0.,0.)) ;
#83602=DIRECTION('center_axis',(0.,1.,0.)) ;
#83603=DIRECTION('ref_axis',(0.,0.,-1.)) ;
#83604=DIRECTION('center_axis',(0.,1.,0.)) ;
#83605=DIRECTION('ref_axis',(1.,0.,0.)) ;
#83606=DIRECTION('center_axis',(4.33680868994204E-15,-1.,-3.03576608295944E-15)) ;
#83607=DIRECTION('ref_axis',(-1.,-4.33680868994204E-15,5.60519385729927E-45)) ;
#83608=DIRECTION('center_axis',(0.,1.,9.34081871679819E-17)) ;
#83609=DIRECTION('ref_axis',(0.,-9.34081871679819E-17,1.)) ;
#83610=DIRECTION('center_axis',(0.,0.,1.)) ;
#83611=DIRECTION('ref_axis',(1.,0.,0.)) ;
#83612=DIRECTION('center_axis',(-2.16840434497102E-15,-3.61400724161847E-16,
1.)) ;
#83613=DIRECTION('ref_axis',(1.,-7.83662900548222E-31,2.16840434497102E-15)) ;
#83614=DIRECTION('center_axis',(0.973328526784575,0.162221421130762,-0.162221421130763)) ;
#83615=DIRECTION('ref_axis',(-0.164398987305358,9.23743777622416E-16,-0.986393923832144)) ;
#83616=DIRECTION('center_axis',(0.973328526784574,0.162221421130765,-0.162221421130767)) ;
#83617=DIRECTION('ref_axis',(-0.164398987305362,1.88956506020588E-16,-0.986393923832143)) ;
#83618=DIRECTION('center_axis',(0.,1.,0.)) ;
#83619=DIRECTION('ref_axis',(1.,0.,0.)) ;
#83620=DIRECTION('center_axis',(0.,1.,-8.79325913341701E-15)) ;
#83621=DIRECTION('ref_axis',(0.,-8.79325913341701E-15,-1.)) ;
#83622=DIRECTION('center_axis',(0.,0.,1.)) ;
#83623=DIRECTION('ref_axis',(1.,0.,0.)) ;
#83624=DIRECTION('center_axis',(0.,-2.28569887277128E-15,1.)) ;
#83625=DIRECTION('ref_axis',(0.,-1.,-2.28569887277128E-15)) ;
#83626=DIRECTION('center_axis',(1.73472347597681E-15,-1.,-2.89120579329468E-16)) ;
#83627=DIRECTION('ref_axis',(1.,1.73472347597681E-15,5.01544256350843E-31)) ;
#83628=DIRECTION('center_axis',(8.67361737988409E-15,1.,-1.44560289664739E-15)) ;
#83629=DIRECTION('ref_axis',(-1.,8.67361737988409E-15,-1.40129846432482E-45)) ;
#83630=DIRECTION('center_axis',(0.,1.,0.)) ;
#83631=DIRECTION('ref_axis',(1.,0.,0.)) ;
#83632=DIRECTION('center_axis',(-0.937042571331634,0.312347523777217,0.156173761888611)) ;
#83633=DIRECTION('ref_axis',(0.316227766016843,0.948683298050512,6.71158276827649E-18)) ;
#83634=DIRECTION('center_axis',(0.937042571331636,-0.312347523777212,-0.156173761888606)) ;
#83635=DIRECTION('ref_axis',(0.316227766016838,0.948683298050514,8.61595672567599E-16)) ;
#83636=DIRECTION('center_axis',(-0.973328526784575,-0.162221421130762,-0.162221421130763)) ;
#83637=DIRECTION('ref_axis',(-0.164398987305358,9.23743777622416E-16,0.986393923832144)) ;
#83638=DIRECTION('center_axis',(0.978231976292141,-0.146734796047223,-0.146734795425461)) ;
#83639=DIRECTION('ref_axis',(0.18231863354965,0.945435290900637,0.270022270526369)) ;
#83640=DIRECTION('center_axis',(0.973328526784574,0.162221421130767,0.162221421130768)) ;
#83641=DIRECTION('ref_axis',(0.164398987305363,-6.69215935033609E-18,-0.986393923832143)) ;
#83642=DIRECTION('center_axis',(0.,0.,1.)) ;
#83643=DIRECTION('ref_axis',(1.,0.,0.)) ;
#83644=DIRECTION('center_axis',(0.,2.19831478335425E-15,-1.)) ;
#83645=DIRECTION('ref_axis',(0.,1.,2.19831478335425E-15)) ;
#83646=DIRECTION('center_axis',(0.,1.,0.)) ;
#83647=DIRECTION('ref_axis',(1.,0.,0.)) ;
#83648=DIRECTION('center_axis',(8.67361737988408E-15,1.,1.44560289664739E-15)) ;
#83649=DIRECTION('ref_axis',(1.,-8.67361737988408E-15,5.60519385729927E-45)) ;
#83650=DIRECTION('center_axis',(1.73472347597681E-15,-1.,2.89120579329468E-16)) ;
#83651=DIRECTION('ref_axis',(1.,1.73472347597681E-15,-5.01544256350843E-31)) ;
#83652=DIRECTION('center_axis',(0.,1.,0.)) ;
#83653=DIRECTION('ref_axis',(0.,0.,1.)) ;
#83654=DIRECTION('center_axis',(0.,0.,1.)) ;
#83655=DIRECTION('ref_axis',(1.,0.,0.)) ;
#83656=DIRECTION('center_axis',(3.25260651745652E-15,-1.08420217248553E-15,
-1.)) ;
#83657=DIRECTION('ref_axis',(-1.,-3.52648305246695E-30,-3.25260651745652E-15)) ;
#83658=DIRECTION('center_axis',(0.,1.,0.)) ;
#83659=DIRECTION('ref_axis',(1.,0.,0.)) ;
#83660=DIRECTION('center_axis',(-0.937042571331635,0.312347523777215,-0.15617376188861)) ;
#83661=DIRECTION('ref_axis',(0.316227766016841,0.948683298050513,6.5590042956861E-18)) ;
#83662=DIRECTION('center_axis',(-0.937042571331636,0.312347523777212,-0.156173761888606)) ;
#83663=DIRECTION('ref_axis',(0.331350514299576,0.6540349591596,-0.680033167478254)) ;
#83664=DIRECTION('center_axis',(0.961519724091092,0.245047216428837,-0.12422432090484)) ;
#83665=DIRECTION('ref_axis',(0.262092069901281,-0.682554728284,0.682221950535173)) ;
#83666=DIRECTION('center_axis',(2.65552944032596E-32,3.29043518662928E-48,
-1.)) ;
#83667=DIRECTION('ref_axis',(-1.,8.7378475095785E-80,-2.65552944032596E-32)) ;
#83668=DIRECTION('center_axis',(2.65552944032596E-32,3.29043518662928E-48,
-1.)) ;
#83669=DIRECTION('ref_axis',(-1.,8.7378475095785E-80,-2.65552944032596E-32)) ;
#83670=DIRECTION('center_axis',(-2.65552944032596E-32,-3.29043518662928E-48,
1.)) ;
#83671=DIRECTION('ref_axis',(-1.,8.7378475095785E-80,-2.65552944032596E-32)) ;
#83672=DIRECTION('center_axis',(0.,0.,1.)) ;
#83673=DIRECTION('ref_axis',(1.,0.,0.)) ;
#83674=DIRECTION('center_axis',(0.,0.,-1.)) ;
#83675=DIRECTION('ref_axis',(-1.,0.,0.)) ;
#83676=DIRECTION('center_axis',(0.,0.,1.)) ;
#83677=DIRECTION('ref_axis',(1.,0.,0.)) ;
#83678=DIRECTION('center_axis',(0.,0.,1.)) ;
#83679=DIRECTION('ref_axis',(1.,0.,0.)) ;
#83680=DIRECTION('center_axis',(0.,0.,-1.)) ;
#83681=DIRECTION('ref_axis',(-1.,0.,0.)) ;
#83682=DIRECTION('center_axis',(0.,0.,-1.)) ;
#83683=DIRECTION('ref_axis',(-1.,0.,0.)) ;
#83684=DIRECTION('center_axis',(1.,1.15648231731787E-15,0.)) ;
#83685=DIRECTION('ref_axis',(1.03435541192675E-15,-1.,5.17177705963374E-16)) ;
#83686=DIRECTION('center_axis',(7.089177613099E-16,-0.612994899008946,-0.790086864711098)) ;
#83687=DIRECTION('ref_axis',(1.7347234759768E-14,-0.790086864711098,0.612994899008946)) ;
#83688=DIRECTION('center_axis',(7.08917761309899E-16,-0.612994899008945,
0.790086864711098)) ;
#83689=DIRECTION('ref_axis',(-1.7347234759768E-14,0.790086864711098,0.612994899008945)) ;
#83690=DIRECTION('center_axis',(0.,0.,-1.)) ;
#83691=DIRECTION('ref_axis',(-1.,0.,0.)) ;
#83692=DIRECTION('center_axis',(0.,0.,1.)) ;
#83693=DIRECTION('ref_axis',(-1.,2.16840434497102E-15,0.)) ;
#83694=DIRECTION('center_axis',(1.08420217248551E-15,-1.,0.)) ;
#83695=DIRECTION('ref_axis',(1.,1.08420217248551E-15,0.)) ;
#83696=DIRECTION('center_axis',(1.44560289664734E-16,-1.,-2.4093381610789E-16)) ;
#83697=DIRECTION('ref_axis',(2.28544744656275E-46,2.4093381610789E-16,-1.)) ;
#83698=DIRECTION('center_axis',(0.,-1.,0.)) ;
#83699=DIRECTION('ref_axis',(0.,0.,-1.)) ;
#83700=DIRECTION('center_axis',(1.,0.,0.)) ;
#83701=DIRECTION('ref_axis',(0.,1.,0.)) ;
#83702=DIRECTION('center_axis',(1.,0.,0.)) ;
#83703=DIRECTION('ref_axis',(0.,0.,-1.)) ;
#83704=DIRECTION('center_axis',(1.,1.23908819712629E-16,8.95614743483648E-33)) ;
#83705=DIRECTION('ref_axis',(-1.23908819712629E-16,1.,-1.10974565782288E-48)) ;
#83706=DIRECTION('center_axis',(1.,0.,0.)) ;
#83707=DIRECTION('ref_axis',(0.,0.,-1.)) ;
#83708=DIRECTION('center_axis',(-1.,0.,0.)) ;
#83709=DIRECTION('ref_axis',(0.,0.,1.)) ;
#83710=DIRECTION('center_axis',(1.,1.23908819712629E-16,8.95614743483648E-33)) ;
#83711=DIRECTION('ref_axis',(-1.23908819712629E-16,1.,-1.10974565782288E-48)) ;
#83712=DIRECTION('center_axis',(-1.,0.,0.)) ;
#83713=DIRECTION('ref_axis',(0.,0.,1.)) ;
#83714=DIRECTION('center_axis',(1.,0.,0.)) ;
#83715=DIRECTION('ref_axis',(0.,-1.,0.)) ;
#83716=DIRECTION('center_axis',(0.,1.,0.)) ;
#83717=DIRECTION('ref_axis',(0.,0.,1.)) ;
#83718=DIRECTION('center_axis',(-1.44560289664734E-16,1.,-7.2280144832367E-17)) ;
#83719=DIRECTION('ref_axis',(0.707106781238332,1.5332934167208E-16,0.707106781134763)) ;
#83720=DIRECTION('center_axis',(-1.0842021724855E-15,1.,0.)) ;
#83721=DIRECTION('ref_axis',(-1.,-1.0842021724855E-15,0.)) ;
#83722=DIRECTION('center_axis',(0.,1.,0.)) ;
#83723=DIRECTION('ref_axis',(0.,0.,1.)) ;
#83724=DIRECTION('center_axis',(0.,-1.,0.)) ;
#83725=DIRECTION('ref_axis',(0.,0.,-1.)) ;
#83726=DIRECTION('center_axis',(0.,1.,0.)) ;
#83727=DIRECTION('ref_axis',(0.,0.,1.)) ;
#83728=DIRECTION('center_axis',(0.,0.,1.)) ;
#83729=DIRECTION('ref_axis',(1.,0.,0.)) ;
#83730=DIRECTION('center_axis',(0.431191646768307,0.0335421424106918,0.901636672080133)) ;
#83731=DIRECTION('ref_axis',(0.899826811386771,0.0573593265856512,-0.432459960184937)) ;
#83732=DIRECTION('center_axis',(0.,0.,1.)) ;
#83733=DIRECTION('ref_axis',(-1.,0.,0.)) ;
#83734=DIRECTION('center_axis',(0.,0.,-1.)) ;
#83735=DIRECTION('ref_axis',(0.707109343403326,-0.707104218960485,0.)) ;
#83736=DIRECTION('center_axis',(-3.25260651745653E-15,0.,1.)) ;
#83737=DIRECTION('ref_axis',(1.,0.,3.25260651745653E-15)) ;
#83738=DIRECTION('center_axis',(0.,0.,1.)) ;
#83739=DIRECTION('ref_axis',(1.,0.,0.)) ;
#83740=DIRECTION('center_axis',(0.431188264322452,0.0335835001127062,-0.901636750155389)) ;
#83741=DIRECTION('ref_axis',(0.899831768110909,0.0572892330930879,0.432458937784851)) ;
#83742=DIRECTION('center_axis',(0.,-1.,0.)) ;
#83743=DIRECTION('ref_axis',(0.,0.,-1.)) ;
#83744=DIRECTION('center_axis',(0.,1.,0.)) ;
#83745=DIRECTION('ref_axis',(0.,0.,1.)) ;
#83746=DIRECTION('center_axis',(0.,0.,1.)) ;
#83747=DIRECTION('ref_axis',(1.,0.,0.)) ;
#83748=DIRECTION('center_axis',(0.,0.,-1.)) ;
#83749=DIRECTION('ref_axis',(-1.,0.,0.)) ;
#83750=DIRECTION('center_axis',(0.,0.,1.)) ;
#83751=DIRECTION('ref_axis',(-0.986393923832144,0.164398987305354,0.)) ;
#83752=DIRECTION('center_axis',(0.98470178743927,-0.164116964573216,0.0585492250433781)) ;
#83753=DIRECTION('ref_axis',(0.164398987305362,0.986393923832143,-7.60669428566932E-17)) ;
#83754=DIRECTION('center_axis',(0.984834538781277,-0.164139089796902,0.0562075655416074)) ;
#83755=DIRECTION('ref_axis',(0.164398987305379,0.98639392383214,1.87706412796466E-17)) ;
#83756=DIRECTION('center_axis',(0.986393923832145,-0.129889480441767,0.100775740620414)) ;
#83757=DIRECTION('ref_axis',(0.,0.612994899008951,0.790086864711094)) ;
#83758=DIRECTION('center_axis',(0.,1.,0.)) ;
#83759=DIRECTION('ref_axis',(1.,0.,0.)) ;
#83760=DIRECTION('center_axis',(0.,0.,-1.)) ;
#83761=DIRECTION('ref_axis',(-1.,0.,0.)) ;
#83762=DIRECTION('center_axis',(1.,2.8359373108165E-15,0.)) ;
#83763=DIRECTION('ref_axis',(-2.8359373108165E-15,1.,0.)) ;
#83764=DIRECTION('center_axis',(0.,0.,-1.)) ;
#83765=DIRECTION('ref_axis',(-1.,0.,0.)) ;
#83766=DIRECTION('center_axis',(0.,0.,1.)) ;
#83767=DIRECTION('ref_axis',(1.,0.,0.)) ;
#83768=DIRECTION('center_axis',(1.,0.,0.)) ;
#83769=DIRECTION('ref_axis',(0.,0.,-1.)) ;
#83770=DIRECTION('center_axis',(1.,0.,0.)) ;
#83771=DIRECTION('ref_axis',(0.,0.,-1.)) ;
#83772=DIRECTION('center_axis',(0.,1.,0.)) ;
#83773=DIRECTION('ref_axis',(1.,0.,0.)) ;
#83774=DIRECTION('center_axis',(1.,-8.50781193244945E-15,0.)) ;
#83775=DIRECTION('ref_axis',(8.50781193244945E-15,1.,0.)) ;
#83776=DIRECTION('center_axis',(0.,1.,0.)) ;
#83777=DIRECTION('ref_axis',(1.,0.,0.)) ;
#83778=DIRECTION('center_axis',(-5.42101086242753E-16,1.70882313734897E-16,
1.)) ;
#83779=DIRECTION('ref_axis',(1.,9.26354878953623E-32,5.42101086242753E-16)) ;
#83780=DIRECTION('center_axis',(-1.,0.,0.)) ;
#83781=DIRECTION('ref_axis',(0.,0.,1.)) ;
#83782=DIRECTION('center_axis',(1.,0.,0.)) ;
#83783=DIRECTION('ref_axis',(0.,0.,-1.)) ;
#83784=DIRECTION('center_axis',(0.,0.,-1.)) ;
#83785=DIRECTION('ref_axis',(-1.,0.,0.)) ;
#83786=DIRECTION('center_axis',(0.,0.,1.)) ;
#83787=DIRECTION('ref_axis',(1.,0.,0.)) ;
#83788=DIRECTION('center_axis',(0.,1.,0.)) ;
#83789=DIRECTION('ref_axis',(1.,0.,0.)) ;
#83790=DIRECTION('center_axis',(0.,1.,0.)) ;
#83791=DIRECTION('ref_axis',(1.,0.,0.)) ;
#83792=DIRECTION('center_axis',(0.,0.,-1.)) ;
#83793=DIRECTION('ref_axis',(-1.,0.,0.)) ;
#83794=DIRECTION('center_axis',(0.,1.,0.)) ;
#83795=DIRECTION('ref_axis',(0.,0.,1.)) ;
#83796=DIRECTION('center_axis',(0.,0.,-1.)) ;
#83797=DIRECTION('ref_axis',(-1.,0.,0.)) ;
#83798=DIRECTION('center_axis',(0.,0.,1.)) ;
#83799=DIRECTION('ref_axis',(1.,0.,0.)) ;
#83800=DIRECTION('center_axis',(1.33440267382831E-16,1.,0.)) ;
#83801=DIRECTION('ref_axis',(-1.,1.33440267382831E-16,0.)) ;
#83802=DIRECTION('center_axis',(0.,1.,0.)) ;
#83803=DIRECTION('ref_axis',(0.,0.,1.)) ;
#83804=DIRECTION('center_axis',(0.,1.,0.)) ;
#83805=DIRECTION('ref_axis',(1.,0.,0.)) ;
#83806=DIRECTION('center_axis',(0.,1.,0.)) ;
#83807=DIRECTION('ref_axis',(0.,0.,1.)) ;
#83808=DIRECTION('center_axis',(0.,1.,0.)) ;
#83809=DIRECTION('ref_axis',(1.,0.,0.)) ;
#83810=DIRECTION('center_axis',(1.37797793267296E-15,-1.62630325872825E-15,
1.)) ;
#83811=DIRECTION('ref_axis',(-2.24101000236165E-30,-1.,-1.62630325872825E-15)) ;
#83812=DIRECTION('center_axis',(-1.33440267382831E-16,-1.,0.)) ;
#83813=DIRECTION('ref_axis',(1.,-1.33440267382831E-16,0.)) ;
#83814=DIRECTION('center_axis',(0.,1.,0.)) ;
#83815=DIRECTION('ref_axis',(0.,0.,1.)) ;
#83816=DIRECTION('center_axis',(0.,0.,-1.)) ;
#83817=DIRECTION('ref_axis',(-1.,0.,0.)) ;
#83818=DIRECTION('center_axis',(0.,0.,1.)) ;
#83819=DIRECTION('ref_axis',(1.,0.,0.)) ;
#83820=DIRECTION('center_axis',(0.,1.,0.)) ;
#83821=DIRECTION('ref_axis',(1.,0.,0.)) ;
#83822=DIRECTION('center_axis',(0.,0.,1.)) ;
#83823=DIRECTION('ref_axis',(1.,0.,0.)) ;
#83824=DIRECTION('center_axis',(0.,0.,1.)) ;
#83825=DIRECTION('ref_axis',(1.,0.,0.)) ;
#83826=DIRECTION('center_axis',(0.,0.,1.)) ;
#83827=DIRECTION('ref_axis',(-0.986393923832144,0.164398987305354,0.)) ;
#83828=DIRECTION('center_axis',(0.984701787439272,-0.164116964573205,-0.0585492250433871)) ;
#83829=DIRECTION('ref_axis',(0.16439898730535,0.986393923832145,-3.2807868055655E-16)) ;
#83830=DIRECTION('center_axis',(0.984834538781259,-0.164139089796881,-0.0562075655419907)) ;
#83831=DIRECTION('ref_axis',(0.164398987305362,0.986393923832143,6.03508511856301E-17)) ;
#83832=DIRECTION('center_axis',(0.,0.,1.)) ;
#83833=DIRECTION('ref_axis',(-0.986393923832144,0.164398987305354,0.)) ;
#83834=DIRECTION('center_axis',(0.,0.,1.)) ;
#83835=DIRECTION('ref_axis',(1.,0.,0.)) ;
#83836=DIRECTION('center_axis',(0.342346838789899,0.100237737301556,-0.934211452504853)) ;
#83837=DIRECTION('ref_axis',(0.878411850385613,0.318727802083594,0.356097190779547)) ;
#83838=DIRECTION('center_axis',(0.,0.,-1.)) ;
#83839=DIRECTION('ref_axis',(-1.,0.,0.)) ;
#83840=DIRECTION('center_axis',(0.,0.,-1.)) ;
#83841=DIRECTION('ref_axis',(-1.,0.,0.)) ;
#83842=DIRECTION('center_axis',(0.,0.,-1.)) ;
#83843=DIRECTION('ref_axis',(-1.,0.,0.)) ;
#83844=DIRECTION('center_axis',(-0.342346838789825,-0.100237737307746,-0.934211452504216)) ;
#83845=DIRECTION('ref_axis',(0.878411777618972,0.318728007761553,-0.356097186184654)) ;
#83846=DIRECTION('center_axis',(0.,0.,1.)) ;
#83847=DIRECTION('ref_axis',(1.,0.,0.)) ;
#83848=DIRECTION('center_axis',(0.967224433240076,0.25169685099469,0.0335498277606827)) ;
#83849=DIRECTION('ref_axis',(0.148186139673085,-0.66680383883963,0.730351633473576)) ;
#83850=DIRECTION('center_axis',(0.,0.707106781186549,-0.707106781186547)) ;
#83851=DIRECTION('ref_axis',(0.,0.707106781186546,0.707106781186549)) ;
#83852=DIRECTION('center_axis',(0.978007532938602,-0.147978541149587,-0.146981688909158)) ;
#83853=DIRECTION('ref_axis',(0.193734423938717,0.383507624691585,0.902988856401092)) ;
#83854=DIRECTION('center_axis',(0.,0.447213595499958,0.894427190999916)) ;
#83855=DIRECTION('ref_axis',(0.,-0.894427190999916,0.447213595499958)) ;
#83856=DIRECTION('center_axis',(0.960001452008135,0.250435160947725,-0.125217579849475)) ;
#83857=DIRECTION('ref_axis',(0.276742394168204,-0.916645079797436,0.288401534242108)) ;
#83858=DIRECTION('center_axis',(0.,1.,0.)) ;
#83859=DIRECTION('ref_axis',(0.,0.,1.)) ;
#83860=DIRECTION('center_axis',(-1.,0.,0.)) ;
#83861=DIRECTION('ref_axis',(0.,0.413905168515859,-0.910320004984982)) ;
#83862=DIRECTION('center_axis',(1.,1.44560289664734E-16,0.)) ;
#83863=DIRECTION('ref_axis',(0.,1.,0.)) ;
#83864=DIRECTION('center_axis',(1.,1.44560289664734E-16,0.)) ;
#83865=DIRECTION('ref_axis',(-1.44560289664734E-16,1.,0.)) ;
#83866=DIRECTION('center_axis',(0.,0.,-1.)) ;
#83867=DIRECTION('ref_axis',(0.,-1.,0.)) ;
#83868=DIRECTION('center_axis',(-1.,-1.44560289664734E-16,0.)) ;
#83869=DIRECTION('ref_axis',(-1.44560289664734E-16,1.,0.)) ;
#83870=DIRECTION('center_axis',(1.,-3.46944695195361E-16,0.)) ;
#83871=DIRECTION('ref_axis',(2.61228946970625E-16,1.,0.)) ;
#83872=DIRECTION('center_axis',(1.,-3.46944695195361E-16,0.)) ;
#83873=DIRECTION('ref_axis',(3.46944695195361E-16,1.,0.)) ;
#83874=DIRECTION('center_axis',(0.,0.,1.)) ;
#83875=DIRECTION('ref_axis',(-3.26536183713281E-16,-1.,0.)) ;
#83876=DIRECTION('center_axis',(-1.,3.46944695195361E-16,0.)) ;
#83877=DIRECTION('ref_axis',(3.46944695195361E-16,1.,0.)) ;
#83878=DIRECTION('center_axis',(-1.,3.46944695195361E-16,0.)) ;
#83879=DIRECTION('ref_axis',(-3.46944695195361E-16,-1.,0.)) ;
#83880=DIRECTION('center_axis',(-1.,0.,0.)) ;
#83881=DIRECTION('ref_axis',(0.,0.,1.)) ;
#83882=DIRECTION('',(1.,-3.46944695195361E-16,0.)) ;
#83883=DIRECTION('center_axis',(-1.,8.01625584951926E-16,-1.08420217248551E-15)) ;
#83884=DIRECTION('ref_axis',(1.08420217248551E-15,2.16840434497102E-15,
-1.)) ;
#83885=DIRECTION('center_axis',(-1.,8.01625584951926E-16,-1.08420217248551E-15)) ;
#83886=DIRECTION('ref_axis',(1.08420217248551E-15,2.16840434497102E-15,
-1.)) ;
#83887=DIRECTION('',(-1.,3.46944695195361E-16,0.)) ;
#83888=DIRECTION('center_axis',(-1.,3.46944695195361E-16,0.)) ;
#83889=DIRECTION('ref_axis',(-3.46944695195361E-16,-1.,0.)) ;
#83890=DIRECTION('center_axis',(-1.,0.,0.)) ;
#83891=DIRECTION('ref_axis',(0.,0.,1.)) ;
#83892=DIRECTION('',(1.,-3.46944695195361E-16,0.)) ;
#83893=DIRECTION('center_axis',(-1.,2.2680138501079E-15,0.)) ;
#83894=DIRECTION('ref_axis',(2.2680138501079E-15,1.,0.)) ;
#83895=DIRECTION('',(-1.,3.46944695195361E-16,0.)) ;
#83896=DIRECTION('center_axis',(-1.,3.18032637262401E-16,0.)) ;
#83897=DIRECTION('ref_axis',(-5.55111512312578E-16,-1.,0.)) ;
#83898=DIRECTION('center_axis',(1.,-3.18032637262401E-16,0.)) ;
#83899=DIRECTION('ref_axis',(-3.18032637262401E-16,-1.,0.)) ;
#83900=DIRECTION('center_axis',(-2.01298417874256E-16,-0.632948931301568,
-0.774193548387096)) ;
#83901=DIRECTION('ref_axis',(1.73472347597681E-14,-0.774193548387096,0.632948931301568)) ;
#83902=DIRECTION('center_axis',(-1.,3.18032637262401E-16,0.)) ;
#83903=DIRECTION('ref_axis',(-3.18032637262401E-16,-1.,0.)) ;
#83904=DIRECTION('center_axis',(-2.01298417874256E-16,-0.632948931301568,
0.774193548387096)) ;
#83905=DIRECTION('ref_axis',(-2.5982535921668E-30,-0.774193548387096,-0.632948931301568)) ;
#83906=DIRECTION('center_axis',(1.,1.44560289664734E-16,0.)) ;
#83907=DIRECTION('ref_axis',(-1.44560289664734E-16,1.,0.)) ;
#83908=DIRECTION('',(-1.,-1.44560289664734E-16,0.)) ;
#83909=DIRECTION('center_axis',(-1.,3.46944695195361E-16,0.)) ;
#83910=DIRECTION('ref_axis',(-3.46944695195361E-16,-1.,0.)) ;
#83911=DIRECTION('',(-1.,3.46944695195361E-16,0.)) ;
#83912=DIRECTION('center_axis',(-1.,3.46944695195361E-16,0.)) ;
#83913=DIRECTION('ref_axis',(3.46944695195361E-16,1.,0.)) ;
#83914=DIRECTION('center_axis',(-1.,3.46944695195361E-16,0.)) ;
#83915=DIRECTION('ref_axis',(3.46944695195361E-16,1.,0.)) ;
#83916=DIRECTION('center_axis',(-1.,3.46944695195361E-16,0.)) ;
#83917=DIRECTION('ref_axis',(-3.46944695195361E-16,-1.,0.)) ;
#83918=DIRECTION('',(1.,-3.46944695195361E-16,0.)) ;
#83919=DIRECTION('center_axis',(-1.,-1.44560289664734E-16,-2.65552944032596E-32)) ;
#83920=DIRECTION('ref_axis',(1.44560289664734E-16,-1.,-2.80018320648271E-64)) ;
#83921=DIRECTION('',(2.65552944032596E-32,3.29043518662928E-48,-1.)) ;
#83922=DIRECTION('',(1.44560289664734E-16,-1.,-2.4093381610789E-16)) ;
#83923=DIRECTION('',(0.,0.,1.)) ;
#83924=DIRECTION('center_axis',(0.999999956301289,0.000282786981395913,
8.61913163589487E-5)) ;
#83925=DIRECTION('ref_axis',(0.000288266391231008,-0.997396273404988,-0.0721151211628269)) ;
#83926=DIRECTION('',(-1.44560289664734E-16,1.,-7.2280144832367E-17)) ;
#83927=DIRECTION('center_axis',(0.316227766016838,0.948683298050514,0.)) ;
#83928=DIRECTION('ref_axis',(-0.948683298050514,0.316227766016838,0.)) ;
#83929=DIRECTION('',(-0.948683298050514,0.316227766016838,0.)) ;
#83930=DIRECTION('',(0.,0.,1.)) ;
#83931=DIRECTION('',(0.937042571331636,-0.312347523777212,-0.156173761888606)) ;
#83932=DIRECTION('',(0.,0.,-1.)) ;
#83933=DIRECTION('center_axis',(1.,1.73472347597681E-15,0.)) ;
#83934=DIRECTION('ref_axis',(-1.73472347597681E-15,1.,0.)) ;
#83935=DIRECTION('',(-1.73472347597681E-15,1.,0.)) ;
#83936=DIRECTION('',(0.,0.,1.)) ;
#83937=DIRECTION('',(1.73472347597681E-15,-1.,-2.89120579329468E-16)) ;
#83938=DIRECTION('',(0.,0.,-1.)) ;
#83939=DIRECTION('center_axis',(0.164398987305357,-0.986393923832144,0.)) ;
#83940=DIRECTION('ref_axis',(0.986393923832144,0.164398987305357,0.)) ;
#83941=DIRECTION('',(-0.973328526784575,-0.162221421130762,0.162221421130763)) ;
#83942=DIRECTION('',(0.,0.,-1.)) ;
#83943=DIRECTION('',(0.986393923832144,0.164398987305357,0.)) ;
#83944=DIRECTION('',(0.,0.,1.)) ;
#83945=DIRECTION('center_axis',(-9.91270557701033E-17,1.,0.)) ;
#83946=DIRECTION('ref_axis',(-1.,-9.91270557701033E-17,0.)) ;
#83947=DIRECTION('',(1.,9.91270557701033E-17,0.)) ;
#83948=DIRECTION('',(0.,0.,-1.)) ;
#83949=DIRECTION('',(-1.,-9.91270557701033E-17,0.)) ;
#83950=DIRECTION('',(0.,0.,1.)) ;
#83951=DIRECTION('center_axis',(-9.91270557701033E-17,1.,0.)) ;
#83952=DIRECTION('ref_axis',(-1.,-9.91270557701033E-17,0.)) ;
#83953=DIRECTION('',(-1.,-9.91270557701033E-17,0.)) ;
#83954=DIRECTION('',(0.,0.,-1.)) ;
#83955=DIRECTION('',(-1.,-9.91270557701033E-17,0.)) ;
#83956=DIRECTION('',(0.,0.,1.)) ;
#83957=DIRECTION('center_axis',(1.,1.15648231731787E-15,0.)) ;
#83958=DIRECTION('ref_axis',(-1.15648231731787E-15,1.,0.)) ;
#83959=DIRECTION('',(-1.15648231731787E-15,1.,0.)) ;
#83960=DIRECTION('',(0.,0.,-1.)) ;
#83961=DIRECTION('',(-1.15648231731787E-15,1.,0.)) ;
#83962=DIRECTION('',(0.,0.,1.)) ;
#83963=DIRECTION('center_axis',(-1.,-1.15648231731787E-15,0.)) ;
#83964=DIRECTION('ref_axis',(-1.15648231731787E-15,1.,0.)) ;
#83965=DIRECTION('',(0.,0.,1.)) ;
#83966=DIRECTION('center_axis',(0.,0.,1.)) ;
#83967=DIRECTION('ref_axis',(1.,0.,0.)) ;
#83968=DIRECTION('',(-1.,0.,0.)) ;
#83969=DIRECTION('center_axis',(0.,0.,-1.)) ;
#83970=DIRECTION('ref_axis',(1.,0.,0.)) ;
#83971=DIRECTION('center_axis',(0.,0.,-1.)) ;
#83972=DIRECTION('ref_axis',(1.,0.,0.)) ;
#83973=DIRECTION('center_axis',(0.,0.,-1.)) ;
#83974=DIRECTION('ref_axis',(1.,0.,0.)) ;
#83975=DIRECTION('center_axis',(0.,0.,-1.)) ;
#83976=DIRECTION('ref_axis',(1.,0.,0.)) ;
#83977=DIRECTION('',(1.,0.,0.)) ;
#83978=DIRECTION('center_axis',(0.,0.,1.)) ;
#83979=DIRECTION('ref_axis',(1.,0.,0.)) ;
#83980=DIRECTION('',(3.46944695195361E-16,1.,0.)) ;
#83981=DIRECTION('center_axis',(0.,0.,1.)) ;
#83982=DIRECTION('ref_axis',(1.,0.,0.)) ;
#83983=DIRECTION('',(1.,-3.46944695195361E-16,0.)) ;
#83984=DIRECTION('center_axis',(0.,0.,-1.)) ;
#83985=DIRECTION('ref_axis',(1.,0.,0.)) ;
#83986=DIRECTION('',(2.71050543121376E-16,1.,0.)) ;
#83987=DIRECTION('center_axis',(0.,0.,-1.)) ;
#83988=DIRECTION('ref_axis',(1.,0.,0.)) ;
#83989=DIRECTION('',(-1.,3.46944695195361E-16,0.)) ;
#83990=DIRECTION('center_axis',(0.,0.,1.)) ;
#83991=DIRECTION('ref_axis',(1.,0.,0.)) ;
#83992=DIRECTION('',(3.46944695195361E-16,1.,0.)) ;
#83993=DIRECTION('center_axis',(0.,0.,1.)) ;
#83994=DIRECTION('ref_axis',(1.,0.,0.)) ;
#83995=DIRECTION('center_axis',(0.,0.,-1.)) ;
#83996=DIRECTION('ref_axis',(1.,0.,0.)) ;
#83997=DIRECTION('',(0.986393923832144,-0.164398987305354,0.)) ;
#83998=DIRECTION('center_axis',(0.,0.,-1.)) ;
#83999=DIRECTION('ref_axis',(1.,-6.50521303491307E-15,0.)) ;
#84000=DIRECTION('center_axis',(0.,0.,-1.)) ;
#84001=DIRECTION('ref_axis',(1.,0.,0.)) ;
#84002=DIRECTION('',(1.,0.,0.)) ;
#84003=DIRECTION('',(1.13380619344889E-16,-1.,0.)) ;
#84004=DIRECTION('center_axis',(0.,0.,-1.)) ;
#84005=DIRECTION('ref_axis',(1.,0.,0.)) ;
#84006=DIRECTION('',(-1.,-1.92747052886312E-16,0.)) ;
#84007=DIRECTION('center_axis',(0.,0.,1.)) ;
#84008=DIRECTION('ref_axis',(1.,0.,0.)) ;
#84009=DIRECTION('',(0.,-1.,0.)) ;
#84010=DIRECTION('center_axis',(0.,0.,-1.)) ;
#84011=DIRECTION('ref_axis',(1.,0.,0.)) ;
#84012=DIRECTION('center_axis',(0.,0.,1.)) ;
#84013=DIRECTION('ref_axis',(1.,0.,0.)) ;
#84014=DIRECTION('',(-0.948683298050514,0.316227766016838,0.)) ;
#84015=DIRECTION('center_axis',(0.,0.,1.)) ;
#84016=DIRECTION('ref_axis',(1.,0.,0.)) ;
#84017=DIRECTION('',(-1.,0.,0.)) ;
#84018=DIRECTION('center_axis',(0.,0.,1.)) ;
#84019=DIRECTION('ref_axis',(1.,0.,0.)) ;
#84020=DIRECTION('',(0.,-1.,0.)) ;
#84021=DIRECTION('center_axis',(0.,0.,-1.)) ;
#84022=DIRECTION('ref_axis',(1.,0.,0.)) ;
#84023=DIRECTION('',(-1.,-1.92747052886312E-16,0.)) ;
#84024=DIRECTION('center_axis',(0.,0.,1.)) ;
#84025=DIRECTION('ref_axis',(1.,0.,0.)) ;
#84026=DIRECTION('',(1.13380619344889E-16,-1.,0.)) ;
#84027=DIRECTION('',(1.,0.,0.)) ;
#84028=DIRECTION('center_axis',(0.,0.,1.)) ;
#84029=DIRECTION('ref_axis',(1.,0.,0.)) ;
#84030=DIRECTION('center_axis',(0.,0.,1.)) ;
#84031=DIRECTION('ref_axis',(1.,0.,0.)) ;
#84032=DIRECTION('',(-0.986393923832144,0.164398987305354,0.)) ;
#84033=DIRECTION('center_axis',(0.,0.,1.)) ;
#84034=DIRECTION('ref_axis',(1.,0.,0.)) ;
#84035=DIRECTION('center_axis',(0.,0.,-1.)) ;
#84036=DIRECTION('ref_axis',(1.,0.,0.)) ;
#84037=DIRECTION('',(-3.46944695195361E-16,-1.,0.)) ;
#84038=DIRECTION('center_axis',(0.,0.,-1.)) ;
#84039=DIRECTION('ref_axis',(1.,0.,0.)) ;
#84040=DIRECTION('',(-1.,3.46944695195361E-16,0.)) ;
#84041=DIRECTION('center_axis',(0.,0.,1.)) ;
#84042=DIRECTION('ref_axis',(1.,0.,0.)) ;
#84043=DIRECTION('',(3.46944695195361E-16,1.,0.)) ;
#84044=DIRECTION('center_axis',(0.,0.,1.)) ;
#84045=DIRECTION('ref_axis',(1.,0.,0.)) ;
#84046=DIRECTION('',(1.,-3.46944695195361E-16,0.)) ;
#84047=DIRECTION('center_axis',(0.,0.,-1.)) ;
#84048=DIRECTION('ref_axis',(1.,0.,0.)) ;
#84049=DIRECTION('',(-3.46944695195361E-16,-1.,0.)) ;
#84050=DIRECTION('center_axis',(0.,0.,-1.)) ;
#84051=DIRECTION('ref_axis',(1.,0.,0.)) ;
#84052=DIRECTION('',(1.,0.,0.)) ;
#84053=DIRECTION('center_axis',(0.,0.,1.)) ;
#84054=DIRECTION('ref_axis',(1.,0.,0.)) ;
#84055=DIRECTION('',(0.986393923832144,0.164398987305357,0.)) ;
#84056=DIRECTION('center_axis',(0.,0.,1.)) ;
#84057=DIRECTION('ref_axis',(1.,0.,0.)) ;
#84058=DIRECTION('',(-1.73472347597681E-15,1.,0.)) ;
#84059=DIRECTION('center_axis',(0.,0.,1.)) ;
#84060=DIRECTION('ref_axis',(1.,0.,0.)) ;
#84061=DIRECTION('center_axis',(-1.92747052886312E-16,1.,0.)) ;
#84062=DIRECTION('ref_axis',(-1.,-1.92747052886312E-16,0.)) ;
#84063=DIRECTION('',(0.,0.,1.)) ;
#84064=DIRECTION('',(0.,0.,-1.)) ;
#84065=DIRECTION('center_axis',(-1.,0.,0.)) ;
#84066=DIRECTION('ref_axis',(0.,0.,1.)) ;
#84067=DIRECTION('',(0.,0.,1.)) ;
#84068=DIRECTION('',(0.,0.,-1.)) ;
#84069=DIRECTION('center_axis',(0.,1.,0.)) ;
#84070=DIRECTION('ref_axis',(0.,0.,1.)) ;
#84071=DIRECTION('',(0.,0.,-1.)) ;
#84072=DIRECTION('',(0.,0.,1.)) ;
#84073=DIRECTION('',(0.,0.,-1.)) ;
#84074=DIRECTION('',(0.,0.,-1.)) ;
#84075=DIRECTION('center_axis',(0.316227766016838,0.948683298050514,0.)) ;
#84076=DIRECTION('ref_axis',(-0.948683298050514,0.316227766016838,0.)) ;
#84077=DIRECTION('center_axis',(-0.316227766016857,-0.948683298050507,-2.67178031360003E-14)) ;
#84078=DIRECTION('ref_axis',(0.831595960751158,-0.277198653583725,-0.48125779423686)) ;
#84079=DIRECTION('',(0.,0.,1.)) ;
#84080=DIRECTION('',(0.,0.,-1.)) ;
#84081=DIRECTION('',(-0.937042571331636,0.312347523777212,-0.156173761888606)) ;
#84082=DIRECTION('center_axis',(1.,1.73472347597681E-15,0.)) ;
#84083=DIRECTION('ref_axis',(-1.73472347597681E-15,1.,0.)) ;
#84084=DIRECTION('',(-1.73472347597681E-15,1.,-2.89120579329468E-16)) ;
#84085=DIRECTION('',(0.,0.,1.)) ;
#84086=DIRECTION('',(0.,0.,-1.)) ;
#84087=DIRECTION('center_axis',(0.164398987305357,-0.986393923832144,0.)) ;
#84088=DIRECTION('ref_axis',(0.986393923832144,0.164398987305357,0.)) ;
#84089=DIRECTION('',(0.973328526784575,0.162221421130762,0.162221421130763)) ;
#84090=DIRECTION('',(0.,0.,1.)) ;
#84091=DIRECTION('',(0.,0.,-1.)) ;
#84092=DIRECTION('center_axis',(0.,-1.,0.)) ;
#84093=DIRECTION('ref_axis',(0.,0.,-1.)) ;
#84094=DIRECTION('',(0.,0.,1.)) ;
#84095=DIRECTION('',(0.,0.,1.)) ;
#84096=DIRECTION('',(0.,0.,1.)) ;
#84097=DIRECTION('',(0.,0.,-1.)) ;
#84098=DIRECTION('',(1.,0.,2.25271179641597E-31)) ;
#84099=DIRECTION('center_axis',(0.,-1.,0.)) ;
#84100=DIRECTION('ref_axis',(0.,0.,-1.)) ;
#84101=DIRECTION('',(0.,0.,-1.)) ;
#84102=DIRECTION('center_axis',(0.,-1.,0.)) ;
#84103=DIRECTION('ref_axis',(0.,0.,-1.)) ;
#84104=DIRECTION('',(-1.,0.,-3.21815970916568E-32)) ;
#84105=DIRECTION('',(0.,0.,-1.)) ;
#84106=DIRECTION('center_axis',(1.,-3.46944695195361E-16,0.)) ;
#84107=DIRECTION('ref_axis',(3.46944695195361E-16,1.,0.)) ;
#84108=DIRECTION('center_axis',(1.,-3.46944695195361E-16,0.)) ;
#84109=DIRECTION('ref_axis',(3.46944695195361E-16,1.,0.)) ;
#84110=DIRECTION('',(1.5529910948782E-31,4.47619207437002E-16,-1.)) ;
#84111=DIRECTION('',(0.,0.,1.)) ;
#84112=DIRECTION('center_axis',(1.,-3.46944695195361E-16,0.)) ;
#84113=DIRECTION('ref_axis',(3.46944695195361E-16,1.,0.)) ;
#84114=DIRECTION('center_axis',(1.,-3.46944695195361E-16,0.)) ;
#84115=DIRECTION('ref_axis',(3.46944695195361E-16,1.,0.)) ;
#84116=DIRECTION('center_axis',(1.,-3.46944695195361E-16,0.)) ;
#84117=DIRECTION('ref_axis',(3.46944695195361E-16,1.,0.)) ;
#84118=DIRECTION('',(3.46944695195361E-16,1.,9.27571383489107E-17)) ;
#84119=DIRECTION('',(0.,0.,1.)) ;
#84120=DIRECTION('',(-3.46944695195361E-16,-1.,-6.49299968442375E-16)) ;
#84121=DIRECTION('center_axis',(1.,-3.46944695195361E-16,0.)) ;
#84122=DIRECTION('ref_axis',(3.46944695195361E-16,1.,0.)) ;
#84123=DIRECTION('center_axis',(1.,-3.46944695195361E-16,0.)) ;
#84124=DIRECTION('ref_axis',(3.46944695195361E-16,1.,0.)) ;
#84125=DIRECTION('center_axis',(1.,-3.46944695195361E-16,0.)) ;
#84126=DIRECTION('ref_axis',(3.46944695195361E-16,1.,0.)) ;
#84127=DIRECTION('',(0.,0.,1.)) ;
#84128=DIRECTION('',(-1.5529910948782E-31,-4.47619207437002E-16,-1.)) ;
#84129=DIRECTION('center_axis',(1.,-3.46944695195361E-16,0.)) ;
#84130=DIRECTION('ref_axis',(3.46944695195361E-16,1.,0.)) ;
#84131=DIRECTION('center_axis',(1.,-3.46944695195361E-16,0.)) ;
#84132=DIRECTION('ref_axis',(3.46944695195361E-16,1.,0.)) ;
#84133=DIRECTION('center_axis',(1.,-3.46944695195361E-16,0.)) ;
#84134=DIRECTION('ref_axis',(3.46944695195361E-16,1.,0.)) ;
#84135=DIRECTION('',(-3.46944695195361E-16,-1.,-1.06487173641454E-15)) ;
#84136=DIRECTION('center_axis',(1.,-3.46944695195361E-16,0.)) ;
#84137=DIRECTION('ref_axis',(3.46944695195361E-16,1.,0.)) ;
#84138=DIRECTION('',(3.46944695195361E-16,1.,2.45739631480277E-16)) ;
#84139=DIRECTION('center_axis',(1.,-3.46944695195361E-16,0.)) ;
#84140=DIRECTION('ref_axis',(3.46944695195361E-16,1.,0.)) ;
#84141=DIRECTION('center_axis',(1.,-3.46944695195361E-16,0.)) ;
#84142=DIRECTION('ref_axis',(3.46944695195361E-16,1.,0.)) ;
#84143=DIRECTION('center_axis',(0.,-1.,0.)) ;
#84144=DIRECTION('ref_axis',(0.,0.,-1.)) ;
#84145=DIRECTION('center_axis',(0.,-1.,0.)) ;
#84146=DIRECTION('ref_axis',(0.,0.,-1.)) ;
#84147=DIRECTION('',(-1.,0.,-1.40488587213121E-32)) ;
#84148=DIRECTION('',(0.,0.,1.)) ;
#84149=DIRECTION('',(0.,0.,1.)) ;
#84150=DIRECTION('',(0.,0.,1.)) ;
#84151=DIRECTION('',(1.,0.,1.40488587213121E-32)) ;
#84152=DIRECTION('center_axis',(0.,-1.,0.)) ;
#84153=DIRECTION('ref_axis',(0.,0.,-1.)) ;
#84154=DIRECTION('',(7.2280144832367E-17,0.,-1.)) ;
#84155=DIRECTION('center_axis',(-1.,-1.13380619344889E-16,0.)) ;
#84156=DIRECTION('ref_axis',(1.13380619344889E-16,-1.,0.)) ;
#84157=DIRECTION('center_axis',(-1.,-1.13380619344889E-16,0.)) ;
#84158=DIRECTION('ref_axis',(1.13380619344889E-16,-1.,0.)) ;
#84159=DIRECTION('',(1.13380619344889E-16,-1.,1.23908819712629E-16)) ;
#84160=DIRECTION('',(0.,0.,-1.)) ;
#84161=DIRECTION('',(-1.13380619344889E-16,1.,-1.23908819712629E-16)) ;
#84162=DIRECTION('center_axis',(-1.,-1.13380619344889E-16,0.)) ;
#84163=DIRECTION('ref_axis',(1.13380619344889E-16,-1.,0.)) ;
#84164=DIRECTION('',(0.,0.,1.)) ;
#84165=DIRECTION('center_axis',(-1.40488587213121E-32,1.23908819712629E-16,
1.)) ;
#84166=DIRECTION('ref_axis',(0.,-1.,1.23908819712629E-16)) ;
#84167=DIRECTION('',(-1.,0.,-1.40488587213121E-32)) ;
#84168=DIRECTION('',(-1.13380619344889E-16,1.,-1.23908819712629E-16)) ;
#84169=DIRECTION('center_axis',(1.40488587213121E-32,-1.23908819712629E-16,
-1.)) ;
#84170=DIRECTION('ref_axis',(-1.74077750246726E-48,-1.,1.23908819712629E-16)) ;
#84171=DIRECTION('center_axis',(1.40488587213121E-32,-1.23908819712629E-16,
-1.)) ;
#84172=DIRECTION('ref_axis',(0.,1.,-1.23908819712629E-16)) ;
#84173=DIRECTION('center_axis',(-1.40488587213121E-32,1.23908819712629E-16,
1.)) ;
#84174=DIRECTION('ref_axis',(1.74077750246726E-48,1.,-1.23908819712629E-16)) ;
#84175=DIRECTION('',(1.13380619344889E-16,-1.,1.23908819712629E-16)) ;
#84176=DIRECTION('',(1.,0.,1.40488587213121E-32)) ;
#84177=DIRECTION('center_axis',(-1.,-1.23908819712629E-16,-8.95614743483648E-33)) ;
#84178=DIRECTION('ref_axis',(1.23908819712629E-16,-1.,5.38566640001825E-66)) ;
#84179=DIRECTION('',(-8.95614743483648E-33,-1.10974565782288E-48,1.)) ;
#84180=DIRECTION('',(1.23908819712629E-16,-1.,7.2280144832367E-17)) ;
#84181=DIRECTION('',(-8.95614743483648E-33,0.,1.)) ;
#84182=DIRECTION('',(-1.23908819712629E-16,1.,-1.23908819712629E-16)) ;
#84183=DIRECTION('',(8.95614743483648E-33,1.0154535431059E-48,-1.)) ;
#84184=DIRECTION('',(1.23908819712629E-16,-1.,1.23908819712629E-16)) ;
#84185=DIRECTION('',(-8.95614743483648E-33,0.,1.)) ;
#84186=DIRECTION('',(-1.23908819712629E-16,1.,2.4093381610789E-16)) ;
#84187=DIRECTION('center_axis',(-1.7912294869673E-32,7.2280144832367E-17,
1.)) ;
#84188=DIRECTION('ref_axis',(0.,-1.,7.2280144832367E-17)) ;
#84189=DIRECTION('',(-1.23908819712629E-16,1.,-7.2280144832367E-17)) ;
#84190=DIRECTION('',(1.,1.23908819712629E-16,8.95614743483648E-33)) ;
#84191=DIRECTION('',(1.44560289664734E-16,-1.,7.2280144832367E-17)) ;
#84192=DIRECTION('',(-1.,0.,-1.7912294869673E-32)) ;
#84193=DIRECTION('center_axis',(-2.08976773479518E-32,2.4093381610789E-16,
-1.)) ;
#84194=DIRECTION('ref_axis',(0.,1.,2.4093381610789E-16)) ;
#84195=DIRECTION('',(-1.44560289664734E-16,1.,2.4093381610789E-16)) ;
#84196=DIRECTION('',(-1.,-1.23908819712629E-16,-8.95614743483648E-33)) ;
#84197=DIRECTION('',(1.23908819712629E-16,-1.,-2.4093381610789E-16)) ;
#84198=DIRECTION('',(1.,0.,-2.08976773479518E-32)) ;
#84199=DIRECTION('center_axis',(-1.23908819712629E-16,1.,0.)) ;
#84200=DIRECTION('ref_axis',(-1.,-1.23908819712629E-16,0.)) ;
#84201=DIRECTION('',(8.95614743483648E-33,1.10974565782288E-48,-1.)) ;
#84202=DIRECTION('',(1.,1.23908819712629E-16,8.95614743483648E-33)) ;
#84203=DIRECTION('',(-2.65552944032596E-32,-3.29043518662928E-48,1.)) ;
#84204=DIRECTION('',(-1.,-1.23908819712629E-16,-8.95614743483648E-33)) ;
#84205=DIRECTION('center_axis',(-1.,-1.44560289664734E-16,-2.65552944032596E-32)) ;
#84206=DIRECTION('ref_axis',(1.44560289664734E-16,-1.,-2.80018320648271E-64)) ;
#84207=DIRECTION('',(1.44560289664734E-16,-1.,-2.4093381610789E-16)) ;
#84208=DIRECTION('',(-2.65552944032596E-32,0.,1.)) ;
#84209=DIRECTION('',(-1.44560289664734E-16,1.,-7.2280144832367E-17)) ;
#84210=DIRECTION('',(0.,0.,-1.)) ;
#84211=DIRECTION('center_axis',(0.,1.,0.)) ;
#84212=DIRECTION('ref_axis',(0.,0.,1.)) ;
#84213=DIRECTION('',(8.95614743483648E-33,0.,-1.)) ;
#84214=DIRECTION('',(1.,0.,1.40488587213121E-32)) ;
#84215=DIRECTION('',(-7.2280144832367E-17,0.,1.)) ;
#84216=DIRECTION('',(-1.,0.,-1.40488587213121E-32)) ;
#84217=DIRECTION('',(8.95614743483648E-33,0.,-1.)) ;
#84218=DIRECTION('',(1.,0.,1.7912294869673E-32)) ;
#84219=DIRECTION('',(2.65552944032596E-32,0.,-1.)) ;
#84220=DIRECTION('',(-1.,0.,2.08976773479518E-32)) ;
#84221=DIRECTION('center_axis',(1.,1.44560289664734E-16,0.)) ;
#84222=DIRECTION('ref_axis',(-1.44560289664734E-16,1.,0.)) ;
#84223=DIRECTION('',(1.44560289664734E-16,-1.,0.)) ;
#84224=DIRECTION('center_axis',(-1.,-1.44560289664734E-16,0.)) ;
#84225=DIRECTION('ref_axis',(-1.44560289664734E-16,1.,-5.20417042793041E-14)) ;
#84226=DIRECTION('',(0.,0.,-1.)) ;
#84227=DIRECTION('center_axis',(-1.,-1.44560289664734E-16,0.)) ;
#84228=DIRECTION('ref_axis',(-1.44560289664734E-16,1.,0.)) ;
#84229=DIRECTION('',(1.44560289664734E-16,-1.,0.)) ;
#84230=DIRECTION('center_axis',(-1.,-1.44560289664734E-16,0.)) ;
#84231=DIRECTION('ref_axis',(-1.44560289664734E-16,1.,0.)) ;
#84232=DIRECTION('',(0.,0.,1.)) ;
#84233=DIRECTION('center_axis',(-1.,-1.44560289664734E-16,0.)) ;
#84234=DIRECTION('ref_axis',(-1.44560289664734E-16,1.,0.)) ;
#84235=DIRECTION('center_axis',(1.,-3.46944695195361E-16,0.)) ;
#84236=DIRECTION('ref_axis',(3.46944695195361E-16,1.,0.)) ;
#84237=DIRECTION('center_axis',(1.,-3.46944695195361E-16,0.)) ;
#84238=DIRECTION('ref_axis',(3.46944695195361E-16,1.,0.)) ;
#84239=DIRECTION('',(0.,0.,-1.)) ;
#84240=DIRECTION('',(-1.5529910948782E-31,-4.47619207437002E-16,1.)) ;
#84241=DIRECTION('center_axis',(-1.,3.46944695195361E-16,0.)) ;
#84242=DIRECTION('ref_axis',(3.46944695195361E-16,1.,-1.87537673078574E-15)) ;
#84243=DIRECTION('',(-3.46944695195361E-16,-1.,-2.45739631480277E-16)) ;
#84244=DIRECTION('center_axis',(1.,-3.46944695195361E-16,0.)) ;
#84245=DIRECTION('ref_axis',(3.46944695195361E-16,1.,0.)) ;
#84246=DIRECTION('center_axis',(3.46944695195361E-16,1.,4.47619207437002E-16)) ;
#84247=DIRECTION('ref_axis',(-8.18685017503995E-48,-4.47619207437002E-16,
1.)) ;
#84248=DIRECTION('',(-1.5529910948782E-31,-4.47619207437002E-16,1.)) ;
#84249=DIRECTION('',(-1.,3.46944695195361E-16,0.)) ;
#84250=DIRECTION('',(1.5529910948782E-31,4.47619207437002E-16,-1.)) ;
#84251=DIRECTION('center_axis',(-8.52580615413453E-32,-2.45739631480277E-16,
1.)) ;
#84252=DIRECTION('ref_axis',(0.,-1.,-2.45739631480277E-16)) ;
#84253=DIRECTION('',(1.,-3.46944695195361E-16,0.)) ;
#84254=DIRECTION('',(-3.46944695195361E-16,-1.,-2.45739631480277E-16)) ;
#84255=DIRECTION('',(3.46944695195361E-16,1.,2.45739631480277E-16)) ;
#84256=DIRECTION('center_axis',(1.,-3.46944695195361E-16,0.)) ;
#84257=DIRECTION('ref_axis',(3.46944695195361E-16,1.,0.)) ;
#84258=DIRECTION('center_axis',(1.,-3.46944695195361E-16,0.)) ;
#84259=DIRECTION('ref_axis',(3.46944695195361E-16,1.,0.)) ;
#84260=DIRECTION('',(1.,-3.46944695195361E-16,0.)) ;
#84261=DIRECTION('center_axis',(-1.,3.46944695195361E-16,0.)) ;
#84262=DIRECTION('ref_axis',(3.46944695195361E-16,1.,1.98254111540207E-15)) ;
#84263=DIRECTION('',(-1.,3.46944695195361E-16,0.)) ;
#84264=DIRECTION('center_axis',(1.,-3.46944695195361E-16,0.)) ;
#84265=DIRECTION('ref_axis',(3.46944695195361E-16,1.,0.)) ;
#84266=DIRECTION('center_axis',(1.,-3.46944695195361E-16,0.)) ;
#84267=DIRECTION('ref_axis',(-3.46944695195361E-16,-1.,-9.91270557701033E-16)) ;
#84268=DIRECTION('',(1.,-3.46944695195361E-16,0.)) ;
#84269=DIRECTION('center_axis',(-1.,3.46944695195361E-16,0.)) ;
#84270=DIRECTION('ref_axis',(3.46944695195361E-16,1.,4.95635278850516E-15)) ;
#84271=DIRECTION('',(-1.,3.46944695195361E-16,0.)) ;
#84272=DIRECTION('center_axis',(3.69451600012496E-31,1.06487173641454E-15,
-1.)) ;
#84273=DIRECTION('ref_axis',(0.,1.,1.06487173641454E-15)) ;
#84274=DIRECTION('',(3.46944695195361E-16,1.,1.06487173641454E-15)) ;
#84275=DIRECTION('',(-1.,3.46944695195361E-16,0.)) ;
#84276=DIRECTION('',(-3.46944695195361E-16,-1.,-1.06487173641454E-15)) ;
#84277=DIRECTION('center_axis',(3.46944695195361E-16,1.,-4.47619207437002E-16)) ;
#84278=DIRECTION('ref_axis',(8.18685017503995E-48,4.47619207437002E-16,
1.)) ;
#84279=DIRECTION('',(1.,-3.46944695195361E-16,0.)) ;
#84280=DIRECTION('',(1.5529910948782E-31,4.47619207437002E-16,1.)) ;
#84281=DIRECTION('',(-1.5529910948782E-31,-4.47619207437002E-16,-1.)) ;
#84282=DIRECTION('center_axis',(-1.,3.46944695195361E-16,0.)) ;
#84283=DIRECTION('ref_axis',(-3.46944695195361E-16,-1.,0.)) ;
#84284=DIRECTION('center_axis',(-1.,3.46944695195361E-16,0.)) ;
#84285=DIRECTION('ref_axis',(-3.46944695195361E-16,-1.,0.)) ;
#84286=DIRECTION('',(1.5529910948782E-31,4.47619207437002E-16,1.)) ;
#84287=DIRECTION('',(0.,0.,-1.)) ;
#84288=DIRECTION('center_axis',(1.,-3.46944695195361E-16,0.)) ;
#84289=DIRECTION('ref_axis',(-3.46944695195361E-16,-1.,0.)) ;
#84290=DIRECTION('center_axis',(1.,-3.46944695195361E-16,0.)) ;
#84291=DIRECTION('ref_axis',(-3.46944695195361E-16,-1.,0.)) ;
#84292=DIRECTION('',(3.46944695195361E-16,1.,1.06487173641454E-15)) ;
#84293=DIRECTION('center_axis',(1.,-3.46944695195361E-16,0.)) ;
#84294=DIRECTION('ref_axis',(3.46944695195361E-16,1.,0.)) ;
#84295=DIRECTION('center_axis',(-1.,3.46944695195361E-16,0.)) ;
#84296=DIRECTION('ref_axis',(3.46944695195361E-16,1.,0.)) ;
#84297=DIRECTION('',(0.,0.,-1.)) ;
#84298=DIRECTION('',(0.,0.,1.)) ;
#84299=DIRECTION('',(-3.46944695195361E-16,-1.,-9.27571383489107E-17)) ;
#84300=DIRECTION('center_axis',(-3.46944695195361E-16,-1.,0.)) ;
#84301=DIRECTION('ref_axis',(1.,-3.46944695195361E-16,0.)) ;
#84302=DIRECTION('',(1.,-3.46944695195361E-16,0.)) ;
#84303=DIRECTION('',(0.,0.,-1.)) ;
#84304=DIRECTION('',(0.,0.,1.)) ;
#84305=DIRECTION('center_axis',(1.,-3.46944695195361E-16,0.)) ;
#84306=DIRECTION('ref_axis',(3.46944695195361E-16,1.,0.)) ;
#84307=DIRECTION('center_axis',(1.,-3.46944695195361E-16,0.)) ;
#84308=DIRECTION('ref_axis',(3.46944695195361E-16,1.,0.)) ;
#84309=DIRECTION('',(1.,-3.46944695195361E-16,0.)) ;
#84310=DIRECTION('center_axis',(-1.,3.46944695195361E-16,0.)) ;
#84311=DIRECTION('ref_axis',(3.46944695195361E-16,1.,0.)) ;
#84312=DIRECTION('',(-1.,3.46944695195361E-16,0.)) ;
#84313=DIRECTION('center_axis',(-3.21815970916568E-32,-9.27571383489107E-17,
1.)) ;
#84314=DIRECTION('ref_axis',(0.,-1.,-9.27571383489107E-17)) ;
#84315=DIRECTION('',(3.46944695195361E-16,1.,9.27571383489107E-17)) ;
#84316=DIRECTION('',(1.,0.,3.21815970916568E-32)) ;
#84317=DIRECTION('',(-3.46944695195361E-16,-1.,-9.27571383489107E-17)) ;
#84318=DIRECTION('',(-1.,3.46944695195361E-16,0.)) ;
#84319=DIRECTION('center_axis',(1.,-3.46944695195361E-16,0.)) ;
#84320=DIRECTION('ref_axis',(3.46944695195361E-16,1.,0.)) ;
#84321=DIRECTION('center_axis',(1.,-3.46944695195361E-16,0.)) ;
#84322=DIRECTION('ref_axis',(-3.46944695195361E-16,-1.,-2.9738116731031E-15)) ;
#84323=DIRECTION('',(1.,-3.46944695195361E-16,0.)) ;
#84324=DIRECTION('center_axis',(-1.,3.46944695195361E-16,0.)) ;
#84325=DIRECTION('ref_axis',(3.46944695195361E-16,1.,-1.98254111540207E-15)) ;
#84326=DIRECTION('',(-1.,3.46944695195361E-16,0.)) ;
#84327=DIRECTION('center_axis',(-3.46944695195361E-16,-1.,0.)) ;
#84328=DIRECTION('ref_axis',(1.,-3.46944695195361E-16,0.)) ;
#84329=DIRECTION('',(0.,0.,-1.)) ;
#84330=DIRECTION('',(-1.,3.46944695195361E-16,0.)) ;
#84331=DIRECTION('',(0.,0.,1.)) ;
#84332=DIRECTION('center_axis',(2.25271179641597E-31,6.49299968442375E-16,
-1.)) ;
#84333=DIRECTION('ref_axis',(0.,1.,6.49299968442375E-16)) ;
#84334=DIRECTION('',(3.46944695195361E-16,1.,6.49299968442375E-16)) ;
#84335=DIRECTION('',(-1.,0.,-2.25271179641597E-31)) ;
#84336=DIRECTION('',(-3.46944695195361E-16,-1.,-6.49299968442375E-16)) ;
#84337=DIRECTION('',(1.,-3.46944695195361E-16,0.)) ;
#84338=DIRECTION('center_axis',(-1.,3.46944695195361E-16,0.)) ;
#84339=DIRECTION('ref_axis',(-3.46944695195361E-16,-1.,0.)) ;
#84340=DIRECTION('',(3.46944695195361E-16,1.,6.49299968442375E-16)) ;
#84341=DIRECTION('',(0.,0.,1.)) ;
#84342=DIRECTION('',(0.,0.,-1.)) ;
#84343=DIRECTION('center_axis',(-1.,3.46944695195361E-16,0.)) ;
#84344=DIRECTION('ref_axis',(-3.46944695195361E-16,-1.,0.)) ;
#84345=DIRECTION('center_axis',(-0.164398987305357,0.,-0.986393923832144)) ;
#84346=DIRECTION('ref_axis',(-0.986393923832144,0.,0.164398987305357)) ;
#84347=DIRECTION('',(-0.937042571331636,0.312347523777212,0.156173761888606)) ;
#84348=DIRECTION('',(0.,-1.,0.)) ;
#84349=DIRECTION('',(0.973328526784575,0.162221421130762,-0.162221421130763)) ;
#84350=DIRECTION('',(-1.73472347597681E-15,1.,2.89120579329468E-16)) ;
#84351=DIRECTION('center_axis',(-1.,0.,0.)) ;
#84352=DIRECTION('ref_axis',(0.,0.,1.)) ;
#84353=DIRECTION('center_axis',(-1.,0.,0.)) ;
#84354=DIRECTION('ref_axis',(0.,0.958782009816033,-0.284142671299347)) ;
#84355=DIRECTION('',(0.,0.,1.)) ;
#84356=DIRECTION('',(0.,-1.,0.)) ;
#84357=DIRECTION('center_axis',(-1.,0.,0.)) ;
#84358=DIRECTION('ref_axis',(0.,0.758706765780369,-0.65143230159326)) ;
#84359=DIRECTION('',(0.,0.,-1.)) ;
#84360=DIRECTION('center_axis',(-1.,0.,0.)) ;
#84361=DIRECTION('ref_axis',(0.,-0.654778303469126,-0.755820992898512)) ;
#84362=DIRECTION('',(0.,1.,0.)) ;
#84363=DIRECTION('center_axis',(-0.164398987305357,0.,0.986393923832144)) ;
#84364=DIRECTION('ref_axis',(0.986393923832144,0.,0.164398987305357)) ;
#84365=DIRECTION('',(-0.973328526784575,-0.162221421130762,-0.162221421130763)) ;
#84366=DIRECTION('',(0.,1.,0.)) ;
#84367=DIRECTION('',(0.937042571331636,-0.312347523777212,0.156173761888606)) ;
#84368=DIRECTION('',(1.73472347597681E-15,-1.,2.89120579329468E-16)) ;
#84369=DIRECTION('center_axis',(-0.573462344363329,0.81923192051904,0.)) ;
#84370=DIRECTION('ref_axis',(-0.81923192051904,-0.573462344363329,0.)) ;
#84371=DIRECTION('',(-0.710669054518702,-0.497468338163091,0.49746833816309)) ;
#84372=DIRECTION('',(0.,0.,-1.)) ;
#84373=DIRECTION('',(0.710669054518702,0.497468338163091,0.49746833816309)) ;
#84374=DIRECTION('',(0.,0.,1.)) ;
#84375=DIRECTION('center_axis',(-1.,0.,0.)) ;
#84376=DIRECTION('ref_axis',(0.,0.,1.)) ;
#84377=DIRECTION('',(0.,0.,1.)) ;
#84378=DIRECTION('',(0.,-1.,-9.34081871679819E-17)) ;
#84379=DIRECTION('',(0.,0.,-1.)) ;
#84380=DIRECTION('',(0.,1.,-9.34081871679819E-17)) ;
#84381=DIRECTION('center_axis',(-0.573462344363329,-0.81923192051904,0.)) ;
#84382=DIRECTION('ref_axis',(0.81923192051904,-0.573462344363329,0.)) ;
#84383=DIRECTION('',(-0.710669054518701,0.497468338163091,-0.497468338163091)) ;
#84384=DIRECTION('',(0.,0.,1.)) ;
#84385=DIRECTION('',(0.710669054518701,-0.497468338163091,-0.497468338163091)) ;
#84386=DIRECTION('',(0.,0.,-1.)) ;
#84387=DIRECTION('center_axis',(0.,0.,1.)) ;
#84388=DIRECTION('ref_axis',(1.,0.,0.)) ;
#84389=DIRECTION('',(1.,6.67201336914158E-17,0.)) ;
#84390=DIRECTION('',(1.33440267382831E-16,1.,0.)) ;
#84391=DIRECTION('',(-1.,1.33440267382831E-16,0.)) ;
#84392=DIRECTION('center_axis',(0.,0.,1.)) ;
#84393=DIRECTION('ref_axis',(1.,0.,0.)) ;
#84394=DIRECTION('',(1.,-1.33440267382831E-16,0.)) ;
#84395=DIRECTION('',(-1.33440267382831E-16,-1.,0.)) ;
#84396=DIRECTION('',(-1.,-6.67201336914158E-17,0.)) ;
#84397=DIRECTION('center_axis',(-6.67201336914158E-17,1.,0.)) ;
#84398=DIRECTION('ref_axis',(-1.,-6.67201336914158E-17,0.)) ;
#84399=DIRECTION('',(1.,6.67201336914158E-17,0.)) ;
#84400=DIRECTION('',(0.,0.,1.)) ;
#84401=DIRECTION('',(-1.,-6.67201336914158E-17,0.)) ;
#84402=DIRECTION('center_axis',(-1.33440267382831E-16,-1.,0.)) ;
#84403=DIRECTION('ref_axis',(1.,-1.33440267382831E-16,0.)) ;
#84404=DIRECTION('',(1.,-1.33440267382831E-16,0.)) ;
#84405=DIRECTION('',(0.,0.,-1.)) ;
#84406=DIRECTION('',(-1.,1.33440267382831E-16,0.)) ;
#84407=DIRECTION('center_axis',(0.,0.,1.)) ;
#84408=DIRECTION('ref_axis',(1.,0.,0.)) ;
#84409=DIRECTION('',(0.,-1.,0.)) ;
#84410=DIRECTION('',(1.,0.,0.)) ;
#84411=DIRECTION('',(0.,1.,0.)) ;
#84412=DIRECTION('center_axis',(0.,0.,-1.)) ;
#84413=DIRECTION('ref_axis',(1.,0.,0.)) ;
#84414=DIRECTION('',(-1.44560289664734E-16,1.,-7.2280144832367E-17)) ;
#84415=DIRECTION('center_axis',(0.,0.,1.)) ;
#84416=DIRECTION('ref_axis',(1.,0.,0.)) ;
#84417=DIRECTION('center_axis',(0.,0.,1.)) ;
#84418=DIRECTION('ref_axis',(1.,0.,0.)) ;
#84419=DIRECTION('',(0.,-1.,0.)) ;
#84420=DIRECTION('',(-1.,0.,0.)) ;
#84421=DIRECTION('',(0.,1.,0.)) ;
#84422=DIRECTION('center_axis',(0.,0.,-1.)) ;
#84423=DIRECTION('ref_axis',(1.,-1.82602471155453E-15,0.)) ;
#84424=DIRECTION('',(1.44560289664734E-16,-1.,-2.4093381610789E-16)) ;
#84425=DIRECTION('center_axis',(0.,0.,1.)) ;
#84426=DIRECTION('ref_axis',(1.,0.,0.)) ;
#84427=DIRECTION('center_axis',(0.,0.,-1.)) ;
#84428=DIRECTION('ref_axis',(-1.,0.,0.)) ;
#84429=DIRECTION('',(0.,0.,-1.)) ;
#84430=DIRECTION('center_axis',(0.,0.,-1.)) ;
#84431=DIRECTION('ref_axis',(1.,0.,0.)) ;
#84432=DIRECTION('center_axis',(0.,0.,1.)) ;
#84433=DIRECTION('ref_axis',(1.,0.,0.)) ;
#84434=DIRECTION('center_axis',(1.,0.,0.)) ;
#84435=DIRECTION('ref_axis',(0.,0.,-1.)) ;
#84436=DIRECTION('',(0.,-1.,0.)) ;
#84437=DIRECTION('',(0.,0.,1.)) ;
#84438=DIRECTION('',(0.,1.,0.)) ;
#84439=DIRECTION('center_axis',(0.81923192051904,0.573462344363329,0.)) ;
#84440=DIRECTION('ref_axis',(-0.573462344363329,0.81923192051904,0.)) ;
#84441=DIRECTION('',(-0.497468338163091,0.710669054518701,0.497468338163091)) ;
#84442=DIRECTION('',(0.,0.,-1.)) ;
#84443=DIRECTION('',(0.497468338163091,-0.710669054518701,0.497468338163091)) ;
#84444=DIRECTION('',(0.,0.,1.)) ;
#84445=DIRECTION('center_axis',(0.,1.,0.)) ;
#84446=DIRECTION('ref_axis',(0.,0.,1.)) ;
#84447=DIRECTION('',(0.,0.,1.)) ;
#84448=DIRECTION('',(-1.,0.,0.)) ;
#84449=DIRECTION('',(0.,0.,-1.)) ;
#84450=DIRECTION('',(1.,0.,0.)) ;
#84451=DIRECTION('center_axis',(-0.81923192051904,0.573462344363329,0.)) ;
#84452=DIRECTION('ref_axis',(-0.573462344363329,-0.81923192051904,0.)) ;
#84453=DIRECTION('',(0.497468338163091,0.710669054518701,-0.497468338163091)) ;
#84454=DIRECTION('',(0.,0.,1.)) ;
#84455=DIRECTION('',(-0.497468338163091,-0.710669054518701,-0.497468338163091)) ;
#84456=DIRECTION('',(0.,0.,-1.)) ;
#84457=DIRECTION('center_axis',(-1.,0.,0.)) ;
#84458=DIRECTION('ref_axis',(0.,0.,1.)) ;
#84459=DIRECTION('',(0.,-1.,0.)) ;
#84460=DIRECTION('',(0.,0.,-1.)) ;
#84461=DIRECTION('',(0.,1.,0.)) ;
#84462=DIRECTION('',(0.,0.,-1.)) ;
#84463=DIRECTION('center_axis',(0.,0.,-1.)) ;
#84464=DIRECTION('ref_axis',(-1.,0.,0.)) ;
#84465=DIRECTION('center_axis',(0.,0.,1.)) ;
#84466=DIRECTION('ref_axis',(1.,0.,0.)) ;
#84467=DIRECTION('center_axis',(0.,0.,-1.)) ;
#84468=DIRECTION('ref_axis',(1.,5.20417042793042E-15,0.)) ;
#84469=DIRECTION('center_axis',(-0.573462344363328,7.65229685658278E-17,
0.819231920519041)) ;
#84470=DIRECTION('ref_axis',(0.819231920519041,1.22423955297878E-32,0.573462344363328)) ;
#84471=DIRECTION('',(-0.710669054518702,-0.497468338163091,-0.497468338163091)) ;
#84472=DIRECTION('',(1.33440267382831E-16,1.,-2.91413396387194E-34)) ;
#84473=DIRECTION('',(0.710669054518701,-0.497468338163091,0.497468338163091)) ;
#84474=DIRECTION('',(5.04890651880155E-33,-1.,9.34081871679819E-17)) ;
#84475=DIRECTION('center_axis',(-0.573462344363328,7.65229685658278E-17,
-0.819231920519041)) ;
#84476=DIRECTION('ref_axis',(-0.819231920519041,-1.22423955297878E-32,0.573462344363328)) ;
#84477=DIRECTION('',(-0.710669054518701,0.497468338163091,0.497468338163091)) ;
#84478=DIRECTION('',(-1.33440267382831E-16,-1.,7.77328292223541E-33)) ;
#84479=DIRECTION('',(0.710669054518702,0.497468338163091,-0.497468338163091)) ;
#84480=DIRECTION('',(-5.04890651880155E-33,1.,9.34081871679819E-17)) ;
#84481=DIRECTION('center_axis',(0.,0.573462344363328,-0.819231920519041)) ;
#84482=DIRECTION('ref_axis',(0.,0.819231920519041,0.573462344363328)) ;
#84483=DIRECTION('',(0.497468338163091,0.710669054518701,0.497468338163091)) ;
#84484=DIRECTION('',(-1.,0.,0.)) ;
#84485=DIRECTION('',(0.497468338163091,-0.710669054518701,-0.497468338163091)) ;
#84486=DIRECTION('',(1.,0.,0.)) ;
#84487=DIRECTION('center_axis',(0.,0.573462344363328,0.819231920519041)) ;
#84488=DIRECTION('ref_axis',(0.,-0.819231920519041,0.573462344363328)) ;
#84489=DIRECTION('',(-0.497468338163091,0.710669054518701,-0.497468338163091)) ;
#84490=DIRECTION('',(1.,0.,0.)) ;
#84491=DIRECTION('',(-0.497468338163091,-0.710669054518701,0.497468338163091)) ;
#84492=DIRECTION('',(-1.,0.,0.)) ;
#84493=DIRECTION('center_axis',(-0.164398987305354,-0.986393923832144,0.)) ;
#84494=DIRECTION('ref_axis',(0.,0.,1.)) ;
#84495=DIRECTION('',(0.,0.,-1.)) ;
#84496=DIRECTION('center_axis',(-0.164398987305294,-0.986393923832154,-1.08493920789696E-12)) ;
#84497=DIRECTION('ref_axis',(-0.057729035738443,0.00962150595530534,0.998285923498805)) ;
#84498=DIRECTION('',(0.,0.,1.)) ;
#84499=DIRECTION('center_axis',(1.,-2.89120579329441E-16,0.)) ;
#84500=DIRECTION('ref_axis',(-2.89120579329441E-16,-1.,1.53777331288036E-13)) ;
#84501=DIRECTION('center_axis',(1.,1.15648231731787E-15,0.)) ;
#84502=DIRECTION('ref_axis',(1.15648231731787E-15,-1.,0.)) ;
#84503=DIRECTION('center_axis',(0.16668982355543,0.983956802853987,0.0635886219415135)) ;
#84504=DIRECTION('ref_axis',(-0.0486480010755861,0.0726194153599019,-0.996172571648174)) ;
#84505=DIRECTION('center_axis',(0.166689823544595,0.983956802870528,-0.0635886217139631)) ;
#84506=DIRECTION('ref_axis',(-0.0462047035076799,0.072214918770576,0.996318287938511)) ;
#84507=DIRECTION('center_axis',(-0.164398987305354,-0.986393923832144,0.)) ;
#84508=DIRECTION('ref_axis',(0.,0.,1.)) ;
#84509=DIRECTION('',(0.,0.,1.)) ;
#84510=DIRECTION('center_axis',(-0.164398987305453,-0.986393923832128,-1.73590273467075E-12)) ;
#84511=DIRECTION('ref_axis',(-0.0554192327903204,0.00923653880014933,-0.998420450004869)) ;
#84512=DIRECTION('',(0.,0.,-1.)) ;
#84513=DIRECTION('center_axis',(0.,0.,1.)) ;
#84514=DIRECTION('ref_axis',(1.,0.,0.)) ;
#84515=DIRECTION('center_axis',(0.,0.,1.)) ;
#84516=DIRECTION('ref_axis',(1.,0.,0.)) ;
#84517=DIRECTION('center_axis',(0.,1.,0.)) ;
#84518=DIRECTION('ref_axis',(1.,0.,0.)) ;
#84519=DIRECTION('center_axis',(0.,-0.888198741900269,0.45945945945946)) ;
#84520=DIRECTION('ref_axis',(0.,0.45945945945946,0.888198741900269)) ;
#84521=DIRECTION('center_axis',(-1.,0.,1.22067519501986E-15)) ;
#84522=DIRECTION('ref_axis',(-1.22067519501986E-15,0.,-1.)) ;
#84523=DIRECTION('center_axis',(0.,0.,1.)) ;
#84524=DIRECTION('ref_axis',(1.,0.,0.)) ;
#84525=DIRECTION('center_axis',(0.,0.,-1.)) ;
#84526=DIRECTION('ref_axis',(-1.,0.,0.)) ;
#84527=DIRECTION('center_axis',(1.,-3.46944695195361E-16,0.)) ;
#84528=DIRECTION('ref_axis',(3.46944695195361E-16,1.,0.)) ;
#84529=DIRECTION('center_axis',(-1.,3.46944695195361E-16,0.)) ;
#84530=DIRECTION('ref_axis',(3.46944695195361E-16,1.,0.)) ;
#84531=DIRECTION('center_axis',(-1.,3.46944695195361E-16,0.)) ;
#84532=DIRECTION('ref_axis',(-3.41607084500048E-16,-1.,0.)) ;
#84533=DIRECTION('center_axis',(0.,-0.459459459459457,0.888198741900271)) ;
#84534=DIRECTION('ref_axis',(0.,-0.888198741900271,-0.459459459459457)) ;
#84535=DIRECTION('center_axis',(1.,-3.46944695195361E-16,0.)) ;
#84536=DIRECTION('ref_axis',(0.,1.,0.)) ;
#84537=DIRECTION('center_axis',(0.,0.888198741900269,-0.45945945945946)) ;
#84538=DIRECTION('ref_axis',(0.,-0.45945945945946,-0.888198741900269)) ;
#84539=DIRECTION('center_axis',(0.,1.,0.)) ;
#84540=DIRECTION('ref_axis',(1.,0.,0.)) ;
#84541=DIRECTION('center_axis',(0.,-1.,0.)) ;
#84542=DIRECTION('ref_axis',(0.,0.,1.)) ;
#84543=DIRECTION('center_axis',(-1.,0.,0.)) ;
#84544=DIRECTION('ref_axis',(0.,0.,-1.)) ;
#84545=DIRECTION('center_axis',(0.,0.,-1.)) ;
#84546=DIRECTION('ref_axis',(-1.,0.,0.)) ;
#84547=DIRECTION('center_axis',(0.,0.,-1.)) ;
#84548=DIRECTION('ref_axis',(-1.,0.,0.)) ;
#84549=DIRECTION('center_axis',(1.,-3.46944695195361E-16,0.)) ;
#84550=DIRECTION('ref_axis',(3.46944695195361E-16,1.,0.)) ;
#84551=DIRECTION('center_axis',(-1.,3.46944695195361E-16,0.)) ;
#84552=DIRECTION('ref_axis',(3.46944695195361E-16,1.,3.46944695195361E-14)) ;
#84553=DIRECTION('center_axis',(1.,0.,0.)) ;
#84554=DIRECTION('ref_axis',(0.,0.,-1.)) ;
#84555=DIRECTION('center_axis',(0.,0.,1.)) ;
#84556=DIRECTION('ref_axis',(1.,0.,0.)) ;
#84557=DIRECTION('center_axis',(0.,0.,1.)) ;
#84558=DIRECTION('ref_axis',(1.,0.,0.)) ;
#84559=DIRECTION('center_axis',(1.,-3.46944695195361E-16,0.)) ;
#84560=DIRECTION('ref_axis',(3.80647894157197E-16,1.,0.)) ;
#84561=DIRECTION('center_axis',(0.,0.459459459459459,-0.888198741900269)) ;
#84562=DIRECTION('ref_axis',(0.,0.888198741900269,0.459459459459459)) ;
#84563=DIRECTION('center_axis',(1.,-3.46944695195361E-16,0.)) ;
#84564=DIRECTION('ref_axis',(3.46944695195361E-16,1.,0.)) ;
#84565=DIRECTION('center_axis',(-1.,3.46944695195361E-16,0.)) ;
#84566=DIRECTION('ref_axis',(3.46944695195361E-16,1.,0.)) ;
#84567=DIRECTION('center_axis',(-3.46944695195361E-16,-1.,-6.49299968442375E-16)) ;
#84568=DIRECTION('ref_axis',(2.25271179641597E-31,6.49299968442375E-16,
-1.)) ;
#84569=DIRECTION('center_axis',(0.,-1.,0.)) ;
#84570=DIRECTION('ref_axis',(0.,0.,-1.)) ;
#84571=DIRECTION('center_axis',(0.,0.,1.)) ;
#84572=DIRECTION('ref_axis',(1.,0.,0.)) ;
#84573=DIRECTION('center_axis',(-3.25260651745651E-15,0.,1.)) ;
#84574=DIRECTION('ref_axis',(1.,0.,3.25260651745651E-15)) ;
#84575=DIRECTION('center_axis',(0.,1.,0.)) ;
#84576=DIRECTION('ref_axis',(1.,0.,0.)) ;
#84577=DIRECTION('center_axis',(0.,-0.888198741900269,-0.45945945945946)) ;
#84578=DIRECTION('ref_axis',(0.,-0.45945945945946,0.888198741900269)) ;
#84579=DIRECTION('center_axis',(1.,-3.46944695195361E-16,0.)) ;
#84580=DIRECTION('ref_axis',(0.,1.,0.)) ;
#84581=DIRECTION('center_axis',(0.,0.888198741900269,0.45945945945946)) ;
#84582=DIRECTION('ref_axis',(0.,0.45945945945946,-0.888198741900269)) ;
#84583=DIRECTION('center_axis',(1.,-3.46944695195361E-16,0.)) ;
#84584=DIRECTION('ref_axis',(0.,1.,0.)) ;
#84585=DIRECTION('center_axis',(0.,1.,0.)) ;
#84586=DIRECTION('ref_axis',(0.,0.,-1.)) ;
#84587=DIRECTION('center_axis',(0.,1.,0.)) ;
#84588=DIRECTION('ref_axis',(1.,0.,0.)) ;
#84589=DIRECTION('center_axis',(-1.,0.,0.)) ;
#84590=DIRECTION('ref_axis',(0.,0.,-1.)) ;
#84591=DIRECTION('center_axis',(1.,-3.46944695195361E-16,0.)) ;
#84592=DIRECTION('ref_axis',(3.41607084500048E-16,1.,0.)) ;
#84593=DIRECTION('center_axis',(-9.62987005567165E-16,-0.459459459459459,
-0.88819874190027)) ;
#84594=DIRECTION('ref_axis',(-7.31984232283282E-30,0.88819874190027,-0.459459459459459)) ;
#84595=DIRECTION('center_axis',(1.,-3.46944695195361E-16,0.)) ;
#84596=DIRECTION('ref_axis',(3.46944695195361E-16,1.,0.)) ;
#84597=DIRECTION('center_axis',(-1.,3.46944695195361E-16,0.)) ;
#84598=DIRECTION('ref_axis',(3.46944695195361E-16,1.,0.)) ;
#84599=DIRECTION('center_axis',(1.,0.,0.)) ;
#84600=DIRECTION('ref_axis',(0.,0.,-1.)) ;
#84601=DIRECTION('center_axis',(1.,-3.46944695195361E-16,0.)) ;
#84602=DIRECTION('ref_axis',(3.80647894157197E-16,1.,0.)) ;
#84603=DIRECTION('center_axis',(0.,0.459459459459459,0.888198741900269)) ;
#84604=DIRECTION('ref_axis',(0.,-0.888198741900269,0.459459459459459)) ;
#84605=DIRECTION('center_axis',(-3.46944695195361E-16,-1.,-6.49299968442375E-16)) ;
#84606=DIRECTION('ref_axis',(2.25271179641597E-31,6.49299968442375E-16,
-1.)) ;
#84607=DIRECTION('center_axis',(0.,1.,0.)) ;
#84608=DIRECTION('ref_axis',(0.,0.,-1.)) ;
#84609=DIRECTION('center_axis',(1.,0.,2.25271179641597E-31)) ;
#84610=DIRECTION('ref_axis',(2.25271179641597E-31,0.,-1.)) ;
#84611=DIRECTION('center_axis',(-1.,0.,0.)) ;
#84612=DIRECTION('ref_axis',(0.,0.,1.)) ;
#84613=DIRECTION('center_axis',(0.,1.,0.)) ;
#84614=DIRECTION('ref_axis',(1.,0.,0.)) ;
#84615=DIRECTION('center_axis',(0.,-1.,0.)) ;
#84616=DIRECTION('ref_axis',(-1.08420217248551E-15,0.,1.)) ;
#84617=DIRECTION('center_axis',(1.,-3.46944695195361E-16,0.)) ;
#84618=DIRECTION('ref_axis',(0.,1.,0.)) ;
#84619=DIRECTION('center_axis',(0.,1.,0.)) ;
#84620=DIRECTION('ref_axis',(0.,0.,-1.)) ;
#84621=DIRECTION('center_axis',(0.,-1.,0.)) ;
#84622=DIRECTION('ref_axis',(0.,0.,-1.)) ;
#84623=DIRECTION('center_axis',(0.,0.,1.)) ;
#84624=DIRECTION('ref_axis',(-1.,0.,0.)) ;
#84625=DIRECTION('center_axis',(0.,0.,-1.)) ;
#84626=DIRECTION('ref_axis',(-1.,0.,0.)) ;
#84627=DIRECTION('center_axis',(0.,0.,-1.)) ;
#84628=DIRECTION('ref_axis',(-1.,0.,0.)) ;
#84629=DIRECTION('center_axis',(-3.46944695195361E-16,-1.,-9.27571383489107E-17)) ;
#84630=DIRECTION('ref_axis',(1.,-3.46944695195361E-16,-3.21815970916568E-32)) ;
#84631=DIRECTION('center_axis',(0.,-1.,0.)) ;
#84632=DIRECTION('ref_axis',(0.,0.,-1.)) ;
#84633=DIRECTION('center_axis',(3.46944695195361E-16,1.,9.27571383489107E-17)) ;
#84634=DIRECTION('ref_axis',(-1.,3.46944695195361E-16,3.21815970916568E-32)) ;
#84635=DIRECTION('center_axis',(0.,1.,0.)) ;
#84636=DIRECTION('ref_axis',(0.,0.,-1.)) ;
#84637=DIRECTION('center_axis',(0.,0.,-1.)) ;
#84638=DIRECTION('ref_axis',(-1.,0.,0.)) ;
#84639=DIRECTION('center_axis',(0.,0.,1.)) ;
#84640=DIRECTION('ref_axis',(1.,0.,0.)) ;
#84641=DIRECTION('center_axis',(0.,1.,0.)) ;
#84642=DIRECTION('ref_axis',(1.,0.,0.)) ;
#84643=DIRECTION('center_axis',(-1.,0.,1.0842021724855E-15)) ;
#84644=DIRECTION('ref_axis',(-1.0842021724855E-15,0.,-1.)) ;
#84645=DIRECTION('center_axis',(0.,-1.,0.)) ;
#84646=DIRECTION('ref_axis',(0.,0.,-1.)) ;
#84647=DIRECTION('center_axis',(1.,0.,0.)) ;
#84648=DIRECTION('ref_axis',(0.,0.,1.)) ;
#84649=DIRECTION('center_axis',(1.,0.,3.21815970916568E-32)) ;
#84650=DIRECTION('ref_axis',(3.21815970916568E-32,0.,-1.)) ;
#84651=DIRECTION('center_axis',(0.,1.,0.)) ;
#84652=DIRECTION('ref_axis',(1.,0.,0.)) ;
#84653=DIRECTION('center_axis',(0.,0.,-1.)) ;
#84654=DIRECTION('ref_axis',(1.,0.,0.)) ;
#84655=DIRECTION('center_axis',(1.,0.,0.)) ;
#84656=DIRECTION('ref_axis',(0.,-1.08420217248551E-15,1.)) ;
#84657=DIRECTION('center_axis',(1.0842021724855E-15,1.,0.)) ;
#84658=DIRECTION('ref_axis',(1.,-1.0842021724855E-15,0.)) ;
#84659=DIRECTION('center_axis',(1.,0.,-2.08976773479518E-32)) ;
#84660=DIRECTION('ref_axis',(-2.08976773479518E-32,0.,-1.)) ;
#84661=DIRECTION('center_axis',(-0.447220452189337,-7.10036081300347E-6,
-0.894423762594191)) ;
#84662=DIRECTION('ref_axis',(0.894325663270266,0.0148067719203444,-0.44717151913052)) ;
#84663=DIRECTION('center_axis',(-1.23908819712629E-16,1.,2.4093381610789E-16)) ;
#84664=DIRECTION('ref_axis',(2.98538247827883E-32,-2.4093381610789E-16,
1.)) ;
#84665=DIRECTION('center_axis',(-5.60223399549347E-6,-0.447219005480232,
-0.894424485971782)) ;
#84666=DIRECTION('ref_axis',(0.0146917039115986,0.894327914920361,-0.447170811245964)) ;
#84667=DIRECTION('center_axis',(-8.95614743483648E-33,0.,1.)) ;
#84668=DIRECTION('ref_axis',(1.,0.,8.95614743483648E-33)) ;
#84669=DIRECTION('center_axis',(1.40488587213121E-32,-1.23908819712629E-16,
-1.)) ;
#84670=DIRECTION('ref_axis',(1.74077750246726E-48,1.,-1.23908819712629E-16)) ;
#84671=DIRECTION('center_axis',(-2.65552944032596E-32,0.,1.)) ;
#84672=DIRECTION('ref_axis',(1.,0.,2.65552944032596E-32)) ;
#84673=DIRECTION('center_axis',(0.89442448597137,-5.60223466363593E-6,0.447219005481056)) ;
#84674=DIRECTION('ref_axis',(0.447170811246728,0.0146917039220712,-0.894327914919807)) ;
#84675=DIRECTION('center_axis',(0.894423762593715,-7.10036087598425E-6,
-0.447220452190288)) ;
#84676=DIRECTION('ref_axis',(0.447171519131212,0.014806771959662,0.894325663269269)) ;
#84677=DIRECTION('center_axis',(-8.95614743483648E-33,-1.10974565782288E-48,
1.)) ;
#84678=DIRECTION('ref_axis',(1.,-9.9390457266313E-81,8.95614743483648E-33)) ;
#84679=DIRECTION('center_axis',(-7.10036049907078E-6,0.894423762593765,
0.44722045219019)) ;
#84680=DIRECTION('ref_axis',(-0.0148067719083974,-0.447171519131448,0.89432566327)) ;
#84681=DIRECTION('center_axis',(-5.60223341193312E-6,0.894424485971936,
-0.447219005479926)) ;
#84682=DIRECTION('ref_axis',(0.0146917039491787,0.447170811245404,0.894327914920024)) ;
#84683=DIRECTION('center_axis',(1.40488587213121E-32,-1.23908819712629E-16,
-1.)) ;
#84684=DIRECTION('ref_axis',(0.,1.,0.)) ;
#84685=DIRECTION('center_axis',(-1.,0.,0.)) ;
#84686=DIRECTION('ref_axis',(0.,0.,-1.)) ;
#84687=DIRECTION('center_axis',(0.,-1.,0.)) ;
#84688=DIRECTION('ref_axis',(0.,0.,1.)) ;
#84689=DIRECTION('center_axis',(-1.,0.,-1.40488587213121E-32)) ;
#84690=DIRECTION('ref_axis',(-1.40488587213121E-32,0.,1.)) ;
#84691=DIRECTION('',(-1.,0.,-1.40488587213121E-32)) ;
#84692=DIRECTION('center_axis',(-1.,0.,0.)) ;
#84693=DIRECTION('ref_axis',(0.,0.,1.)) ;
#84694=DIRECTION('center_axis',(0.,1.,0.)) ;
#84695=DIRECTION('ref_axis',(1.,0.,0.)) ;
#84696=DIRECTION('center_axis',(0.,1.,0.)) ;
#84697=DIRECTION('ref_axis',(0.,0.,-1.)) ;
#84698=DIRECTION('center_axis',(0.,0.,-1.)) ;
#84699=DIRECTION('ref_axis',(1.,0.,0.)) ;
#84700=DIRECTION('center_axis',(-1.,0.,-1.7912294869673E-32)) ;
#84701=DIRECTION('ref_axis',(-1.7912294869673E-32,0.,1.)) ;
#84702=DIRECTION('center_axis',(-0.447219005479784,-5.60223355926168E-6,
0.894424485972007)) ;
#84703=DIRECTION('ref_axis',(0.894327914920142,0.014691703945553,0.447170811245287)) ;
#84704=DIRECTION('center_axis',(-1.,0.,0.)) ;
#84705=DIRECTION('ref_axis',(0.,0.,1.)) ;
#84706=DIRECTION('center_axis',(1.23908819712629E-16,-1.,7.2280144832367E-17)) ;
#84707=DIRECTION('ref_axis',(1.,1.23908819712629E-16,-8.95614743483648E-33)) ;
#84708=DIRECTION('center_axis',(-7.10036028217959E-6,-0.447220452189357,
0.894423762594181)) ;
#84709=DIRECTION('ref_axis',(-0.0148067719368954,-0.89432566327004,-0.447171519130424)) ;
#84710=DIRECTION('center_axis',(0.,-1.,1.0842021724855E-15)) ;
#84711=DIRECTION('ref_axis',(0.,-1.0842021724855E-15,-1.)) ;
#84712=DIRECTION('center_axis',(1.23908819712629E-16,-1.,1.23908819712629E-16)) ;
#84713=DIRECTION('ref_axis',(-9.81657386420148E-47,-1.23908819712629E-16,
-1.)) ;
#84714=DIRECTION('center_axis',(0.,-1.,0.)) ;
#84715=DIRECTION('ref_axis',(0.,0.,-1.)) ;
#84716=DIRECTION('',(-1.23908819712629E-16,1.,-1.23908819712629E-16)) ;
#84717=DIRECTION('center_axis',(1.,0.,1.40488587213121E-32)) ;
#84718=DIRECTION('ref_axis',(1.40488587213121E-32,0.,-1.)) ;
#84719=DIRECTION('center_axis',(-0.707106781186547,0.707106781186548,-6.41152859744984E-16)) ;
#84720=DIRECTION('ref_axis',(0.707106781186548,0.707106781186547,-2.22751953561763E-12)) ;
#84721=DIRECTION('center_axis',(1.,0.,0.)) ;
#84722=DIRECTION('ref_axis',(0.,0.,-1.)) ;
#84723=DIRECTION('center_axis',(0.,-1.,0.)) ;
#84724=DIRECTION('ref_axis',(0.,0.,-1.)) ;
#84725=DIRECTION('center_axis',(0.,0.,1.)) ;
#84726=DIRECTION('ref_axis',(-1.,0.,0.)) ;
#84727=DIRECTION('center_axis',(7.2280144832367E-17,0.,-1.)) ;
#84728=DIRECTION('ref_axis',(-1.,0.,-7.2280144832367E-17)) ;
#84729=DIRECTION('',(7.2280144832367E-17,0.,-1.)) ;
#84730=DIRECTION('center_axis',(0.,0.,-1.)) ;
#84731=DIRECTION('ref_axis',(-1.,0.,0.)) ;
#84732=DIRECTION('center_axis',(0.,1.,0.)) ;
#84733=DIRECTION('ref_axis',(1.,0.,0.)) ;
#84734=DIRECTION('center_axis',(0.,0.,1.)) ;
#84735=DIRECTION('ref_axis',(-1.,0.,0.)) ;
#84736=DIRECTION('center_axis',(0.,1.,0.)) ;
#84737=DIRECTION('ref_axis',(1.,0.,0.)) ;
#84738=DIRECTION('center_axis',(1.,0.,0.)) ;
#84739=DIRECTION('ref_axis',(0.,0.,1.)) ;
#84740=DIRECTION('center_axis',(0.,0.,-1.)) ;
#84741=DIRECTION('ref_axis',(1.,0.,0.)) ;
#84742=DIRECTION('center_axis',(-1.13380619344889E-16,1.,-1.23908819712629E-16)) ;
#84743=DIRECTION('ref_axis',(-1.40488587213121E-32,1.23908819712629E-16,
1.)) ;
#84744=DIRECTION('center_axis',(0.,1.,0.)) ;
#84745=DIRECTION('ref_axis',(0.,0.,1.)) ;
#84746=DIRECTION('center_axis',(7.2280144832367E-17,0.,-1.)) ;
#84747=DIRECTION('ref_axis',(-1.,0.,-7.2280144832367E-17)) ;
#84748=DIRECTION('center_axis',(0.,0.,1.)) ;
#84749=DIRECTION('ref_axis',(1.,0.,0.)) ;
#84750=DIRECTION('center_axis',(0.,1.,0.)) ;
#84751=DIRECTION('ref_axis',(1.,0.,0.)) ;
#84752=DIRECTION('center_axis',(0.,1.,0.)) ;
#84753=DIRECTION('ref_axis',(0.,0.,-1.)) ;
#84754=DIRECTION('center_axis',(1.,2.16840434497101E-15,-2.93873587705572E-31)) ;
#84755=DIRECTION('ref_axis',(2.16840434497101E-15,-1.,-1.03035812136257E-62)) ;
#84756=DIRECTION('center_axis',(-8.95614743483648E-33,0.,1.)) ;
#84757=DIRECTION('ref_axis',(1.,0.,8.95614743483648E-33)) ;
#84758=DIRECTION('center_axis',(-1.40488587213121E-32,1.23908819712629E-16,
1.)) ;
#84759=DIRECTION('ref_axis',(-1.74077750246726E-48,-1.,1.23908819712629E-16)) ;
#84760=DIRECTION('center_axis',(8.95614743483648E-33,1.0154535431059E-48,
-1.)) ;
#84761=DIRECTION('ref_axis',(-1.,9.09455164528354E-81,-8.95614743483648E-33)) ;
#84762=DIRECTION('center_axis',(2.16840434497101E-15,0.,-1.)) ;
#84763=DIRECTION('ref_axis',(-1.,0.,-2.16840434497101E-15)) ;
#84764=DIRECTION('',(-8.95614743483648E-33,-1.0154535431059E-48,1.)) ;
#84765=DIRECTION('center_axis',(-1.,-1.13380619344889E-16,0.)) ;
#84766=DIRECTION('ref_axis',(0.,-1.,0.)) ;
#84767=DIRECTION('center_axis',(0.,0.,1.)) ;
#84768=DIRECTION('ref_axis',(-1.,0.,0.)) ;
#84769=DIRECTION('center_axis',(0.,-1.,0.)) ;
#84770=DIRECTION('ref_axis',(0.,0.,-1.)) ;
#84771=DIRECTION('center_axis',(-1.,0.,0.)) ;
#84772=DIRECTION('ref_axis',(0.,0.,-1.)) ;
#84773=DIRECTION('center_axis',(1.,0.,1.40488587213121E-32)) ;
#84774=DIRECTION('ref_axis',(1.40488587213121E-32,0.,-1.)) ;
#84775=DIRECTION('',(1.,0.,1.40488587213121E-32)) ;
#84776=DIRECTION('center_axis',(1.,0.,0.)) ;
#84777=DIRECTION('ref_axis',(0.,0.,-1.)) ;
#84778=DIRECTION('center_axis',(-1.40488587213121E-32,1.23908819712629E-16,
1.)) ;
#84779=DIRECTION('ref_axis',(0.,-1.,0.)) ;
#84780=DIRECTION('center_axis',(0.,-1.,0.)) ;
#84781=DIRECTION('ref_axis',(0.,0.,1.)) ;
#84782=DIRECTION('center_axis',(0.,1.,0.)) ;
#84783=DIRECTION('ref_axis',(1.,0.,0.)) ;
#84784=DIRECTION('center_axis',(1.,0.,0.)) ;
#84785=DIRECTION('ref_axis',(0.,0.,1.)) ;
#84786=DIRECTION('center_axis',(0.,1.,0.)) ;
#84787=DIRECTION('ref_axis',(0.,0.,-1.)) ;
#84788=DIRECTION('center_axis',(0.,0.,1.)) ;
#84789=DIRECTION('ref_axis',(1.,0.,0.)) ;
#84790=DIRECTION('center_axis',(0.,0.,1.)) ;
#84791=DIRECTION('ref_axis',(1.,0.,0.)) ;
#84792=DIRECTION('center_axis',(1.,0.,1.40488587213121E-32)) ;
#84793=DIRECTION('ref_axis',(1.40488587213121E-32,0.,-1.)) ;
#84794=DIRECTION('center_axis',(-0.707106781186552,0.707106781186543,-7.9502954608381E-15)) ;
#84795=DIRECTION('ref_axis',(0.707106781186543,0.707106781186552,-7.24201771566408E-13)) ;
#84796=DIRECTION('center_axis',(-1.23908819712629E-16,1.,-1.23908819712629E-16)) ;
#84797=DIRECTION('ref_axis',(9.81657386420148E-47,1.23908819712629E-16,
1.)) ;
#84798=DIRECTION('',(1.23908819712629E-16,-1.,1.23908819712629E-16)) ;
#84799=DIRECTION('center_axis',(-1.,-1.13380619344889E-16,0.)) ;
#84800=DIRECTION('ref_axis',(0.,-1.,0.)) ;
#84801=DIRECTION('center_axis',(0.,-1.,0.)) ;
#84802=DIRECTION('ref_axis',(0.,0.,1.)) ;
#84803=DIRECTION('center_axis',(1.13380619344889E-16,-1.,1.23908819712629E-16)) ;
#84804=DIRECTION('ref_axis',(1.40488587213121E-32,-1.23908819712629E-16,
-1.)) ;
#84805=DIRECTION('center_axis',(-1.5529910948782E-31,-4.47619207437002E-16,
1.)) ;
#84806=DIRECTION('ref_axis',(6.951486430461E-47,-1.,-4.47619207437002E-16)) ;
#84807=DIRECTION('center_axis',(0.,2.16840434497101E-15,-1.)) ;
#84808=DIRECTION('ref_axis',(0.,1.,2.16840434497101E-15)) ;
#84809=DIRECTION('center_axis',(0.,1.,0.)) ;
#84810=DIRECTION('ref_axis',(1.,0.,0.)) ;
#84811=DIRECTION('center_axis',(3.85194802226865E-15,0.888198741900269,
-0.45945945945946)) ;
#84812=DIRECTION('ref_axis',(3.25260651745654E-15,-0.45945945945946,-0.888198741900269)) ;
#84813=DIRECTION('center_axis',(-1.,0.,1.22067519501986E-15)) ;
#84814=DIRECTION('ref_axis',(-1.22067519501986E-15,3.46944695195364E-14,
-1.)) ;
#84815=DIRECTION('center_axis',(1.5529910948782E-31,4.47619207437002E-16,
-1.)) ;
#84816=DIRECTION('ref_axis',(-6.951486430461E-47,1.,4.47619207437002E-16)) ;
#84817=DIRECTION('center_axis',(0.,0.,1.)) ;
#84818=DIRECTION('ref_axis',(1.,0.,0.)) ;
#84819=DIRECTION('center_axis',(1.,-3.46944695195361E-16,0.)) ;
#84820=DIRECTION('ref_axis',(3.46944695195361E-16,1.,0.)) ;
#84821=DIRECTION('center_axis',(-1.,3.46944695195361E-16,0.)) ;
#84822=DIRECTION('ref_axis',(3.46944695195361E-16,1.,3.46944695195362E-14)) ;
#84823=DIRECTION('center_axis',(1.,-3.46944695195361E-16,0.)) ;
#84824=DIRECTION('ref_axis',(3.41607084500048E-16,1.,0.)) ;
#84825=DIRECTION('center_axis',(0.,0.459459459459457,-0.888198741900271)) ;
#84826=DIRECTION('ref_axis',(0.,0.888198741900271,0.459459459459457)) ;
#84827=DIRECTION('center_axis',(0.,0.,1.)) ;
#84828=DIRECTION('ref_axis',(1.,0.,0.)) ;
#84829=DIRECTION('center_axis',(0.,0.,-1.)) ;
#84830=DIRECTION('ref_axis',(-1.,0.,0.)) ;
#84831=DIRECTION('center_axis',(-1.,3.46944695195361E-16,0.)) ;
#84832=DIRECTION('ref_axis',(-3.46944695195361E-16,-1.,0.)) ;
#84833=DIRECTION('center_axis',(-1.,3.46944695195361E-16,0.)) ;
#84834=DIRECTION('ref_axis',(-3.46944695195361E-16,-1.,0.)) ;
#84835=DIRECTION('center_axis',(-1.,3.46944695195361E-16,0.)) ;
#84836=DIRECTION('ref_axis',(3.46944695195361E-16,1.,6.93889390390722E-14)) ;
#84837=DIRECTION('center_axis',(1.,-3.46944695195361E-16,0.)) ;
#84838=DIRECTION('ref_axis',(0.,1.,0.)) ;
#84839=DIRECTION('center_axis',(0.,-0.888198741900269,0.459459459459461)) ;
#84840=DIRECTION('ref_axis',(0.,0.459459459459461,0.888198741900269)) ;
#84841=DIRECTION('center_axis',(0.,1.,0.)) ;
#84842=DIRECTION('ref_axis',(1.,0.,0.)) ;
#84843=DIRECTION('center_axis',(0.,1.,0.)) ;
#84844=DIRECTION('ref_axis',(0.,0.,-1.)) ;
#84845=DIRECTION('center_axis',(-1.,0.,0.)) ;
#84846=DIRECTION('ref_axis',(0.,-8.67361737988409E-15,-1.)) ;
#84847=DIRECTION('center_axis',(1.,-3.46944695195361E-16,0.)) ;
#84848=DIRECTION('ref_axis',(3.70074341541719E-16,1.,0.)) ;
#84849=DIRECTION('center_axis',(0.,0.63294893130157,-0.774193548387094)) ;
#84850=DIRECTION('ref_axis',(-1.08420217248549E-15,-0.774193548387094,-0.63294893130157)) ;
#84851=DIRECTION('center_axis',(1.,-3.46944695195361E-16,0.)) ;
#84852=DIRECTION('ref_axis',(3.80647894157197E-16,1.,0.)) ;
#84853=DIRECTION('center_axis',(0.,-0.45945945945946,0.888198741900269)) ;
#84854=DIRECTION('ref_axis',(0.,-0.888198741900269,-0.45945945945946)) ;
#84855=DIRECTION('center_axis',(1.,-3.46944695195361E-16,0.)) ;
#84856=DIRECTION('ref_axis',(3.46944695195361E-16,1.,0.)) ;
#84857=DIRECTION('center_axis',(-1.,3.46944695195361E-16,0.)) ;
#84858=DIRECTION('ref_axis',(3.46944695195361E-16,1.,0.)) ;
#84859=DIRECTION('center_axis',(-3.46944695195361E-16,-1.,-2.45739631480277E-16)) ;
#84860=DIRECTION('ref_axis',(1.,-3.46944695195361E-16,-8.52580615413453E-32)) ;
#84861=DIRECTION('center_axis',(0.,1.,0.)) ;
#84862=DIRECTION('ref_axis',(0.,0.,1.)) ;
#84863=DIRECTION('center_axis',(1.,-3.46944695195361E-16,0.)) ;
#84864=DIRECTION('ref_axis',(3.33066907387547E-16,1.,0.)) ;
#84865=DIRECTION('center_axis',(8.02036034720251E-16,0.293103448275862,
-0.956080733311157)) ;
#84866=DIRECTION('ref_axis',(1.13164713162994E-29,0.956080733311157,0.293103448275862)) ;
#84867=DIRECTION('center_axis',(-1.,3.46944695195361E-16,0.)) ;
#84868=DIRECTION('ref_axis',(-3.46944695195361E-16,-1.,0.)) ;
#84869=DIRECTION('center_axis',(-1.,3.46944695195361E-16,0.)) ;
#84870=DIRECTION('ref_axis',(-3.46944695195361E-16,-1.,0.)) ;
#84871=DIRECTION('center_axis',(-1.,3.46944695195361E-16,0.)) ;
#84872=DIRECTION('ref_axis',(-3.46944695195361E-16,-1.,0.)) ;
#84873=DIRECTION('center_axis',(0.,0.,-1.)) ;
#84874=DIRECTION('ref_axis',(-1.,0.,0.)) ;
#84875=DIRECTION('center_axis',(0.,0.,1.)) ;
#84876=DIRECTION('ref_axis',(1.,0.,0.)) ;
#84877=DIRECTION('center_axis',(-1.5529910948782E-31,-4.47619207437002E-16,
-1.)) ;
#84878=DIRECTION('ref_axis',(-6.95148643046101E-47,1.,-4.47619207437002E-16)) ;
#84879=DIRECTION('center_axis',(2.16840434497101E-15,0.,1.)) ;
#84880=DIRECTION('ref_axis',(1.,0.,-2.16840434497101E-15)) ;
#84881=DIRECTION('center_axis',(1.,-3.46944695195361E-16,0.)) ;
#84882=DIRECTION('ref_axis',(0.,1.,0.)) ;
#84883=DIRECTION('center_axis',(0.,-1.,0.)) ;
#84884=DIRECTION('ref_axis',(0.,0.,1.)) ;
#84885=DIRECTION('center_axis',(0.577350269189627,0.577350269189627,0.577350269189623)) ;
#84886=DIRECTION('ref_axis',(-0.707106781186548,2.22044604925032E-15,0.707106781186547)) ;
#84887=DIRECTION('center_axis',(-1.,3.46944695195361E-16,0.)) ;
#84888=DIRECTION('ref_axis',(-3.70074341541719E-16,-1.,0.)) ;
#84889=DIRECTION('center_axis',(0.,0.63294893130157,0.774193548387094)) ;
#84890=DIRECTION('ref_axis',(0.,0.774193548387094,-0.63294893130157)) ;
#84891=DIRECTION('center_axis',(0.,1.,0.)) ;
#84892=DIRECTION('ref_axis',(1.,0.,0.)) ;
#84893=DIRECTION('center_axis',(-1.,0.,0.)) ;
#84894=DIRECTION('ref_axis',(0.,1.73472347597682E-14,-1.)) ;
#84895=DIRECTION('center_axis',(0.,0.888198741900271,0.459459459459457)) ;
#84896=DIRECTION('ref_axis',(-1.08420217248551E-15,0.459459459459457,-0.888198741900271)) ;
#84897=DIRECTION('center_axis',(3.46944695195361E-16,1.,2.45739631480277E-16)) ;
#84898=DIRECTION('ref_axis',(-1.,3.46944695195361E-16,8.52580615413453E-32)) ;
#84899=DIRECTION('center_axis',(-1.,3.46944695195361E-16,0.)) ;
#84900=DIRECTION('ref_axis',(-3.33066907387547E-16,-1.,0.)) ;
#84901=DIRECTION('center_axis',(0.,0.293103448275864,0.956080733311156)) ;
#84902=DIRECTION('ref_axis',(0.,-0.956080733311156,0.293103448275864)) ;
#84903=DIRECTION('center_axis',(-3.46944695195361E-16,-1.,-1.06487173641454E-15)) ;
#84904=DIRECTION('ref_axis',(3.69451600012496E-31,1.06487173641454E-15,
-1.)) ;
#84905=DIRECTION('center_axis',(0.,-1.,0.)) ;
#84906=DIRECTION('ref_axis',(0.,0.,-1.)) ;
#84907=DIRECTION('center_axis',(0.,1.,0.)) ;
#84908=DIRECTION('ref_axis',(0.,0.,1.)) ;
#84909=DIRECTION('center_axis',(-1.,3.46944695195361E-16,0.)) ;
#84910=DIRECTION('ref_axis',(-3.41607084500048E-16,-1.,0.)) ;
#84911=DIRECTION('center_axis',(-4.88154879316133E-15,0.45945945945946,
0.888198741900269)) ;
#84912=DIRECTION('ref_axis',(-3.39148554690438E-29,-0.888198741900269,0.45945945945946)) ;
#84913=DIRECTION('center_axis',(1.,-3.46944695195361E-16,0.)) ;
#84914=DIRECTION('ref_axis',(3.46944695195361E-16,1.,0.)) ;
#84915=DIRECTION('center_axis',(-1.,3.46944695195361E-16,0.)) ;
#84916=DIRECTION('ref_axis',(3.46944695195361E-16,1.,0.)) ;
#84917=DIRECTION('center_axis',(-1.5529910948782E-31,-4.47619207437002E-16,
-1.)) ;
#84918=DIRECTION('ref_axis',(-6.95148643046101E-47,1.,-4.47619207437002E-16)) ;
#84919=DIRECTION('center_axis',(0.,0.,-1.)) ;
#84920=DIRECTION('ref_axis',(-1.,0.,0.)) ;
#84921=DIRECTION('center_axis',(0.,0.224137931034483,-0.974557431797419)) ;
#84922=DIRECTION('ref_axis',(0.,-0.974557431797419,-0.224137931034483)) ;
#84923=DIRECTION('center_axis',(0.577350269189627,0.577350269189627,0.577350269189623)) ;
#84924=DIRECTION('ref_axis',(-0.707106781186548,2.22044604925032E-15,0.707106781186547)) ;
#84925=DIRECTION('center_axis',(0.408248290463864,-0.816496580927725,0.408248290463864)) ;
#84926=DIRECTION('ref_axis',(0.707106781186545,-2.77555756156289E-15,-0.70710678118655)) ;
#84927=DIRECTION('center_axis',(0.,1.,0.)) ;
#84928=DIRECTION('ref_axis',(1.,0.,0.)) ;
#84929=DIRECTION('center_axis',(-1.,0.,0.)) ;
#84930=DIRECTION('ref_axis',(0.,0.,-1.)) ;
#84931=DIRECTION('center_axis',(1.,-3.46944695195361E-16,0.)) ;
#84932=DIRECTION('ref_axis',(0.,1.,0.)) ;
#84933=DIRECTION('center_axis',(9.96293888229924E-16,-0.888198741900269,
-0.45945945945946)) ;
#84934=DIRECTION('ref_axis',(-3.00809911926502E-30,-0.45945945945946,0.888198741900269)) ;
#84935=DIRECTION('center_axis',(1.,-3.46944695195361E-16,0.)) ;
#84936=DIRECTION('ref_axis',(-3.70074341541719E-16,-1.,0.)) ;
#84937=DIRECTION('center_axis',(1.58436874053304E-16,-0.224137931034483,
-0.974557431797419)) ;
#84938=DIRECTION('ref_axis',(2.18893094986727E-31,0.974557431797419,-0.224137931034483)) ;
#84939=DIRECTION('center_axis',(1.,-3.46944695195361E-16,0.)) ;
#84940=DIRECTION('ref_axis',(3.46944695195361E-16,1.,0.)) ;
#84941=DIRECTION('center_axis',(-1.,3.46944695195361E-16,0.)) ;
#84942=DIRECTION('ref_axis',(3.46944695195361E-16,1.,0.)) ;
#84943=DIRECTION('center_axis',(1.,-3.46944695195361E-16,0.)) ;
#84944=DIRECTION('ref_axis',(3.80647894157197E-16,1.,0.)) ;
#84945=DIRECTION('center_axis',(0.,-0.45945945945946,-0.888198741900269)) ;
#84946=DIRECTION('ref_axis',(0.,0.888198741900269,-0.45945945945946)) ;
#84947=DIRECTION('center_axis',(1.,-3.46944695195361E-16,0.)) ;
#84948=DIRECTION('ref_axis',(0.,1.,0.)) ;
#84949=DIRECTION('center_axis',(0.,-1.,0.)) ;
#84950=DIRECTION('ref_axis',(0.,0.,1.)) ;
#84951=DIRECTION('center_axis',(-3.46944695195361E-16,-1.,-1.06487173641454E-15)) ;
#84952=DIRECTION('ref_axis',(3.69451600012496E-31,1.06487173641454E-15,
-1.)) ;
#84953=DIRECTION('center_axis',(0.,0.,1.)) ;
#84954=DIRECTION('ref_axis',(1.,0.,0.)) ;
#84955=DIRECTION('center_axis',(0.,-1.,0.)) ;
#84956=DIRECTION('ref_axis',(0.,0.,-1.)) ;
#84957=DIRECTION('center_axis',(0.,-1.,0.)) ;
#84958=DIRECTION('ref_axis',(0.,0.,-1.)) ;
#84959=DIRECTION('center_axis',(0.,1.,0.)) ;
#84960=DIRECTION('ref_axis',(0.,0.,-1.)) ;
#84961=DIRECTION('center_axis',(0.,0.,1.)) ;
#84962=DIRECTION('ref_axis',(1.,0.,0.)) ;
#84963=DIRECTION('center_axis',(8.67361737988404E-15,-1.,0.)) ;
#84964=DIRECTION('ref_axis',(1.,8.67361737988404E-15,0.)) ;
#84965=DIRECTION('center_axis',(0.497468338163091,-0.710669054518702,0.497468338163091)) ;
#84966=DIRECTION('ref_axis',(0.81923192051904,0.573462344363328,8.04804396179112E-16)) ;
#84967=DIRECTION('center_axis',(0.497468338163091,-0.710669054518702,0.497468338163091)) ;
#84968=DIRECTION('ref_axis',(0.81923192051904,0.573462344363328,7.6535433881835E-16)) ;
#84969=DIRECTION('center_axis',(0.497468338163092,-0.7106690545187,0.497468338163092)) ;
#84970=DIRECTION('ref_axis',(-1.24903860074368E-15,-0.57346234436333,-0.819231920519039)) ;
#84971=DIRECTION('center_axis',(0.,0.,1.)) ;
#84972=DIRECTION('ref_axis',(1.,0.,0.)) ;
#84973=DIRECTION('center_axis',(0.,-1.,0.)) ;
#84974=DIRECTION('ref_axis',(0.,0.,-1.)) ;
#84975=DIRECTION('center_axis',(0.,1.,0.)) ;
#84976=DIRECTION('ref_axis',(0.,0.,1.)) ;
#84977=DIRECTION('center_axis',(0.,1.,0.)) ;
#84978=DIRECTION('ref_axis',(0.,0.,1.)) ;
#84979=DIRECTION('center_axis',(0.,1.,0.)) ;
#84980=DIRECTION('ref_axis',(1.,0.,0.)) ;
#84981=DIRECTION('center_axis',(-1.98515611757154E-15,0.,1.)) ;
#84982=DIRECTION('ref_axis',(-1.,0.,-1.98515611757154E-15)) ;
#84983=DIRECTION('center_axis',(1.,-4.06575814682065E-16,2.84603070277446E-16)) ;
#84984=DIRECTION('ref_axis',(-4.06575814682065E-16,-1.,6.48893816316174E-47)) ;
#84985=DIRECTION('center_axis',(0.,1.,0.)) ;
#84986=DIRECTION('ref_axis',(0.,0.,1.)) ;
#84987=DIRECTION('center_axis',(0.,1.,0.)) ;
#84988=DIRECTION('ref_axis',(0.,0.,1.)) ;
#84989=DIRECTION('center_axis',(0.497468338163091,0.710669054518702,-0.497468338163091)) ;
#84990=DIRECTION('ref_axis',(-0.81923192051904,0.573462344363328,7.6535433881835E-16)) ;
#84991=DIRECTION('center_axis',(-0.497468338163091,-0.710669054518702,0.497468338163091)) ;
#84992=DIRECTION('ref_axis',(-0.81923192051904,0.573462344363329,2.81956803083991E-15)) ;
#84993=DIRECTION('center_axis',(-0.497468338163093,-0.7106690545187,0.497468338163091)) ;
#84994=DIRECTION('ref_axis',(0.819231920519039,-0.573462344363331,1.48853464230757E-16)) ;
#84995=DIRECTION('center_axis',(1.,0.,0.)) ;
#84996=DIRECTION('ref_axis',(0.,0.,-1.)) ;
#84997=DIRECTION('center_axis',(1.,0.,-9.9257805878577E-16)) ;
#84998=DIRECTION('ref_axis',(-9.9257805878577E-16,0.,-1.)) ;
#84999=DIRECTION('center_axis',(0.,0.,-1.)) ;
#85000=DIRECTION('ref_axis',(-1.,0.,0.)) ;
#85001=DIRECTION('center_axis',(-1.23327997120227E-15,1.76182853028895E-15,
1.)) ;
#85002=DIRECTION('ref_axis',(-2.17282783909808E-30,-1.,1.76182853028895E-15)) ;
#85003=DIRECTION('center_axis',(-0.497468338163091,0.710669054518702,0.497468338163091)) ;
#85004=DIRECTION('ref_axis',(-0.81923192051904,-0.573462344363328,7.6535433881835E-16)) ;
#85005=DIRECTION('center_axis',(0.497468338163091,-0.710669054518702,-0.497468338163091)) ;
#85006=DIRECTION('ref_axis',(-0.819231920519018,-0.57346234436336,6.87084924063159E-14)) ;
#85007=DIRECTION('center_axis',(0.497468338163093,-0.7106690545187,-0.497468338163091)) ;
#85008=DIRECTION('ref_axis',(0.819231920519039,0.573462344363331,2.16059097207149E-16)) ;
#85009=DIRECTION('center_axis',(0.,1.,0.)) ;
#85010=DIRECTION('ref_axis',(1.,0.,0.)) ;
#85011=DIRECTION('center_axis',(-1.13841228110978E-15,-1.62630325872826E-15,
1.)) ;
#85012=DIRECTION('ref_axis',(3.52365706057789E-15,1.,1.62630325872826E-15)) ;
#85013=DIRECTION('center_axis',(0.,1.,0.)) ;
#85014=DIRECTION('ref_axis',(1.,0.,0.)) ;
#85015=DIRECTION('center_axis',(1.,0.,-1.65429676464295E-16)) ;
#85016=DIRECTION('ref_axis',(1.65429676464295E-16,4.33680868994204E-15,
1.)) ;
#85017=DIRECTION('center_axis',(0.,0.,-1.)) ;
#85018=DIRECTION('ref_axis',(-1.,0.,0.)) ;
#85019=DIRECTION('center_axis',(3.3085935292859E-16,0.,1.)) ;
#85020=DIRECTION('ref_axis',(1.,0.,-3.3085935292859E-16)) ;
#85021=DIRECTION('center_axis',(1.,0.,0.)) ;
#85022=DIRECTION('ref_axis',(0.,0.,-1.)) ;
#85023=DIRECTION('center_axis',(1.,1.21972744404619E-15,8.53809210832338E-16)) ;
#85024=DIRECTION('ref_axis',(-1.21972744404619E-15,1.,-2.84382165153726E-47)) ;
#85025=DIRECTION('center_axis',(0.,1.,0.)) ;
#85026=DIRECTION('ref_axis',(1.,0.,0.)) ;
#85027=DIRECTION('center_axis',(0.497468338163092,0.710669054518701,0.497468338163092)) ;
#85028=DIRECTION('ref_axis',(1.11733937654106E-14,0.573462344363324,-0.819231920519043)) ;
#85029=DIRECTION('center_axis',(-0.497468338163091,-0.710669054518702,-0.497468338163091)) ;
#85030=DIRECTION('ref_axis',(0.81923192051904,-0.573462344363328,7.6535433881835E-16)) ;
#85031=DIRECTION('center_axis',(-0.497468338163091,-0.710669054518702,-0.497468338163091)) ;
#85032=DIRECTION('ref_axis',(0.81923192051904,-0.573462344363328,7.6535433881835E-16)) ;
#85033=DIRECTION('center_axis',(0.,-1.,0.)) ;
#85034=DIRECTION('ref_axis',(0.,0.,-1.)) ;
#85035=DIRECTION('center_axis',(0.,1.,0.)) ;
#85036=DIRECTION('ref_axis',(0.,0.,-1.)) ;
#85037=DIRECTION('center_axis',(-8.67361737988403E-15,1.,0.)) ;
#85038=DIRECTION('ref_axis',(-1.,-8.67361737988403E-15,0.)) ;
#85039=DIRECTION('center_axis',(0.,0.,1.)) ;
#85040=DIRECTION('ref_axis',(1.,0.,0.)) ;
#85041=DIRECTION('center_axis',(1.,6.67201336914158E-17,0.)) ;
#85042=DIRECTION('ref_axis',(-6.67201336914158E-17,1.,0.)) ;
#85043=DIRECTION('center_axis',(-1.,-6.67201336914158E-17,0.)) ;
#85044=DIRECTION('ref_axis',(-6.67201336914158E-17,1.,0.)) ;
#85045=DIRECTION('center_axis',(-1.,1.33440267382831E-16,0.)) ;
#85046=DIRECTION('ref_axis',(-1.33440267382831E-16,-1.,0.)) ;
#85047=DIRECTION('center_axis',(-1.,1.33440267382831E-16,0.)) ;
#85048=DIRECTION('ref_axis',(-1.33440267382831E-16,-1.,0.)) ;
#85049=DIRECTION('center_axis',(0.710669054518702,0.497468338163091,0.497468338163091)) ;
#85050=DIRECTION('ref_axis',(-0.573462344363328,0.819231920519041,3.92980824865032E-16)) ;
#85051=DIRECTION('center_axis',(0.710669054518702,0.497468338163091,0.497468338163091)) ;
#85052=DIRECTION('ref_axis',(-0.573462344363328,0.819231920519041,3.92980824865032E-16)) ;
#85053=DIRECTION('center_axis',(0.710669054518701,0.497468338163091,0.497468338163092)) ;
#85054=DIRECTION('ref_axis',(0.57346234436333,-1.81382726107456E-15,-0.819231920519039)) ;
#85055=DIRECTION('center_axis',(-0.710669054518702,0.497468338163091,-0.497468338163091)) ;
#85056=DIRECTION('ref_axis',(-0.573462344363328,-0.819231920519041,6.69271761853466E-16)) ;
#85057=DIRECTION('center_axis',(0.710669054518702,-0.497468338163091,0.497468338163091)) ;
#85058=DIRECTION('ref_axis',(-0.573462344363328,-0.819231920519041,6.69271761853466E-16)) ;
#85059=DIRECTION('center_axis',(0.7106690545187,-0.497468338163094,0.497468338163091)) ;
#85060=DIRECTION('ref_axis',(0.573462344363331,0.819231920519038,2.86772422505918E-16)) ;
#85061=DIRECTION('center_axis',(0.,1.,-9.34081871679819E-17)) ;
#85062=DIRECTION('ref_axis',(0.,9.34081871679819E-17,1.)) ;
#85063=DIRECTION('center_axis',(-4.33680868994205E-15,-1.,-3.03576608295944E-15)) ;
#85064=DIRECTION('ref_axis',(1.,-4.33680868994205E-15,-1.12103877145985E-44)) ;
#85065=DIRECTION('center_axis',(0.,1.,5.29374964685745E-15)) ;
#85066=DIRECTION('ref_axis',(0.,-5.29374964685745E-15,1.)) ;
#85067=DIRECTION('center_axis',(0.,1.,0.)) ;
#85068=DIRECTION('ref_axis',(1.,0.,0.)) ;
#85069=DIRECTION('center_axis',(0.,6.45175738210751E-15,1.)) ;
#85070=DIRECTION('ref_axis',(0.,1.,-6.45175738210751E-15)) ;
#85071=DIRECTION('center_axis',(-1.,-6.67201336914158E-17,0.)) ;
#85072=DIRECTION('ref_axis',(6.67201336914158E-17,-1.,0.)) ;
#85073=DIRECTION('center_axis',(-1.,-6.67201336914158E-17,0.)) ;
#85074=DIRECTION('ref_axis',(6.67201336914158E-17,-1.,0.)) ;
#85075=DIRECTION('center_axis',(1.,-1.33440267382831E-16,0.)) ;
#85076=DIRECTION('ref_axis',(1.33440267382831E-16,1.,0.)) ;
#85077=DIRECTION('center_axis',(-1.,1.33440267382831E-16,0.)) ;
#85078=DIRECTION('ref_axis',(1.33440267382831E-16,1.,0.)) ;
#85079=DIRECTION('center_axis',(0.,1.,0.)) ;
#85080=DIRECTION('ref_axis',(1.,0.,0.)) ;
#85081=DIRECTION('center_axis',(1.76182853028896E-15,-1.23327997120227E-15,
1.)) ;
#85082=DIRECTION('ref_axis',(-1.,-2.1728278390981E-30,1.76182853028896E-15)) ;
#85083=DIRECTION('center_axis',(0.,0.,-1.)) ;
#85084=DIRECTION('ref_axis',(-1.,0.,0.)) ;
#85085=DIRECTION('center_axis',(-2.71050543121378E-16,-1.89735380184965E-16,
1.)) ;
#85086=DIRECTION('ref_axis',(1.,-5.14278778484758E-32,2.71050543121378E-16)) ;
#85087=DIRECTION('center_axis',(-0.710669054518702,-0.497468338163091,0.497468338163091)) ;
#85088=DIRECTION('ref_axis',(0.573462344363328,-0.819231920519041,3.92980824865032E-16)) ;
#85089=DIRECTION('center_axis',(0.710669054518702,0.497468338163091,-0.497468338163091)) ;
#85090=DIRECTION('ref_axis',(0.573462344363328,-0.819231920519041,3.92980824865032E-16)) ;
#85091=DIRECTION('center_axis',(0.710669054518701,0.497468338163091,-0.497468338163092)) ;
#85092=DIRECTION('ref_axis',(-0.57346234436333,1.88103289405095E-15,-0.819231920519039)) ;
#85093=DIRECTION('center_axis',(0.710669054518702,-0.497468338163091,-0.497468338163091)) ;
#85094=DIRECTION('ref_axis',(0.573462344363328,0.819231920519041,6.69271761853466E-16)) ;
#85095=DIRECTION('center_axis',(0.710669054518702,-0.497468338163091,-0.497468338163091)) ;
#85096=DIRECTION('ref_axis',(0.573462344363328,0.819231920519041,6.69271761853466E-16)) ;
#85097=DIRECTION('center_axis',(0.7106690545187,-0.497468338163091,-0.497468338163093)) ;
#85098=DIRECTION('ref_axis',(-0.573462344363331,-1.17187023180681E-15,-0.819231920519038)) ;
#85099=DIRECTION('center_axis',(0.,0.,-1.)) ;
#85100=DIRECTION('ref_axis',(-1.,0.,0.)) ;
#85101=DIRECTION('center_axis',(0.,1.15800773525007E-15,1.)) ;
#85102=DIRECTION('ref_axis',(0.,-1.,1.15800773525007E-15)) ;
#85103=DIRECTION('center_axis',(0.,1.,0.)) ;
#85104=DIRECTION('ref_axis',(1.,0.,0.)) ;
#85105=DIRECTION('center_axis',(0.,1.,0.)) ;
#85106=DIRECTION('ref_axis',(0.,0.,-1.)) ;
#85107=DIRECTION('center_axis',(0.,1.,0.)) ;
#85108=DIRECTION('ref_axis',(1.,0.,0.)) ;
#85109=DIRECTION('center_axis',(4.33680868994204E-15,-1.,-3.03576608295944E-15)) ;
#85110=DIRECTION('ref_axis',(-1.,-4.33680868994204E-15,5.60519385729927E-45)) ;
#85111=DIRECTION('center_axis',(0.,1.,9.34081871679819E-17)) ;
#85112=DIRECTION('ref_axis',(0.,-9.34081871679819E-17,1.)) ;
#85113=DIRECTION('center_axis',(0.,0.,1.)) ;
#85114=DIRECTION('ref_axis',(1.,0.,0.)) ;
#85115=DIRECTION('center_axis',(-2.16840434497102E-15,-3.61400724161847E-16,
1.)) ;
#85116=DIRECTION('ref_axis',(1.,-7.83662900548222E-31,2.16840434497102E-15)) ;
#85117=DIRECTION('center_axis',(0.973328526784575,0.162221421130762,-0.162221421130763)) ;
#85118=DIRECTION('ref_axis',(-0.164398987305358,9.23743777622416E-16,-0.986393923832144)) ;
#85119=DIRECTION('center_axis',(0.973328526784574,0.162221421130765,-0.162221421130767)) ;
#85120=DIRECTION('ref_axis',(-0.164398987305362,1.88956506020588E-16,-0.986393923832143)) ;
#85121=DIRECTION('center_axis',(0.,1.,0.)) ;
#85122=DIRECTION('ref_axis',(1.,0.,0.)) ;
#85123=DIRECTION('center_axis',(0.,1.,-8.79325913341701E-15)) ;
#85124=DIRECTION('ref_axis',(1.73472347597682E-14,-8.79325913341701E-15,
-1.)) ;
#85125=DIRECTION('center_axis',(0.,0.,1.)) ;
#85126=DIRECTION('ref_axis',(1.,0.,0.)) ;
#85127=DIRECTION('center_axis',(0.,-2.28569887277128E-15,1.)) ;
#85128=DIRECTION('ref_axis',(0.,-1.,-2.28569887277128E-15)) ;
#85129=DIRECTION('center_axis',(1.73472347597681E-15,-1.,-2.89120579329468E-16)) ;
#85130=DIRECTION('ref_axis',(1.,1.73472347597681E-15,5.01544256350843E-31)) ;
#85131=DIRECTION('center_axis',(8.67361737988409E-15,1.,-1.44560289664739E-15)) ;
#85132=DIRECTION('ref_axis',(-1.,8.67361737988409E-15,-1.40129846432482E-45)) ;
#85133=DIRECTION('center_axis',(0.,1.,0.)) ;
#85134=DIRECTION('ref_axis',(1.,0.,0.)) ;
#85135=DIRECTION('center_axis',(-0.937042571331634,0.312347523777217,0.156173761888611)) ;
#85136=DIRECTION('ref_axis',(0.316227766016843,0.948683298050512,6.71158276827649E-18)) ;
#85137=DIRECTION('center_axis',(0.937042571331636,-0.312347523777212,-0.156173761888606)) ;
#85138=DIRECTION('ref_axis',(0.316227766016838,0.948683298050514,8.61595672567599E-16)) ;
#85139=DIRECTION('center_axis',(-0.973328526784575,-0.162221421130762,-0.162221421130763)) ;
#85140=DIRECTION('ref_axis',(-0.164398987305358,9.23743777622416E-16,0.986393923832144)) ;
#85141=DIRECTION('center_axis',(0.978231976292136,-0.146734796047237,-0.146734795425481)) ;
#85142=DIRECTION('ref_axis',(0.182318633544167,0.945435290916785,0.270022270473533)) ;
#85143=DIRECTION('center_axis',(0.973328526784574,0.162221421130767,0.162221421130768)) ;
#85144=DIRECTION('ref_axis',(0.164398987305363,-6.69215935033609E-18,-0.986393923832143)) ;
#85145=DIRECTION('center_axis',(0.,0.,1.)) ;
#85146=DIRECTION('ref_axis',(1.,0.,0.)) ;
#85147=DIRECTION('center_axis',(0.,2.19831478335425E-15,-1.)) ;
#85148=DIRECTION('ref_axis',(0.,1.,2.19831478335425E-15)) ;
#85149=DIRECTION('center_axis',(0.,1.,0.)) ;
#85150=DIRECTION('ref_axis',(1.,0.,0.)) ;
#85151=DIRECTION('center_axis',(8.67361737988408E-15,1.,1.44560289664739E-15)) ;
#85152=DIRECTION('ref_axis',(1.,-8.67361737988408E-15,5.60519385729927E-45)) ;
#85153=DIRECTION('center_axis',(1.73472347597681E-15,-1.,2.89120579329468E-16)) ;
#85154=DIRECTION('ref_axis',(1.,1.73472347597681E-15,-5.01544256350843E-31)) ;
#85155=DIRECTION('center_axis',(0.,1.,0.)) ;
#85156=DIRECTION('ref_axis',(0.,0.,1.)) ;
#85157=DIRECTION('center_axis',(0.,0.,1.)) ;
#85158=DIRECTION('ref_axis',(1.,0.,0.)) ;
#85159=DIRECTION('center_axis',(3.25260651745652E-15,-1.08420217248553E-15,
-1.)) ;
#85160=DIRECTION('ref_axis',(-1.,-3.52648305246695E-30,-3.25260651745652E-15)) ;
#85161=DIRECTION('center_axis',(0.,1.,0.)) ;
#85162=DIRECTION('ref_axis',(1.,0.,0.)) ;
#85163=DIRECTION('center_axis',(-0.937042571331635,0.312347523777215,-0.15617376188861)) ;
#85164=DIRECTION('ref_axis',(0.316227766016841,0.948683298050513,6.5590042956861E-18)) ;
#85165=DIRECTION('center_axis',(-0.937042571331636,0.312347523777212,-0.156173761888606)) ;
#85166=DIRECTION('ref_axis',(0.331350514299552,0.654034959159453,-0.680033167478407)) ;
#85167=DIRECTION('center_axis',(0.96151972409117,0.245047216428557,-0.124224320904791)) ;
#85168=DIRECTION('ref_axis',(0.262092069904638,-0.682554728314085,0.682221950503784)) ;
#85169=DIRECTION('center_axis',(2.65552944032596E-32,3.29043518662928E-48,
-1.)) ;
#85170=DIRECTION('ref_axis',(-1.,8.7378475095785E-80,-2.65552944032596E-32)) ;
#85171=DIRECTION('center_axis',(2.65552944032596E-32,3.29043518662928E-48,
-1.)) ;
#85172=DIRECTION('ref_axis',(-1.,8.7378475095785E-80,-2.65552944032596E-32)) ;
#85173=DIRECTION('center_axis',(-2.65552944032596E-32,-3.29043518662928E-48,
1.)) ;
#85174=DIRECTION('ref_axis',(-1.,8.7378475095785E-80,-2.65552944032596E-32)) ;
#85175=DIRECTION('center_axis',(0.,0.,1.)) ;
#85176=DIRECTION('ref_axis',(1.,0.,0.)) ;
#85177=DIRECTION('center_axis',(0.,0.,-1.)) ;
#85178=DIRECTION('ref_axis',(-1.,0.,0.)) ;
#85179=DIRECTION('center_axis',(0.,0.,1.)) ;
#85180=DIRECTION('ref_axis',(1.,0.,0.)) ;
#85181=DIRECTION('center_axis',(0.,0.,1.)) ;
#85182=DIRECTION('ref_axis',(1.,0.,0.)) ;
#85183=DIRECTION('center_axis',(0.,0.,-1.)) ;
#85184=DIRECTION('ref_axis',(-1.,0.,0.)) ;
#85185=DIRECTION('center_axis',(0.,0.,-1.)) ;
#85186=DIRECTION('ref_axis',(-1.,0.,0.)) ;
#85187=DIRECTION('center_axis',(1.,1.15648231731787E-15,0.)) ;
#85188=DIRECTION('ref_axis',(1.03435541192675E-15,-1.,5.17177705963374E-16)) ;
#85189=DIRECTION('center_axis',(7.089177613099E-16,-0.612994899008946,-0.790086864711098)) ;
#85190=DIRECTION('ref_axis',(-1.7347234759768E-14,-0.790086864711098,0.612994899008946)) ;
#85191=DIRECTION('center_axis',(7.08917761309899E-16,-0.612994899008945,
0.790086864711098)) ;
#85192=DIRECTION('ref_axis',(-3.46944695195361E-14,0.790086864711098,0.612994899008945)) ;
#85193=DIRECTION('center_axis',(0.,0.,-1.)) ;
#85194=DIRECTION('ref_axis',(-1.,0.,0.)) ;
#85195=DIRECTION('center_axis',(0.,0.,1.)) ;
#85196=DIRECTION('ref_axis',(-1.,2.16840434497102E-15,0.)) ;
#85197=DIRECTION('center_axis',(1.08420217248551E-15,-1.,0.)) ;
#85198=DIRECTION('ref_axis',(1.,1.08420217248551E-15,0.)) ;
#85199=DIRECTION('center_axis',(1.44560289664734E-16,-1.,-2.4093381610789E-16)) ;
#85200=DIRECTION('ref_axis',(2.28544744656275E-46,2.4093381610789E-16,-1.)) ;
#85201=DIRECTION('center_axis',(0.,-1.,0.)) ;
#85202=DIRECTION('ref_axis',(0.,0.,-1.)) ;
#85203=DIRECTION('center_axis',(1.,0.,0.)) ;
#85204=DIRECTION('ref_axis',(0.,1.,0.)) ;
#85205=DIRECTION('center_axis',(1.,0.,0.)) ;
#85206=DIRECTION('ref_axis',(0.,0.,-1.)) ;
#85207=DIRECTION('center_axis',(1.,1.23908819712629E-16,8.95614743483648E-33)) ;
#85208=DIRECTION('ref_axis',(-1.23908819712629E-16,1.,-1.10974565782288E-48)) ;
#85209=DIRECTION('center_axis',(1.,0.,0.)) ;
#85210=DIRECTION('ref_axis',(0.,0.,-1.)) ;
#85211=DIRECTION('center_axis',(-1.,0.,0.)) ;
#85212=DIRECTION('ref_axis',(0.,0.,1.)) ;
#85213=DIRECTION('center_axis',(1.,1.23908819712629E-16,8.95614743483648E-33)) ;
#85214=DIRECTION('ref_axis',(-1.23908819712629E-16,1.,-1.10974565782288E-48)) ;
#85215=DIRECTION('center_axis',(-1.,0.,0.)) ;
#85216=DIRECTION('ref_axis',(0.,0.,1.)) ;
#85217=DIRECTION('center_axis',(1.,0.,0.)) ;
#85218=DIRECTION('ref_axis',(0.,-1.,0.)) ;
#85219=DIRECTION('center_axis',(0.,1.,0.)) ;
#85220=DIRECTION('ref_axis',(0.,0.,1.)) ;
#85221=DIRECTION('center_axis',(-1.44560289664734E-16,1.,-7.2280144832367E-17)) ;
#85222=DIRECTION('ref_axis',(0.707106781238328,1.5332934167208E-16,0.707106781134767)) ;
#85223=DIRECTION('center_axis',(-1.0842021724855E-15,1.,0.)) ;
#85224=DIRECTION('ref_axis',(-1.,-1.0842021724855E-15,0.)) ;
#85225=DIRECTION('center_axis',(0.,1.,0.)) ;
#85226=DIRECTION('ref_axis',(0.,0.,1.)) ;
#85227=DIRECTION('center_axis',(0.,-1.,0.)) ;
#85228=DIRECTION('ref_axis',(0.,0.,-1.)) ;
#85229=DIRECTION('center_axis',(0.,1.,0.)) ;
#85230=DIRECTION('ref_axis',(0.,0.,1.)) ;
#85231=DIRECTION('center_axis',(0.,0.,1.)) ;
#85232=DIRECTION('ref_axis',(1.,0.,0.)) ;
#85233=DIRECTION('center_axis',(0.43119164676634,0.0335421424328467,0.901636672080249)) ;
#85234=DIRECTION('ref_axis',(0.899826811350493,0.0573593271358461,-0.432459960187447)) ;
#85235=DIRECTION('center_axis',(0.,0.,1.)) ;
#85236=DIRECTION('ref_axis',(-1.,0.,0.)) ;
#85237=DIRECTION('center_axis',(0.,0.,-1.)) ;
#85238=DIRECTION('ref_axis',(0.707109343403326,-0.707104218960485,0.)) ;
#85239=DIRECTION('center_axis',(-3.25260651745653E-15,0.,1.)) ;
#85240=DIRECTION('ref_axis',(1.,0.,3.25260651745653E-15)) ;
#85241=DIRECTION('center_axis',(0.,0.,1.)) ;
#85242=DIRECTION('ref_axis',(1.,0.,0.)) ;
#85243=DIRECTION('center_axis',(0.431188264321889,0.0335835001222771,-0.901636750155302)) ;
#85244=DIRECTION('ref_axis',(0.899831768148625,0.0572892325239029,0.432458937781775)) ;
#85245=DIRECTION('center_axis',(0.,-1.,0.)) ;
#85246=DIRECTION('ref_axis',(0.,0.,-1.)) ;
#85247=DIRECTION('center_axis',(0.,1.,0.)) ;
#85248=DIRECTION('ref_axis',(0.,0.,1.)) ;
#85249=DIRECTION('center_axis',(0.,0.,1.)) ;
#85250=DIRECTION('ref_axis',(1.,0.,0.)) ;
#85251=DIRECTION('center_axis',(0.,0.,-1.)) ;
#85252=DIRECTION('ref_axis',(-1.,0.,0.)) ;
#85253=DIRECTION('center_axis',(0.,0.,1.)) ;
#85254=DIRECTION('ref_axis',(-0.986393923832144,0.164398987305354,0.)) ;
#85255=DIRECTION('center_axis',(0.98470178743927,-0.164116964573216,0.0585492250433781)) ;
#85256=DIRECTION('ref_axis',(0.164398987305362,0.986393923832143,-7.60669428566932E-17)) ;
#85257=DIRECTION('center_axis',(0.984834538781277,-0.164139089796902,0.0562075655416074)) ;
#85258=DIRECTION('ref_axis',(0.164398987305379,0.98639392383214,1.87706412796466E-17)) ;
#85259=DIRECTION('center_axis',(0.986393923832145,-0.129889480441767,0.100775740620414)) ;
#85260=DIRECTION('ref_axis',(0.,0.612994899008951,0.790086864711094)) ;
#85261=DIRECTION('center_axis',(0.,1.,0.)) ;
#85262=DIRECTION('ref_axis',(1.,0.,0.)) ;
#85263=DIRECTION('center_axis',(0.,0.,-1.)) ;
#85264=DIRECTION('ref_axis',(-1.,0.,0.)) ;
#85265=DIRECTION('center_axis',(1.,2.8359373108165E-15,0.)) ;
#85266=DIRECTION('ref_axis',(-2.8359373108165E-15,1.,0.)) ;
#85267=DIRECTION('center_axis',(0.,0.,-1.)) ;
#85268=DIRECTION('ref_axis',(-1.,0.,0.)) ;
#85269=DIRECTION('center_axis',(0.,0.,1.)) ;
#85270=DIRECTION('ref_axis',(1.,0.,0.)) ;
#85271=DIRECTION('center_axis',(1.,0.,0.)) ;
#85272=DIRECTION('ref_axis',(0.,0.,-1.)) ;
#85273=DIRECTION('center_axis',(1.,0.,0.)) ;
#85274=DIRECTION('ref_axis',(0.,0.,-1.)) ;
#85275=DIRECTION('center_axis',(0.,1.,0.)) ;
#85276=DIRECTION('ref_axis',(1.,0.,0.)) ;
#85277=DIRECTION('center_axis',(1.,-8.50781193244945E-15,0.)) ;
#85278=DIRECTION('ref_axis',(8.50781193244945E-15,1.,0.)) ;
#85279=DIRECTION('center_axis',(0.,1.,0.)) ;
#85280=DIRECTION('ref_axis',(1.,0.,0.)) ;
#85281=DIRECTION('center_axis',(-5.42101086242753E-16,1.70882313734897E-16,
1.)) ;
#85282=DIRECTION('ref_axis',(1.,9.26354878953623E-32,5.42101086242753E-16)) ;
#85283=DIRECTION('center_axis',(-1.,0.,0.)) ;
#85284=DIRECTION('ref_axis',(0.,0.,1.)) ;
#85285=DIRECTION('center_axis',(1.,0.,0.)) ;
#85286=DIRECTION('ref_axis',(0.,0.,-1.)) ;
#85287=DIRECTION('center_axis',(0.,0.,-1.)) ;
#85288=DIRECTION('ref_axis',(-1.,0.,0.)) ;
#85289=DIRECTION('center_axis',(0.,0.,1.)) ;
#85290=DIRECTION('ref_axis',(1.,0.,0.)) ;
#85291=DIRECTION('center_axis',(0.,1.,0.)) ;
#85292=DIRECTION('ref_axis',(1.,0.,0.)) ;
#85293=DIRECTION('center_axis',(0.,1.,0.)) ;
#85294=DIRECTION('ref_axis',(1.,0.,0.)) ;
#85295=DIRECTION('center_axis',(0.,0.,-1.)) ;
#85296=DIRECTION('ref_axis',(-1.,0.,0.)) ;
#85297=DIRECTION('center_axis',(0.,1.,0.)) ;
#85298=DIRECTION('ref_axis',(0.,0.,1.)) ;
#85299=DIRECTION('center_axis',(0.,0.,-1.)) ;
#85300=DIRECTION('ref_axis',(-1.,0.,0.)) ;
#85301=DIRECTION('center_axis',(0.,0.,1.)) ;
#85302=DIRECTION('ref_axis',(1.,0.,0.)) ;
#85303=DIRECTION('center_axis',(1.33440267382831E-16,1.,0.)) ;
#85304=DIRECTION('ref_axis',(-1.,1.33440267382831E-16,0.)) ;
#85305=DIRECTION('center_axis',(0.,1.,0.)) ;
#85306=DIRECTION('ref_axis',(0.,0.,1.)) ;
#85307=DIRECTION('center_axis',(0.,1.,0.)) ;
#85308=DIRECTION('ref_axis',(1.,0.,0.)) ;
#85309=DIRECTION('center_axis',(0.,1.,0.)) ;
#85310=DIRECTION('ref_axis',(0.,0.,1.)) ;
#85311=DIRECTION('center_axis',(0.,1.,0.)) ;
#85312=DIRECTION('ref_axis',(1.,0.,0.)) ;
#85313=DIRECTION('center_axis',(1.37797793267296E-15,-1.62630325872825E-15,
1.)) ;
#85314=DIRECTION('ref_axis',(-2.24101000236165E-30,-1.,-1.62630325872825E-15)) ;
#85315=DIRECTION('center_axis',(-1.33440267382831E-16,-1.,0.)) ;
#85316=DIRECTION('ref_axis',(1.,-1.33440267382831E-16,0.)) ;
#85317=DIRECTION('center_axis',(0.,1.,0.)) ;
#85318=DIRECTION('ref_axis',(0.,0.,1.)) ;
#85319=DIRECTION('center_axis',(0.,0.,-1.)) ;
#85320=DIRECTION('ref_axis',(-1.,0.,0.)) ;
#85321=DIRECTION('center_axis',(0.,0.,1.)) ;
#85322=DIRECTION('ref_axis',(1.,0.,0.)) ;
#85323=DIRECTION('center_axis',(0.,1.,0.)) ;
#85324=DIRECTION('ref_axis',(1.,0.,0.)) ;
#85325=DIRECTION('center_axis',(0.,0.,1.)) ;
#85326=DIRECTION('ref_axis',(1.,0.,0.)) ;
#85327=DIRECTION('center_axis',(0.,0.,1.)) ;
#85328=DIRECTION('ref_axis',(1.,0.,0.)) ;
#85329=DIRECTION('center_axis',(0.,0.,1.)) ;
#85330=DIRECTION('ref_axis',(-0.986393923832144,0.164398987305354,0.)) ;
#85331=DIRECTION('center_axis',(0.984701787439272,-0.164116964573205,-0.0585492250433871)) ;
#85332=DIRECTION('ref_axis',(0.16439898730535,0.986393923832145,-3.2807868055655E-16)) ;
#85333=DIRECTION('center_axis',(0.984834538781259,-0.164139089796881,-0.0562075655419907)) ;
#85334=DIRECTION('ref_axis',(0.164398987305362,0.986393923832143,6.03508511856301E-17)) ;
#85335=DIRECTION('center_axis',(0.,0.,1.)) ;
#85336=DIRECTION('ref_axis',(-0.986393923832144,0.164398987305354,0.)) ;
#85337=DIRECTION('center_axis',(0.,0.,1.)) ;
#85338=DIRECTION('ref_axis',(1.,0.,0.)) ;
#85339=DIRECTION('center_axis',(0.342346838787153,0.100237737284617,-0.934211452507677)) ;
#85340=DIRECTION('ref_axis',(0.878411919475056,0.318727606806516,0.356097195135737)) ;
#85341=DIRECTION('center_axis',(0.,0.,-1.)) ;
#85342=DIRECTION('ref_axis',(-1.,0.,0.)) ;
#85343=DIRECTION('center_axis',(0.,0.,-1.)) ;
#85344=DIRECTION('ref_axis',(-1.,0.,0.)) ;
#85345=DIRECTION('center_axis',(0.,0.,-1.)) ;
#85346=DIRECTION('ref_axis',(-1.,0.,0.)) ;
#85347=DIRECTION('center_axis',(-0.34234683878929,-0.100237737302457,-0.93421145250498)) ;
#85348=DIRECTION('ref_axis',(0.878411847182506,0.318727811137727,-0.356097190576915)) ;
#85349=DIRECTION('center_axis',(0.,0.,1.)) ;
#85350=DIRECTION('ref_axis',(1.,0.,0.)) ;
#85351=DIRECTION('center_axis',(0.967224433215112,0.251696851080207,0.0335498278387964)) ;
#85352=DIRECTION('ref_axis',(0.148186147792394,-0.666803866446761,0.730351606621154)) ;
#85353=DIRECTION('center_axis',(0.,0.707106781186549,-0.707106781186547)) ;
#85354=DIRECTION('ref_axis',(0.,0.707106781186546,0.707106781186549)) ;
#85355=DIRECTION('center_axis',(0.978007532938648,-0.147978541149372,-0.146981688909074)) ;
#85356=DIRECTION('ref_axis',(0.193734423938021,0.383507624685324,0.9029888564039)) ;
#85357=DIRECTION('center_axis',(0.,0.447213595499958,0.894427190999916)) ;
#85358=DIRECTION('ref_axis',(0.,-0.894427190999916,0.447213595499958)) ;
#85359=DIRECTION('center_axis',(0.960001452008207,0.250435160947592,-0.125217579849191)) ;
#85360=DIRECTION('ref_axis',(0.276742394167975,-0.916645079797593,0.28840153424183)) ;
#85361=DIRECTION('center_axis',(0.,1.,0.)) ;
#85362=DIRECTION('ref_axis',(0.,0.,1.)) ;
#85363=DIRECTION('center_axis',(-1.,0.,0.)) ;
#85364=DIRECTION('ref_axis',(0.,0.41390516857167,-0.910320004959606)) ;
#85365=DIRECTION('center_axis',(1.,1.44560289664734E-16,0.)) ;
#85366=DIRECTION('ref_axis',(0.,1.,0.)) ;
#85367=DIRECTION('center_axis',(1.,1.44560289664734E-16,0.)) ;
#85368=DIRECTION('ref_axis',(-1.44560289664734E-16,1.,0.)) ;
#85369=DIRECTION('center_axis',(0.,0.,-1.)) ;
#85370=DIRECTION('ref_axis',(0.,-1.,0.)) ;
#85371=DIRECTION('center_axis',(-1.,-1.44560289664734E-16,0.)) ;
#85372=DIRECTION('ref_axis',(-1.44560289664734E-16,1.,0.)) ;
#85373=DIRECTION('center_axis',(1.,-3.46944695195361E-16,0.)) ;
#85374=DIRECTION('ref_axis',(2.61228946970625E-16,1.,0.)) ;
#85375=DIRECTION('center_axis',(1.,-3.46944695195361E-16,0.)) ;
#85376=DIRECTION('ref_axis',(3.46944695195361E-16,1.,0.)) ;
#85377=DIRECTION('center_axis',(0.,0.,1.)) ;
#85378=DIRECTION('ref_axis',(-3.26536183713281E-16,-1.,0.)) ;
#85379=DIRECTION('center_axis',(-1.,3.46944695195361E-16,0.)) ;
#85380=DIRECTION('ref_axis',(3.46944695195361E-16,1.,0.)) ;
#85381=DIRECTION('center_axis',(-1.,3.46944695195361E-16,0.)) ;
#85382=DIRECTION('ref_axis',(-3.46944695195361E-16,-1.,0.)) ;
#85383=DIRECTION('center_axis',(-1.,0.,0.)) ;
#85384=DIRECTION('ref_axis',(0.,0.,1.)) ;
#85385=DIRECTION('',(1.,-3.46944695195361E-16,0.)) ;
#85386=DIRECTION('center_axis',(-1.,8.01625584951926E-16,-1.08420217248551E-15)) ;
#85387=DIRECTION('ref_axis',(1.08420217248552E-15,6.50521303491307E-15,
-1.)) ;
#85388=DIRECTION('center_axis',(-1.,8.01625584951926E-16,-1.08420217248551E-15)) ;
#85389=DIRECTION('ref_axis',(1.08420217248552E-15,6.50521303491307E-15,
-1.)) ;
#85390=DIRECTION('',(-1.,3.46944695195361E-16,0.)) ;
#85391=DIRECTION('center_axis',(-1.,3.46944695195361E-16,0.)) ;
#85392=DIRECTION('ref_axis',(-3.46944695195361E-16,-1.,0.)) ;
#85393=DIRECTION('center_axis',(-1.,0.,0.)) ;
#85394=DIRECTION('ref_axis',(0.,0.,1.)) ;
#85395=DIRECTION('',(1.,-3.46944695195361E-16,0.)) ;
#85396=DIRECTION('center_axis',(-1.,2.2680138501079E-15,0.)) ;
#85397=DIRECTION('ref_axis',(2.2680138501079E-15,1.,0.)) ;
#85398=DIRECTION('',(-1.,3.46944695195361E-16,0.)) ;
#85399=DIRECTION('center_axis',(-1.,3.18032637262401E-16,0.)) ;
#85400=DIRECTION('ref_axis',(-5.55111512312578E-16,-1.,0.)) ;
#85401=DIRECTION('center_axis',(1.,-3.18032637262401E-16,0.)) ;
#85402=DIRECTION('ref_axis',(-3.18032637262401E-16,-1.,0.)) ;
#85403=DIRECTION('center_axis',(-2.01298417874256E-16,-0.632948931301568,
-0.774193548387096)) ;
#85404=DIRECTION('ref_axis',(-1.73472347597679E-14,-0.774193548387096,0.632948931301568)) ;
#85405=DIRECTION('center_axis',(-1.,3.18032637262401E-16,0.)) ;
#85406=DIRECTION('ref_axis',(-3.18032637262401E-16,-1.,0.)) ;
#85407=DIRECTION('center_axis',(-2.01298417874256E-16,-0.632948931301568,
0.774193548387096)) ;
#85408=DIRECTION('ref_axis',(-2.5982535921668E-30,-0.774193548387096,-0.632948931301568)) ;
#85409=DIRECTION('center_axis',(1.,1.44560289664734E-16,0.)) ;
#85410=DIRECTION('ref_axis',(-1.44560289664734E-16,1.,0.)) ;
#85411=DIRECTION('',(-1.,-1.44560289664734E-16,0.)) ;
#85412=DIRECTION('center_axis',(-1.,3.46944695195361E-16,0.)) ;
#85413=DIRECTION('ref_axis',(-3.46944695195361E-16,-1.,0.)) ;
#85414=DIRECTION('',(-1.,3.46944695195361E-16,0.)) ;
#85415=DIRECTION('center_axis',(-1.,3.46944695195361E-16,0.)) ;
#85416=DIRECTION('ref_axis',(3.46944695195361E-16,1.,0.)) ;
#85417=DIRECTION('center_axis',(-1.,3.46944695195361E-16,0.)) ;
#85418=DIRECTION('ref_axis',(3.46944695195361E-16,1.,0.)) ;
#85419=DIRECTION('center_axis',(-1.,3.46944695195361E-16,0.)) ;
#85420=DIRECTION('ref_axis',(-3.46944695195361E-16,-1.,0.)) ;
#85421=DIRECTION('',(1.,-3.46944695195361E-16,0.)) ;
#85422=DIRECTION('center_axis',(-1.,-1.44560289664734E-16,-2.65552944032596E-32)) ;
#85423=DIRECTION('ref_axis',(1.44560289664734E-16,-1.,-2.80018320648271E-64)) ;
#85424=DIRECTION('',(2.65552944032596E-32,3.29043518662928E-48,-1.)) ;
#85425=DIRECTION('',(1.44560289664734E-16,-1.,-2.4093381610789E-16)) ;
#85426=DIRECTION('',(0.,0.,1.)) ;
#85427=DIRECTION('center_axis',(0.999999956301289,0.000282786981350015,
8.61913163546712E-5)) ;
#85428=DIRECTION('ref_axis',(0.000288266391185019,-0.997396273404882,-0.0721151211643056)) ;
#85429=DIRECTION('',(-1.44560289664734E-16,1.,-7.2280144832367E-17)) ;
#85430=DIRECTION('center_axis',(0.316227766016838,0.948683298050514,0.)) ;
#85431=DIRECTION('ref_axis',(-0.948683298050514,0.316227766016838,0.)) ;
#85432=DIRECTION('',(-0.948683298050514,0.316227766016838,0.)) ;
#85433=DIRECTION('',(0.,0.,1.)) ;
#85434=DIRECTION('',(0.937042571331636,-0.312347523777212,-0.156173761888606)) ;
#85435=DIRECTION('',(0.,0.,-1.)) ;
#85436=DIRECTION('center_axis',(1.,1.73472347597681E-15,0.)) ;
#85437=DIRECTION('ref_axis',(-1.73472347597681E-15,1.,0.)) ;
#85438=DIRECTION('',(-1.73472347597681E-15,1.,0.)) ;
#85439=DIRECTION('',(0.,0.,1.)) ;
#85440=DIRECTION('',(1.73472347597681E-15,-1.,-2.89120579329468E-16)) ;
#85441=DIRECTION('',(0.,0.,-1.)) ;
#85442=DIRECTION('center_axis',(0.164398987305357,-0.986393923832144,0.)) ;
#85443=DIRECTION('ref_axis',(0.986393923832144,0.164398987305357,0.)) ;
#85444=DIRECTION('',(-0.973328526784575,-0.162221421130762,0.162221421130763)) ;
#85445=DIRECTION('',(0.,0.,-1.)) ;
#85446=DIRECTION('',(0.986393923832144,0.164398987305357,0.)) ;
#85447=DIRECTION('',(0.,0.,1.)) ;
#85448=DIRECTION('center_axis',(-9.91270557701033E-17,1.,0.)) ;
#85449=DIRECTION('ref_axis',(-1.,-9.91270557701033E-17,0.)) ;
#85450=DIRECTION('',(1.,9.91270557701033E-17,0.)) ;
#85451=DIRECTION('',(0.,0.,-1.)) ;
#85452=DIRECTION('',(-1.,-9.91270557701033E-17,0.)) ;
#85453=DIRECTION('',(0.,0.,1.)) ;
#85454=DIRECTION('center_axis',(-9.91270557701033E-17,1.,0.)) ;
#85455=DIRECTION('ref_axis',(-1.,-9.91270557701033E-17,0.)) ;
#85456=DIRECTION('',(-1.,-9.91270557701033E-17,0.)) ;
#85457=DIRECTION('',(0.,0.,-1.)) ;
#85458=DIRECTION('',(-1.,-9.91270557701033E-17,0.)) ;
#85459=DIRECTION('',(0.,0.,1.)) ;
#85460=DIRECTION('center_axis',(1.,1.15648231731787E-15,0.)) ;
#85461=DIRECTION('ref_axis',(-1.15648231731787E-15,1.,0.)) ;
#85462=DIRECTION('',(-1.15648231731787E-15,1.,0.)) ;
#85463=DIRECTION('',(0.,0.,-1.)) ;
#85464=DIRECTION('',(-1.15648231731787E-15,1.,0.)) ;
#85465=DIRECTION('',(0.,0.,1.)) ;
#85466=DIRECTION('center_axis',(-1.,-1.15648231731787E-15,0.)) ;
#85467=DIRECTION('ref_axis',(-1.15648231731787E-15,1.,0.)) ;
#85468=DIRECTION('',(0.,0.,1.)) ;
#85469=DIRECTION('center_axis',(0.,0.,1.)) ;
#85470=DIRECTION('ref_axis',(1.,0.,0.)) ;
#85471=DIRECTION('',(-1.,0.,0.)) ;
#85472=DIRECTION('center_axis',(0.,0.,-1.)) ;
#85473=DIRECTION('ref_axis',(1.,0.,0.)) ;
#85474=DIRECTION('center_axis',(0.,0.,-1.)) ;
#85475=DIRECTION('ref_axis',(1.,0.,0.)) ;
#85476=DIRECTION('center_axis',(0.,0.,-1.)) ;
#85477=DIRECTION('ref_axis',(1.,0.,0.)) ;
#85478=DIRECTION('center_axis',(0.,0.,-1.)) ;
#85479=DIRECTION('ref_axis',(1.,0.,0.)) ;
#85480=DIRECTION('',(1.,0.,0.)) ;
#85481=DIRECTION('center_axis',(0.,0.,1.)) ;
#85482=DIRECTION('ref_axis',(1.,0.,0.)) ;
#85483=DIRECTION('',(3.46944695195361E-16,1.,0.)) ;
#85484=DIRECTION('center_axis',(0.,0.,1.)) ;
#85485=DIRECTION('ref_axis',(1.,0.,0.)) ;
#85486=DIRECTION('',(1.,-3.46944695195361E-16,0.)) ;
#85487=DIRECTION('center_axis',(0.,0.,-1.)) ;
#85488=DIRECTION('ref_axis',(1.,0.,0.)) ;
#85489=DIRECTION('',(2.71050543121376E-16,1.,0.)) ;
#85490=DIRECTION('center_axis',(0.,0.,-1.)) ;
#85491=DIRECTION('ref_axis',(1.,0.,0.)) ;
#85492=DIRECTION('',(-1.,3.46944695195361E-16,0.)) ;
#85493=DIRECTION('center_axis',(0.,0.,1.)) ;
#85494=DIRECTION('ref_axis',(1.,0.,0.)) ;
#85495=DIRECTION('',(3.46944695195361E-16,1.,0.)) ;
#85496=DIRECTION('center_axis',(0.,0.,1.)) ;
#85497=DIRECTION('ref_axis',(1.,0.,0.)) ;
#85498=DIRECTION('center_axis',(0.,0.,-1.)) ;
#85499=DIRECTION('ref_axis',(1.,0.,0.)) ;
#85500=DIRECTION('',(0.986393923832144,-0.164398987305354,0.)) ;
#85501=DIRECTION('center_axis',(0.,0.,-1.)) ;
#85502=DIRECTION('ref_axis',(1.,-6.50521303491307E-15,0.)) ;
#85503=DIRECTION('center_axis',(0.,0.,-1.)) ;
#85504=DIRECTION('ref_axis',(1.,0.,0.)) ;
#85505=DIRECTION('',(1.,0.,0.)) ;
#85506=DIRECTION('',(1.13380619344889E-16,-1.,0.)) ;
#85507=DIRECTION('center_axis',(0.,0.,-1.)) ;
#85508=DIRECTION('ref_axis',(1.,0.,0.)) ;
#85509=DIRECTION('',(-1.,-1.92747052886312E-16,0.)) ;
#85510=DIRECTION('center_axis',(0.,0.,1.)) ;
#85511=DIRECTION('ref_axis',(1.,0.,0.)) ;
#85512=DIRECTION('',(0.,-1.,0.)) ;
#85513=DIRECTION('center_axis',(0.,0.,-1.)) ;
#85514=DIRECTION('ref_axis',(1.,0.,0.)) ;
#85515=DIRECTION('center_axis',(0.,0.,1.)) ;
#85516=DIRECTION('ref_axis',(1.,0.,0.)) ;
#85517=DIRECTION('',(-0.948683298050514,0.316227766016838,0.)) ;
#85518=DIRECTION('center_axis',(0.,0.,1.)) ;
#85519=DIRECTION('ref_axis',(1.,0.,0.)) ;
#85520=DIRECTION('',(-1.,0.,0.)) ;
#85521=DIRECTION('center_axis',(0.,0.,1.)) ;
#85522=DIRECTION('ref_axis',(1.,0.,0.)) ;
#85523=DIRECTION('',(0.,-1.,0.)) ;
#85524=DIRECTION('center_axis',(0.,0.,-1.)) ;
#85525=DIRECTION('ref_axis',(1.,0.,0.)) ;
#85526=DIRECTION('',(-1.,-1.92747052886312E-16,0.)) ;
#85527=DIRECTION('center_axis',(0.,0.,1.)) ;
#85528=DIRECTION('ref_axis',(1.,0.,0.)) ;
#85529=DIRECTION('',(1.13380619344889E-16,-1.,0.)) ;
#85530=DIRECTION('',(1.,0.,0.)) ;
#85531=DIRECTION('center_axis',(0.,0.,1.)) ;
#85532=DIRECTION('ref_axis',(1.,0.,0.)) ;
#85533=DIRECTION('center_axis',(0.,0.,1.)) ;
#85534=DIRECTION('ref_axis',(1.,0.,0.)) ;
#85535=DIRECTION('',(-0.986393923832144,0.164398987305354,0.)) ;
#85536=DIRECTION('center_axis',(0.,0.,1.)) ;
#85537=DIRECTION('ref_axis',(1.,0.,0.)) ;
#85538=DIRECTION('center_axis',(0.,0.,-1.)) ;
#85539=DIRECTION('ref_axis',(1.,0.,0.)) ;
#85540=DIRECTION('',(-3.46944695195361E-16,-1.,0.)) ;
#85541=DIRECTION('center_axis',(0.,0.,-1.)) ;
#85542=DIRECTION('ref_axis',(1.,0.,0.)) ;
#85543=DIRECTION('',(-1.,3.46944695195361E-16,0.)) ;
#85544=DIRECTION('center_axis',(0.,0.,1.)) ;
#85545=DIRECTION('ref_axis',(1.,0.,0.)) ;
#85546=DIRECTION('',(3.46944695195361E-16,1.,0.)) ;
#85547=DIRECTION('center_axis',(0.,0.,1.)) ;
#85548=DIRECTION('ref_axis',(1.,0.,0.)) ;
#85549=DIRECTION('',(1.,-3.46944695195361E-16,0.)) ;
#85550=DIRECTION('center_axis',(0.,0.,-1.)) ;
#85551=DIRECTION('ref_axis',(1.,0.,0.)) ;
#85552=DIRECTION('',(-3.46944695195361E-16,-1.,0.)) ;
#85553=DIRECTION('center_axis',(0.,0.,-1.)) ;
#85554=DIRECTION('ref_axis',(1.,0.,0.)) ;
#85555=DIRECTION('',(1.,0.,0.)) ;
#85556=DIRECTION('center_axis',(0.,0.,1.)) ;
#85557=DIRECTION('ref_axis',(1.,0.,0.)) ;
#85558=DIRECTION('',(0.986393923832144,0.164398987305357,0.)) ;
#85559=DIRECTION('center_axis',(0.,0.,1.)) ;
#85560=DIRECTION('ref_axis',(1.,0.,0.)) ;
#85561=DIRECTION('',(-1.73472347597681E-15,1.,0.)) ;
#85562=DIRECTION('center_axis',(0.,0.,1.)) ;
#85563=DIRECTION('ref_axis',(1.,0.,0.)) ;
#85564=DIRECTION('center_axis',(-1.92747052886312E-16,1.,0.)) ;
#85565=DIRECTION('ref_axis',(-1.,-1.92747052886312E-16,0.)) ;
#85566=DIRECTION('',(0.,0.,1.)) ;
#85567=DIRECTION('',(0.,0.,-1.)) ;
#85568=DIRECTION('center_axis',(-1.,0.,0.)) ;
#85569=DIRECTION('ref_axis',(0.,0.,1.)) ;
#85570=DIRECTION('',(0.,0.,1.)) ;
#85571=DIRECTION('',(0.,0.,-1.)) ;
#85572=DIRECTION('center_axis',(0.,1.,0.)) ;
#85573=DIRECTION('ref_axis',(0.,0.,1.)) ;
#85574=DIRECTION('',(0.,0.,-1.)) ;
#85575=DIRECTION('',(0.,0.,1.)) ;
#85576=DIRECTION('',(0.,0.,-1.)) ;
#85577=DIRECTION('',(0.,0.,-1.)) ;
#85578=DIRECTION('center_axis',(0.316227766016838,0.948683298050514,0.)) ;
#85579=DIRECTION('ref_axis',(-0.948683298050514,0.316227766016838,0.)) ;
#85580=DIRECTION('center_axis',(-0.316227766016838,-0.948683298050514,0.)) ;
#85581=DIRECTION('ref_axis',(0.83159596074681,-0.27719865358227,-0.481257794245212)) ;
#85582=DIRECTION('',(0.,0.,1.)) ;
#85583=DIRECTION('',(0.,0.,-1.)) ;
#85584=DIRECTION('',(-0.937042571331636,0.312347523777212,-0.156173761888606)) ;
#85585=DIRECTION('center_axis',(1.,1.73472347597681E-15,0.)) ;
#85586=DIRECTION('ref_axis',(-1.73472347597681E-15,1.,0.)) ;
#85587=DIRECTION('',(-1.73472347597681E-15,1.,-2.89120579329468E-16)) ;
#85588=DIRECTION('',(0.,0.,1.)) ;
#85589=DIRECTION('',(0.,0.,-1.)) ;
#85590=DIRECTION('center_axis',(0.164398987305357,-0.986393923832144,0.)) ;
#85591=DIRECTION('ref_axis',(0.986393923832144,0.164398987305357,0.)) ;
#85592=DIRECTION('',(0.973328526784575,0.162221421130762,0.162221421130763)) ;
#85593=DIRECTION('',(0.,0.,1.)) ;
#85594=DIRECTION('',(0.,0.,-1.)) ;
#85595=DIRECTION('center_axis',(0.,-1.,0.)) ;
#85596=DIRECTION('ref_axis',(0.,0.,-1.)) ;
#85597=DIRECTION('',(0.,0.,1.)) ;
#85598=DIRECTION('',(0.,0.,1.)) ;
#85599=DIRECTION('',(0.,0.,1.)) ;
#85600=DIRECTION('',(0.,0.,-1.)) ;
#85601=DIRECTION('',(1.,0.,2.25271179641597E-31)) ;
#85602=DIRECTION('center_axis',(0.,-1.,0.)) ;
#85603=DIRECTION('ref_axis',(0.,0.,-1.)) ;
#85604=DIRECTION('',(0.,0.,-1.)) ;
#85605=DIRECTION('center_axis',(0.,-1.,0.)) ;
#85606=DIRECTION('ref_axis',(0.,0.,-1.)) ;
#85607=DIRECTION('',(-1.,0.,-3.21815970916568E-32)) ;
#85608=DIRECTION('',(0.,0.,-1.)) ;
#85609=DIRECTION('center_axis',(1.,-3.46944695195361E-16,0.)) ;
#85610=DIRECTION('ref_axis',(3.46944695195361E-16,1.,0.)) ;
#85611=DIRECTION('center_axis',(1.,-3.46944695195361E-16,0.)) ;
#85612=DIRECTION('ref_axis',(3.46944695195361E-16,1.,0.)) ;
#85613=DIRECTION('',(1.5529910948782E-31,4.47619207437002E-16,-1.)) ;
#85614=DIRECTION('',(0.,0.,1.)) ;
#85615=DIRECTION('center_axis',(1.,-3.46944695195361E-16,0.)) ;
#85616=DIRECTION('ref_axis',(3.46944695195361E-16,1.,0.)) ;
#85617=DIRECTION('center_axis',(1.,-3.46944695195361E-16,0.)) ;
#85618=DIRECTION('ref_axis',(3.46944695195361E-16,1.,0.)) ;
#85619=DIRECTION('center_axis',(1.,-3.46944695195361E-16,0.)) ;
#85620=DIRECTION('ref_axis',(3.46944695195361E-16,1.,0.)) ;
#85621=DIRECTION('',(3.46944695195361E-16,1.,9.27571383489107E-17)) ;
#85622=DIRECTION('',(0.,0.,1.)) ;
#85623=DIRECTION('',(-3.46944695195361E-16,-1.,-6.49299968442375E-16)) ;
#85624=DIRECTION('center_axis',(1.,-3.46944695195361E-16,0.)) ;
#85625=DIRECTION('ref_axis',(3.46944695195361E-16,1.,0.)) ;
#85626=DIRECTION('center_axis',(1.,-3.46944695195361E-16,0.)) ;
#85627=DIRECTION('ref_axis',(3.46944695195361E-16,1.,0.)) ;
#85628=DIRECTION('center_axis',(1.,-3.46944695195361E-16,0.)) ;
#85629=DIRECTION('ref_axis',(3.46944695195361E-16,1.,0.)) ;
#85630=DIRECTION('',(0.,0.,1.)) ;
#85631=DIRECTION('',(-1.5529910948782E-31,-4.47619207437002E-16,-1.)) ;
#85632=DIRECTION('center_axis',(1.,-3.46944695195361E-16,0.)) ;
#85633=DIRECTION('ref_axis',(3.46944695195361E-16,1.,0.)) ;
#85634=DIRECTION('center_axis',(1.,-3.46944695195361E-16,0.)) ;
#85635=DIRECTION('ref_axis',(3.46944695195361E-16,1.,0.)) ;
#85636=DIRECTION('center_axis',(1.,-3.46944695195361E-16,0.)) ;
#85637=DIRECTION('ref_axis',(3.46944695195361E-16,1.,0.)) ;
#85638=DIRECTION('',(-3.46944695195361E-16,-1.,-1.06487173641454E-15)) ;
#85639=DIRECTION('center_axis',(1.,-3.46944695195361E-16,0.)) ;
#85640=DIRECTION('ref_axis',(3.46944695195361E-16,1.,0.)) ;
#85641=DIRECTION('',(3.46944695195361E-16,1.,2.45739631480277E-16)) ;
#85642=DIRECTION('center_axis',(1.,-3.46944695195361E-16,0.)) ;
#85643=DIRECTION('ref_axis',(3.46944695195361E-16,1.,0.)) ;
#85644=DIRECTION('center_axis',(1.,-3.46944695195361E-16,0.)) ;
#85645=DIRECTION('ref_axis',(3.46944695195361E-16,1.,0.)) ;
#85646=DIRECTION('center_axis',(0.,-1.,0.)) ;
#85647=DIRECTION('ref_axis',(0.,0.,-1.)) ;
#85648=DIRECTION('center_axis',(0.,-1.,0.)) ;
#85649=DIRECTION('ref_axis',(0.,0.,-1.)) ;
#85650=DIRECTION('',(-1.,0.,-1.40488587213121E-32)) ;
#85651=DIRECTION('',(0.,0.,1.)) ;
#85652=DIRECTION('',(0.,0.,1.)) ;
#85653=DIRECTION('',(0.,0.,1.)) ;
#85654=DIRECTION('',(1.,0.,1.40488587213121E-32)) ;
#85655=DIRECTION('center_axis',(0.,-1.,0.)) ;
#85656=DIRECTION('ref_axis',(0.,0.,-1.)) ;
#85657=DIRECTION('',(7.2280144832367E-17,0.,-1.)) ;
#85658=DIRECTION('center_axis',(-1.,-1.13380619344889E-16,0.)) ;
#85659=DIRECTION('ref_axis',(1.13380619344889E-16,-1.,0.)) ;
#85660=DIRECTION('center_axis',(-1.,-1.13380619344889E-16,0.)) ;
#85661=DIRECTION('ref_axis',(1.13380619344889E-16,-1.,0.)) ;
#85662=DIRECTION('',(1.13380619344889E-16,-1.,1.23908819712629E-16)) ;
#85663=DIRECTION('',(0.,0.,-1.)) ;
#85664=DIRECTION('',(-1.13380619344889E-16,1.,-1.23908819712629E-16)) ;
#85665=DIRECTION('center_axis',(-1.,-1.13380619344889E-16,0.)) ;
#85666=DIRECTION('ref_axis',(1.13380619344889E-16,-1.,0.)) ;
#85667=DIRECTION('',(0.,0.,1.)) ;
#85668=DIRECTION('center_axis',(-1.40488587213121E-32,1.23908819712629E-16,
1.)) ;
#85669=DIRECTION('ref_axis',(0.,-1.,1.23908819712629E-16)) ;
#85670=DIRECTION('',(-1.,0.,-1.40488587213121E-32)) ;
#85671=DIRECTION('',(-1.13380619344889E-16,1.,-1.23908819712629E-16)) ;
#85672=DIRECTION('center_axis',(1.40488587213121E-32,-1.23908819712629E-16,
-1.)) ;
#85673=DIRECTION('ref_axis',(-1.74077750246726E-48,-1.,1.23908819712629E-16)) ;
#85674=DIRECTION('center_axis',(1.40488587213121E-32,-1.23908819712629E-16,
-1.)) ;
#85675=DIRECTION('ref_axis',(0.,1.,-1.23908819712629E-16)) ;
#85676=DIRECTION('center_axis',(-1.40488587213121E-32,1.23908819712629E-16,
1.)) ;
#85677=DIRECTION('ref_axis',(1.74077750246726E-48,1.,-1.23908819712629E-16)) ;
#85678=DIRECTION('',(1.13380619344889E-16,-1.,1.23908819712629E-16)) ;
#85679=DIRECTION('',(1.,0.,1.40488587213121E-32)) ;
#85680=DIRECTION('center_axis',(-1.,-1.23908819712629E-16,-8.95614743483648E-33)) ;
#85681=DIRECTION('ref_axis',(1.23908819712629E-16,-1.,5.38566640001825E-66)) ;
#85682=DIRECTION('',(-8.95614743483648E-33,-1.10974565782288E-48,1.)) ;
#85683=DIRECTION('',(1.23908819712629E-16,-1.,7.2280144832367E-17)) ;
#85684=DIRECTION('',(-8.95614743483648E-33,0.,1.)) ;
#85685=DIRECTION('',(-1.23908819712629E-16,1.,-1.23908819712629E-16)) ;
#85686=DIRECTION('',(8.95614743483648E-33,1.0154535431059E-48,-1.)) ;
#85687=DIRECTION('',(1.23908819712629E-16,-1.,1.23908819712629E-16)) ;
#85688=DIRECTION('',(-8.95614743483648E-33,0.,1.)) ;
#85689=DIRECTION('',(-1.23908819712629E-16,1.,2.4093381610789E-16)) ;
#85690=DIRECTION('center_axis',(-1.7912294869673E-32,7.2280144832367E-17,
1.)) ;
#85691=DIRECTION('ref_axis',(0.,-1.,7.2280144832367E-17)) ;
#85692=DIRECTION('',(-1.23908819712629E-16,1.,-7.2280144832367E-17)) ;
#85693=DIRECTION('',(1.,1.23908819712629E-16,8.95614743483648E-33)) ;
#85694=DIRECTION('',(1.44560289664734E-16,-1.,7.2280144832367E-17)) ;
#85695=DIRECTION('',(-1.,0.,-1.7912294869673E-32)) ;
#85696=DIRECTION('center_axis',(-2.08976773479518E-32,2.4093381610789E-16,
-1.)) ;
#85697=DIRECTION('ref_axis',(0.,1.,2.4093381610789E-16)) ;
#85698=DIRECTION('',(-1.44560289664734E-16,1.,2.4093381610789E-16)) ;
#85699=DIRECTION('',(-1.,-1.23908819712629E-16,-8.95614743483648E-33)) ;
#85700=DIRECTION('',(1.23908819712629E-16,-1.,-2.4093381610789E-16)) ;
#85701=DIRECTION('',(1.,0.,-2.08976773479518E-32)) ;
#85702=DIRECTION('center_axis',(-1.23908819712629E-16,1.,0.)) ;
#85703=DIRECTION('ref_axis',(-1.,-1.23908819712629E-16,0.)) ;
#85704=DIRECTION('',(8.95614743483648E-33,1.10974565782288E-48,-1.)) ;
#85705=DIRECTION('',(1.,1.23908819712629E-16,8.95614743483648E-33)) ;
#85706=DIRECTION('',(-2.65552944032596E-32,-3.29043518662928E-48,1.)) ;
#85707=DIRECTION('',(-1.,-1.23908819712629E-16,-8.95614743483648E-33)) ;
#85708=DIRECTION('center_axis',(-1.,-1.44560289664734E-16,-2.65552944032596E-32)) ;
#85709=DIRECTION('ref_axis',(1.44560289664734E-16,-1.,-2.80018320648271E-64)) ;
#85710=DIRECTION('',(1.44560289664734E-16,-1.,-2.4093381610789E-16)) ;
#85711=DIRECTION('',(-2.65552944032596E-32,0.,1.)) ;
#85712=DIRECTION('',(-1.44560289664734E-16,1.,-7.2280144832367E-17)) ;
#85713=DIRECTION('',(0.,0.,-1.)) ;
#85714=DIRECTION('center_axis',(0.,1.,0.)) ;
#85715=DIRECTION('ref_axis',(0.,0.,1.)) ;
#85716=DIRECTION('',(8.95614743483648E-33,0.,-1.)) ;
#85717=DIRECTION('',(1.,0.,1.40488587213121E-32)) ;
#85718=DIRECTION('',(-7.2280144832367E-17,0.,1.)) ;
#85719=DIRECTION('',(-1.,0.,-1.40488587213121E-32)) ;
#85720=DIRECTION('',(8.95614743483648E-33,0.,-1.)) ;
#85721=DIRECTION('',(1.,0.,1.7912294869673E-32)) ;
#85722=DIRECTION('',(2.65552944032596E-32,0.,-1.)) ;
#85723=DIRECTION('',(-1.,0.,2.08976773479518E-32)) ;
#85724=DIRECTION('center_axis',(1.,1.44560289664734E-16,0.)) ;
#85725=DIRECTION('ref_axis',(-1.44560289664734E-16,1.,0.)) ;
#85726=DIRECTION('',(1.44560289664734E-16,-1.,0.)) ;
#85727=DIRECTION('center_axis',(-1.,-1.44560289664734E-16,0.)) ;
#85728=DIRECTION('ref_axis',(-1.44560289664734E-16,1.,0.)) ;
#85729=DIRECTION('',(0.,0.,-1.)) ;
#85730=DIRECTION('center_axis',(-1.,-1.44560289664734E-16,0.)) ;
#85731=DIRECTION('ref_axis',(-1.44560289664734E-16,1.,0.)) ;
#85732=DIRECTION('',(1.44560289664734E-16,-1.,0.)) ;
#85733=DIRECTION('center_axis',(-1.,-1.44560289664734E-16,0.)) ;
#85734=DIRECTION('ref_axis',(-1.44560289664734E-16,1.,0.)) ;
#85735=DIRECTION('',(0.,0.,1.)) ;
#85736=DIRECTION('center_axis',(-1.,-1.44560289664734E-16,0.)) ;
#85737=DIRECTION('ref_axis',(-1.44560289664734E-16,1.,0.)) ;
#85738=DIRECTION('center_axis',(1.,-3.46944695195361E-16,0.)) ;
#85739=DIRECTION('ref_axis',(3.46944695195361E-16,1.,0.)) ;
#85740=DIRECTION('center_axis',(1.,-3.46944695195361E-16,0.)) ;
#85741=DIRECTION('ref_axis',(3.46944695195361E-16,1.,0.)) ;
#85742=DIRECTION('',(0.,0.,-1.)) ;
#85743=DIRECTION('',(-1.5529910948782E-31,-4.47619207437002E-16,1.)) ;
#85744=DIRECTION('center_axis',(-1.,3.46944695195361E-16,0.)) ;
#85745=DIRECTION('ref_axis',(3.46944695195361E-16,1.,-1.87537673078574E-15)) ;
#85746=DIRECTION('',(-3.46944695195361E-16,-1.,-2.45739631480277E-16)) ;
#85747=DIRECTION('center_axis',(1.,-3.46944695195361E-16,0.)) ;
#85748=DIRECTION('ref_axis',(3.46944695195361E-16,1.,0.)) ;
#85749=DIRECTION('center_axis',(3.46944695195361E-16,1.,4.47619207437002E-16)) ;
#85750=DIRECTION('ref_axis',(-8.18685017503995E-48,-4.47619207437002E-16,
1.)) ;
#85751=DIRECTION('',(-1.5529910948782E-31,-4.47619207437002E-16,1.)) ;
#85752=DIRECTION('',(-1.,3.46944695195361E-16,0.)) ;
#85753=DIRECTION('',(1.5529910948782E-31,4.47619207437002E-16,-1.)) ;
#85754=DIRECTION('center_axis',(-8.52580615413453E-32,-2.45739631480277E-16,
1.)) ;
#85755=DIRECTION('ref_axis',(0.,-1.,-2.45739631480277E-16)) ;
#85756=DIRECTION('',(1.,-3.46944695195361E-16,0.)) ;
#85757=DIRECTION('',(-3.46944695195361E-16,-1.,-2.45739631480277E-16)) ;
#85758=DIRECTION('',(3.46944695195361E-16,1.,2.45739631480277E-16)) ;
#85759=DIRECTION('center_axis',(1.,-3.46944695195361E-16,0.)) ;
#85760=DIRECTION('ref_axis',(3.46944695195361E-16,1.,0.)) ;
#85761=DIRECTION('center_axis',(1.,-3.46944695195361E-16,0.)) ;
#85762=DIRECTION('ref_axis',(3.46944695195361E-16,1.,0.)) ;
#85763=DIRECTION('',(1.,-3.46944695195361E-16,0.)) ;
#85764=DIRECTION('center_axis',(-1.,3.46944695195361E-16,0.)) ;
#85765=DIRECTION('ref_axis',(3.46944695195361E-16,1.,1.98254111540207E-15)) ;
#85766=DIRECTION('',(-1.,3.46944695195361E-16,0.)) ;
#85767=DIRECTION('center_axis',(1.,-3.46944695195361E-16,0.)) ;
#85768=DIRECTION('ref_axis',(3.46944695195361E-16,1.,0.)) ;
#85769=DIRECTION('center_axis',(1.,-3.46944695195361E-16,0.)) ;
#85770=DIRECTION('ref_axis',(-3.46944695195361E-16,-1.,1.18952466924124E-14)) ;
#85771=DIRECTION('',(1.,-3.46944695195361E-16,0.)) ;
#85772=DIRECTION('center_axis',(-1.,3.46944695195361E-16,0.)) ;
#85773=DIRECTION('ref_axis',(3.46944695195361E-16,1.,5.9476233462062E-15)) ;
#85774=DIRECTION('',(-1.,3.46944695195361E-16,0.)) ;
#85775=DIRECTION('center_axis',(3.69451600012496E-31,1.06487173641454E-15,
-1.)) ;
#85776=DIRECTION('ref_axis',(0.,1.,1.06487173641454E-15)) ;
#85777=DIRECTION('',(3.46944695195361E-16,1.,1.06487173641454E-15)) ;
#85778=DIRECTION('',(-1.,3.46944695195361E-16,0.)) ;
#85779=DIRECTION('',(-3.46944695195361E-16,-1.,-1.06487173641454E-15)) ;
#85780=DIRECTION('center_axis',(3.46944695195361E-16,1.,-4.47619207437002E-16)) ;
#85781=DIRECTION('ref_axis',(8.18685017503995E-48,4.47619207437002E-16,
1.)) ;
#85782=DIRECTION('',(1.,-3.46944695195361E-16,0.)) ;
#85783=DIRECTION('',(1.5529910948782E-31,4.47619207437002E-16,1.)) ;
#85784=DIRECTION('',(-1.5529910948782E-31,-4.47619207437002E-16,-1.)) ;
#85785=DIRECTION('center_axis',(-1.,3.46944695195361E-16,0.)) ;
#85786=DIRECTION('ref_axis',(-3.46944695195361E-16,-1.,0.)) ;
#85787=DIRECTION('center_axis',(-1.,3.46944695195361E-16,0.)) ;
#85788=DIRECTION('ref_axis',(-3.46944695195361E-16,-1.,0.)) ;
#85789=DIRECTION('',(1.5529910948782E-31,4.47619207437002E-16,1.)) ;
#85790=DIRECTION('',(0.,0.,-1.)) ;
#85791=DIRECTION('center_axis',(1.,-3.46944695195361E-16,0.)) ;
#85792=DIRECTION('ref_axis',(-3.46944695195361E-16,-1.,0.)) ;
#85793=DIRECTION('center_axis',(1.,-3.46944695195361E-16,0.)) ;
#85794=DIRECTION('ref_axis',(-3.46944695195361E-16,-1.,1.07672491612354E-14)) ;
#85795=DIRECTION('',(3.46944695195361E-16,1.,1.06487173641454E-15)) ;
#85796=DIRECTION('center_axis',(1.,-3.46944695195361E-16,0.)) ;
#85797=DIRECTION('ref_axis',(3.46944695195361E-16,1.,0.)) ;
#85798=DIRECTION('center_axis',(-1.,3.46944695195361E-16,0.)) ;
#85799=DIRECTION('ref_axis',(3.46944695195361E-16,1.,0.)) ;
#85800=DIRECTION('',(0.,0.,-1.)) ;
#85801=DIRECTION('',(0.,0.,1.)) ;
#85802=DIRECTION('',(-3.46944695195361E-16,-1.,-9.27571383489107E-17)) ;
#85803=DIRECTION('center_axis',(-3.46944695195361E-16,-1.,0.)) ;
#85804=DIRECTION('ref_axis',(1.,-3.46944695195361E-16,0.)) ;
#85805=DIRECTION('',(1.,-3.46944695195361E-16,0.)) ;
#85806=DIRECTION('',(0.,0.,-1.)) ;
#85807=DIRECTION('',(0.,0.,1.)) ;
#85808=DIRECTION('center_axis',(1.,-3.46944695195361E-16,0.)) ;
#85809=DIRECTION('ref_axis',(3.46944695195361E-16,1.,0.)) ;
#85810=DIRECTION('center_axis',(1.,-3.46944695195361E-16,0.)) ;
#85811=DIRECTION('ref_axis',(3.46944695195361E-16,1.,0.)) ;
#85812=DIRECTION('',(1.,-3.46944695195361E-16,0.)) ;
#85813=DIRECTION('center_axis',(-1.,3.46944695195361E-16,0.)) ;
#85814=DIRECTION('ref_axis',(3.46944695195361E-16,1.,0.)) ;
#85815=DIRECTION('',(-1.,3.46944695195361E-16,0.)) ;
#85816=DIRECTION('center_axis',(-3.21815970916568E-32,-9.27571383489107E-17,
1.)) ;
#85817=DIRECTION('ref_axis',(0.,-1.,-9.27571383489107E-17)) ;
#85818=DIRECTION('',(3.46944695195361E-16,1.,9.27571383489107E-17)) ;
#85819=DIRECTION('',(1.,0.,3.21815970916568E-32)) ;
#85820=DIRECTION('',(-3.46944695195361E-16,-1.,-9.27571383489107E-17)) ;
#85821=DIRECTION('',(-1.,3.46944695195361E-16,0.)) ;
#85822=DIRECTION('center_axis',(1.,-3.46944695195361E-16,0.)) ;
#85823=DIRECTION('ref_axis',(3.46944695195361E-16,1.,0.)) ;
#85824=DIRECTION('center_axis',(1.,-3.46944695195361E-16,0.)) ;
#85825=DIRECTION('ref_axis',(-3.46944695195361E-16,-1.,-5.9476233462062E-15)) ;
#85826=DIRECTION('',(1.,-3.46944695195361E-16,0.)) ;
#85827=DIRECTION('center_axis',(-1.,3.46944695195361E-16,0.)) ;
#85828=DIRECTION('ref_axis',(3.46944695195361E-16,1.,-1.98254111540207E-15)) ;
#85829=DIRECTION('',(-1.,3.46944695195361E-16,0.)) ;
#85830=DIRECTION('center_axis',(-3.46944695195361E-16,-1.,0.)) ;
#85831=DIRECTION('ref_axis',(1.,-3.46944695195361E-16,0.)) ;
#85832=DIRECTION('',(0.,0.,-1.)) ;
#85833=DIRECTION('',(-1.,3.46944695195361E-16,0.)) ;
#85834=DIRECTION('',(0.,0.,1.)) ;
#85835=DIRECTION('center_axis',(2.25271179641597E-31,6.49299968442375E-16,
-1.)) ;
#85836=DIRECTION('ref_axis',(0.,1.,6.49299968442375E-16)) ;
#85837=DIRECTION('',(3.46944695195361E-16,1.,6.49299968442375E-16)) ;
#85838=DIRECTION('',(-1.,0.,-2.25271179641597E-31)) ;
#85839=DIRECTION('',(-3.46944695195361E-16,-1.,-6.49299968442375E-16)) ;
#85840=DIRECTION('',(1.,-3.46944695195361E-16,0.)) ;
#85841=DIRECTION('center_axis',(-1.,3.46944695195361E-16,0.)) ;
#85842=DIRECTION('ref_axis',(-3.46944695195361E-16,-1.,0.)) ;
#85843=DIRECTION('',(3.46944695195361E-16,1.,6.49299968442375E-16)) ;
#85844=DIRECTION('',(0.,0.,1.)) ;
#85845=DIRECTION('',(0.,0.,-1.)) ;
#85846=DIRECTION('center_axis',(-1.,3.46944695195361E-16,0.)) ;
#85847=DIRECTION('ref_axis',(-3.46944695195361E-16,-1.,0.)) ;
#85848=DIRECTION('center_axis',(-0.164398987305357,0.,-0.986393923832144)) ;
#85849=DIRECTION('ref_axis',(-0.986393923832144,0.,0.164398987305357)) ;
#85850=DIRECTION('',(-0.937042571331636,0.312347523777212,0.156173761888606)) ;
#85851=DIRECTION('',(0.,-1.,0.)) ;
#85852=DIRECTION('',(0.973328526784575,0.162221421130762,-0.162221421130763)) ;
#85853=DIRECTION('',(-1.73472347597681E-15,1.,2.89120579329468E-16)) ;
#85854=DIRECTION('center_axis',(-1.,0.,0.)) ;
#85855=DIRECTION('ref_axis',(0.,0.,1.)) ;
#85856=DIRECTION('center_axis',(-1.,0.,0.)) ;
#85857=DIRECTION('ref_axis',(0.,0.958781999165857,-0.284142707236211)) ;
#85858=DIRECTION('',(0.,0.,1.)) ;
#85859=DIRECTION('',(0.,-1.,0.)) ;
#85860=DIRECTION('center_axis',(-1.,0.,0.)) ;
#85861=DIRECTION('ref_axis',(0.,0.758706341404794,-0.65143279585246)) ;
#85862=DIRECTION('',(0.,0.,-1.)) ;
#85863=DIRECTION('center_axis',(-1.,0.,0.)) ;
#85864=DIRECTION('ref_axis',(0.,-0.654779380094552,-0.755820060201497)) ;
#85865=DIRECTION('',(0.,1.,0.)) ;
#85866=DIRECTION('center_axis',(-0.164398987305357,0.,0.986393923832144)) ;
#85867=DIRECTION('ref_axis',(0.986393923832144,0.,0.164398987305357)) ;
#85868=DIRECTION('',(-0.973328526784575,-0.162221421130762,-0.162221421130763)) ;
#85869=DIRECTION('',(0.,1.,0.)) ;
#85870=DIRECTION('',(0.937042571331636,-0.312347523777212,0.156173761888606)) ;
#85871=DIRECTION('',(1.73472347597681E-15,-1.,2.89120579329468E-16)) ;
#85872=DIRECTION('center_axis',(-0.573462344363329,0.81923192051904,0.)) ;
#85873=DIRECTION('ref_axis',(-0.81923192051904,-0.573462344363329,0.)) ;
#85874=DIRECTION('',(-0.710669054518702,-0.497468338163091,0.49746833816309)) ;
#85875=DIRECTION('',(0.,0.,-1.)) ;
#85876=DIRECTION('',(0.710669054518702,0.497468338163091,0.49746833816309)) ;
#85877=DIRECTION('',(0.,0.,1.)) ;
#85878=DIRECTION('center_axis',(-1.,0.,0.)) ;
#85879=DIRECTION('ref_axis',(0.,0.,1.)) ;
#85880=DIRECTION('',(0.,0.,1.)) ;
#85881=DIRECTION('',(0.,-1.,-9.34081871679819E-17)) ;
#85882=DIRECTION('',(0.,0.,-1.)) ;
#85883=DIRECTION('',(0.,1.,-9.34081871679819E-17)) ;
#85884=DIRECTION('center_axis',(-0.573462344363329,-0.81923192051904,0.)) ;
#85885=DIRECTION('ref_axis',(0.81923192051904,-0.573462344363329,0.)) ;
#85886=DIRECTION('',(-0.710669054518701,0.497468338163091,-0.497468338163091)) ;
#85887=DIRECTION('',(0.,0.,1.)) ;
#85888=DIRECTION('',(0.710669054518701,-0.497468338163091,-0.497468338163091)) ;
#85889=DIRECTION('',(0.,0.,-1.)) ;
#85890=DIRECTION('center_axis',(0.,0.,1.)) ;
#85891=DIRECTION('ref_axis',(1.,0.,0.)) ;
#85892=DIRECTION('',(1.,6.67201336914158E-17,0.)) ;
#85893=DIRECTION('',(1.33440267382831E-16,1.,0.)) ;
#85894=DIRECTION('',(-1.,1.33440267382831E-16,0.)) ;
#85895=DIRECTION('center_axis',(0.,0.,1.)) ;
#85896=DIRECTION('ref_axis',(1.,0.,0.)) ;
#85897=DIRECTION('',(1.,-1.33440267382831E-16,0.)) ;
#85898=DIRECTION('',(-1.33440267382831E-16,-1.,0.)) ;
#85899=DIRECTION('',(-1.,-6.67201336914158E-17,0.)) ;
#85900=DIRECTION('center_axis',(-6.67201336914158E-17,1.,0.)) ;
#85901=DIRECTION('ref_axis',(-1.,-6.67201336914158E-17,0.)) ;
#85902=DIRECTION('',(1.,6.67201336914158E-17,0.)) ;
#85903=DIRECTION('',(0.,0.,1.)) ;
#85904=DIRECTION('',(-1.,-6.67201336914158E-17,0.)) ;
#85905=DIRECTION('center_axis',(-1.33440267382831E-16,-1.,0.)) ;
#85906=DIRECTION('ref_axis',(1.,-1.33440267382831E-16,0.)) ;
#85907=DIRECTION('',(1.,-1.33440267382831E-16,0.)) ;
#85908=DIRECTION('',(0.,0.,-1.)) ;
#85909=DIRECTION('',(-1.,1.33440267382831E-16,0.)) ;
#85910=DIRECTION('center_axis',(0.,0.,1.)) ;
#85911=DIRECTION('ref_axis',(1.,0.,0.)) ;
#85912=DIRECTION('',(0.,-1.,0.)) ;
#85913=DIRECTION('',(1.,0.,0.)) ;
#85914=DIRECTION('',(0.,1.,0.)) ;
#85915=DIRECTION('center_axis',(0.,0.,-1.)) ;
#85916=DIRECTION('ref_axis',(1.,0.,0.)) ;
#85917=DIRECTION('',(-1.44560289664734E-16,1.,-7.2280144832367E-17)) ;
#85918=DIRECTION('center_axis',(0.,0.,1.)) ;
#85919=DIRECTION('ref_axis',(1.,0.,0.)) ;
#85920=DIRECTION('center_axis',(0.,0.,1.)) ;
#85921=DIRECTION('ref_axis',(1.,0.,0.)) ;
#85922=DIRECTION('',(0.,-1.,0.)) ;
#85923=DIRECTION('',(-1.,0.,0.)) ;
#85924=DIRECTION('',(0.,1.,0.)) ;
#85925=DIRECTION('center_axis',(0.,0.,-1.)) ;
#85926=DIRECTION('ref_axis',(1.,-1.82602471155453E-15,0.)) ;
#85927=DIRECTION('',(1.44560289664734E-16,-1.,-2.4093381610789E-16)) ;
#85928=DIRECTION('center_axis',(0.,0.,1.)) ;
#85929=DIRECTION('ref_axis',(1.,0.,0.)) ;
#85930=DIRECTION('center_axis',(0.,0.,-1.)) ;
#85931=DIRECTION('ref_axis',(-1.,0.,0.)) ;
#85932=DIRECTION('',(0.,0.,-1.)) ;
#85933=DIRECTION('center_axis',(0.,0.,-1.)) ;
#85934=DIRECTION('ref_axis',(1.,0.,0.)) ;
#85935=DIRECTION('center_axis',(0.,0.,1.)) ;
#85936=DIRECTION('ref_axis',(1.,0.,0.)) ;
#85937=DIRECTION('center_axis',(1.,0.,0.)) ;
#85938=DIRECTION('ref_axis',(0.,0.,-1.)) ;
#85939=DIRECTION('',(0.,-1.,0.)) ;
#85940=DIRECTION('',(0.,0.,1.)) ;
#85941=DIRECTION('',(0.,1.,0.)) ;
#85942=DIRECTION('center_axis',(0.81923192051904,0.573462344363329,0.)) ;
#85943=DIRECTION('ref_axis',(-0.573462344363329,0.81923192051904,0.)) ;
#85944=DIRECTION('',(-0.497468338163091,0.710669054518701,0.497468338163091)) ;
#85945=DIRECTION('',(0.,0.,-1.)) ;
#85946=DIRECTION('',(0.497468338163091,-0.710669054518701,0.497468338163091)) ;
#85947=DIRECTION('',(0.,0.,1.)) ;
#85948=DIRECTION('center_axis',(0.,1.,0.)) ;
#85949=DIRECTION('ref_axis',(0.,0.,1.)) ;
#85950=DIRECTION('',(0.,0.,1.)) ;
#85951=DIRECTION('',(-1.,0.,0.)) ;
#85952=DIRECTION('',(0.,0.,-1.)) ;
#85953=DIRECTION('',(1.,0.,0.)) ;
#85954=DIRECTION('center_axis',(-0.81923192051904,0.573462344363329,0.)) ;
#85955=DIRECTION('ref_axis',(-0.573462344363329,-0.81923192051904,0.)) ;
#85956=DIRECTION('',(0.497468338163091,0.710669054518701,-0.497468338163091)) ;
#85957=DIRECTION('',(0.,0.,1.)) ;
#85958=DIRECTION('',(-0.497468338163091,-0.710669054518701,-0.497468338163091)) ;
#85959=DIRECTION('',(0.,0.,-1.)) ;
#85960=DIRECTION('center_axis',(-1.,0.,0.)) ;
#85961=DIRECTION('ref_axis',(0.,0.,1.)) ;
#85962=DIRECTION('',(0.,-1.,0.)) ;
#85963=DIRECTION('',(0.,0.,-1.)) ;
#85964=DIRECTION('',(0.,1.,0.)) ;
#85965=DIRECTION('',(0.,0.,-1.)) ;
#85966=DIRECTION('center_axis',(0.,0.,-1.)) ;
#85967=DIRECTION('ref_axis',(-1.,0.,0.)) ;
#85968=DIRECTION('center_axis',(0.,0.,1.)) ;
#85969=DIRECTION('ref_axis',(1.,0.,0.)) ;
#85970=DIRECTION('center_axis',(0.,0.,-1.)) ;
#85971=DIRECTION('ref_axis',(1.,5.20417042793042E-15,0.)) ;
#85972=DIRECTION('center_axis',(-0.573462344363328,7.65229685658278E-17,
0.819231920519041)) ;
#85973=DIRECTION('ref_axis',(0.819231920519041,1.22423955297878E-32,0.573462344363328)) ;
#85974=DIRECTION('',(-0.710669054518702,-0.497468338163091,-0.497468338163091)) ;
#85975=DIRECTION('',(1.33440267382831E-16,1.,-2.91413396387194E-34)) ;
#85976=DIRECTION('',(0.710669054518701,-0.497468338163091,0.497468338163091)) ;
#85977=DIRECTION('',(5.04890651880155E-33,-1.,9.34081871679819E-17)) ;
#85978=DIRECTION('center_axis',(-0.573462344363328,7.65229685658278E-17,
-0.819231920519041)) ;
#85979=DIRECTION('ref_axis',(-0.819231920519041,-1.22423955297878E-32,0.573462344363328)) ;
#85980=DIRECTION('',(-0.710669054518701,0.497468338163091,0.497468338163091)) ;
#85981=DIRECTION('',(-1.33440267382831E-16,-1.,7.77328292223541E-33)) ;
#85982=DIRECTION('',(0.710669054518702,0.497468338163091,-0.497468338163091)) ;
#85983=DIRECTION('',(-5.04890651880155E-33,1.,9.34081871679819E-17)) ;
#85984=DIRECTION('center_axis',(0.,0.573462344363328,-0.819231920519041)) ;
#85985=DIRECTION('ref_axis',(0.,0.819231920519041,0.573462344363328)) ;
#85986=DIRECTION('',(0.497468338163091,0.710669054518701,0.497468338163091)) ;
#85987=DIRECTION('',(-1.,0.,0.)) ;
#85988=DIRECTION('',(0.497468338163091,-0.710669054518701,-0.497468338163091)) ;
#85989=DIRECTION('',(1.,0.,0.)) ;
#85990=DIRECTION('center_axis',(0.,0.573462344363328,0.819231920519041)) ;
#85991=DIRECTION('ref_axis',(0.,-0.819231920519041,0.573462344363328)) ;
#85992=DIRECTION('',(-0.497468338163091,0.710669054518701,-0.497468338163091)) ;
#85993=DIRECTION('',(1.,0.,0.)) ;
#85994=DIRECTION('',(-0.497468338163091,-0.710669054518701,0.497468338163091)) ;
#85995=DIRECTION('',(-1.,0.,0.)) ;
#85996=DIRECTION('center_axis',(-0.164398987305354,-0.986393923832144,0.)) ;
#85997=DIRECTION('ref_axis',(0.,0.,1.)) ;
#85998=DIRECTION('',(0.,0.,-1.)) ;
#85999=DIRECTION('center_axis',(-0.164398987305316,-0.986393923832151,-6.5096352405955E-13)) ;
#86000=DIRECTION('ref_axis',(-0.0577290357396871,0.00962150595595322,0.998285923498727)) ;
#86001=DIRECTION('',(0.,0.,1.)) ;
#86002=DIRECTION('center_axis',(1.,-2.89120579329441E-16,0.)) ;
#86003=DIRECTION('ref_axis',(-2.89120579329441E-16,-1.,-7.6571373978539E-16)) ;
#86004=DIRECTION('center_axis',(1.,1.15648231731787E-15,0.)) ;
#86005=DIRECTION('ref_axis',(1.15648231731787E-15,-1.,0.)) ;
#86006=DIRECTION('center_axis',(0.166689823555444,0.983956802853964,0.0635886219418303)) ;
#86007=DIRECTION('ref_axis',(-0.048648001075619,0.072619415360229,-0.996172571648148)) ;
#86008=DIRECTION('center_axis',(0.166689823591591,0.983956802798768,-0.0635886227011592)) ;
#86009=DIRECTION('ref_axis',(-0.0462047033417876,0.072214919745475,0.996318287875542)) ;
#86010=DIRECTION('center_axis',(-0.164398987305354,-0.986393923832144,0.)) ;
#86011=DIRECTION('ref_axis',(0.,0.,1.)) ;
#86012=DIRECTION('',(0.,0.,1.)) ;
#86013=DIRECTION('center_axis',(-0.164398987305377,-0.98639392383214,-4.33975683666443E-13)) ;
#86014=DIRECTION('ref_axis',(-0.0554192327903482,0.00923653879883178,-0.99842045000488)) ;
#86015=DIRECTION('',(0.,0.,-1.)) ;
#86016=DIRECTION('center_axis',(0.,0.,1.)) ;
#86017=DIRECTION('ref_axis',(1.,0.,0.)) ;
#86018=DIRECTION('center_axis',(0.,0.,1.)) ;
#86019=DIRECTION('ref_axis',(1.,0.,0.)) ;
#86020=DIRECTION('center_axis',(0.,1.,0.)) ;
#86021=DIRECTION('ref_axis',(1.,0.,0.)) ;
#86022=DIRECTION('center_axis',(0.,-0.888198741900269,0.45945945945946)) ;
#86023=DIRECTION('ref_axis',(0.,0.45945945945946,0.888198741900269)) ;
#86024=DIRECTION('center_axis',(-1.,0.,1.22067519501986E-15)) ;
#86025=DIRECTION('ref_axis',(-1.22067519501986E-15,0.,-1.)) ;
#86026=DIRECTION('center_axis',(0.,0.,1.)) ;
#86027=DIRECTION('ref_axis',(1.,0.,0.)) ;
#86028=DIRECTION('center_axis',(0.,0.,-1.)) ;
#86029=DIRECTION('ref_axis',(-1.,0.,0.)) ;
#86030=DIRECTION('center_axis',(1.,-3.46944695195361E-16,0.)) ;
#86031=DIRECTION('ref_axis',(3.46944695195361E-16,1.,0.)) ;
#86032=DIRECTION('center_axis',(-1.,3.46944695195361E-16,0.)) ;
#86033=DIRECTION('ref_axis',(3.46944695195361E-16,1.,0.)) ;
#86034=DIRECTION('center_axis',(-1.,3.46944695195361E-16,0.)) ;
#86035=DIRECTION('ref_axis',(-3.41607084500048E-16,-1.,0.)) ;
#86036=DIRECTION('center_axis',(0.,-0.459459459459457,0.888198741900271)) ;
#86037=DIRECTION('ref_axis',(0.,-0.888198741900271,-0.459459459459457)) ;
#86038=DIRECTION('center_axis',(1.,-3.46944695195361E-16,0.)) ;
#86039=DIRECTION('ref_axis',(0.,1.,0.)) ;
#86040=DIRECTION('center_axis',(0.,0.888198741900269,-0.45945945945946)) ;
#86041=DIRECTION('ref_axis',(0.,-0.45945945945946,-0.888198741900269)) ;
#86042=DIRECTION('center_axis',(0.,1.,0.)) ;
#86043=DIRECTION('ref_axis',(1.,0.,0.)) ;
#86044=DIRECTION('center_axis',(0.,-1.,0.)) ;
#86045=DIRECTION('ref_axis',(0.,0.,1.)) ;
#86046=DIRECTION('center_axis',(-1.,0.,0.)) ;
#86047=DIRECTION('ref_axis',(0.,0.,-1.)) ;
#86048=DIRECTION('center_axis',(0.,0.,-1.)) ;
#86049=DIRECTION('ref_axis',(-1.,0.,0.)) ;
#86050=DIRECTION('center_axis',(0.,0.,-1.)) ;
#86051=DIRECTION('ref_axis',(-1.,0.,0.)) ;
#86052=DIRECTION('center_axis',(1.,-3.46944695195361E-16,0.)) ;
#86053=DIRECTION('ref_axis',(3.46944695195361E-16,1.,0.)) ;
#86054=DIRECTION('center_axis',(-1.,3.46944695195361E-16,0.)) ;
#86055=DIRECTION('ref_axis',(3.46944695195361E-16,1.,3.46944695195361E-14)) ;
#86056=DIRECTION('center_axis',(1.,0.,0.)) ;
#86057=DIRECTION('ref_axis',(0.,0.,-1.)) ;
#86058=DIRECTION('center_axis',(0.,0.,1.)) ;
#86059=DIRECTION('ref_axis',(1.,0.,0.)) ;
#86060=DIRECTION('center_axis',(0.,0.,1.)) ;
#86061=DIRECTION('ref_axis',(1.,0.,0.)) ;
#86062=DIRECTION('center_axis',(1.,-3.46944695195361E-16,0.)) ;
#86063=DIRECTION('ref_axis',(3.80647894157197E-16,1.,0.)) ;
#86064=DIRECTION('center_axis',(0.,0.459459459459459,-0.888198741900269)) ;
#86065=DIRECTION('ref_axis',(0.,0.888198741900269,0.459459459459459)) ;
#86066=DIRECTION('center_axis',(1.,-3.46944695195361E-16,0.)) ;
#86067=DIRECTION('ref_axis',(3.46944695195361E-16,1.,0.)) ;
#86068=DIRECTION('center_axis',(-1.,3.46944695195361E-16,0.)) ;
#86069=DIRECTION('ref_axis',(3.46944695195361E-16,1.,0.)) ;
#86070=DIRECTION('center_axis',(-3.46944695195361E-16,-1.,-6.49299968442375E-16)) ;
#86071=DIRECTION('ref_axis',(2.25271179641597E-31,6.49299968442375E-16,
-1.)) ;
#86072=DIRECTION('center_axis',(0.,-1.,0.)) ;
#86073=DIRECTION('ref_axis',(0.,0.,-1.)) ;
#86074=DIRECTION('center_axis',(0.,0.,1.)) ;
#86075=DIRECTION('ref_axis',(1.,0.,0.)) ;
#86076=DIRECTION('center_axis',(-3.25260651745651E-15,0.,1.)) ;
#86077=DIRECTION('ref_axis',(1.,0.,3.25260651745651E-15)) ;
#86078=DIRECTION('center_axis',(0.,1.,0.)) ;
#86079=DIRECTION('ref_axis',(1.,0.,0.)) ;
#86080=DIRECTION('center_axis',(0.,-0.888198741900269,-0.45945945945946)) ;
#86081=DIRECTION('ref_axis',(0.,-0.45945945945946,0.888198741900269)) ;
#86082=DIRECTION('center_axis',(1.,-3.46944695195361E-16,0.)) ;
#86083=DIRECTION('ref_axis',(0.,1.,0.)) ;
#86084=DIRECTION('center_axis',(0.,0.888198741900269,0.45945945945946)) ;
#86085=DIRECTION('ref_axis',(0.,0.45945945945946,-0.888198741900269)) ;
#86086=DIRECTION('center_axis',(1.,-3.46944695195361E-16,0.)) ;
#86087=DIRECTION('ref_axis',(0.,1.,0.)) ;
#86088=DIRECTION('center_axis',(0.,1.,0.)) ;
#86089=DIRECTION('ref_axis',(0.,0.,-1.)) ;
#86090=DIRECTION('center_axis',(0.,1.,0.)) ;
#86091=DIRECTION('ref_axis',(1.,0.,0.)) ;
#86092=DIRECTION('center_axis',(-1.,0.,0.)) ;
#86093=DIRECTION('ref_axis',(0.,0.,-1.)) ;
#86094=DIRECTION('center_axis',(1.,-3.46944695195361E-16,0.)) ;
#86095=DIRECTION('ref_axis',(3.41607084500048E-16,1.,0.)) ;
#86096=DIRECTION('center_axis',(-9.62987005567165E-16,-0.459459459459459,
-0.88819874190027)) ;
#86097=DIRECTION('ref_axis',(-7.31984232283282E-30,0.88819874190027,-0.459459459459459)) ;
#86098=DIRECTION('center_axis',(1.,-3.46944695195361E-16,0.)) ;
#86099=DIRECTION('ref_axis',(3.46944695195361E-16,1.,0.)) ;
#86100=DIRECTION('center_axis',(-1.,3.46944695195361E-16,0.)) ;
#86101=DIRECTION('ref_axis',(3.46944695195361E-16,1.,0.)) ;
#86102=DIRECTION('center_axis',(1.,0.,0.)) ;
#86103=DIRECTION('ref_axis',(0.,0.,-1.)) ;
#86104=DIRECTION('center_axis',(1.,-3.46944695195361E-16,0.)) ;
#86105=DIRECTION('ref_axis',(3.80647894157197E-16,1.,0.)) ;
#86106=DIRECTION('center_axis',(0.,0.459459459459459,0.888198741900269)) ;
#86107=DIRECTION('ref_axis',(0.,-0.888198741900269,0.459459459459459)) ;
#86108=DIRECTION('center_axis',(-3.46944695195361E-16,-1.,-6.49299968442375E-16)) ;
#86109=DIRECTION('ref_axis',(2.25271179641597E-31,6.49299968442375E-16,
-1.)) ;
#86110=DIRECTION('center_axis',(0.,1.,0.)) ;
#86111=DIRECTION('ref_axis',(0.,0.,-1.)) ;
#86112=DIRECTION('center_axis',(1.,0.,2.25271179641597E-31)) ;
#86113=DIRECTION('ref_axis',(2.25271179641597E-31,0.,-1.)) ;
#86114=DIRECTION('center_axis',(-1.,0.,0.)) ;
#86115=DIRECTION('ref_axis',(0.,0.,1.)) ;
#86116=DIRECTION('center_axis',(0.,1.,0.)) ;
#86117=DIRECTION('ref_axis',(1.,0.,0.)) ;
#86118=DIRECTION('center_axis',(0.,-1.,0.)) ;
#86119=DIRECTION('ref_axis',(-1.08420217248551E-15,0.,1.)) ;
#86120=DIRECTION('center_axis',(1.,-3.46944695195361E-16,0.)) ;
#86121=DIRECTION('ref_axis',(0.,1.,0.)) ;
#86122=DIRECTION('center_axis',(0.,1.,0.)) ;
#86123=DIRECTION('ref_axis',(0.,0.,-1.)) ;
#86124=DIRECTION('center_axis',(0.,-1.,0.)) ;
#86125=DIRECTION('ref_axis',(0.,0.,-1.)) ;
#86126=DIRECTION('center_axis',(0.,0.,1.)) ;
#86127=DIRECTION('ref_axis',(-1.,0.,0.)) ;
#86128=DIRECTION('center_axis',(0.,0.,-1.)) ;
#86129=DIRECTION('ref_axis',(-1.,0.,0.)) ;
#86130=DIRECTION('center_axis',(0.,0.,-1.)) ;
#86131=DIRECTION('ref_axis',(-1.,0.,0.)) ;
#86132=DIRECTION('center_axis',(-3.46944695195361E-16,-1.,-9.27571383489107E-17)) ;
#86133=DIRECTION('ref_axis',(1.,-3.46944695195361E-16,-3.21815970916568E-32)) ;
#86134=DIRECTION('center_axis',(0.,-1.,0.)) ;
#86135=DIRECTION('ref_axis',(0.,0.,-1.)) ;
#86136=DIRECTION('center_axis',(3.46944695195361E-16,1.,9.27571383489107E-17)) ;
#86137=DIRECTION('ref_axis',(-1.,3.46944695195361E-16,3.21815970916568E-32)) ;
#86138=DIRECTION('center_axis',(0.,1.,0.)) ;
#86139=DIRECTION('ref_axis',(0.,0.,-1.)) ;
#86140=DIRECTION('center_axis',(0.,0.,-1.)) ;
#86141=DIRECTION('ref_axis',(-1.,0.,0.)) ;
#86142=DIRECTION('center_axis',(0.,0.,1.)) ;
#86143=DIRECTION('ref_axis',(1.,0.,0.)) ;
#86144=DIRECTION('center_axis',(0.,1.,0.)) ;
#86145=DIRECTION('ref_axis',(1.,0.,0.)) ;
#86146=DIRECTION('center_axis',(-1.,0.,1.0842021724855E-15)) ;
#86147=DIRECTION('ref_axis',(-1.0842021724855E-15,0.,-1.)) ;
#86148=DIRECTION('center_axis',(0.,-1.,0.)) ;
#86149=DIRECTION('ref_axis',(0.,0.,-1.)) ;
#86150=DIRECTION('center_axis',(1.,0.,0.)) ;
#86151=DIRECTION('ref_axis',(0.,0.,1.)) ;
#86152=DIRECTION('center_axis',(1.,0.,3.21815970916568E-32)) ;
#86153=DIRECTION('ref_axis',(3.21815970916568E-32,0.,-1.)) ;
#86154=DIRECTION('center_axis',(0.,1.,0.)) ;
#86155=DIRECTION('ref_axis',(1.,0.,0.)) ;
#86156=DIRECTION('center_axis',(0.,0.,-1.)) ;
#86157=DIRECTION('ref_axis',(1.,0.,0.)) ;
#86158=DIRECTION('center_axis',(1.,0.,0.)) ;
#86159=DIRECTION('ref_axis',(0.,-1.08420217248551E-15,1.)) ;
#86160=DIRECTION('center_axis',(1.0842021724855E-15,1.,0.)) ;
#86161=DIRECTION('ref_axis',(1.,-1.0842021724855E-15,0.)) ;
#86162=DIRECTION('center_axis',(1.,0.,-2.08976773479518E-32)) ;
#86163=DIRECTION('ref_axis',(-2.08976773479518E-32,0.,-1.)) ;
#86164=DIRECTION('center_axis',(-0.447220452189282,-7.10036080930881E-6,
-0.894423762594219)) ;
#86165=DIRECTION('ref_axis',(0.894325663270107,0.0148067719344852,-0.447171519130372)) ;
#86166=DIRECTION('center_axis',(-1.23908819712629E-16,1.,2.4093381610789E-16)) ;
#86167=DIRECTION('ref_axis',(2.98538247827883E-32,-2.4093381610789E-16,
1.)) ;
#86168=DIRECTION('center_axis',(-5.60223364641742E-6,-0.447219005479868,
-0.894424485971965)) ;
#86169=DIRECTION('ref_axis',(0.0146917039307497,0.894327914920294,-0.44717081124547)) ;
#86170=DIRECTION('center_axis',(-8.95614743483648E-33,0.,1.)) ;
#86171=DIRECTION('ref_axis',(1.,0.,8.95614743483648E-33)) ;
#86172=DIRECTION('center_axis',(1.40488587213121E-32,-1.23908819712629E-16,
-1.)) ;
#86173=DIRECTION('ref_axis',(1.74077750246726E-48,1.,-1.23908819712629E-16)) ;
#86174=DIRECTION('center_axis',(-2.65552944032596E-32,0.,1.)) ;
#86175=DIRECTION('ref_axis',(1.,0.,2.65552944032596E-32)) ;
#86176=DIRECTION('center_axis',(0.894424485971418,-5.60223458619776E-6,
0.447219005480961)) ;
#86177=DIRECTION('ref_axis',(0.447170811246815,0.0146917038942881,-0.89432791492022)) ;
#86178=DIRECTION('center_axis',(0.894423762593897,-7.10036028474965E-6,
-0.447220452189924)) ;
#86179=DIRECTION('ref_axis',(0.447171519131165,0.0148067719106287,0.894325663270105)) ;
#86180=DIRECTION('center_axis',(-8.95614743483648E-33,-1.10974565782288E-48,
1.)) ;
#86181=DIRECTION('ref_axis',(1.,-9.9390457266313E-81,8.95614743483648E-33)) ;
#86182=DIRECTION('center_axis',(-7.10036046195813E-6,0.894423762593789,
0.44722045219014)) ;
#86183=DIRECTION('ref_axis',(-0.0148067719149123,-0.447171519131355,0.894325663269939)) ;
#86184=DIRECTION('center_axis',(-5.60223476175893E-6,0.894424485971284,
-0.447219005481229)) ;
#86185=DIRECTION('ref_axis',(0.0146917038893733,0.447170811247117,0.89432791492015)) ;
#86186=DIRECTION('center_axis',(1.40488587213121E-32,-1.23908819712629E-16,
-1.)) ;
#86187=DIRECTION('ref_axis',(0.,1.,0.)) ;
#86188=DIRECTION('center_axis',(-1.,0.,0.)) ;
#86189=DIRECTION('ref_axis',(0.,0.,-1.)) ;
#86190=DIRECTION('center_axis',(0.,-1.,0.)) ;
#86191=DIRECTION('ref_axis',(0.,0.,1.)) ;
#86192=DIRECTION('center_axis',(-1.,0.,-1.40488587213121E-32)) ;
#86193=DIRECTION('ref_axis',(-1.40488587213121E-32,0.,1.)) ;
#86194=DIRECTION('',(-1.,0.,-1.40488587213121E-32)) ;
#86195=DIRECTION('center_axis',(-1.,0.,0.)) ;
#86196=DIRECTION('ref_axis',(0.,0.,1.)) ;
#86197=DIRECTION('center_axis',(0.,1.,0.)) ;
#86198=DIRECTION('ref_axis',(1.,0.,0.)) ;
#86199=DIRECTION('center_axis',(0.,1.,0.)) ;
#86200=DIRECTION('ref_axis',(0.,0.,-1.)) ;
#86201=DIRECTION('center_axis',(0.,0.,-1.)) ;
#86202=DIRECTION('ref_axis',(1.,0.,0.)) ;
#86203=DIRECTION('center_axis',(-1.,0.,-1.7912294869673E-32)) ;
#86204=DIRECTION('ref_axis',(-1.7912294869673E-32,0.,1.)) ;
#86205=DIRECTION('center_axis',(-0.44721900547972,-5.60223438155825E-6,
0.894424485972038)) ;
#86206=DIRECTION('ref_axis',(0.894327914920351,0.0146917039315984,0.447170811245326)) ;
#86207=DIRECTION('center_axis',(-1.,0.,0.)) ;
#86208=DIRECTION('ref_axis',(0.,0.,1.)) ;
#86209=DIRECTION('center_axis',(1.23908819712629E-16,-1.,7.2280144832367E-17)) ;
#86210=DIRECTION('ref_axis',(1.,1.23908819712629E-16,-8.95614743483648E-33)) ;
#86211=DIRECTION('center_axis',(-7.10035968146942E-6,-0.447220452189183,
0.894423762594268)) ;
#86212=DIRECTION('ref_axis',(-0.0148067719292095,-0.894325663270233,-0.447171519130293)) ;
#86213=DIRECTION('center_axis',(0.,-1.,1.0842021724855E-15)) ;
#86214=DIRECTION('ref_axis',(0.,-1.0842021724855E-15,-1.)) ;
#86215=DIRECTION('center_axis',(1.23908819712629E-16,-1.,1.23908819712629E-16)) ;
#86216=DIRECTION('ref_axis',(-9.81657386420148E-47,-1.23908819712629E-16,
-1.)) ;
#86217=DIRECTION('center_axis',(0.,-1.,0.)) ;
#86218=DIRECTION('ref_axis',(0.,0.,-1.)) ;
#86219=DIRECTION('',(-1.23908819712629E-16,1.,-1.23908819712629E-16)) ;
#86220=DIRECTION('center_axis',(1.,0.,1.40488587213121E-32)) ;
#86221=DIRECTION('ref_axis',(1.40488587213121E-32,0.,-1.)) ;
#86222=DIRECTION('center_axis',(-0.707106781186547,0.707106781186548,-6.41152859744984E-16)) ;
#86223=DIRECTION('ref_axis',(0.707106781186548,0.707106781186547,-1.43971204814373E-12)) ;
#86224=DIRECTION('center_axis',(1.,0.,0.)) ;
#86225=DIRECTION('ref_axis',(0.,0.,-1.)) ;
#86226=DIRECTION('center_axis',(0.,-1.,0.)) ;
#86227=DIRECTION('ref_axis',(0.,0.,-1.)) ;
#86228=DIRECTION('center_axis',(0.,0.,1.)) ;
#86229=DIRECTION('ref_axis',(-1.,0.,0.)) ;
#86230=DIRECTION('center_axis',(7.2280144832367E-17,0.,-1.)) ;
#86231=DIRECTION('ref_axis',(-1.,0.,-7.2280144832367E-17)) ;
#86232=DIRECTION('',(7.2280144832367E-17,0.,-1.)) ;
#86233=DIRECTION('center_axis',(0.,0.,-1.)) ;
#86234=DIRECTION('ref_axis',(-1.,0.,0.)) ;
#86235=DIRECTION('center_axis',(0.,1.,0.)) ;
#86236=DIRECTION('ref_axis',(1.,0.,0.)) ;
#86237=DIRECTION('center_axis',(0.,0.,1.)) ;
#86238=DIRECTION('ref_axis',(-1.,0.,0.)) ;
#86239=DIRECTION('center_axis',(0.,1.,0.)) ;
#86240=DIRECTION('ref_axis',(1.,0.,0.)) ;
#86241=DIRECTION('center_axis',(1.,0.,0.)) ;
#86242=DIRECTION('ref_axis',(0.,0.,1.)) ;
#86243=DIRECTION('center_axis',(0.,0.,-1.)) ;
#86244=DIRECTION('ref_axis',(1.,0.,0.)) ;
#86245=DIRECTION('center_axis',(-1.13380619344889E-16,1.,-1.23908819712629E-16)) ;
#86246=DIRECTION('ref_axis',(-1.40488587213121E-32,1.23908819712629E-16,
1.)) ;
#86247=DIRECTION('center_axis',(0.,1.,0.)) ;
#86248=DIRECTION('ref_axis',(0.,0.,1.)) ;
#86249=DIRECTION('center_axis',(7.2280144832367E-17,0.,-1.)) ;
#86250=DIRECTION('ref_axis',(-1.,0.,-7.2280144832367E-17)) ;
#86251=DIRECTION('center_axis',(0.,0.,1.)) ;
#86252=DIRECTION('ref_axis',(1.,0.,0.)) ;
#86253=DIRECTION('center_axis',(0.,1.,0.)) ;
#86254=DIRECTION('ref_axis',(1.,0.,0.)) ;
#86255=DIRECTION('center_axis',(0.,1.,0.)) ;
#86256=DIRECTION('ref_axis',(0.,0.,-1.)) ;
#86257=DIRECTION('center_axis',(1.,2.16840434497101E-15,-2.93873587705572E-31)) ;
#86258=DIRECTION('ref_axis',(2.16840434497101E-15,-1.,-1.03035812136257E-62)) ;
#86259=DIRECTION('center_axis',(-8.95614743483648E-33,0.,1.)) ;
#86260=DIRECTION('ref_axis',(1.,0.,8.95614743483648E-33)) ;
#86261=DIRECTION('center_axis',(-1.40488587213121E-32,1.23908819712629E-16,
1.)) ;
#86262=DIRECTION('ref_axis',(-1.74077750246726E-48,-1.,1.23908819712629E-16)) ;
#86263=DIRECTION('center_axis',(8.95614743483648E-33,1.0154535431059E-48,
-1.)) ;
#86264=DIRECTION('ref_axis',(-1.,9.09455164528354E-81,-8.95614743483648E-33)) ;
#86265=DIRECTION('center_axis',(2.16840434497101E-15,0.,-1.)) ;
#86266=DIRECTION('ref_axis',(-1.,0.,-2.16840434497101E-15)) ;
#86267=DIRECTION('',(-8.95614743483648E-33,-1.0154535431059E-48,1.)) ;
#86268=DIRECTION('center_axis',(-1.,-1.13380619344889E-16,0.)) ;
#86269=DIRECTION('ref_axis',(0.,-1.,0.)) ;
#86270=DIRECTION('center_axis',(0.,0.,1.)) ;
#86271=DIRECTION('ref_axis',(-1.,0.,0.)) ;
#86272=DIRECTION('center_axis',(0.,-1.,0.)) ;
#86273=DIRECTION('ref_axis',(0.,0.,-1.)) ;
#86274=DIRECTION('center_axis',(-1.,0.,0.)) ;
#86275=DIRECTION('ref_axis',(0.,0.,-1.)) ;
#86276=DIRECTION('center_axis',(1.,0.,1.40488587213121E-32)) ;
#86277=DIRECTION('ref_axis',(1.40488587213121E-32,0.,-1.)) ;
#86278=DIRECTION('',(1.,0.,1.40488587213121E-32)) ;
#86279=DIRECTION('center_axis',(1.,0.,0.)) ;
#86280=DIRECTION('ref_axis',(0.,0.,-1.)) ;
#86281=DIRECTION('center_axis',(-1.40488587213121E-32,1.23908819712629E-16,
1.)) ;
#86282=DIRECTION('ref_axis',(0.,-1.,0.)) ;
#86283=DIRECTION('center_axis',(0.,-1.,0.)) ;
#86284=DIRECTION('ref_axis',(0.,0.,1.)) ;
#86285=DIRECTION('center_axis',(0.,1.,0.)) ;
#86286=DIRECTION('ref_axis',(1.,0.,0.)) ;
#86287=DIRECTION('center_axis',(1.,0.,0.)) ;
#86288=DIRECTION('ref_axis',(0.,0.,1.)) ;
#86289=DIRECTION('center_axis',(0.,1.,0.)) ;
#86290=DIRECTION('ref_axis',(0.,0.,-1.)) ;
#86291=DIRECTION('center_axis',(0.,0.,1.)) ;
#86292=DIRECTION('ref_axis',(1.,0.,0.)) ;
#86293=DIRECTION('center_axis',(0.,0.,1.)) ;
#86294=DIRECTION('ref_axis',(1.,0.,0.)) ;
#86295=DIRECTION('center_axis',(1.,0.,1.40488587213121E-32)) ;
#86296=DIRECTION('ref_axis',(1.40488587213121E-32,0.,-1.)) ;
#86297=DIRECTION('center_axis',(-0.707106781186552,0.707106781186543,-7.95029546083828E-15)) ;
#86298=DIRECTION('ref_axis',(0.707106781186543,0.707106781186552,-1.6468249326304E-12)) ;
#86299=DIRECTION('center_axis',(-1.23908819712629E-16,1.,-1.23908819712629E-16)) ;
#86300=DIRECTION('ref_axis',(9.81657386420148E-47,1.23908819712629E-16,
1.)) ;
#86301=DIRECTION('',(1.23908819712629E-16,-1.,1.23908819712629E-16)) ;
#86302=DIRECTION('center_axis',(-1.,-1.13380619344889E-16,0.)) ;
#86303=DIRECTION('ref_axis',(0.,-1.,0.)) ;
#86304=DIRECTION('center_axis',(0.,-1.,0.)) ;
#86305=DIRECTION('ref_axis',(0.,0.,1.)) ;
#86306=DIRECTION('center_axis',(1.13380619344889E-16,-1.,1.23908819712629E-16)) ;
#86307=DIRECTION('ref_axis',(1.40488587213121E-32,-1.23908819712629E-16,
-1.)) ;
#86308=DIRECTION('center_axis',(-1.5529910948782E-31,-4.47619207437002E-16,
1.)) ;
#86309=DIRECTION('ref_axis',(6.951486430461E-47,-1.,-4.47619207437002E-16)) ;
#86310=DIRECTION('center_axis',(0.,2.16840434497101E-15,-1.)) ;
#86311=DIRECTION('ref_axis',(0.,1.,2.16840434497101E-15)) ;
#86312=DIRECTION('center_axis',(0.,1.,0.)) ;
#86313=DIRECTION('ref_axis',(1.,0.,0.)) ;
#86314=DIRECTION('center_axis',(3.85194802226865E-15,0.888198741900269,
-0.45945945945946)) ;
#86315=DIRECTION('ref_axis',(3.25260651745654E-15,-0.45945945945946,-0.888198741900269)) ;
#86316=DIRECTION('center_axis',(-1.,0.,1.22067519501986E-15)) ;
#86317=DIRECTION('ref_axis',(-1.22067519501986E-15,3.46944695195364E-14,
-1.)) ;
#86318=DIRECTION('center_axis',(1.5529910948782E-31,4.47619207437002E-16,
-1.)) ;
#86319=DIRECTION('ref_axis',(-6.951486430461E-47,1.,4.47619207437002E-16)) ;
#86320=DIRECTION('center_axis',(0.,0.,1.)) ;
#86321=DIRECTION('ref_axis',(1.,0.,0.)) ;
#86322=DIRECTION('center_axis',(1.,-3.46944695195361E-16,0.)) ;
#86323=DIRECTION('ref_axis',(3.46944695195361E-16,1.,0.)) ;
#86324=DIRECTION('center_axis',(-1.,3.46944695195361E-16,0.)) ;
#86325=DIRECTION('ref_axis',(3.46944695195361E-16,1.,3.46944695195362E-14)) ;
#86326=DIRECTION('center_axis',(1.,-3.46944695195361E-16,0.)) ;
#86327=DIRECTION('ref_axis',(3.41607084500048E-16,1.,0.)) ;
#86328=DIRECTION('center_axis',(0.,0.459459459459457,-0.888198741900271)) ;
#86329=DIRECTION('ref_axis',(0.,0.888198741900271,0.459459459459457)) ;
#86330=DIRECTION('center_axis',(0.,0.,1.)) ;
#86331=DIRECTION('ref_axis',(1.,0.,0.)) ;
#86332=DIRECTION('center_axis',(0.,0.,-1.)) ;
#86333=DIRECTION('ref_axis',(-1.,0.,0.)) ;
#86334=DIRECTION('center_axis',(-1.,3.46944695195361E-16,0.)) ;
#86335=DIRECTION('ref_axis',(-3.46944695195361E-16,-1.,0.)) ;
#86336=DIRECTION('center_axis',(-1.,3.46944695195361E-16,0.)) ;
#86337=DIRECTION('ref_axis',(-3.46944695195361E-16,-1.,0.)) ;
#86338=DIRECTION('center_axis',(-1.,3.46944695195361E-16,0.)) ;
#86339=DIRECTION('ref_axis',(3.46944695195361E-16,1.,6.93889390390722E-14)) ;
#86340=DIRECTION('center_axis',(1.,-3.46944695195361E-16,0.)) ;
#86341=DIRECTION('ref_axis',(0.,1.,0.)) ;
#86342=DIRECTION('center_axis',(0.,-0.888198741900269,0.459459459459461)) ;
#86343=DIRECTION('ref_axis',(0.,0.459459459459461,0.888198741900269)) ;
#86344=DIRECTION('center_axis',(0.,1.,0.)) ;
#86345=DIRECTION('ref_axis',(1.,0.,0.)) ;
#86346=DIRECTION('center_axis',(0.,1.,0.)) ;
#86347=DIRECTION('ref_axis',(0.,0.,-1.)) ;
#86348=DIRECTION('center_axis',(-1.,0.,0.)) ;
#86349=DIRECTION('ref_axis',(0.,-8.67361737988409E-15,-1.)) ;
#86350=DIRECTION('center_axis',(1.,-3.46944695195361E-16,0.)) ;
#86351=DIRECTION('ref_axis',(3.70074341541719E-16,1.,0.)) ;
#86352=DIRECTION('center_axis',(0.,0.63294893130157,-0.774193548387094)) ;
#86353=DIRECTION('ref_axis',(-1.08420217248549E-15,-0.774193548387094,-0.63294893130157)) ;
#86354=DIRECTION('center_axis',(1.,-3.46944695195361E-16,0.)) ;
#86355=DIRECTION('ref_axis',(3.80647894157197E-16,1.,0.)) ;
#86356=DIRECTION('center_axis',(0.,-0.45945945945946,0.888198741900269)) ;
#86357=DIRECTION('ref_axis',(0.,-0.888198741900269,-0.45945945945946)) ;
#86358=DIRECTION('center_axis',(1.,-3.46944695195361E-16,0.)) ;
#86359=DIRECTION('ref_axis',(3.46944695195361E-16,1.,0.)) ;
#86360=DIRECTION('center_axis',(-1.,3.46944695195361E-16,0.)) ;
#86361=DIRECTION('ref_axis',(3.46944695195361E-16,1.,0.)) ;
#86362=DIRECTION('center_axis',(-3.46944695195361E-16,-1.,-2.45739631480277E-16)) ;
#86363=DIRECTION('ref_axis',(1.,-3.46944695195361E-16,-8.52580615413453E-32)) ;
#86364=DIRECTION('center_axis',(0.,1.,0.)) ;
#86365=DIRECTION('ref_axis',(0.,0.,1.)) ;
#86366=DIRECTION('center_axis',(1.,-3.46944695195361E-16,0.)) ;
#86367=DIRECTION('ref_axis',(3.33066907387547E-16,1.,0.)) ;
#86368=DIRECTION('center_axis',(8.02036034720251E-16,0.293103448275862,
-0.956080733311157)) ;
#86369=DIRECTION('ref_axis',(1.13164713162994E-29,0.956080733311157,0.293103448275862)) ;
#86370=DIRECTION('center_axis',(-1.,3.46944695195361E-16,0.)) ;
#86371=DIRECTION('ref_axis',(-3.46944695195361E-16,-1.,0.)) ;
#86372=DIRECTION('center_axis',(-1.,3.46944695195361E-16,0.)) ;
#86373=DIRECTION('ref_axis',(-3.46944695195361E-16,-1.,0.)) ;
#86374=DIRECTION('center_axis',(-1.,3.46944695195361E-16,0.)) ;
#86375=DIRECTION('ref_axis',(-3.46944695195361E-16,-1.,0.)) ;
#86376=DIRECTION('center_axis',(0.,0.,-1.)) ;
#86377=DIRECTION('ref_axis',(-1.,0.,0.)) ;
#86378=DIRECTION('center_axis',(0.,0.,1.)) ;
#86379=DIRECTION('ref_axis',(1.,0.,0.)) ;
#86380=DIRECTION('center_axis',(-1.5529910948782E-31,-4.47619207437002E-16,
-1.)) ;
#86381=DIRECTION('ref_axis',(-6.95148643046101E-47,1.,-4.47619207437002E-16)) ;
#86382=DIRECTION('center_axis',(2.16840434497101E-15,0.,1.)) ;
#86383=DIRECTION('ref_axis',(1.,0.,-2.16840434497101E-15)) ;
#86384=DIRECTION('center_axis',(1.,-3.46944695195361E-16,0.)) ;
#86385=DIRECTION('ref_axis',(0.,1.,0.)) ;
#86386=DIRECTION('center_axis',(0.,-1.,0.)) ;
#86387=DIRECTION('ref_axis',(0.,0.,1.)) ;
#86388=DIRECTION('center_axis',(0.577350269189627,0.577350269189627,0.577350269189623)) ;
#86389=DIRECTION('ref_axis',(-0.707106781186548,2.22044604925032E-15,0.707106781186547)) ;
#86390=DIRECTION('center_axis',(-1.,3.46944695195361E-16,0.)) ;
#86391=DIRECTION('ref_axis',(-3.70074341541719E-16,-1.,0.)) ;
#86392=DIRECTION('center_axis',(0.,0.63294893130157,0.774193548387094)) ;
#86393=DIRECTION('ref_axis',(0.,0.774193548387094,-0.63294893130157)) ;
#86394=DIRECTION('center_axis',(0.,1.,0.)) ;
#86395=DIRECTION('ref_axis',(1.,0.,0.)) ;
#86396=DIRECTION('center_axis',(-1.,0.,0.)) ;
#86397=DIRECTION('ref_axis',(0.,3.46944695195364E-14,-1.)) ;
#86398=DIRECTION('center_axis',(0.,0.888198741900271,0.459459459459457)) ;
#86399=DIRECTION('ref_axis',(-1.08420217248551E-15,0.459459459459457,-0.888198741900271)) ;
#86400=DIRECTION('center_axis',(3.46944695195361E-16,1.,2.45739631480277E-16)) ;
#86401=DIRECTION('ref_axis',(-1.,3.46944695195361E-16,8.52580615413453E-32)) ;
#86402=DIRECTION('center_axis',(-1.,3.46944695195361E-16,0.)) ;
#86403=DIRECTION('ref_axis',(-3.33066907387547E-16,-1.,0.)) ;
#86404=DIRECTION('center_axis',(0.,0.293103448275864,0.956080733311156)) ;
#86405=DIRECTION('ref_axis',(0.,-0.956080733311156,0.293103448275864)) ;
#86406=DIRECTION('center_axis',(-3.46944695195361E-16,-1.,-1.06487173641454E-15)) ;
#86407=DIRECTION('ref_axis',(3.69451600012496E-31,1.06487173641454E-15,
-1.)) ;
#86408=DIRECTION('center_axis',(0.,-1.,0.)) ;
#86409=DIRECTION('ref_axis',(0.,0.,-1.)) ;
#86410=DIRECTION('center_axis',(0.,1.,0.)) ;
#86411=DIRECTION('ref_axis',(0.,0.,1.)) ;
#86412=DIRECTION('center_axis',(-1.,3.46944695195361E-16,0.)) ;
#86413=DIRECTION('ref_axis',(-3.41607084500048E-16,-1.,0.)) ;
#86414=DIRECTION('center_axis',(-4.88154879316133E-15,0.45945945945946,
0.888198741900269)) ;
#86415=DIRECTION('ref_axis',(-3.39148554690438E-29,-0.888198741900269,0.45945945945946)) ;
#86416=DIRECTION('center_axis',(1.,-3.46944695195361E-16,0.)) ;
#86417=DIRECTION('ref_axis',(3.46944695195361E-16,1.,0.)) ;
#86418=DIRECTION('center_axis',(-1.,3.46944695195361E-16,0.)) ;
#86419=DIRECTION('ref_axis',(3.46944695195361E-16,1.,0.)) ;
#86420=DIRECTION('center_axis',(-1.5529910948782E-31,-4.47619207437002E-16,
-1.)) ;
#86421=DIRECTION('ref_axis',(-6.95148643046101E-47,1.,-4.47619207437002E-16)) ;
#86422=DIRECTION('center_axis',(0.,0.,-1.)) ;
#86423=DIRECTION('ref_axis',(-1.,0.,0.)) ;
#86424=DIRECTION('center_axis',(0.,0.224137931034483,-0.974557431797419)) ;
#86425=DIRECTION('ref_axis',(0.,-0.974557431797419,-0.224137931034483)) ;
#86426=DIRECTION('center_axis',(0.577350269189627,0.577350269189627,0.577350269189623)) ;
#86427=DIRECTION('ref_axis',(-0.707106781186548,2.22044604925032E-15,0.707106781186547)) ;
#86428=DIRECTION('center_axis',(0.408248290463864,-0.816496580927725,0.408248290463864)) ;
#86429=DIRECTION('ref_axis',(0.707106781186545,-2.77555756156289E-15,-0.70710678118655)) ;
#86430=DIRECTION('center_axis',(0.,1.,0.)) ;
#86431=DIRECTION('ref_axis',(1.,0.,0.)) ;
#86432=DIRECTION('center_axis',(-1.,0.,0.)) ;
#86433=DIRECTION('ref_axis',(0.,0.,-1.)) ;
#86434=DIRECTION('center_axis',(1.,-3.46944695195361E-16,0.)) ;
#86435=DIRECTION('ref_axis',(0.,1.,0.)) ;
#86436=DIRECTION('center_axis',(9.96293888229924E-16,-0.888198741900269,
-0.45945945945946)) ;
#86437=DIRECTION('ref_axis',(-3.00809911926502E-30,-0.45945945945946,0.888198741900269)) ;
#86438=DIRECTION('center_axis',(1.,-3.46944695195361E-16,0.)) ;
#86439=DIRECTION('ref_axis',(-3.70074341541719E-16,-1.,-1.1842378929335E-15)) ;
#86440=DIRECTION('center_axis',(1.58436874053304E-16,-0.224137931034483,
-0.974557431797419)) ;
#86441=DIRECTION('ref_axis',(-2.46331010218511E-30,0.974557431797419,-0.224137931034483)) ;
#86442=DIRECTION('center_axis',(1.,-3.46944695195361E-16,0.)) ;
#86443=DIRECTION('ref_axis',(3.46944695195361E-16,1.,0.)) ;
#86444=DIRECTION('center_axis',(-1.,3.46944695195361E-16,0.)) ;
#86445=DIRECTION('ref_axis',(3.46944695195361E-16,1.,0.)) ;
#86446=DIRECTION('center_axis',(1.,-3.46944695195361E-16,0.)) ;
#86447=DIRECTION('ref_axis',(3.80647894157197E-16,1.,0.)) ;
#86448=DIRECTION('center_axis',(0.,-0.45945945945946,-0.888198741900269)) ;
#86449=DIRECTION('ref_axis',(0.,0.888198741900269,-0.45945945945946)) ;
#86450=DIRECTION('center_axis',(1.,-3.46944695195361E-16,0.)) ;
#86451=DIRECTION('ref_axis',(0.,1.,0.)) ;
#86452=DIRECTION('center_axis',(0.,-1.,0.)) ;
#86453=DIRECTION('ref_axis',(0.,0.,1.)) ;
#86454=DIRECTION('center_axis',(-3.46944695195361E-16,-1.,-1.06487173641454E-15)) ;
#86455=DIRECTION('ref_axis',(3.69451600012496E-31,1.06487173641454E-15,
-1.)) ;
#86456=DIRECTION('center_axis',(0.,0.,1.)) ;
#86457=DIRECTION('ref_axis',(1.,0.,0.)) ;
#86458=DIRECTION('center_axis',(0.,-1.,0.)) ;
#86459=DIRECTION('ref_axis',(0.,0.,-1.)) ;
#86460=DIRECTION('center_axis',(0.,-1.,0.)) ;
#86461=DIRECTION('ref_axis',(0.,0.,-1.)) ;
#86462=DIRECTION('center_axis',(0.,1.,0.)) ;
#86463=DIRECTION('ref_axis',(0.,0.,-1.)) ;
#86464=DIRECTION('center_axis',(0.,0.,1.)) ;
#86465=DIRECTION('ref_axis',(1.,0.,0.)) ;
#86466=DIRECTION('center_axis',(8.67361737988404E-15,-1.,0.)) ;
#86467=DIRECTION('ref_axis',(1.,8.67361737988404E-15,0.)) ;
#86468=DIRECTION('center_axis',(0.497468338163091,-0.710669054518702,0.497468338163091)) ;
#86469=DIRECTION('ref_axis',(0.81923192051904,0.573462344363328,8.04804396179112E-16)) ;
#86470=DIRECTION('center_axis',(0.497468338163091,-0.710669054518702,0.497468338163091)) ;
#86471=DIRECTION('ref_axis',(0.81923192051904,0.573462344363328,7.6535433881835E-16)) ;
#86472=DIRECTION('center_axis',(0.497468338163092,-0.7106690545187,0.497468338163092)) ;
#86473=DIRECTION('ref_axis',(-1.24903860074368E-15,-0.57346234436333,-0.819231920519039)) ;
#86474=DIRECTION('center_axis',(0.,0.,1.)) ;
#86475=DIRECTION('ref_axis',(1.,0.,0.)) ;
#86476=DIRECTION('center_axis',(0.,-1.,0.)) ;
#86477=DIRECTION('ref_axis',(0.,0.,-1.)) ;
#86478=DIRECTION('center_axis',(0.,1.,0.)) ;
#86479=DIRECTION('ref_axis',(0.,0.,1.)) ;
#86480=DIRECTION('center_axis',(0.,1.,0.)) ;
#86481=DIRECTION('ref_axis',(0.,0.,1.)) ;
#86482=DIRECTION('center_axis',(0.,1.,0.)) ;
#86483=DIRECTION('ref_axis',(1.,0.,0.)) ;
#86484=DIRECTION('center_axis',(-1.98515611757154E-15,0.,1.)) ;
#86485=DIRECTION('ref_axis',(-1.,0.,-1.98515611757154E-15)) ;
#86486=DIRECTION('center_axis',(1.,-4.06575814682065E-16,2.84603070277446E-16)) ;
#86487=DIRECTION('ref_axis',(-4.06575814682065E-16,-1.,6.48893816316174E-47)) ;
#86488=DIRECTION('center_axis',(0.,1.,0.)) ;
#86489=DIRECTION('ref_axis',(0.,0.,1.)) ;
#86490=DIRECTION('center_axis',(0.,1.,0.)) ;
#86491=DIRECTION('ref_axis',(0.,0.,1.)) ;
#86492=DIRECTION('center_axis',(0.497468338163091,0.710669054518702,-0.497468338163091)) ;
#86493=DIRECTION('ref_axis',(-0.81923192051904,0.573462344363328,7.6535433881835E-16)) ;
#86494=DIRECTION('center_axis',(-0.497468338163091,-0.710669054518702,0.497468338163091)) ;
#86495=DIRECTION('ref_axis',(-0.81923192051904,0.573462344363329,2.81956803083991E-15)) ;
#86496=DIRECTION('center_axis',(-0.497468338163093,-0.7106690545187,0.497468338163091)) ;
#86497=DIRECTION('ref_axis',(0.819231920519039,-0.573462344363331,1.48853464230757E-16)) ;
#86498=DIRECTION('center_axis',(1.,0.,0.)) ;
#86499=DIRECTION('ref_axis',(0.,0.,-1.)) ;
#86500=DIRECTION('center_axis',(1.,0.,-9.9257805878577E-16)) ;
#86501=DIRECTION('ref_axis',(-9.9257805878577E-16,0.,-1.)) ;
#86502=DIRECTION('center_axis',(0.,0.,-1.)) ;
#86503=DIRECTION('ref_axis',(-1.,0.,0.)) ;
#86504=DIRECTION('center_axis',(-1.23327997120227E-15,1.76182853028895E-15,
1.)) ;
#86505=DIRECTION('ref_axis',(-2.17282783909808E-30,-1.,1.76182853028895E-15)) ;
#86506=DIRECTION('center_axis',(-0.497468338163091,0.710669054518702,0.497468338163091)) ;
#86507=DIRECTION('ref_axis',(-0.81923192051904,-0.573462344363328,7.6535433881835E-16)) ;
#86508=DIRECTION('center_axis',(0.497468338163091,-0.710669054518702,-0.497468338163091)) ;
#86509=DIRECTION('ref_axis',(-0.81923192051904,-0.57346234436333,3.28127423742392E-15)) ;
#86510=DIRECTION('center_axis',(0.497468338163093,-0.7106690545187,-0.497468338163091)) ;
#86511=DIRECTION('ref_axis',(0.819231920519039,0.573462344363331,2.16059097207149E-16)) ;
#86512=DIRECTION('center_axis',(0.,1.,0.)) ;
#86513=DIRECTION('ref_axis',(1.,0.,0.)) ;
#86514=DIRECTION('center_axis',(-1.13841228110978E-15,-1.62630325872826E-15,
1.)) ;
#86515=DIRECTION('ref_axis',(3.52365706057789E-15,1.,1.62630325872826E-15)) ;
#86516=DIRECTION('center_axis',(0.,1.,0.)) ;
#86517=DIRECTION('ref_axis',(1.,0.,0.)) ;
#86518=DIRECTION('center_axis',(1.,0.,-1.65429676464295E-16)) ;
#86519=DIRECTION('ref_axis',(1.65429676464295E-16,2.60208521396523E-14,
1.)) ;
#86520=DIRECTION('center_axis',(0.,0.,-1.)) ;
#86521=DIRECTION('ref_axis',(-1.,0.,0.)) ;
#86522=DIRECTION('center_axis',(3.3085935292859E-16,0.,1.)) ;
#86523=DIRECTION('ref_axis',(1.,0.,-3.3085935292859E-16)) ;
#86524=DIRECTION('center_axis',(1.,0.,0.)) ;
#86525=DIRECTION('ref_axis',(0.,0.,-1.)) ;
#86526=DIRECTION('center_axis',(1.,1.21972744404619E-15,8.53809210832338E-16)) ;
#86527=DIRECTION('ref_axis',(-1.21972744404619E-15,1.,-2.84382165153726E-47)) ;
#86528=DIRECTION('center_axis',(0.,1.,0.)) ;
#86529=DIRECTION('ref_axis',(1.,0.,0.)) ;
#86530=DIRECTION('center_axis',(0.497468338163092,0.710669054518701,0.497468338163092)) ;
#86531=DIRECTION('ref_axis',(1.16990632765504E-14,0.573462344363324,-0.819231920519044)) ;
#86532=DIRECTION('center_axis',(-0.497468338163091,-0.710669054518702,-0.497468338163091)) ;
#86533=DIRECTION('ref_axis',(0.81923192051904,-0.573462344363328,7.6535433881835E-16)) ;
#86534=DIRECTION('center_axis',(-0.497468338163091,-0.710669054518702,-0.497468338163091)) ;
#86535=DIRECTION('ref_axis',(0.81923192051904,-0.573462344363328,7.6535433881835E-16)) ;
#86536=DIRECTION('center_axis',(0.,-1.,0.)) ;
#86537=DIRECTION('ref_axis',(0.,0.,-1.)) ;
#86538=DIRECTION('center_axis',(0.,1.,0.)) ;
#86539=DIRECTION('ref_axis',(0.,0.,-1.)) ;
#86540=DIRECTION('center_axis',(-8.67361737988403E-15,1.,0.)) ;
#86541=DIRECTION('ref_axis',(-1.,-8.67361737988403E-15,0.)) ;
#86542=DIRECTION('center_axis',(0.,0.,1.)) ;
#86543=DIRECTION('ref_axis',(1.,0.,0.)) ;
#86544=DIRECTION('center_axis',(1.,6.67201336914158E-17,0.)) ;
#86545=DIRECTION('ref_axis',(-6.67201336914158E-17,1.,0.)) ;
#86546=DIRECTION('center_axis',(-1.,-6.67201336914158E-17,0.)) ;
#86547=DIRECTION('ref_axis',(-6.67201336914158E-17,1.,0.)) ;
#86548=DIRECTION('center_axis',(-1.,1.33440267382831E-16,0.)) ;
#86549=DIRECTION('ref_axis',(-1.33440267382831E-16,-1.,0.)) ;
#86550=DIRECTION('center_axis',(-1.,1.33440267382831E-16,0.)) ;
#86551=DIRECTION('ref_axis',(-1.33440267382831E-16,-1.,0.)) ;
#86552=DIRECTION('center_axis',(0.710669054518702,0.497468338163091,0.497468338163091)) ;
#86553=DIRECTION('ref_axis',(-0.573462344363328,0.819231920519041,3.92980824865032E-16)) ;
#86554=DIRECTION('center_axis',(0.710669054518702,0.497468338163091,0.497468338163091)) ;
#86555=DIRECTION('ref_axis',(-0.573462344363328,0.819231920519041,3.92980824865032E-16)) ;
#86556=DIRECTION('center_axis',(0.710669054518701,0.497468338163091,0.497468338163092)) ;
#86557=DIRECTION('ref_axis',(0.57346234436333,-1.81382726107456E-15,-0.819231920519039)) ;
#86558=DIRECTION('center_axis',(-0.710669054518702,0.497468338163091,-0.497468338163091)) ;
#86559=DIRECTION('ref_axis',(-0.573462344363328,-0.819231920519041,6.69271761853466E-16)) ;
#86560=DIRECTION('center_axis',(0.710669054518702,-0.497468338163091,0.497468338163091)) ;
#86561=DIRECTION('ref_axis',(-0.573462344363328,-0.819231920519041,6.69271761853466E-16)) ;
#86562=DIRECTION('center_axis',(0.7106690545187,-0.497468338163094,0.497468338163091)) ;
#86563=DIRECTION('ref_axis',(0.573462344363331,0.819231920519038,2.86772422505918E-16)) ;
#86564=DIRECTION('center_axis',(0.,1.,-9.34081871679819E-17)) ;
#86565=DIRECTION('ref_axis',(0.,9.34081871679819E-17,1.)) ;
#86566=DIRECTION('center_axis',(-4.33680868994205E-15,-1.,-3.03576608295944E-15)) ;
#86567=DIRECTION('ref_axis',(1.,-4.33680868994205E-15,-1.12103877145985E-44)) ;
#86568=DIRECTION('center_axis',(0.,1.,5.29374964685745E-15)) ;
#86569=DIRECTION('ref_axis',(0.,-5.29374964685745E-15,1.)) ;
#86570=DIRECTION('center_axis',(0.,1.,0.)) ;
#86571=DIRECTION('ref_axis',(1.,0.,0.)) ;
#86572=DIRECTION('center_axis',(0.,6.45175738210751E-15,1.)) ;
#86573=DIRECTION('ref_axis',(0.,1.,-6.45175738210751E-15)) ;
#86574=DIRECTION('center_axis',(-1.,-6.67201336914158E-17,0.)) ;
#86575=DIRECTION('ref_axis',(6.67201336914158E-17,-1.,0.)) ;
#86576=DIRECTION('center_axis',(-1.,-6.67201336914158E-17,0.)) ;
#86577=DIRECTION('ref_axis',(6.67201336914158E-17,-1.,0.)) ;
#86578=DIRECTION('center_axis',(1.,-1.33440267382831E-16,0.)) ;
#86579=DIRECTION('ref_axis',(1.33440267382831E-16,1.,0.)) ;
#86580=DIRECTION('center_axis',(-1.,1.33440267382831E-16,0.)) ;
#86581=DIRECTION('ref_axis',(1.33440267382831E-16,1.,0.)) ;
#86582=DIRECTION('center_axis',(0.,1.,0.)) ;
#86583=DIRECTION('ref_axis',(1.,0.,0.)) ;
#86584=DIRECTION('center_axis',(1.76182853028896E-15,-1.23327997120227E-15,
1.)) ;
#86585=DIRECTION('ref_axis',(-1.,-2.1728278390981E-30,1.76182853028896E-15)) ;
#86586=DIRECTION('center_axis',(0.,0.,-1.)) ;
#86587=DIRECTION('ref_axis',(-1.,0.,0.)) ;
#86588=DIRECTION('center_axis',(-2.71050543121378E-16,-1.89735380184965E-16,
1.)) ;
#86589=DIRECTION('ref_axis',(1.,-5.14278778484758E-32,2.71050543121378E-16)) ;
#86590=DIRECTION('center_axis',(-0.710669054518702,-0.497468338163091,0.497468338163091)) ;
#86591=DIRECTION('ref_axis',(0.573462344363328,-0.819231920519041,3.92980824865032E-16)) ;
#86592=DIRECTION('center_axis',(0.710669054518702,0.497468338163091,-0.497468338163091)) ;
#86593=DIRECTION('ref_axis',(0.573462344363345,-0.819231920519029,3.5916041727749E-14)) ;
#86594=DIRECTION('center_axis',(0.710669054518701,0.497468338163091,-0.497468338163092)) ;
#86595=DIRECTION('ref_axis',(-0.57346234436333,1.88103289405095E-15,-0.819231920519039)) ;
#86596=DIRECTION('center_axis',(0.710669054518702,-0.497468338163091,-0.497468338163091)) ;
#86597=DIRECTION('ref_axis',(0.573462344363328,0.819231920519041,6.69271761853466E-16)) ;
#86598=DIRECTION('center_axis',(0.710669054518702,-0.497468338163091,-0.497468338163091)) ;
#86599=DIRECTION('ref_axis',(0.573462344363328,0.819231920519041,6.69271761853466E-16)) ;
#86600=DIRECTION('center_axis',(0.7106690545187,-0.497468338163091,-0.497468338163093)) ;
#86601=DIRECTION('ref_axis',(-0.573462344363331,-1.17187023180681E-15,-0.819231920519038)) ;
#86602=DIRECTION('center_axis',(0.,0.,-1.)) ;
#86603=DIRECTION('ref_axis',(-1.,0.,0.)) ;
#86604=DIRECTION('center_axis',(0.,1.15800773525007E-15,1.)) ;
#86605=DIRECTION('ref_axis',(0.,-1.,1.15800773525007E-15)) ;
#86606=DIRECTION('center_axis',(0.,1.,0.)) ;
#86607=DIRECTION('ref_axis',(1.,0.,0.)) ;
#86608=DIRECTION('center_axis',(0.,1.,0.)) ;
#86609=DIRECTION('ref_axis',(1.04083408558609E-13,0.,-1.)) ;
#86610=DIRECTION('center_axis',(0.,1.,0.)) ;
#86611=DIRECTION('ref_axis',(1.,0.,0.)) ;
#86612=DIRECTION('center_axis',(4.33680868994204E-15,-1.,-3.03576608295944E-15)) ;
#86613=DIRECTION('ref_axis',(-1.,-4.33680868994225E-15,6.93889390390727E-14)) ;
#86614=DIRECTION('center_axis',(0.,1.,9.34081871679819E-17)) ;
#86615=DIRECTION('ref_axis',(0.,-9.34081871679819E-17,1.)) ;
#86616=DIRECTION('center_axis',(0.,0.,1.)) ;
#86617=DIRECTION('ref_axis',(1.,0.,0.)) ;
#86618=DIRECTION('center_axis',(-2.16840434497102E-15,-3.61400724161847E-16,
1.)) ;
#86619=DIRECTION('ref_axis',(1.,-7.83662900548222E-31,2.16840434497102E-15)) ;
#86620=DIRECTION('center_axis',(0.973328526784575,0.162221421130762,-0.162221421130763)) ;
#86621=DIRECTION('ref_axis',(-0.164398987305358,9.23743777622416E-16,-0.986393923832144)) ;
#86622=DIRECTION('center_axis',(0.973328526784574,0.162221421130765,-0.162221421130767)) ;
#86623=DIRECTION('ref_axis',(-0.164398987305362,1.88956506020588E-16,-0.986393923832143)) ;
#86624=DIRECTION('center_axis',(0.,1.,0.)) ;
#86625=DIRECTION('ref_axis',(1.,0.,0.)) ;
#86626=DIRECTION('center_axis',(0.,1.,-8.79325913341701E-15)) ;
#86627=DIRECTION('ref_axis',(1.73472347597682E-14,-8.79325913341701E-15,
-1.)) ;
#86628=DIRECTION('center_axis',(0.,0.,1.)) ;
#86629=DIRECTION('ref_axis',(1.,0.,0.)) ;
#86630=DIRECTION('center_axis',(0.,-2.28569887277128E-15,1.)) ;
#86631=DIRECTION('ref_axis',(0.,-1.,-2.28569887277128E-15)) ;
#86632=DIRECTION('center_axis',(1.73472347597681E-15,-1.,-2.89120579329468E-16)) ;
#86633=DIRECTION('ref_axis',(1.,1.73472347597681E-15,5.01544256350843E-31)) ;
#86634=DIRECTION('center_axis',(8.67361737988409E-15,1.,-1.44560289664739E-15)) ;
#86635=DIRECTION('ref_axis',(-1.,8.67361737988409E-15,-1.40129846432482E-45)) ;
#86636=DIRECTION('center_axis',(0.,1.,0.)) ;
#86637=DIRECTION('ref_axis',(1.,0.,0.)) ;
#86638=DIRECTION('center_axis',(-0.937042571331634,0.312347523777217,0.156173761888611)) ;
#86639=DIRECTION('ref_axis',(0.316227766016843,0.948683298050512,6.71158276827649E-18)) ;
#86640=DIRECTION('center_axis',(0.937042571331636,-0.312347523777212,-0.156173761888606)) ;
#86641=DIRECTION('ref_axis',(0.316227766016838,0.948683298050514,8.61595672567599E-16)) ;
#86642=DIRECTION('center_axis',(-0.973328526784575,-0.162221421130762,-0.162221421130763)) ;
#86643=DIRECTION('ref_axis',(-0.164398987305358,9.23743777622416E-16,0.986393923832144)) ;
#86644=DIRECTION('center_axis',(0.978231976292088,-0.146734796047319,-0.146734795425719)) ;
#86645=DIRECTION('ref_axis',(0.182318633536231,0.945435290940488,0.270022270395899)) ;
#86646=DIRECTION('center_axis',(0.973328526784574,0.162221421130767,0.162221421130768)) ;
#86647=DIRECTION('ref_axis',(0.164398987305363,-6.69215935033609E-18,-0.986393923832143)) ;
#86648=DIRECTION('center_axis',(0.,0.,1.)) ;
#86649=DIRECTION('ref_axis',(1.,0.,0.)) ;
#86650=DIRECTION('center_axis',(0.,2.19831478335425E-15,-1.)) ;
#86651=DIRECTION('ref_axis',(0.,1.,2.19831478335425E-15)) ;
#86652=DIRECTION('center_axis',(0.,1.,0.)) ;
#86653=DIRECTION('ref_axis',(1.,0.,0.)) ;
#86654=DIRECTION('center_axis',(8.67361737988408E-15,1.,1.44560289664739E-15)) ;
#86655=DIRECTION('ref_axis',(1.,-8.67361737988408E-15,5.60519385729927E-45)) ;
#86656=DIRECTION('center_axis',(1.73472347597681E-15,-1.,2.89120579329468E-16)) ;
#86657=DIRECTION('ref_axis',(1.,1.73472347597681E-15,-5.01544256350843E-31)) ;
#86658=DIRECTION('center_axis',(0.,1.,0.)) ;
#86659=DIRECTION('ref_axis',(0.,0.,1.)) ;
#86660=DIRECTION('center_axis',(0.,0.,1.)) ;
#86661=DIRECTION('ref_axis',(1.,0.,0.)) ;
#86662=DIRECTION('center_axis',(3.25260651745652E-15,-1.08420217248553E-15,
-1.)) ;
#86663=DIRECTION('ref_axis',(-1.,-3.52648305246695E-30,-3.25260651745652E-15)) ;
#86664=DIRECTION('center_axis',(0.,1.,0.)) ;
#86665=DIRECTION('ref_axis',(1.,0.,0.)) ;
#86666=DIRECTION('center_axis',(-0.937042571331635,0.312347523777215,-0.15617376188861)) ;
#86667=DIRECTION('ref_axis',(0.316227766016841,0.948683298050513,6.5590042956861E-18)) ;
#86668=DIRECTION('center_axis',(-0.937042571331636,0.312347523777212,-0.156173761888606)) ;
#86669=DIRECTION('ref_axis',(0.331350514299552,0.654034959159455,-0.680033167478405)) ;
#86670=DIRECTION('center_axis',(0.96151972409117,0.245047216428555,-0.124224320904791)) ;
#86671=DIRECTION('ref_axis',(0.262092069886556,-0.68255472816298,0.68222195066191)) ;
#86672=DIRECTION('center_axis',(2.65552944032596E-32,3.29043518662928E-48,
-1.)) ;
#86673=DIRECTION('ref_axis',(-1.,8.7378475095785E-80,-2.65552944032596E-32)) ;
#86674=DIRECTION('center_axis',(2.65552944032596E-32,3.29043518662928E-48,
-1.)) ;
#86675=DIRECTION('ref_axis',(-1.,8.7378475095785E-80,-2.65552944032596E-32)) ;
#86676=DIRECTION('center_axis',(-2.65552944032596E-32,-3.29043518662928E-48,
1.)) ;
#86677=DIRECTION('ref_axis',(-1.,8.7378475095785E-80,-2.65552944032596E-32)) ;
#86678=DIRECTION('center_axis',(0.,0.,1.)) ;
#86679=DIRECTION('ref_axis',(1.,0.,0.)) ;
#86680=DIRECTION('center_axis',(0.,0.,-1.)) ;
#86681=DIRECTION('ref_axis',(-1.,0.,0.)) ;
#86682=DIRECTION('center_axis',(0.,0.,1.)) ;
#86683=DIRECTION('ref_axis',(1.,0.,0.)) ;
#86684=DIRECTION('center_axis',(0.,0.,1.)) ;
#86685=DIRECTION('ref_axis',(1.,0.,0.)) ;
#86686=DIRECTION('center_axis',(0.,0.,-1.)) ;
#86687=DIRECTION('ref_axis',(-1.,0.,0.)) ;
#86688=DIRECTION('center_axis',(0.,0.,-1.)) ;
#86689=DIRECTION('ref_axis',(-1.,0.,0.)) ;
#86690=DIRECTION('center_axis',(1.,1.15648231731787E-15,0.)) ;
#86691=DIRECTION('ref_axis',(1.03435541192675E-15,-1.,0.)) ;
#86692=DIRECTION('center_axis',(7.089177613099E-16,-0.612994899008946,-0.790086864711098)) ;
#86693=DIRECTION('ref_axis',(-5.20417042793041E-14,-0.790086864711098,0.612994899008946)) ;
#86694=DIRECTION('center_axis',(7.08917761309899E-16,-0.612994899008945,
0.790086864711098)) ;
#86695=DIRECTION('ref_axis',(-3.46944695195361E-14,0.790086864711098,0.612994899008945)) ;
#86696=DIRECTION('center_axis',(0.,0.,-1.)) ;
#86697=DIRECTION('ref_axis',(-1.,0.,0.)) ;
#86698=DIRECTION('center_axis',(0.,0.,1.)) ;
#86699=DIRECTION('ref_axis',(-1.,2.16840434497102E-15,0.)) ;
#86700=DIRECTION('center_axis',(1.08420217248551E-15,-1.,0.)) ;
#86701=DIRECTION('ref_axis',(1.,1.08420217248551E-15,0.)) ;
#86702=DIRECTION('center_axis',(1.44560289664734E-16,-1.,-2.4093381610789E-16)) ;
#86703=DIRECTION('ref_axis',(2.28544744656275E-46,2.4093381610789E-16,-1.)) ;
#86704=DIRECTION('center_axis',(0.,-1.,0.)) ;
#86705=DIRECTION('ref_axis',(0.,0.,-1.)) ;
#86706=DIRECTION('center_axis',(1.,0.,0.)) ;
#86707=DIRECTION('ref_axis',(0.,1.,0.)) ;
#86708=DIRECTION('center_axis',(1.,0.,0.)) ;
#86709=DIRECTION('ref_axis',(0.,0.,-1.)) ;
#86710=DIRECTION('center_axis',(1.,1.23908819712629E-16,8.95614743483648E-33)) ;
#86711=DIRECTION('ref_axis',(-1.23908819712629E-16,1.,-1.10974565782288E-48)) ;
#86712=DIRECTION('center_axis',(1.,0.,0.)) ;
#86713=DIRECTION('ref_axis',(0.,0.,-1.)) ;
#86714=DIRECTION('center_axis',(-1.,0.,0.)) ;
#86715=DIRECTION('ref_axis',(0.,0.,1.)) ;
#86716=DIRECTION('center_axis',(1.,1.23908819712629E-16,8.95614743483648E-33)) ;
#86717=DIRECTION('ref_axis',(-1.23908819712629E-16,1.,-1.10974565782288E-48)) ;
#86718=DIRECTION('center_axis',(-1.,0.,0.)) ;
#86719=DIRECTION('ref_axis',(0.,0.,1.)) ;
#86720=DIRECTION('center_axis',(1.,0.,0.)) ;
#86721=DIRECTION('ref_axis',(0.,-1.,0.)) ;
#86722=DIRECTION('center_axis',(0.,1.,0.)) ;
#86723=DIRECTION('ref_axis',(0.,0.,1.)) ;
#86724=DIRECTION('center_axis',(-1.44560289664734E-16,1.,-7.2280144832367E-17)) ;
#86725=DIRECTION('ref_axis',(0.707106781238304,1.53329341672078E-16,0.707106781134791)) ;
#86726=DIRECTION('center_axis',(-1.0842021724855E-15,1.,0.)) ;
#86727=DIRECTION('ref_axis',(-1.,-1.0842021724855E-15,0.)) ;
#86728=DIRECTION('center_axis',(0.,1.,0.)) ;
#86729=DIRECTION('ref_axis',(0.,0.,1.)) ;
#86730=DIRECTION('center_axis',(0.,-1.,0.)) ;
#86731=DIRECTION('ref_axis',(0.,0.,-1.)) ;
#86732=DIRECTION('center_axis',(0.,1.,0.)) ;
#86733=DIRECTION('ref_axis',(0.,0.,1.)) ;
#86734=DIRECTION('center_axis',(0.,0.,1.)) ;
#86735=DIRECTION('ref_axis',(1.,0.,0.)) ;
#86736=DIRECTION('center_axis',(0.431191646766499,0.0335421424315027,0.901636672080223)) ;
#86737=DIRECTION('ref_axis',(0.899826811355995,0.0573593270524375,-0.432459960187061)) ;
#86738=DIRECTION('center_axis',(0.,0.,1.)) ;
#86739=DIRECTION('ref_axis',(-1.,0.,0.)) ;
#86740=DIRECTION('center_axis',(0.,0.,-1.)) ;
#86741=DIRECTION('ref_axis',(0.707109343403322,-0.707104218960488,0.)) ;
#86742=DIRECTION('center_axis',(-3.25260651745653E-15,0.,1.)) ;
#86743=DIRECTION('ref_axis',(1.,0.,3.25260651745653E-15)) ;
#86744=DIRECTION('center_axis',(0.,0.,1.)) ;
#86745=DIRECTION('ref_axis',(1.,0.,0.)) ;
#86746=DIRECTION('center_axis',(0.431188264324026,0.0335835000973875,-0.901636750155207)) ;
#86747=DIRECTION('ref_axis',(0.899831768145072,0.0572892325739573,0.432458937782537)) ;
#86748=DIRECTION('center_axis',(0.,-1.,0.)) ;
#86749=DIRECTION('ref_axis',(0.,0.,-1.)) ;
#86750=DIRECTION('center_axis',(0.,1.,0.)) ;
#86751=DIRECTION('ref_axis',(0.,0.,1.)) ;
#86752=DIRECTION('center_axis',(0.,0.,1.)) ;
#86753=DIRECTION('ref_axis',(1.,0.,0.)) ;
#86754=DIRECTION('center_axis',(0.,0.,-1.)) ;
#86755=DIRECTION('ref_axis',(-1.,0.,0.)) ;
#86756=DIRECTION('center_axis',(0.,0.,1.)) ;
#86757=DIRECTION('ref_axis',(-0.986393923832144,0.164398987305354,0.)) ;
#86758=DIRECTION('center_axis',(0.98470178743927,-0.164116964573216,0.0585492250433781)) ;
#86759=DIRECTION('ref_axis',(0.164398987305362,0.986393923832143,-7.60669428566932E-17)) ;
#86760=DIRECTION('center_axis',(0.984834538781277,-0.164139089796902,0.0562075655416074)) ;
#86761=DIRECTION('ref_axis',(0.164398987305379,0.98639392383214,1.87706412796466E-17)) ;
#86762=DIRECTION('center_axis',(0.986393923832145,-0.129889480441767,0.100775740620414)) ;
#86763=DIRECTION('ref_axis',(0.,0.612994899008949,0.790086864711095)) ;
#86764=DIRECTION('center_axis',(0.,1.,0.)) ;
#86765=DIRECTION('ref_axis',(1.,0.,0.)) ;
#86766=DIRECTION('center_axis',(0.,0.,-1.)) ;
#86767=DIRECTION('ref_axis',(-1.,0.,0.)) ;
#86768=DIRECTION('center_axis',(1.,2.8359373108165E-15,0.)) ;
#86769=DIRECTION('ref_axis',(-2.8359373108165E-15,1.,0.)) ;
#86770=DIRECTION('center_axis',(0.,0.,-1.)) ;
#86771=DIRECTION('ref_axis',(-1.,0.,0.)) ;
#86772=DIRECTION('center_axis',(0.,0.,1.)) ;
#86773=DIRECTION('ref_axis',(1.,0.,0.)) ;
#86774=DIRECTION('center_axis',(1.,0.,0.)) ;
#86775=DIRECTION('ref_axis',(0.,0.,-1.)) ;
#86776=DIRECTION('center_axis',(1.,0.,0.)) ;
#86777=DIRECTION('ref_axis',(0.,0.,-1.)) ;
#86778=DIRECTION('center_axis',(0.,1.,0.)) ;
#86779=DIRECTION('ref_axis',(1.,0.,0.)) ;
#86780=DIRECTION('center_axis',(1.,-8.50781193244945E-15,0.)) ;
#86781=DIRECTION('ref_axis',(8.50781193244945E-15,1.,0.)) ;
#86782=DIRECTION('center_axis',(0.,1.,0.)) ;
#86783=DIRECTION('ref_axis',(1.,0.,0.)) ;
#86784=DIRECTION('center_axis',(-5.42101086242753E-16,1.70882313734897E-16,
1.)) ;
#86785=DIRECTION('ref_axis',(1.,9.26354878953623E-32,5.42101086242753E-16)) ;
#86786=DIRECTION('center_axis',(-1.,0.,0.)) ;
#86787=DIRECTION('ref_axis',(0.,0.,1.)) ;
#86788=DIRECTION('center_axis',(1.,0.,0.)) ;
#86789=DIRECTION('ref_axis',(0.,0.,-1.)) ;
#86790=DIRECTION('center_axis',(0.,0.,-1.)) ;
#86791=DIRECTION('ref_axis',(-1.,0.,0.)) ;
#86792=DIRECTION('center_axis',(0.,0.,1.)) ;
#86793=DIRECTION('ref_axis',(1.,0.,0.)) ;
#86794=DIRECTION('center_axis',(0.,1.,0.)) ;
#86795=DIRECTION('ref_axis',(1.,0.,0.)) ;
#86796=DIRECTION('center_axis',(0.,1.,0.)) ;
#86797=DIRECTION('ref_axis',(1.,0.,0.)) ;
#86798=DIRECTION('center_axis',(0.,0.,-1.)) ;
#86799=DIRECTION('ref_axis',(-1.,0.,0.)) ;
#86800=DIRECTION('center_axis',(0.,1.,0.)) ;
#86801=DIRECTION('ref_axis',(0.,0.,1.)) ;
#86802=DIRECTION('center_axis',(0.,0.,-1.)) ;
#86803=DIRECTION('ref_axis',(-1.,0.,0.)) ;
#86804=DIRECTION('center_axis',(0.,0.,1.)) ;
#86805=DIRECTION('ref_axis',(1.,0.,0.)) ;
#86806=DIRECTION('center_axis',(1.33440267382831E-16,1.,0.)) ;
#86807=DIRECTION('ref_axis',(-1.,1.33440267382831E-16,0.)) ;
#86808=DIRECTION('center_axis',(0.,1.,0.)) ;
#86809=DIRECTION('ref_axis',(0.,0.,1.)) ;
#86810=DIRECTION('center_axis',(0.,1.,0.)) ;
#86811=DIRECTION('ref_axis',(1.,0.,0.)) ;
#86812=DIRECTION('center_axis',(0.,1.,0.)) ;
#86813=DIRECTION('ref_axis',(0.,0.,1.)) ;
#86814=DIRECTION('center_axis',(0.,1.,0.)) ;
#86815=DIRECTION('ref_axis',(1.,0.,0.)) ;
#86816=DIRECTION('center_axis',(1.37797793267296E-15,-1.62630325872825E-15,
1.)) ;
#86817=DIRECTION('ref_axis',(-2.24101000236165E-30,-1.,-1.62630325872825E-15)) ;
#86818=DIRECTION('center_axis',(-1.33440267382831E-16,-1.,0.)) ;
#86819=DIRECTION('ref_axis',(1.,-1.33440267382831E-16,0.)) ;
#86820=DIRECTION('center_axis',(0.,1.,0.)) ;
#86821=DIRECTION('ref_axis',(0.,0.,1.)) ;
#86822=DIRECTION('center_axis',(0.,0.,-1.)) ;
#86823=DIRECTION('ref_axis',(-1.,0.,0.)) ;
#86824=DIRECTION('center_axis',(0.,0.,1.)) ;
#86825=DIRECTION('ref_axis',(1.,0.,0.)) ;
#86826=DIRECTION('center_axis',(0.,1.,0.)) ;
#86827=DIRECTION('ref_axis',(1.,0.,0.)) ;
#86828=DIRECTION('center_axis',(0.,0.,1.)) ;
#86829=DIRECTION('ref_axis',(1.,0.,0.)) ;
#86830=DIRECTION('center_axis',(0.,0.,1.)) ;
#86831=DIRECTION('ref_axis',(1.,0.,0.)) ;
#86832=DIRECTION('center_axis',(0.,0.,1.)) ;
#86833=DIRECTION('ref_axis',(-0.986393923832144,0.164398987305354,0.)) ;
#86834=DIRECTION('center_axis',(0.984701787439272,-0.164116964573205,-0.0585492250433871)) ;
#86835=DIRECTION('ref_axis',(0.16439898730535,0.986393923832145,-3.2807868055655E-16)) ;
#86836=DIRECTION('center_axis',(0.984834538781259,-0.164139089796881,-0.0562075655419907)) ;
#86837=DIRECTION('ref_axis',(0.164398987305362,0.986393923832143,6.03508511856301E-17)) ;
#86838=DIRECTION('center_axis',(0.,0.,1.)) ;
#86839=DIRECTION('ref_axis',(-0.986393923832144,0.164398987305354,0.)) ;
#86840=DIRECTION('center_axis',(0.,0.,1.)) ;
#86841=DIRECTION('ref_axis',(1.,0.,0.)) ;
#86842=DIRECTION('center_axis',(0.342346838786525,0.100237737278944,-0.934211452508516)) ;
#86843=DIRECTION('ref_axis',(0.878411850175152,0.318727802690732,0.356097190755283)) ;
#86844=DIRECTION('center_axis',(0.,0.,-1.)) ;
#86845=DIRECTION('ref_axis',(-1.,0.,0.)) ;
#86846=DIRECTION('center_axis',(0.,0.,-1.)) ;
#86847=DIRECTION('ref_axis',(-1.,0.,0.)) ;
#86848=DIRECTION('center_axis',(0.,0.,-1.)) ;
#86849=DIRECTION('ref_axis',(-1.,0.,0.)) ;
#86850=DIRECTION('center_axis',(-0.342346838787816,-0.100237737288811,-0.934211452506984)) ;
#86851=DIRECTION('ref_axis',(0.878411919034117,0.318727608050549,-0.356097195109952)) ;
#86852=DIRECTION('center_axis',(0.,0.,1.)) ;
#86853=DIRECTION('ref_axis',(1.,0.,0.)) ;
#101184=CARTESIAN_POINT('',(0.,0.,0.)) ;
#101185=CARTESIAN_POINT('Ctrl Pts',(8.55305389383868,6.58518362856711,0.660183628567108)) ;
#101186=CARTESIAN_POINT('Ctrl Pts',(8.56447181517253,6.58947636230805,0.664476362308047)) ;
#101187=CARTESIAN_POINT('Ctrl Pts',(8.57705842661295,6.59157413088145,0.66657413088145)) ;
#101188=CARTESIAN_POINT('Ctrl Pts',(8.55305102515198,6.55898702014116,0.686379540222498)) ;
#101189=CARTESIAN_POINT('Ctrl Pts',(8.56446969712852,6.56479854221784,0.68915347690881)) ;
#101190=CARTESIAN_POINT('Ctrl Pts',(8.57705842709768,6.56766897765923,0.690479284265246)) ;
#101191=CARTESIAN_POINT('Ctrl Pts',(8.55608440539073,6.54967077654144,0.726527573965357)) ;
#101192=CARTESIAN_POINT('Ctrl Pts',(8.56803673427363,6.55578248257735,0.726868875765167)) ;
#101193=CARTESIAN_POINT('Ctrl Pts',(8.58110225049763,6.55837193275,0.726735153349558)) ;
#101194=CARTESIAN_POINT('Ctrl Pts',(8.56106007075016,6.56033186051354,0.763021538403806)) ;
#101195=CARTESIAN_POINT('Ctrl Pts',(8.57385418571953,6.56560017282096,0.761796116238336)) ;
#101196=CARTESIAN_POINT('Ctrl Pts',(8.58763814880121,6.56727264871055,0.761407094307452)) ;
#101197=CARTESIAN_POINT('',(8.56104219912065,6.56017369985344,0.762366149055595)) ;
#101198=CARTESIAN_POINT('',(8.55704445183394,6.58320973295714,0.665168358807856)) ;
#101199=CARTESIAN_POINT('Ctrl Pts',(8.56104219912065,6.56017369985344,0.762366149055595)) ;
#101200=CARTESIAN_POINT('Ctrl Pts',(8.56172006948825,6.55755272988493,0.749490016573775)) ;
#101201=CARTESIAN_POINT('Ctrl Pts',(8.56178854742204,6.55691761311389,0.735981136540874)) ;
#101202=CARTESIAN_POINT('Ctrl Pts',(8.56147572200372,6.55855061087387,0.722928962845481)) ;
#101203=CARTESIAN_POINT('Ctrl Pts',(8.56116227470662,6.56018685493861,0.709850842186457)) ;
#101204=CARTESIAN_POINT('Ctrl Pts',(8.5604843297899,6.56417103596015,0.696870920866104)) ;
#101205=CARTESIAN_POINT('Ctrl Pts',(8.55945615587251,6.57017322470283,0.685177787303522)) ;
#101206=CARTESIAN_POINT('Ctrl Pts',(8.55883284154061,6.57381195760861,0.678089008244737)) ;
#101207=CARTESIAN_POINT('Ctrl Pts',(8.55807185541709,6.57823677723146,0.671364951604696)) ;
#101208=CARTESIAN_POINT('Ctrl Pts',(8.55704487707426,6.58320791316502,0.665167537880534)) ;
#101209=CARTESIAN_POINT('',(8.55635403291171,6.58636921675996,0.661369767825604)) ;
#101210=CARTESIAN_POINT('Origin',(8.54420289523221,6.6281733287991,0.698058895172689)) ;
#101211=CARTESIAN_POINT('',(8.57705842661295,6.59157413088145,0.66657413088145)) ;
#101212=CARTESIAN_POINT('Origin',(8.6,6.52274941072028,0.597749410720281)) ;
#101213=CARTESIAN_POINT('',(8.58355189313842,6.56397635572684,0.737566223574004)) ;
#101214=CARTESIAN_POINT('Origin',(8.597771292818,6.65641294722129,0.739117764068465)) ;
#101215=CARTESIAN_POINT('Ctrl Pts',(8.56104311409707,6.56017375480331,0.762365190627708)) ;
#101216=CARTESIAN_POINT('Ctrl Pts',(8.56569547918968,6.5609490208508,0.756877613830519)) ;
#101217=CARTESIAN_POINT('Ctrl Pts',(8.57049938306334,6.56176641478979,0.751490748652533)) ;
#101218=CARTESIAN_POINT('Ctrl Pts',(8.57538893105717,6.56259599225628,0.746213733861456)) ;
#101219=CARTESIAN_POINT('Ctrl Pts',(8.57808773793836,6.56305388107911,0.743301063028025)) ;
#101220=CARTESIAN_POINT('Ctrl Pts',(8.58081254036867,6.56351521010419,0.740420620632313)) ;
#101221=CARTESIAN_POINT('Ctrl Pts',(8.58355195315297,6.56397636517831,0.7375663802795)) ;
#101222=CARTESIAN_POINT('Ctrl Pts',(8.5,8.3521616921714,0.647593901749794)) ;
#101223=CARTESIAN_POINT('Ctrl Pts',(8.5,8.2900428850829,0.678653305294049)) ;
#101224=CARTESIAN_POINT('Ctrl Pts',(8.56507848521152,8.26835005667905,0.689499719495969)) ;
#101225=CARTESIAN_POINT('Ctrl Pts',(8.5,8.31945293993531,0.582176402731433)) ;
#101226=CARTESIAN_POINT('Ctrl Pts',(8.5,8.26922013491182,0.637007811203667)) ;
#101227=CARTESIAN_POINT('Ctrl Pts',(8.56507848600996,8.25199117628908,0.656781959381388)) ;
#101228=CARTESIAN_POINT('Ctrl Pts',(8.5,8.24922766844397,0.540287293148598)) ;
#101229=CARTESIAN_POINT('Ctrl Pts',(8.5,8.21777561643093,0.615522630177237)) ;
#101230=CARTESIAN_POINT('Ctrl Pts',(8.57228151929423,8.21451202732349,0.637046919882372)) ;
#101231=CARTESIAN_POINT('Ctrl Pts',(8.5,8.17221734381475,0.540287291161696)) ;
#101232=CARTESIAN_POINT('Ctrl Pts',(8.5,8.17221734381475,0.625)) ;
#101233=CARTESIAN_POINT('Ctrl Pts',(8.58356010126947,8.17221734381475,0.638926683544911)) ;
#101234=CARTESIAN_POINT('',(8.50000000249538,8.20000280433619,0.542095256361575)) ;
#101235=CARTESIAN_POINT('',(8.54742025481395,8.27608084305204,0.685634338044055)) ;
#101236=CARTESIAN_POINT('Ctrl Pts',(8.50000000249538,8.20000280433619,0.542095256361575)) ;
#101237=CARTESIAN_POINT('Ctrl Pts',(8.50000274011724,8.20154143765779,0.554364551548918)) ;
#101238=CARTESIAN_POINT('Ctrl Pts',(8.50225788919788,8.20358050335012,0.566733525020421)) ;
#101239=CARTESIAN_POINT('Ctrl Pts',(8.50614710304112,8.20657022673326,0.578084018986108)) ;
#101240=CARTESIAN_POINT('Ctrl Pts',(8.51002595055128,8.20955198129041,0.589404259279535)) ;
#101241=CARTESIAN_POINT('Ctrl Pts',(8.51564213392183,8.21362262975068,0.599953866479339)) ;
#101242=CARTESIAN_POINT('Ctrl Pts',(8.52129493663065,8.21921832196825,0.609378207766048)) ;
#101243=CARTESIAN_POINT('Ctrl Pts',(8.52933132065201,8.22717351408127,0.622776451014487)) ;
#101244=CARTESIAN_POINT('Ctrl Pts',(8.53683691159804,8.23885362788864,0.634337556556648)) ;
#101245=CARTESIAN_POINT('Ctrl Pts',(8.54097226482464,8.25011947738646,0.647118830382909)) ;
#101246=CARTESIAN_POINT('Ctrl Pts',(8.54447125915462,8.25965170869904,0.657933288591762)) ;
#101247=CARTESIAN_POINT('Ctrl Pts',(8.54617119150717,8.26873789958222,0.67006038981035)) ;
#101248=CARTESIAN_POINT('Ctrl Pts',(8.54724932284106,8.27506683274844,0.683433539748685)) ;
#101249=CARTESIAN_POINT('Ctrl Pts',(8.54730817192851,8.27541229338911,0.684163504313674)) ;
#101250=CARTESIAN_POINT('Ctrl Pts',(8.5473651061662,8.27575037116516,0.684897167393986)) ;
#101251=CARTESIAN_POINT('Ctrl Pts',(8.54742024083733,8.27608084608571,0.685634324792657)) ;
#101252=CARTESIAN_POINT('',(8.56507848521152,8.26835005667905,0.68949971949597)) ;
#101253=CARTESIAN_POINT('Origin',(8.6,8.3521616921714,0.647593901749795)) ;
#101254=CARTESIAN_POINT('',(8.58356010126947,8.17221734381475,0.638926683544911)) ;
#101255=CARTESIAN_POINT('Origin',(8.59670327708548,8.16883734299703,0.732931030480332)) ;
#101256=CARTESIAN_POINT('',(8.5,8.17221734381475,0.540287291161696)) ;
#101257=CARTESIAN_POINT('Origin',(8.6,8.17221734381475,0.540287291161696)) ;
#101258=CARTESIAN_POINT('Origin',(8.5,8.16642648774923,0.762892247498121)) ;
#101259=CARTESIAN_POINT('Origin',(2.9,3.8,0.)) ;
#101260=CARTESIAN_POINT('',(3.,2.4,-1.7145055188063E-16)) ;
#101261=CARTESIAN_POINT('Origin',(3.,3.8,0.)) ;
#101262=CARTESIAN_POINT('',(2.9,2.3,-1.83697019872103E-16)) ;
#101263=CARTESIAN_POINT('Origin',(2.9,2.4,-1.71450551880629E-16)) ;
#101264=CARTESIAN_POINT('Origin',(2.9,3.8,0.)) ;
#101265=CARTESIAN_POINT('Origin',(1.35,3.8,0.)) ;
#101266=CARTESIAN_POINT('',(1.35,2.3,-1.83697019872103E-16)) ;
#101267=CARTESIAN_POINT('Origin',(1.35,3.8,0.)) ;
#101268=CARTESIAN_POINT('',(1.25,2.2,-1.95943487863577E-16)) ;
#101269=CARTESIAN_POINT('Origin',(1.35,2.2,-1.95943487863577E-16)) ;
#101270=CARTESIAN_POINT('Origin',(1.25,3.8,0.)) ;
#101271=CARTESIAN_POINT('Origin',(13.9153543900904,1.02736587339764,0.849999999999999)) ;
#101272=CARTESIAN_POINT('',(1.15,1.02736587339764,0.749999999999999)) ;
#101273=CARTESIAN_POINT('',(1.15,0.931757800066529,0.879310344827585)) ;
#101274=CARTESIAN_POINT('Origin',(1.15,1.02736587339764,0.849999999999999)) ;
#101275=CARTESIAN_POINT('',(-0.900000000000002,1.02736587339765,0.749999999999999)) ;
#101276=CARTESIAN_POINT('',(-1.,1.02736587339765,0.749999999999999)) ;
#101277=CARTESIAN_POINT('',(-0.900000000000002,0.982644513847654,0.760557280900007)) ;
#101278=CARTESIAN_POINT('Origin',(-0.900000000000002,1.02736587339765,0.849999999999999)) ;
#101279=CARTESIAN_POINT('',(-0.900000000000002,0.93175780006653,0.879310344827585)) ;
#101280=CARTESIAN_POINT('Origin',(-0.900000000000002,1.02736587339765,0.849999999999999)) ;
#101281=CARTESIAN_POINT('',(13.9153543900904,0.931757800066525,0.879310344827585)) ;
#101282=CARTESIAN_POINT('Origin',(13.9153543900904,1.02736587339764,-0.850000000000001)) ;
#101283=CARTESIAN_POINT('',(1.15,0.93175780006653,-0.879310344827587)) ;
#101284=CARTESIAN_POINT('',(1.15,1.02736587339765,-0.750000000000001)) ;
#101285=CARTESIAN_POINT('Origin',(1.15,1.02736587339765,-0.850000000000001)) ;
#101286=CARTESIAN_POINT('',(-0.900000000000002,0.931757800066531,-0.879310344827587)) ;
#101287=CARTESIAN_POINT('',(13.9153543900904,0.931757800066525,-0.879310344827587)) ;
#101288=CARTESIAN_POINT('',(-0.900000000000002,1.02736587339765,-0.750000000000001)) ;
#101289=CARTESIAN_POINT('Origin',(-0.900000000000002,1.02736587339765,-0.850000000000001)) ;
#101290=CARTESIAN_POINT('',(-1.,1.02736587339765,-0.750000000000001)) ;
#101291=CARTESIAN_POINT('Origin',(8.49172374697003,3.8,0.)) ;
#101292=CARTESIAN_POINT('',(8.49172374697003,1.47741935483871,1.89884679390471)) ;
#101293=CARTESIAN_POINT('',(8.49172374697003,1.47741935483871,-1.89884679390471)) ;
#101294=CARTESIAN_POINT('Origin',(8.49172374697003,3.8,0.)) ;
#101295=CARTESIAN_POINT('',(8.50816364570057,1.47636598119991,1.89970798904167)) ;
#101296=CARTESIAN_POINT('Origin',(8.49172374697003,1.4,1.96214168703486)) ;
#101297=CARTESIAN_POINT('',(8.50816364570057,1.47636598119991,-1.89970798904167)) ;
#101298=CARTESIAN_POINT('Origin',(8.50816364570057,3.8,0.)) ;
#101299=CARTESIAN_POINT('Origin',(8.49172374697003,1.4,-1.96214168703486)) ;
#101300=CARTESIAN_POINT('Origin',(1.25,3.8,0.)) ;
#101301=CARTESIAN_POINT('',(1.25,2.3,-1.83697019872103E-16)) ;
#101302=CARTESIAN_POINT('Origin',(13.9153543900904,3.8,0.)) ;
#101303=CARTESIAN_POINT('',(-0.900000000000002,1.47741935483872,-1.89884679390471)) ;
#101304=CARTESIAN_POINT('',(13.9153543900904,1.47741935483871,-1.89884679390471)) ;
#101305=CARTESIAN_POINT('Origin',(-0.900000000000001,3.8,0.)) ;
#101306=CARTESIAN_POINT('',(1.35,0.876327704607742,-0.672413793103449)) ;
#101307=CARTESIAN_POINT('Ctrl Pts',(1.35,0.876327704607742,-0.672413793103449)) ;
#101308=CARTESIAN_POINT('Ctrl Pts',(1.35,0.888571289407569,-0.725649211595278)) ;
#101309=CARTESIAN_POINT('Ctrl Pts',(1.32969623836296,0.902340613578954,
-0.77792959702133)) ;
#101310=CARTESIAN_POINT('Ctrl Pts',(1.25741074236298,0.924142973728496,
-0.855015053715771)) ;
#101311=CARTESIAN_POINT('Ctrl Pts',(1.20472523187106,0.93175780006653,-0.879310344827587)) ;
#101312=CARTESIAN_POINT('Ctrl Pts',(1.15,0.93175780006653,-0.879310344827587)) ;
#101313=CARTESIAN_POINT('',(1.35,0.876327704607742,0.672413793103447)) ;
#101314=CARTESIAN_POINT('Origin',(1.35,3.8,0.)) ;
#101315=CARTESIAN_POINT('Ctrl Pts',(1.15,0.931757800066529,0.879310344827585)) ;
#101316=CARTESIAN_POINT('Ctrl Pts',(1.20475877631964,0.931757800066529,
0.879310344827585)) ;
#101317=CARTESIAN_POINT('Ctrl Pts',(1.2574100247738,0.924155896380523,0.855065639111651)) ;
#101318=CARTESIAN_POINT('Ctrl Pts',(1.32987646938161,0.9022735155524,0.777687454472096)) ;
#101319=CARTESIAN_POINT('Ctrl Pts',(1.35,0.888577265820266,0.725675197189874)) ;
#101320=CARTESIAN_POINT('Ctrl Pts',(1.35,0.876327704607742,0.672413793103447)) ;
#101321=CARTESIAN_POINT('',(-0.900000000000002,1.47741935483872,1.89884679390471)) ;
#101322=CARTESIAN_POINT('Origin',(-0.900000000000001,3.8,0.)) ;
#101323=CARTESIAN_POINT('',(13.9153543900904,1.47741935483871,1.89884679390471)) ;
#101324=CARTESIAN_POINT('Origin',(0.55,3.09772049281573E-17,-2.67525834540015E-32)) ;
#101325=CARTESIAN_POINT('',(0.549999999999999,4.4,0.45)) ;
#101326=CARTESIAN_POINT('',(0.549999999999999,4.4,-0.45)) ;
#101327=CARTESIAN_POINT('',(0.549999999999999,4.4,-2.67525834540015E-32)) ;
#101328=CARTESIAN_POINT('',(0.55,4.04473197180486,-0.45)) ;
#101329=CARTESIAN_POINT('',(0.55,1.39397422176708E-16,-0.450000000000001)) ;
#101330=CARTESIAN_POINT('',(0.55,4.05997159067981,-0.4)) ;
#101331=CARTESIAN_POINT('Ctrl Pts',(0.549999999999999,4.04473197180486,
-0.450000000000001)) ;
#101332=CARTESIAN_POINT('Ctrl Pts',(0.549999999999999,4.04764757798806,
-0.445564861127741)) ;
#101333=CARTESIAN_POINT('Ctrl Pts',(0.55,4.05014503921306,-0.440948144865881)) ;
#101334=CARTESIAN_POINT('Ctrl Pts',(0.549999999999999,4.0569489863933,-0.425681445690252)) ;
#101335=CARTESIAN_POINT('Ctrl Pts',(0.549999999999999,4.0599715906798,-0.411821456441416)) ;
#101336=CARTESIAN_POINT('Ctrl Pts',(0.549999999999999,4.0599715906798,-0.4)) ;
#101337=CARTESIAN_POINT('',(0.55,4.05997159067981,0.4)) ;
#101338=CARTESIAN_POINT('',(0.55,4.05997159067981,0.5)) ;
#101339=CARTESIAN_POINT('',(0.55,4.04473197181449,0.449999999985356)) ;
#101340=CARTESIAN_POINT('Origin',(0.55003450380262,3.93869457791467,0.39758397030464)) ;
#101341=CARTESIAN_POINT('',(0.55,6.35032701027224E-17,0.450000000000001)) ;
#101342=CARTESIAN_POINT('Origin',(10.,7.8,-2.54)) ;
#101343=CARTESIAN_POINT('',(9.93162277660169,7.82279240779944,-2.54)) ;
#101344=CARTESIAN_POINT('',(8.51539501058484,8.29486832980505,-2.54)) ;
#101345=CARTESIAN_POINT('',(10.,7.8,-2.54)) ;
#101346=CARTESIAN_POINT('',(8.5154009551171,8.29487265903615,-0.769060759934173)) ;
#101347=CARTESIAN_POINT('',(8.51539501058484,8.29486832980505,-2.54)) ;
#101348=CARTESIAN_POINT('',(8.54856023413469,8.28398586203114,-0.756008066565519)) ;
#101349=CARTESIAN_POINT('Ctrl Pts',(8.5154009551171,8.29487265903615,-0.769060759934173)) ;
#101350=CARTESIAN_POINT('Ctrl Pts',(8.51716444659958,8.29428466923188,-0.769642482818871)) ;
#101351=CARTESIAN_POINT('Ctrl Pts',(8.51901954868166,8.29366521079576,-0.769970450858189)) ;
#101352=CARTESIAN_POINT('Ctrl Pts',(8.52087614409666,8.2930450194617,-0.770072502578372)) ;
#101353=CARTESIAN_POINT('Ctrl Pts',(8.52171779595217,8.29276386763785,-0.770118765764716)) ;
#101354=CARTESIAN_POINT('Ctrl Pts',(8.52256005861364,8.29248252453828,-0.770119087778023)) ;
#101355=CARTESIAN_POINT('Ctrl Pts',(8.52339613191994,8.29220315552769,-0.770079446014073)) ;
#101356=CARTESIAN_POINT('Ctrl Pts',(8.52456316579569,8.29181319797644,-0.770024112012765)) ;
#101357=CARTESIAN_POINT('Ctrl Pts',(8.52573147766847,8.29142195356396,-0.769893004995753)) ;
#101358=CARTESIAN_POINT('Ctrl Pts',(8.52689074379088,8.29103442649366,-0.769691327086012)) ;
#101359=CARTESIAN_POINT('Ctrl Pts',(8.52858695132694,8.29046740713169,-0.76939623730141)) ;
#101360=CARTESIAN_POINT('Ctrl Pts',(8.53026630212632,8.28992123633277,-0.768943921814253)) ;
#101361=CARTESIAN_POINT('Ctrl Pts',(8.53190117913127,8.28939883282065,-0.768368372916171)) ;
#101362=CARTESIAN_POINT('Ctrl Pts',(8.53241671440281,8.28923410028379,-0.76818688173576)) ;
#101363=CARTESIAN_POINT('Ctrl Pts',(8.5329279003779,8.28907155799427,-0.767993397517365)) ;
#101364=CARTESIAN_POINT('Ctrl Pts',(8.53343404910736,8.28891083250768,-0.767789837955259)) ;
#101365=CARTESIAN_POINT('Ctrl Pts',(8.53529681408171,8.28831931900687,-0.767040683407564)) ;
#101366=CARTESIAN_POINT('Ctrl Pts',(8.53711612169874,8.28774836357889,-0.766131008833549)) ;
#101367=CARTESIAN_POINT('Ctrl Pts',(8.53885192161983,8.28720494689876,-0.765061264748013)) ;
#101368=CARTESIAN_POINT('Ctrl Pts',(8.5401592515911,8.28679566878773,-0.764255579433931)) ;
#101369=CARTESIAN_POINT('Ctrl Pts',(8.54141951580281,8.286401527759,-0.763359746191826)) ;
#101370=CARTESIAN_POINT('Ctrl Pts',(8.54261761299017,8.28602171215282,-0.762392710785422)) ;
#101371=CARTESIAN_POINT('Ctrl Pts',(8.54427390694789,8.28549664098145,-0.761055845197686)) ;
#101372=CARTESIAN_POINT('Ctrl Pts',(8.54582756795259,8.28499592220792,-0.759557433696207)) ;
#101373=CARTESIAN_POINT('Ctrl Pts',(8.54719190273355,8.28456181678112,-0.757913976052287)) ;
#101374=CARTESIAN_POINT('Ctrl Pts',(8.54768505754695,8.28440490428153,-0.757319929005303)) ;
#101375=CARTESIAN_POINT('Ctrl Pts',(8.54815358395156,8.28425671205377,-0.756707432307545)) ;
#101376=CARTESIAN_POINT('Ctrl Pts',(8.54859369700692,8.28411936587099,-0.756078854561789)) ;
#101377=CARTESIAN_POINT('',(8.56837597005373,8.27720399148448,-0.732505421266908)) ;
#101378=CARTESIAN_POINT('Ctrl Pts',(8.5485198670553,8.28382649282421,-0.756014052775836)) ;
#101379=CARTESIAN_POINT('Ctrl Pts',(8.55267891820636,8.28243778061537,-0.750563127305208)) ;
#101380=CARTESIAN_POINT('Ctrl Pts',(8.55701747195692,8.28096933708252,-0.745259057781419)) ;
#101381=CARTESIAN_POINT('Ctrl Pts',(8.56150853123457,8.27945301063652,-0.740113210213359)) ;
#101382=CARTESIAN_POINT('Ctrl Pts',(8.56331520072595,8.27884302075226,-0.738043131589642)) ;
#101383=CARTESIAN_POINT('Ctrl Pts',(8.56514663435535,8.27822544298232,-0.7359980022295)) ;
#101384=CARTESIAN_POINT('Ctrl Pts',(8.56700126712395,8.27760232477898,-0.733975785658495)) ;
#101385=CARTESIAN_POINT('Ctrl Pts',(8.56745273479657,8.27745064099026,-0.73348352356526)) ;
#101386=CARTESIAN_POINT('Ctrl Pts',(8.56790562999349,8.27729861980368,-0.732995195362696)) ;
#101387=CARTESIAN_POINT('Ctrl Pts',(8.56835731300613,8.27714712982919,-0.732505596582496)) ;
#101388=CARTESIAN_POINT('',(9.93162277660169,7.82279240779944,-0.959712708838304)) ;
#101389=CARTESIAN_POINT('',(9.98593528106273,7.80468823964576,-0.968764792915145)) ;
#101390=CARTESIAN_POINT('',(9.93162277660169,7.82279240779944,-2.54)) ;
#101391=CARTESIAN_POINT('Origin',(10.,6.8,-2.54)) ;
#101392=CARTESIAN_POINT('',(10.,6.8847127088383,-2.54)) ;
#101393=CARTESIAN_POINT('',(10.,7.72792407799439,-2.54)) ;
#101394=CARTESIAN_POINT('',(10.,6.8,-2.54)) ;
#101395=CARTESIAN_POINT('',(10.,7.72792407799439,-0.959712708838304)) ;
#101396=CARTESIAN_POINT('',(10.,7.72792407799439,-2.54)) ;
#101397=CARTESIAN_POINT('',(10.,6.8847127088383,-0.959712708838304)) ;
#101398=CARTESIAN_POINT('',(10.,6.8,-0.959712708838304)) ;
#101399=CARTESIAN_POINT('',(10.,6.8847127088383,-2.54)) ;
#101400=CARTESIAN_POINT('Origin',(8.5,6.55,-2.54)) ;
#101401=CARTESIAN_POINT('',(9.91643989873054,6.78607331645509,-0.959712708838304)) ;
#101402=CARTESIAN_POINT('',(8.58355805979357,6.56393854759965,-0.737566541570668)) ;
#101403=CARTESIAN_POINT('',(8.48442535909739,6.54740422651623,-0.721043618899445)) ;
#101404=CARTESIAN_POINT('',(8.56107669735261,6.56009388000089,-0.762383847222383)) ;
#101405=CARTESIAN_POINT('Ctrl Pts',(8.58354728038624,6.56400494118525,-0.737566748635123)) ;
#101406=CARTESIAN_POINT('Ctrl Pts',(8.5783885388571,6.56313097816981,-0.742936569647583)) ;
#101407=CARTESIAN_POINT('Ctrl Pts',(8.5733012794658,6.56225500583444,-0.748388168656423)) ;
#101408=CARTESIAN_POINT('Ctrl Pts',(8.56834297134844,6.5614089984297,-0.753960783789144)) ;
#101409=CARTESIAN_POINT('Ctrl Pts',(8.56587587079896,6.56098805134781,-0.756733544483026)) ;
#101410=CARTESIAN_POINT('Ctrl Pts',(8.56344049907325,6.56057499921407,-0.75953530332024)) ;
#101411=CARTESIAN_POINT('Ctrl Pts',(8.56104288133097,6.56017406260212,-0.762365036245923)) ;
#101412=CARTESIAN_POINT('',(8.50816305748499,6.55136011924236,-0.777372622105259)) ;
#101413=CARTESIAN_POINT('Ctrl Pts',(8.56125813732197,6.56020968955366,-0.76255063535366)) ;
#101414=CARTESIAN_POINT('Ctrl Pts',(8.55737139916473,6.55956189986079,-0.767208599473684)) ;
#101415=CARTESIAN_POINT('Ctrl Pts',(8.553063351902,6.55884389198366,-0.769967466087569)) ;
#101416=CARTESIAN_POINT('Ctrl Pts',(8.54121332232624,6.55686888705437,-0.776523740784031)) ;
#101417=CARTESIAN_POINT('Ctrl Pts',(8.53496267038527,6.55582711173088,-0.777961360668917)) ;
#101418=CARTESIAN_POINT('Ctrl Pts',(8.52888665185105,6.55481444197518,-0.779279553931391)) ;
#101419=CARTESIAN_POINT('Ctrl Pts',(8.52471102104665,6.55411850350777,-0.779597749401341)) ;
#101420=CARTESIAN_POINT('Ctrl Pts',(8.52011475164503,6.55335245860751,-0.779702959935202)) ;
#101421=CARTESIAN_POINT('Ctrl Pts',(8.51754797133863,6.55292466188977,-0.779718645942938)) ;
#101422=CARTESIAN_POINT('Ctrl Pts',(8.51248317870075,6.55208052978346,-0.778963822862177)) ;
#101423=CARTESIAN_POINT('Ctrl Pts',(8.51021540604914,6.55170256767486,-0.778370896111508)) ;
#101424=CARTESIAN_POINT('Ctrl Pts',(8.50816120922224,6.55136020153704,-0.777376411526063)) ;
#101425=CARTESIAN_POINT('',(8.50816364570071,6.55136060761679,-2.54)) ;
#101426=CARTESIAN_POINT('',(8.50816364570071,6.55136060761679,-2.54)) ;
#101427=CARTESIAN_POINT('',(9.91643989873054,6.78607331645509,-2.54)) ;
#101428=CARTESIAN_POINT('',(8.5,6.55,-2.54)) ;
#101429=CARTESIAN_POINT('',(9.91643989873054,6.78607331645509,-2.54)) ;
#101430=CARTESIAN_POINT('Origin',(10.,1.5,-2.54)) ;
#101431=CARTESIAN_POINT('',(-0.900000000000002,1.5,-1.96214168703487)) ;
#101432=CARTESIAN_POINT('',(8.49172374697003,1.5,-1.96214168703487)) ;
#101433=CARTESIAN_POINT('',(10.,1.5,-1.96214168703487)) ;
#101434=CARTESIAN_POINT('',(8.49172374697003,1.5,-2.54)) ;
#101435=CARTESIAN_POINT('',(8.49172374697003,1.5,-2.54)) ;
#101436=CARTESIAN_POINT('',(-0.900000000000001,1.5,-2.54)) ;
#101437=CARTESIAN_POINT('',(10.,1.5,-2.54)) ;
#101438=CARTESIAN_POINT('',(-0.900000000000002,1.5,-1.92613602842582)) ;
#101439=CARTESIAN_POINT('Origin',(10.,1.5,-2.54)) ;
#101440=CARTESIAN_POINT('',(8.49172374697003,1.5,2.54)) ;
#101441=CARTESIAN_POINT('',(-0.900000000000001,1.5,2.54)) ;
#101442=CARTESIAN_POINT('',(10.,1.5,2.54)) ;
#101443=CARTESIAN_POINT('',(8.49172374697003,1.5,1.96214168703487)) ;
#101444=CARTESIAN_POINT('',(8.49172374697003,1.5,-2.54)) ;
#101445=CARTESIAN_POINT('',(-0.900000000000002,1.5,1.96214168703487)) ;
#101446=CARTESIAN_POINT('',(10.,1.5,1.96214168703487)) ;
#101447=CARTESIAN_POINT('',(-0.900000000000001,1.5,-2.54)) ;
#101448=CARTESIAN_POINT('Origin',(10.,0.,-2.54)) ;
#101449=CARTESIAN_POINT('',(10.,0.1,2.54)) ;
#101450=CARTESIAN_POINT('',(10.,1.16528729116168,2.54)) ;
#101451=CARTESIAN_POINT('',(10.,0.,2.54)) ;
#101452=CARTESIAN_POINT('',(10.,0.1,-2.54)) ;
#101453=CARTESIAN_POINT('',(10.,0.1,-2.54)) ;
#101454=CARTESIAN_POINT('',(10.,1.16528729116168,-2.54)) ;
#101455=CARTESIAN_POINT('',(10.,0.,-2.54)) ;
#101456=CARTESIAN_POINT('',(10.,1.16528729116168,-2.04416188017819)) ;
#101457=CARTESIAN_POINT('',(10.,1.16528729116168,-2.54)) ;
#101458=CARTESIAN_POINT('',(10.,1.16528729116168,2.04416188017819)) ;
#101459=CARTESIAN_POINT('Origin',(10.,3.8,0.)) ;
#101460=CARTESIAN_POINT('',(10.,1.16528729116168,-2.54)) ;
#101461=CARTESIAN_POINT('Origin',(0.,0.,-2.54)) ;
#101462=CARTESIAN_POINT('',(8.48377223398316,8.3,-2.54)) ;
#101463=CARTESIAN_POINT('',(7.1,8.3,-2.54)) ;
#101464=CARTESIAN_POINT('',(8.5,8.3,-2.54)) ;
#101465=CARTESIAN_POINT('Origin',(8.48377223398316,8.2,-2.54)) ;
#101466=CARTESIAN_POINT('Origin',(9.9,7.72792407799439,-2.54)) ;
#101467=CARTESIAN_POINT('Origin',(9.9,6.8847127088383,-2.54)) ;
#101468=CARTESIAN_POINT('',(8.49172374697018,6.55,-2.54)) ;
#101469=CARTESIAN_POINT('Origin',(8.49172374697018,6.65,-2.54)) ;
#101470=CARTESIAN_POINT('',(-0.900000000000001,6.55,-2.54)) ;
#101471=CARTESIAN_POINT('',(1.25,6.55,-2.54)) ;
#101472=CARTESIAN_POINT('',(-1.,6.45,-2.54)) ;
#101473=CARTESIAN_POINT('Origin',(-0.9,6.45,-2.54)) ;
#101474=CARTESIAN_POINT('',(-1.,4.65,-2.54)) ;
#101475=CARTESIAN_POINT('',(-1.,3.46944695195362E-16,-2.54)) ;
#101476=CARTESIAN_POINT('',(-0.900000000000001,4.55,-2.54)) ;
#101477=CARTESIAN_POINT('Origin',(-0.900000000000001,4.65,-2.54)) ;
#101478=CARTESIAN_POINT('',(1.15,4.55,-2.54)) ;
#101479=CARTESIAN_POINT('',(1.57859836313889E-15,4.55,-2.54)) ;
#101480=CARTESIAN_POINT('',(1.25,4.45,-2.54)) ;
#101481=CARTESIAN_POINT('Origin',(1.15,4.45,-2.54)) ;
#101482=CARTESIAN_POINT('',(1.25,3.15,-2.54)) ;
#101483=CARTESIAN_POINT('',(1.25,1.5,-2.54)) ;
#101484=CARTESIAN_POINT('',(1.15,3.05,-2.54)) ;
#101485=CARTESIAN_POINT('Origin',(1.15,3.15,-2.54)) ;
#101486=CARTESIAN_POINT('',(-0.900000000000002,3.05,-2.54)) ;
#101487=CARTESIAN_POINT('',(1.05818132034585E-15,3.05,-2.54)) ;
#101488=CARTESIAN_POINT('',(-1.,2.95,-2.54)) ;
#101489=CARTESIAN_POINT('Origin',(-0.900000000000002,2.95,-2.54)) ;
#101490=CARTESIAN_POINT('',(-1.,1.6,-2.54)) ;
#101491=CARTESIAN_POINT('',(-1.,3.46944695195362E-16,-2.54)) ;
#101492=CARTESIAN_POINT('Origin',(-0.900000000000002,1.6,-2.54)) ;
#101493=CARTESIAN_POINT('',(8.50816364570057,1.49863939238321,-2.54)) ;
#101494=CARTESIAN_POINT('Origin',(8.49172374697003,1.4,-2.54)) ;
#101495=CARTESIAN_POINT('',(9.91643989873054,1.26392668354489,-2.54)) ;
#101496=CARTESIAN_POINT('',(10.,1.24999999999998,-2.54)) ;
#101497=CARTESIAN_POINT('Origin',(9.9,1.16528729116168,-2.54)) ;
#101498=CARTESIAN_POINT('',(9.9,0.,-2.54)) ;
#101499=CARTESIAN_POINT('Origin',(9.9,0.1,-2.54)) ;
#101500=CARTESIAN_POINT('',(-2.,0.,-2.54)) ;
#101501=CARTESIAN_POINT('',(-2.,0.,-2.54)) ;
#101502=CARTESIAN_POINT('',(-2.,7.55,-2.54)) ;
#101503=CARTESIAN_POINT('',(-2.,7.65,-2.54)) ;
#101504=CARTESIAN_POINT('',(-1.9,7.65,-2.54)) ;
#101505=CARTESIAN_POINT('Origin',(-1.9,7.55,-2.54)) ;
#101506=CARTESIAN_POINT('',(6.9,7.65,-2.54)) ;
#101507=CARTESIAN_POINT('',(7.,7.65,-2.54)) ;
#101508=CARTESIAN_POINT('',(7.,7.75,-2.54)) ;
#101509=CARTESIAN_POINT('Origin',(6.9,7.75,-2.54)) ;
#101510=CARTESIAN_POINT('',(7.,8.2,-2.54)) ;
#101511=CARTESIAN_POINT('',(7.,8.3,-2.54)) ;
#101512=CARTESIAN_POINT('Origin',(7.1,8.2,-2.54)) ;
#101513=CARTESIAN_POINT('Origin',(0.,0.,2.54)) ;
#101514=CARTESIAN_POINT('',(9.93162277660169,7.82279240779944,2.54)) ;
#101515=CARTESIAN_POINT('',(8.51539501058484,8.29486832980505,2.54)) ;
#101516=CARTESIAN_POINT('',(10.,7.8,2.54)) ;
#101517=CARTESIAN_POINT('',(8.48377223398316,8.3,2.54)) ;
#101518=CARTESIAN_POINT('Origin',(8.48377223398316,8.2,2.54)) ;
#101519=CARTESIAN_POINT('',(7.1,8.3,2.54)) ;
#101520=CARTESIAN_POINT('',(8.5,8.3,2.54)) ;
#101521=CARTESIAN_POINT('',(7.,8.2,2.54)) ;
#101522=CARTESIAN_POINT('Origin',(7.1,8.2,2.54)) ;
#101523=CARTESIAN_POINT('',(7.,7.75,2.54)) ;
#101524=CARTESIAN_POINT('',(7.,8.3,2.54)) ;
#101525=CARTESIAN_POINT('',(6.9,7.65,2.54)) ;
#101526=CARTESIAN_POINT('Origin',(6.9,7.75,2.54)) ;
#101527=CARTESIAN_POINT('',(-1.9,7.65,2.54)) ;
#101528=CARTESIAN_POINT('',(7.,7.65,2.54)) ;
#101529=CARTESIAN_POINT('',(-2.,7.55,2.54)) ;
#101530=CARTESIAN_POINT('Origin',(-1.9,7.55,2.54)) ;
#101531=CARTESIAN_POINT('',(-2.,0.,2.54)) ;
#101532=CARTESIAN_POINT('',(-2.,7.65,2.54)) ;
#101533=CARTESIAN_POINT('',(9.9,0.,2.54)) ;
#101534=CARTESIAN_POINT('',(-2.,0.,2.54)) ;
#101535=CARTESIAN_POINT('Origin',(9.9,0.1,2.54)) ;
#101536=CARTESIAN_POINT('',(9.91643989873054,1.26392668354489,2.54)) ;
#101537=CARTESIAN_POINT('Origin',(9.9,1.16528729116168,2.54)) ;
#101538=CARTESIAN_POINT('',(8.50816364570057,1.49863939238321,2.54)) ;
#101539=CARTESIAN_POINT('',(0.472972972972955,2.83783783783779,2.54)) ;
#101540=CARTESIAN_POINT('Origin',(8.49172374697003,1.4,2.54)) ;
#101541=CARTESIAN_POINT('',(-1.,1.6,2.54)) ;
#101542=CARTESIAN_POINT('Origin',(-0.900000000000002,1.6,2.54)) ;
#101543=CARTESIAN_POINT('',(-1.,2.95,2.54)) ;
#101544=CARTESIAN_POINT('',(-1.,3.46944695195362E-16,2.54)) ;
#101545=CARTESIAN_POINT('',(-0.900000000000002,3.05,2.54)) ;
#101546=CARTESIAN_POINT('Origin',(-0.900000000000002,2.95,2.54)) ;
#101547=CARTESIAN_POINT('',(1.15,3.05,2.54)) ;
#101548=CARTESIAN_POINT('',(1.05818132034585E-15,3.05,2.54)) ;
#101549=CARTESIAN_POINT('',(1.25,3.15,2.54)) ;
#101550=CARTESIAN_POINT('Origin',(1.15,3.15,2.54)) ;
#101551=CARTESIAN_POINT('',(1.25,4.45,2.54)) ;
#101552=CARTESIAN_POINT('',(1.25,5.3,2.54)) ;
#101553=CARTESIAN_POINT('',(1.15,4.55,2.54)) ;
#101554=CARTESIAN_POINT('Origin',(1.15,4.45,2.54)) ;
#101555=CARTESIAN_POINT('',(-0.900000000000001,4.55,2.54)) ;
#101556=CARTESIAN_POINT('',(1.57859836313889E-15,4.55,2.54)) ;
#101557=CARTESIAN_POINT('',(-1.,4.65,2.54)) ;
#101558=CARTESIAN_POINT('Origin',(-0.900000000000001,4.65,2.54)) ;
#101559=CARTESIAN_POINT('',(-1.,6.45,2.54)) ;
#101560=CARTESIAN_POINT('',(-1.,3.46944695195362E-16,2.54)) ;
#101561=CARTESIAN_POINT('',(-0.900000000000001,6.55,2.54)) ;
#101562=CARTESIAN_POINT('Origin',(-0.9,6.45,2.54)) ;
#101563=CARTESIAN_POINT('',(8.49172374697018,6.55,2.54)) ;
#101564=CARTESIAN_POINT('',(1.25,6.55,2.54)) ;
#101565=CARTESIAN_POINT('',(8.50816364570071,6.55136060761679,2.54)) ;
#101566=CARTESIAN_POINT('Origin',(8.49172374697018,6.65,2.54)) ;
#101567=CARTESIAN_POINT('',(9.91643989873054,6.78607331645509,2.54)) ;
#101568=CARTESIAN_POINT('',(8.5,6.55,2.54)) ;
#101569=CARTESIAN_POINT('',(10.,6.8847127088383,2.54)) ;
#101570=CARTESIAN_POINT('Origin',(9.9,6.8847127088383,2.54)) ;
#101571=CARTESIAN_POINT('',(10.,7.72792407799439,2.54)) ;
#101572=CARTESIAN_POINT('',(10.,6.8,2.54)) ;
#101573=CARTESIAN_POINT('Origin',(9.9,7.72792407799439,2.54)) ;
#101574=CARTESIAN_POINT('Origin',(7.,7.65,-2.54)) ;
#101575=CARTESIAN_POINT('',(-1.9,7.65,-2.54)) ;
#101576=CARTESIAN_POINT('',(6.9,7.65,-2.54)) ;
#101577=CARTESIAN_POINT('Origin',(7.,8.3,-2.54)) ;
#101578=CARTESIAN_POINT('',(7.,7.75,2.54)) ;
#101579=CARTESIAN_POINT('',(7.,8.2,-2.54)) ;
#101580=CARTESIAN_POINT('Origin',(8.5,8.3,-2.54)) ;
#101581=CARTESIAN_POINT('',(8.4,8.3,-0.542072889850983)) ;
#101582=CARTESIAN_POINT('',(8.48377267093845,8.29999999999968,-0.758052545004225)) ;
#101583=CARTESIAN_POINT('Ctrl Pts',(8.40000000000001,8.3,-0.542072889850983)) ;
#101584=CARTESIAN_POINT('Ctrl Pts',(8.40000007660114,8.3,-0.559229650193567)) ;
#101585=CARTESIAN_POINT('Ctrl Pts',(8.40222537906589,8.3,-0.576196239113767)) ;
#101586=CARTESIAN_POINT('Ctrl Pts',(8.40642689896062,8.3,-0.592616256499238)) ;
#101587=CARTESIAN_POINT('Ctrl Pts',(8.41084238024274,8.3,-0.609872459310139)) ;
#101588=CARTESIAN_POINT('Ctrl Pts',(8.41744096860901,8.3,-0.626526744361822)) ;
#101589=CARTESIAN_POINT('Ctrl Pts',(8.42598957610089,8.3,-0.642162200721529)) ;
#101590=CARTESIAN_POINT('Ctrl Pts',(8.429275781256,8.3,-0.648172690423003)) ;
#101591=CARTESIAN_POINT('Ctrl Pts',(8.43285067318442,8.3,-0.654032446959054)) ;
#101592=CARTESIAN_POINT('Ctrl Pts',(8.43670279785317,8.3,-0.659716786785451)) ;
#101593=CARTESIAN_POINT('Ctrl Pts',(8.43684245837178,8.3,-0.659922875091612)) ;
#101594=CARTESIAN_POINT('Ctrl Pts',(8.4369824793911,8.3,-0.660128726822443)) ;
#101595=CARTESIAN_POINT('Ctrl Pts',(8.43712286024713,8.3,-0.660334340694031)) ;
#101596=CARTESIAN_POINT('Ctrl Pts',(8.4430409279857,8.3,-0.669002451535619)) ;
#101597=CARTESIAN_POINT('Ctrl Pts',(8.4496323269955,8.300000000002,-0.677331731364526)) ;
#101598=CARTESIAN_POINT('Ctrl Pts',(8.45667836512368,8.29999999999776,-0.685188273964224)) ;
#101599=CARTESIAN_POINT('Ctrl Pts',(8.46347186896914,8.29999999999367,-0.692763233309057)) ;
#101600=CARTESIAN_POINT('Ctrl Pts',(8.47075094334182,8.29999999998296,-0.699909865515332)) ;
#101601=CARTESIAN_POINT('Ctrl Pts',(8.47818849074308,8.29999999991001,-0.70688161282847)) ;
#101602=CARTESIAN_POINT('Ctrl Pts',(8.47846436286148,8.2999999999073,-0.707140207577044)) ;
#101603=CARTESIAN_POINT('Ctrl Pts',(8.47874045306876,8.29999999990447,-0.707398560599132)) ;
#101604=CARTESIAN_POINT('Ctrl Pts',(8.47901674447045,8.29999999990152,-0.707656685200035)) ;
#101605=CARTESIAN_POINT('Ctrl Pts',(8.48287938578321,8.29999999986032,-0.711265348883327)) ;
#101606=CARTESIAN_POINT('Ctrl Pts',(8.48681205529409,8.29999999978803,-0.714807936727803)) ;
#101607=CARTESIAN_POINT('Ctrl Pts',(8.49047938959116,8.29999999977836,-0.718602706021786)) ;
#101608=CARTESIAN_POINT('Ctrl Pts',(8.49231307405274,8.29999999977353,-0.720500108583422)) ;
#101609=CARTESIAN_POINT('Ctrl Pts',(8.49410676862313,8.29999999978935,-0.722469327124991)) ;
#101610=CARTESIAN_POINT('Ctrl Pts',(8.49555027122445,8.29999999981726,-0.724696807009918)) ;
#101611=CARTESIAN_POINT('Ctrl Pts',(8.49675259850851,8.2999999998405,-0.726552127421465)) ;
#101612=CARTESIAN_POINT('Ctrl Pts',(8.49764594203226,8.29999999986456,-0.728636815743195)) ;
#101613=CARTESIAN_POINT('Ctrl Pts',(8.49795530287013,8.29999999987615,-0.730811037449387)) ;
#101614=CARTESIAN_POINT('Ctrl Pts',(8.49801735255452,8.29999999987847,-0.731247129398159)) ;
#101615=CARTESIAN_POINT('Ctrl Pts',(8.49805590844335,8.29999999988033,-0.731686822978028)) ;
#101616=CARTESIAN_POINT('Ctrl Pts',(8.49806875158487,8.29999999988168,-0.732128989661398)) ;
#101617=CARTESIAN_POINT('Ctrl Pts',(8.49822249685463,8.2999999998978,-0.737422167806758)) ;
#101618=CARTESIAN_POINT('Ctrl Pts',(8.49538250015675,8.29999999989889,-0.742355344268398)) ;
#101619=CARTESIAN_POINT('Ctrl Pts',(8.49246863081132,8.29999999993393,-0.746722860550965)) ;
#101620=CARTESIAN_POINT('Ctrl Pts',(8.48983292606215,8.29999999996562,-0.750673443793859)) ;
#101621=CARTESIAN_POINT('Ctrl Pts',(8.48683766317129,8.3,-0.754392211069768)) ;
#101622=CARTESIAN_POINT('Ctrl Pts',(8.48377316486173,8.3,-0.75805195629754)) ;
#101623=CARTESIAN_POINT('',(8.48377223398316,8.3,-2.54)) ;
#101624=CARTESIAN_POINT('',(7.1,8.3,-2.54)) ;
#101625=CARTESIAN_POINT('',(8.48377267093845,8.29999999999968,0.758052545004229)) ;
#101626=CARTESIAN_POINT('',(8.48377223398316,8.3,-2.54)) ;
#101627=CARTESIAN_POINT('',(8.4,8.3,0.542072889850983)) ;
#101628=CARTESIAN_POINT('Ctrl Pts',(8.48377316486173,8.3,0.758051956297541)) ;
#101629=CARTESIAN_POINT('Ctrl Pts',(8.48683766317129,8.3,0.754392211069772)) ;
#101630=CARTESIAN_POINT('Ctrl Pts',(8.48983292606214,8.29999999996562,0.750673443793859)) ;
#101631=CARTESIAN_POINT('Ctrl Pts',(8.49246863081131,8.29999999993393,0.746722860550971)) ;
#101632=CARTESIAN_POINT('Ctrl Pts',(8.49538250015675,8.29999999989889,0.742355344268411)) ;
#101633=CARTESIAN_POINT('Ctrl Pts',(8.49822249685463,8.2999999998978,0.737422167806773)) ;
#101634=CARTESIAN_POINT('Ctrl Pts',(8.49806875158486,8.29999999988168,0.732128989661413)) ;
#101635=CARTESIAN_POINT('Ctrl Pts',(8.49805590844334,8.29999999988033,0.731686822978042)) ;
#101636=CARTESIAN_POINT('Ctrl Pts',(8.49801735255452,8.29999999987847,0.731247129398171)) ;
#101637=CARTESIAN_POINT('Ctrl Pts',(8.49795530287013,8.29999999987615,0.730811037449398)) ;
#101638=CARTESIAN_POINT('Ctrl Pts',(8.49764594190814,8.29999999986456,0.728636814870931)) ;
#101639=CARTESIAN_POINT('Ctrl Pts',(8.49675259754384,8.2999999998405,0.726552125932736)) ;
#101640=CARTESIAN_POINT('Ctrl Pts',(8.49555027122432,8.29999999981726,0.72469680701002)) ;
#101641=CARTESIAN_POINT('Ctrl Pts',(8.49410676570211,8.29999999978935,0.722469322618388)) ;
#101642=CARTESIAN_POINT('Ctrl Pts',(8.49231306928119,8.29999999977353,0.720500103647998)) ;
#101643=CARTESIAN_POINT('Ctrl Pts',(8.49047938958768,8.29999999977836,0.718602706025179)) ;
#101644=CARTESIAN_POINT('Ctrl Pts',(8.48681202348067,8.29999999978804,0.714807903826052)) ;
#101645=CARTESIAN_POINT('Ctrl Pts',(8.48287934332708,8.29999999986032,0.711265309269797)) ;
#101646=CARTESIAN_POINT('Ctrl Pts',(8.47901674443308,8.29999999990152,0.707656685240044)) ;
#101647=CARTESIAN_POINT('Ctrl Pts',(8.47874052296043,8.29999999990447,0.707398625971892)) ;
#101648=CARTESIAN_POINT('Ctrl Pts',(8.47846450284309,8.2999999999073,0.707140338643466)) ;
#101649=CARTESIAN_POINT('Ctrl Pts',(8.47818870097126,8.29999999991001,0.706881809970104)) ;
#101650=CARTESIAN_POINT('Ctrl Pts',(8.47075185325581,8.29999999998296,0.699910724672022)) ;
#101651=CARTESIAN_POINT('Ctrl Pts',(8.46347271757075,8.29999999998104,0.692763178993)) ;
#101652=CARTESIAN_POINT('Ctrl Pts',(8.45667934899942,8.29999999998018,0.685187391684601)) ;
#101653=CARTESIAN_POINT('Ctrl Pts',(8.44963335392746,8.29999999997929,0.677329881896828)) ;
#101654=CARTESIAN_POINT('Ctrl Pts',(8.44304226791565,8.29999999996634,0.668999743655032)) ;
#101655=CARTESIAN_POINT('Ctrl Pts',(8.43712466127421,8.29999999997622,0.660333111058006)) ;
#101656=CARTESIAN_POINT('Ctrl Pts',(8.43698358608697,8.29999999997646,0.660126499349853)) ;
#101657=CARTESIAN_POINT('Ctrl Pts',(8.43684287437574,8.29999999997671,0.659919648720668)) ;
#101658=CARTESIAN_POINT('Ctrl Pts',(8.43670252680326,8.29999999997696,0.659712560504486)) ;
#101659=CARTESIAN_POINT('Ctrl Pts',(8.42665365624175,8.29999999999548,0.644885067285366)) ;
#101660=CARTESIAN_POINT('Ctrl Pts',(8.41848789916264,8.29999999999779,0.628865136807051)) ;
#101661=CARTESIAN_POINT('Ctrl Pts',(8.4124226058234,8.29999999999911,0.612081948601152)) ;
#101662=CARTESIAN_POINT('Ctrl Pts',(8.40662497274128,8.30000000000037,0.596039399342023)) ;
#101663=CARTESIAN_POINT('Ctrl Pts',(8.40274598945885,8.3,0.579297806080646)) ;
#101664=CARTESIAN_POINT('Ctrl Pts',(8.40101973895688,8.3,0.562220211658976)) ;
#101665=CARTESIAN_POINT('Ctrl Pts',(8.40034533497805,8.3,0.555548411932522)) ;
#101666=CARTESIAN_POINT('Ctrl Pts',(8.40000003014814,8.3,0.548825326960162)) ;
#101667=CARTESIAN_POINT('Ctrl Pts',(8.4,8.3,0.542072889850983)) ;
#101668=CARTESIAN_POINT('',(8.4,8.3,-0.583654556300909)) ;
#101669=CARTESIAN_POINT('Origin',(10.,7.8,-2.54)) ;
#101670=CARTESIAN_POINT('',(8.56837722373805,8.27720759208727,0.732505116750499)) ;
#101671=CARTESIAN_POINT('',(8.54843785958925,8.28385404680359,0.756019687739306)) ;
#101672=CARTESIAN_POINT('Ctrl Pts',(8.56837722339832,8.27720759220056,0.732505116637743)) ;
#101673=CARTESIAN_POINT('Ctrl Pts',(8.56792584473107,8.27735805175631,0.732995309772253)) ;
#101674=CARTESIAN_POINT('Ctrl Pts',(8.56747319573485,8.27750893475505,0.733484206736226)) ;
#101675=CARTESIAN_POINT('Ctrl Pts',(8.56702308739659,8.2776589708678,0.733975696041276)) ;
#101676=CARTESIAN_POINT('Ctrl Pts',(8.56055949575605,8.27981350141465,0.741033521665688)) ;
#101677=CARTESIAN_POINT('Ctrl Pts',(8.55435459773969,8.28188180075344,0.748371604530841)) ;
#101678=CARTESIAN_POINT('Ctrl Pts',(8.54852002808959,8.28382665730347,0.756014133648572)) ;
#101679=CARTESIAN_POINT('',(8.51539953939799,8.29486682020067,0.769059669877081)) ;
#101680=CARTESIAN_POINT('Origin',(8.52916905055952,8.29027698314683,0.749265529521156)) ;
#101681=CARTESIAN_POINT('',(8.51539501058484,8.29486832980505,-2.54)) ;
#101682=CARTESIAN_POINT('',(9.93162277660169,7.82279240779944,0.959712708838304)) ;
#101683=CARTESIAN_POINT('',(9.93162277660169,7.82279240779944,-2.54)) ;
#101684=CARTESIAN_POINT('',(8.48593528106273,8.30468823964576,0.718764792915145)) ;
#101685=CARTESIAN_POINT('Origin',(10.,6.8,-2.54)) ;
#101686=CARTESIAN_POINT('',(10.,6.8847127088383,0.959712708838305)) ;
#101687=CARTESIAN_POINT('',(10.,7.72792407799439,0.959712708838304)) ;
#101688=CARTESIAN_POINT('',(10.,7.8,0.959712708838304)) ;
#101689=CARTESIAN_POINT('',(10.,7.72792407799439,-2.54)) ;
#101690=CARTESIAN_POINT('',(10.,6.8847127088383,-2.54)) ;
#101691=CARTESIAN_POINT('Origin',(8.5,6.55,-2.54)) ;
#101692=CARTESIAN_POINT('',(8.50816305748853,6.55136011924294,0.777372622108107)) ;
#101693=CARTESIAN_POINT('Ctrl Pts',(8.5081612092262,6.5513602015377,0.777376411528006)) ;
#101694=CARTESIAN_POINT('Ctrl Pts',(8.5098233077521,6.55163721795868,0.778181072182122)) ;
#101695=CARTESIAN_POINT('Ctrl Pts',(8.51162127657737,6.55193687942956,0.778720971558941)) ;
#101696=CARTESIAN_POINT('Ctrl Pts',(8.51523682141473,6.55253947023579,0.779428907664883)) ;
#101697=CARTESIAN_POINT('Ctrl Pts',(8.51710259142427,6.55285043190404,0.77960653206074)) ;
#101698=CARTESIAN_POINT('Ctrl Pts',(8.52217030373272,6.55369505062212,0.779764308873419)) ;
#101699=CARTESIAN_POINT('Ctrl Pts',(8.52587381749938,6.55431230291657,0.779516116605555)) ;
#101700=CARTESIAN_POINT('Ctrl Pts',(8.53482421527959,6.55580403587993,0.778270149815854)) ;
#101701=CARTESIAN_POINT('Ctrl Pts',(8.53952102462637,6.55658683673477,0.776779552576415)) ;
#101702=CARTESIAN_POINT('Ctrl Pts',(8.54640674065797,6.55773445607337,0.773631787754093)) ;
#101703=CARTESIAN_POINT('Ctrl Pts',(8.55013419152225,6.55835569858704,0.771763269769364)) ;
#101704=CARTESIAN_POINT('Ctrl Pts',(8.55581906875147,6.55930317812525,0.767956624570398)) ;
#101705=CARTESIAN_POINT('Ctrl Pts',(8.55861150732124,6.55976858455354,0.76572244443715)) ;
#101706=CARTESIAN_POINT('Ctrl Pts',(8.56125821409731,6.56020970234955,0.762550543343891)) ;
#101707=CARTESIAN_POINT('',(9.91643989873054,6.78607331645509,0.959712708838304)) ;
#101708=CARTESIAN_POINT('',(9.98442535909739,6.79740422651623,0.971043618899446)) ;
#101709=CARTESIAN_POINT('',(9.91643989873054,6.78607331645509,-2.54)) ;
#101710=CARTESIAN_POINT('',(8.50816364570071,6.55136060761679,-2.54)) ;
#101711=CARTESIAN_POINT('Origin',(1.25,6.55,-2.54)) ;
#101712=CARTESIAN_POINT('',(8.49172372711481,6.55000000000007,-0.7694558427306)) ;
#101713=CARTESIAN_POINT('',(8.49172374697018,6.55,-2.54)) ;
#101714=CARTESIAN_POINT('',(8.4,6.55,-0.540678001899701)) ;
#101715=CARTESIAN_POINT('Ctrl Pts',(8.49172374697018,6.55000000000105,-0.769455745655721)) ;
#101716=CARTESIAN_POINT('Ctrl Pts',(8.49606803673628,6.55000000001052,-0.765950586326939)) ;
#101717=CARTESIAN_POINT('Ctrl Pts',(8.50046735944502,6.54999999990302,-0.762511904249297)) ;
#101718=CARTESIAN_POINT('Ctrl Pts',(8.50920280475187,6.55000000136501,-0.755516026702047)) ;
#101719=CARTESIAN_POINT('Ctrl Pts',(8.51365366733357,6.55000000372466,-0.752018918292477)) ;
#101720=CARTESIAN_POINT('Ctrl Pts',(8.51786969589098,6.55000000840872,-0.7475740514919)) ;
#101721=CARTESIAN_POINT('Ctrl Pts',(8.51824835575331,6.5500000088438,-0.747162834355834)) ;
#101722=CARTESIAN_POINT('Ctrl Pts',(8.51893753951064,6.55000000964298,-0.74638941226421)) ;
#101723=CARTESIAN_POINT('Ctrl Pts',(8.51925555226618,6.55000001000021,-0.746024683061041)) ;
#101724=CARTESIAN_POINT('Ctrl Pts',(8.5212536251891,6.55000001218547,-0.743636966400871)) ;
#101725=CARTESIAN_POINT('Ctrl Pts',(8.5228013177651,6.55000000862054,-0.741362521573822)) ;
#101726=CARTESIAN_POINT('Ctrl Pts',(8.52354796988917,6.55000000490364,-0.736217268201258)) ;
#101727=CARTESIAN_POINT('Ctrl Pts',(8.52233587755859,6.5500000056078,-0.733562917823344)) ;
#101728=CARTESIAN_POINT('Ctrl Pts',(8.52032554216557,6.55000000470579,-0.731161010570529)) ;
#101729=CARTESIAN_POINT('Ctrl Pts',(8.52004618744965,6.55000000456892,-0.730855467224597)) ;
#101730=CARTESIAN_POINT('Ctrl Pts',(8.51943244221713,6.55000000425258,-0.730237557550688)) ;
#101731=CARTESIAN_POINT('Ctrl Pts',(8.51910103101863,6.55000000405877,-0.729917277321387)) ;
#101732=CARTESIAN_POINT('Ctrl Pts',(8.51460799223814,6.5500000014124,-0.725734931004252)) ;
#101733=CARTESIAN_POINT('Ctrl Pts',(8.50969722522567,6.55000000036127,-0.722960241153036)) ;
#101734=CARTESIAN_POINT('Ctrl Pts',(8.50463600502766,6.55000000021577,-0.719663474838837)) ;
#101735=CARTESIAN_POINT('Ctrl Pts',(8.50427412871952,6.55000000020764,-0.719427280126575)) ;
#101736=CARTESIAN_POINT('Ctrl Pts',(8.49410349041856,6.55000000002642,-0.712774331281524)) ;
#101737=CARTESIAN_POINT('Ctrl Pts',(8.48448997361529,6.54999999999179,-0.706080938962322)) ;
#101738=CARTESIAN_POINT('Ctrl Pts',(8.46629237463083,6.55000000001684,-0.690977024388696)) ;
#101739=CARTESIAN_POINT('Ctrl Pts',(8.45766562693777,6.55000000000152,-0.682593931661903)) ;
#101740=CARTESIAN_POINT('Ctrl Pts',(8.44955830666695,6.55,-0.673212334268187)) ;
#101741=CARTESIAN_POINT('Ctrl Pts',(8.44937081015221,6.55,-0.672994428311737)) ;
#101742=CARTESIAN_POINT('Ctrl Pts',(8.43720071044349,6.5500000000026,-0.65878927402097)) ;
#101743=CARTESIAN_POINT('Ctrl Pts',(8.42721384365643,6.55000000009149,-0.643256668187946)) ;
#101744=CARTESIAN_POINT('Ctrl Pts',(8.41184903642185,6.55000000007035,-0.610595055314441)) ;
#101745=CARTESIAN_POINT('Ctrl Pts',(8.4063554780816,6.5500000000232,-0.593517332523761)) ;
#101746=CARTESIAN_POINT('Ctrl Pts',(8.40108598764536,6.5499999999995,-0.564358808750087)) ;
#101747=CARTESIAN_POINT('Ctrl Pts',(8.4,6.55,-0.552559527935716)) ;
#101748=CARTESIAN_POINT('Ctrl Pts',(8.4,6.55,-0.540678001899701)) ;
#101749=CARTESIAN_POINT('',(8.4,6.55,0.540678001899701)) ;
#101750=CARTESIAN_POINT('',(8.4,6.55,0.723639392383214)) ;
#101751=CARTESIAN_POINT('',(8.4917237271148,6.5500000000004,0.769455842731608)) ;
#101752=CARTESIAN_POINT('Ctrl Pts',(8.4,6.55000000000001,0.540678001899701)) ;
#101753=CARTESIAN_POINT('Ctrl Pts',(8.4,6.55000000000001,0.558539648405557)) ;
#101754=CARTESIAN_POINT('Ctrl Pts',(8.40245177849658,6.55000000000111,0.57621494191016)) ;
#101755=CARTESIAN_POINT('Ctrl Pts',(8.40709634751528,6.55000000003439,0.593248151244056)) ;
#101756=CARTESIAN_POINT('Ctrl Pts',(8.41193897064627,6.55000000006908,0.611007692158)) ;
#101757=CARTESIAN_POINT('Ctrl Pts',(8.4191659430817,6.55000000013771,0.628071111857661)) ;
#101758=CARTESIAN_POINT('Ctrl Pts',(8.42853896333683,6.55000000013582,0.643918732683401)) ;
#101759=CARTESIAN_POINT('Ctrl Pts',(8.43455058705941,6.55000000013461,0.654083005320109)) ;
#101760=CARTESIAN_POINT('Ctrl Pts',(8.44144611055298,6.55000000009671,0.663746999277865)) ;
#101761=CARTESIAN_POINT('Ctrl Pts',(8.44917210140207,6.55000000005186,0.672767316898348)) ;
#101762=CARTESIAN_POINT('Ctrl Pts',(8.4493621952364,6.55000000005075,0.672989256944207)) ;
#101763=CARTESIAN_POINT('Ctrl Pts',(8.44955278293316,6.55000000004968,0.673210797713723)) ;
#101764=CARTESIAN_POINT('Ctrl Pts',(8.44974386351697,6.55000000004864,0.67343193698325)) ;
#101765=CARTESIAN_POINT('Ctrl Pts',(8.45766118910685,6.55000000000559,0.682594728736607)) ;
#101766=CARTESIAN_POINT('Ctrl Pts',(8.4662887064648,6.54999999999865,0.690978448496742)) ;
#101767=CARTESIAN_POINT('Ctrl Pts',(8.47555348469885,6.55000000000007,0.69866472405094)) ;
#101768=CARTESIAN_POINT('Ctrl Pts',(8.48448851770303,6.55000000000144,0.70607743529141)) ;
#101769=CARTESIAN_POINT('Ctrl Pts',(8.49410273695376,6.5500000000304,0.712765307029448)) ;
#101770=CARTESIAN_POINT('Ctrl Pts',(8.50391213313781,6.55000000016212,0.719176104228815)) ;
#101771=CARTESIAN_POINT('Ctrl Pts',(8.50409415224108,6.55000000016456,0.719295060333305)) ;
#101772=CARTESIAN_POINT('Ctrl Pts',(8.50427622716234,6.55000000016576,0.719413940206856)) ;
#101773=CARTESIAN_POINT('Ctrl Pts',(8.50445835579895,6.55000000016577,0.71953274536795)) ;
#101774=CARTESIAN_POINT('Ctrl Pts',(8.50464048443556,6.55000000016577,0.719651550529044)) ;
#101775=CARTESIAN_POINT('Ctrl Pts',(8.50482266678753,6.55000000016459,0.719770280977681)) ;
#101776=CARTESIAN_POINT('Ctrl Pts',(8.50500490075221,6.55000000016234,0.719888938232344)) ;
#101777=CARTESIAN_POINT('Ctrl Pts',(8.50970297364421,6.55000000010443,0.722947975182689)) ;
#101778=CARTESIAN_POINT('Ctrl Pts',(8.51460443926436,6.55000000028677,0.725724345929427)) ;
#101779=CARTESIAN_POINT('Ctrl Pts',(8.51874830926329,6.55000000038295,0.729563015271579)) ;
#101780=CARTESIAN_POINT('Ctrl Pts',(8.51909542442957,6.550000000391,0.729884565017908)) ;
#101781=CARTESIAN_POINT('Ctrl Pts',(8.51943721516333,6.55000000039357,0.730213585498476)) ;
#101782=CARTESIAN_POINT('Ctrl Pts',(8.51977310187182,6.55000000039098,0.730550883852702)) ;
#101783=CARTESIAN_POINT('Ctrl Pts',(8.52085916897635,6.5500000003826,0.731641515418871)) ;
#101784=CARTESIAN_POINT('Ctrl Pts',(8.52182399801739,6.55000000033868,0.732955379118005)) ;
#101785=CARTESIAN_POINT('Ctrl Pts',(8.52246334063462,6.55000000029842,0.734373233340337)) ;
#101786=CARTESIAN_POINT('Ctrl Pts',(8.52278301194323,6.55000000027828,0.735082160451502)) ;
#101787=CARTESIAN_POINT('Ctrl Pts',(8.52302131164589,6.55000000025926,0.735817085193467)) ;
#101788=CARTESIAN_POINT('Ctrl Pts',(8.52315270869756,6.55000000024662,0.73656310236501)) ;
#101789=CARTESIAN_POINT('Ctrl Pts',(8.52328410574922,6.55000000023398,0.737309119536553)) ;
#101790=CARTESIAN_POINT('Ctrl Pts',(8.5233086001499,6.55000000022778,0.738066229137675)) ;
#101791=CARTESIAN_POINT('Ctrl Pts',(8.52320066085453,6.55000000023233,0.738819525967153)) ;
#101792=CARTESIAN_POINT('Ctrl Pts',(8.52284031330749,6.55000000024754,0.741334353063084)) ;
#101793=CARTESIAN_POINT('Ctrl Pts',(8.52133564423351,6.55000000029586,0.743593261986886)) ;
#101794=CARTESIAN_POINT('Ctrl Pts',(8.5196587899188,6.55000000031744,0.745601348504568)) ;
#101795=CARTESIAN_POINT('Ctrl Pts',(8.51932554032813,6.55000000032173,0.746000425516912)) ;
#101796=CARTESIAN_POINT('Ctrl Pts',(8.51898545723479,6.55000000032523,0.746389624235137)) ;
#101797=CARTESIAN_POINT('Ctrl Pts',(8.51864615038491,6.5500000003277,0.74676898768062)) ;
#101798=CARTESIAN_POINT('Ctrl Pts',(8.5145508165866,6.55000000035749,0.751347792796721)) ;
#101799=CARTESIAN_POINT('Ctrl Pts',(8.50963987409779,6.55000000028078,0.755179791381347)) ;
#101800=CARTESIAN_POINT('Ctrl Pts',(8.50482177382261,6.55000000018958,0.759031129874613)) ;
#101801=CARTESIAN_POINT('Ctrl Pts',(8.50046402923751,6.5500000001071,0.762514483998816)) ;
#101802=CARTESIAN_POINT('Ctrl Pts',(8.49606692679174,6.55000000001227,0.765950989453777)) ;
#101803=CARTESIAN_POINT('Ctrl Pts',(8.49172374697017,6.55000000000105,0.769455745656203)) ;
#101804=CARTESIAN_POINT('',(8.49172374697018,6.55,-2.54)) ;
#101805=CARTESIAN_POINT('',(-0.9,6.55,0.850000000000003)) ;
#101806=CARTESIAN_POINT('',(-0.900000000000001,6.55,-2.54)) ;
#101807=CARTESIAN_POINT('',(1.15,6.55,0.850000000000003)) ;
#101808=CARTESIAN_POINT('',(1.25,6.55,0.850000000000003)) ;
#101809=CARTESIAN_POINT('',(1.35,6.55,0.650000000000003)) ;
#101810=CARTESIAN_POINT('Origin',(1.15,6.55,0.650000000000003)) ;
#101811=CARTESIAN_POINT('',(1.35,6.55,-0.65)) ;
#101812=CARTESIAN_POINT('',(1.35,6.55,-0.75)) ;
#101813=CARTESIAN_POINT('',(1.15,6.55,-0.85)) ;
#101814=CARTESIAN_POINT('Origin',(1.15,6.55,-0.65)) ;
#101815=CARTESIAN_POINT('',(-0.9,6.55,-0.85)) ;
#101816=CARTESIAN_POINT('',(1.25,6.55,-0.85)) ;
#101817=CARTESIAN_POINT('',(-0.9,6.55,-2.54)) ;
#101818=CARTESIAN_POINT('Origin',(1.25,5.3,-2.54)) ;
#101819=CARTESIAN_POINT('',(1.25,3.15,-1.6431676725155)) ;
#101820=CARTESIAN_POINT('',(1.25,3.04189189189189,-1.46552792413544)) ;
#101821=CARTESIAN_POINT('Origin',(1.25,2.95,-1.6431676725155)) ;
#101822=CARTESIAN_POINT('',(1.25,3.15,-2.54)) ;
#101823=CARTESIAN_POINT('',(1.25,4.45,-1.6431676725155)) ;
#101824=CARTESIAN_POINT('',(1.25,4.45,-1.58113883008419)) ;
#101825=CARTESIAN_POINT('',(1.25,4.55810810810811,-1.46552792413544)) ;
#101826=CARTESIAN_POINT('Origin',(1.25,4.65,-1.6431676725155)) ;
#101827=CARTESIAN_POINT('',(1.25,5.26552792413544,-0.758108108108109)) ;
#101828=CARTESIAN_POINT('Origin',(1.25,3.8,0.)) ;
#101829=CARTESIAN_POINT('',(1.25,5.4431676725155,-0.65)) ;
#101830=CARTESIAN_POINT('Origin',(1.25,5.4431676725155,-0.850000000000001)) ;
#101831=CARTESIAN_POINT('',(1.25,6.45,-0.65)) ;
#101832=CARTESIAN_POINT('',(1.25,6.55,-0.65)) ;
#101833=CARTESIAN_POINT('',(1.25,6.45,0.650000000000003)) ;
#101834=CARTESIAN_POINT('',(1.25,6.45,0.750000000000003)) ;
#101835=CARTESIAN_POINT('',(1.25,5.4431676725155,0.650000000000002)) ;
#101836=CARTESIAN_POINT('',(1.25,5.38113883008419,0.650000000000002)) ;
#101837=CARTESIAN_POINT('',(1.25,5.26552792413544,0.75810810810811)) ;
#101838=CARTESIAN_POINT('Origin',(1.25,5.4431676725155,0.850000000000002)) ;
#101839=CARTESIAN_POINT('',(1.25,4.55810810810811,1.46552792413544)) ;
#101840=CARTESIAN_POINT('Origin',(1.25,3.8,0.)) ;
#101841=CARTESIAN_POINT('',(1.25,4.45,1.6431676725155)) ;
#101842=CARTESIAN_POINT('Origin',(1.25,4.65,1.6431676725155)) ;
#101843=CARTESIAN_POINT('',(1.25,4.45,2.54)) ;
#101844=CARTESIAN_POINT('',(1.25,3.15,1.6431676725155)) ;
#101845=CARTESIAN_POINT('',(1.25,3.15,1.58113883008419)) ;
#101846=CARTESIAN_POINT('',(1.25,3.04189189189189,1.46552792413544)) ;
#101847=CARTESIAN_POINT('Origin',(1.25,2.95,1.6431676725155)) ;
#101848=CARTESIAN_POINT('',(1.25,2.33447207586456,0.758108108108108)) ;
#101849=CARTESIAN_POINT('Origin',(1.25,3.8,0.)) ;
#101850=CARTESIAN_POINT('',(1.25,2.1568323274845,0.65)) ;
#101851=CARTESIAN_POINT('Origin',(1.25,2.1568323274845,0.850000000000001)) ;
#101852=CARTESIAN_POINT('',(1.25,0.973783447787483,0.649999999999999)) ;
#101853=CARTESIAN_POINT('',(1.25,0.895262490344437,0.649999999999999)) ;
#101854=CARTESIAN_POINT('',(1.25,0.973783447787483,-0.650000000000001)) ;
#101855=CARTESIAN_POINT('Origin',(1.25,3.8,0.)) ;
#101856=CARTESIAN_POINT('',(1.25,2.1568323274845,-0.65)) ;
#101857=CARTESIAN_POINT('',(1.25,2.21886116991581,-0.65)) ;
#101858=CARTESIAN_POINT('',(1.25,2.33447207586456,-0.758108108108109)) ;
#101859=CARTESIAN_POINT('Origin',(1.25,2.1568323274845,-0.850000000000001)) ;
#101860=CARTESIAN_POINT('Origin',(1.25,3.8,0.)) ;
#101861=CARTESIAN_POINT('Origin',(-2.,0.,-2.54)) ;
#101862=CARTESIAN_POINT('',(0.899999999999999,0.,-1.6)) ;
#101863=CARTESIAN_POINT('',(1.1,0.,-1.4)) ;
#101864=CARTESIAN_POINT('Origin',(0.899999999999999,0.,-1.4)) ;
#101865=CARTESIAN_POINT('',(-2.,0.,-1.6)) ;
#101866=CARTESIAN_POINT('',(-2.,0.,-1.6)) ;
#101867=CARTESIAN_POINT('',(-2.,0.,-2.54)) ;
#101868=CARTESIAN_POINT('',(9.9,0.,-2.54)) ;
#101869=CARTESIAN_POINT('',(-2.,0.,1.6)) ;
#101870=CARTESIAN_POINT('',(-2.,0.,-2.54)) ;
#101871=CARTESIAN_POINT('',(0.899999999999999,0.,1.6)) ;
#101872=CARTESIAN_POINT('',(0.999999999999999,0.,1.6)) ;
#101873=CARTESIAN_POINT('',(1.1,0.,1.4)) ;
#101874=CARTESIAN_POINT('Origin',(0.899999999999999,0.,1.4)) ;
#101875=CARTESIAN_POINT('',(1.1,0.,-1.5)) ;
#101876=CARTESIAN_POINT('Origin',(-2.,7.65,-2.54)) ;
#101877=CARTESIAN_POINT('',(-2.,6.9,1.6)) ;
#101878=CARTESIAN_POINT('',(-2.,7.1,1.4)) ;
#101879=CARTESIAN_POINT('Origin',(-2.,6.9,1.4)) ;
#101880=CARTESIAN_POINT('',(-2.,-1.13380619344889E-17,1.6)) ;
#101881=CARTESIAN_POINT('',(-2.,7.55,-2.54)) ;
#101882=CARTESIAN_POINT('',(-2.,6.9,-1.6)) ;
#101883=CARTESIAN_POINT('',(-2.,7.,-1.6)) ;
#101884=CARTESIAN_POINT('',(-2.,7.1,-1.4)) ;
#101885=CARTESIAN_POINT('Origin',(-2.,6.9,-1.4)) ;
#101886=CARTESIAN_POINT('',(-2.,7.1,1.5)) ;
#101887=CARTESIAN_POINT('Origin',(-1.8,7.,1.5)) ;
#101888=CARTESIAN_POINT('',(-1.7,0.1,1.5)) ;
#101889=CARTESIAN_POINT('',(-1.9,0.1,1.5)) ;
#101890=CARTESIAN_POINT('',(-2.,0.1,1.5)) ;
#101891=CARTESIAN_POINT('',(-1.9,0.3,1.5)) ;
#101892=CARTESIAN_POINT('',(-1.9,7.,1.5)) ;
#101893=CARTESIAN_POINT('Origin',(-1.7,0.3,1.5)) ;
#101894=CARTESIAN_POINT('Origin',(-1.8,7.,-1.5)) ;
#101895=CARTESIAN_POINT('',(-1.9,0.3,-1.5)) ;
#101896=CARTESIAN_POINT('',(-1.7,0.1,-1.5)) ;
#101897=CARTESIAN_POINT('Origin',(-1.7,0.3,-1.5)) ;
#101898=CARTESIAN_POINT('',(-1.9,0.1,-1.5)) ;
#101899=CARTESIAN_POINT('',(-1.9,1.23908819712629E-17,-1.5)) ;
#101900=CARTESIAN_POINT('',(0.999999999999999,0.1,-1.5)) ;
#101901=CARTESIAN_POINT('Origin',(-1.8,-2.2514151555628E-16,-1.7912294869673E-32)) ;
#101902=CARTESIAN_POINT('',(-1.8,4.6,-0.65)) ;
#101903=CARTESIAN_POINT('',(-1.8,4.6,0.65)) ;
#101904=CARTESIAN_POINT('',(-1.8,4.6,0.55)) ;
#101905=CARTESIAN_POINT('',(-1.8,0.3,0.650000000000001)) ;
#101906=CARTESIAN_POINT('',(-1.8,0.2,0.650000000000001)) ;
#101907=CARTESIAN_POINT('',(-1.8,0.3,1.4)) ;
#101908=CARTESIAN_POINT('',(-1.8,0.3,1.5)) ;
#101909=CARTESIAN_POINT('',(-1.8,6.9,1.4)) ;
#101910=CARTESIAN_POINT('',(-1.8,-5.16691679585995E-17,1.4)) ;
#101911=CARTESIAN_POINT('',(-1.8,6.9,-1.4)) ;
#101912=CARTESIAN_POINT('',(-1.8,6.9,-1.7912294869673E-32)) ;
#101913=CARTESIAN_POINT('',(-1.8,0.3,-1.4)) ;
#101914=CARTESIAN_POINT('',(-1.8,-3.98613863153961E-16,-1.4)) ;
#101915=CARTESIAN_POINT('',(-1.8,0.3,-0.65)) ;
#101916=CARTESIAN_POINT('',(-1.8,0.3,-0.550000000000001)) ;
#101917=CARTESIAN_POINT('',(-1.8,4.5,-0.65)) ;
#101918=CARTESIAN_POINT('Origin',(0.549999999999999,4.5,0.55)) ;
#101919=CARTESIAN_POINT('',(-1.7,0.3,0.550000000000001)) ;
#101920=CARTESIAN_POINT('',(-1.7,4.4,0.55)) ;
#101921=CARTESIAN_POINT('',(-1.7,4.5,0.55)) ;
#101922=CARTESIAN_POINT('',(0.45,4.4,0.55)) ;
#101923=CARTESIAN_POINT('',(0.45,4.4,0.55)) ;
#101924=CARTESIAN_POINT('',(0.45,0.3,0.550000000000001)) ;
#101925=CARTESIAN_POINT('',(0.45,4.5,0.55)) ;
#101926=CARTESIAN_POINT('',(0.549999999999999,0.3,0.550000000000001)) ;
#101927=CARTESIAN_POINT('Origin',(0.549999999999999,4.5,-0.549999999999999)) ;
#101928=CARTESIAN_POINT('',(0.45,0.3,-0.55)) ;
#101929=CARTESIAN_POINT('',(0.45,4.4,-0.549999999999999)) ;
#101930=CARTESIAN_POINT('',(0.45,4.5,-0.549999999999999)) ;
#101931=CARTESIAN_POINT('',(-1.7,4.4,-0.55)) ;
#101932=CARTESIAN_POINT('',(-1.7,4.4,-0.549999999999999)) ;
#101933=CARTESIAN_POINT('',(-1.7,0.3,-0.55)) ;
#101934=CARTESIAN_POINT('',(-1.7,0.2,-0.550000000000001)) ;
#101935=CARTESIAN_POINT('',(0.549999999999999,0.3,-0.55)) ;
#101936=CARTESIAN_POINT('Origin',(0.549999999999999,4.5,-0.549999999999999)) ;
#101937=CARTESIAN_POINT('',(-1.7,4.5,0.45)) ;
#101938=CARTESIAN_POINT('',(-1.7,4.5,-0.45)) ;
#101939=CARTESIAN_POINT('',(-1.7,4.5,-0.549999999999999)) ;
#101940=CARTESIAN_POINT('',(0.45,4.5,-0.45)) ;
#101941=CARTESIAN_POINT('',(0.45,4.5,-0.45)) ;
#101942=CARTESIAN_POINT('',(0.45,4.5,0.45)) ;
#101943=CARTESIAN_POINT('',(0.45,4.5,-0.549999999999999)) ;
#101944=CARTESIAN_POINT('',(-1.7,4.5,0.45)) ;
#101945=CARTESIAN_POINT('Origin',(0.55,3.09772049281573E-17,-2.67525834540015E-32)) ;
#101946=CARTESIAN_POINT('',(0.55,2.61224989991992,-0.4)) ;
#101947=CARTESIAN_POINT('',(0.55,2.65280931275608,-0.45)) ;
#101948=CARTESIAN_POINT('Ctrl Pts',(0.55,2.61224989991992,-0.4)) ;
#101949=CARTESIAN_POINT('Ctrl Pts',(0.55,2.61224989991992,-0.403869744161984)) ;
#101950=CARTESIAN_POINT('Ctrl Pts',(0.55,2.61317624258758,-0.408420103915689)) ;
#101951=CARTESIAN_POINT('Ctrl Pts',(0.55,2.61634258087509,-0.416633000858876)) ;
#101952=CARTESIAN_POINT('Ctrl Pts',(0.55,2.61951410407877,-0.421630428645295)) ;
#101953=CARTESIAN_POINT('Ctrl Pts',(0.55,2.63040394024853,-0.43493871907015)) ;
#101954=CARTESIAN_POINT('Ctrl Pts',(0.55,2.64148366881061,-0.443170580967422)) ;
#101955=CARTESIAN_POINT('Ctrl Pts',(0.55,2.65280931275608,-0.449999999999997)) ;
#101956=CARTESIAN_POINT('',(0.55,0.3,-0.450000000000001)) ;
#101957=CARTESIAN_POINT('',(0.55,1.39397422176708E-16,-0.450000000000001)) ;
#101958=CARTESIAN_POINT('',(0.55,0.3,0.450000000000001)) ;
#101959=CARTESIAN_POINT('',(0.55,0.3,0.550000000000001)) ;
#101960=CARTESIAN_POINT('',(0.55,2.65280931275594,0.449999999999914)) ;
#101961=CARTESIAN_POINT('',(0.55,6.35032701027224E-17,0.450000000000001)) ;
#101962=CARTESIAN_POINT('',(0.55,2.61224989991992,0.4)) ;
#101963=CARTESIAN_POINT('Ctrl Pts',(0.55,2.65280931275594,0.449999999999911)) ;
#101964=CARTESIAN_POINT('Ctrl Pts',(0.55,2.64148366881051,0.443170580967354)) ;
#101965=CARTESIAN_POINT('Ctrl Pts',(0.55,2.6304039402485,0.434938719070111)) ;
#101966=CARTESIAN_POINT('Ctrl Pts',(0.55,2.61951410407877,0.421630428645295)) ;
#101967=CARTESIAN_POINT('Ctrl Pts',(0.55,2.61634258087509,0.416633000858876)) ;
#101968=CARTESIAN_POINT('Ctrl Pts',(0.55,2.61317624258758,0.408420103915689)) ;
#101969=CARTESIAN_POINT('Ctrl Pts',(0.55,2.61224989991992,0.403869744161984)) ;
#101970=CARTESIAN_POINT('Ctrl Pts',(0.55,2.61224989991992,0.4)) ;
#101971=CARTESIAN_POINT('',(0.55,2.61224989991992,0.5)) ;
#101972=CARTESIAN_POINT('Origin',(0.,0.2,0.)) ;
#101973=CARTESIAN_POINT('',(-1.7,0.2,-0.65)) ;
#101974=CARTESIAN_POINT('',(-1.7,0.2,-1.4)) ;
#101975=CARTESIAN_POINT('',(-1.7,0.2,-1.5)) ;
#101976=CARTESIAN_POINT('',(0.899999999999999,0.2,-1.4)) ;
#101977=CARTESIAN_POINT('',(0.999999999999999,0.2,-1.4)) ;
#101978=CARTESIAN_POINT('',(0.899999999999999,0.2,1.4)) ;
#101979=CARTESIAN_POINT('',(0.899999999999999,0.2,1.5)) ;
#101980=CARTESIAN_POINT('',(-1.7,0.2,1.4)) ;
#101981=CARTESIAN_POINT('',(-1.8,0.2,1.4)) ;
#101982=CARTESIAN_POINT('',(-1.7,0.2,0.650000000000001)) ;
#101983=CARTESIAN_POINT('',(-1.7,0.2,0.550000000000001)) ;
#101984=CARTESIAN_POINT('',(0.65,0.2,0.650000000000001)) ;
#101985=CARTESIAN_POINT('',(-1.16429916652874E-32,0.2,0.650000000000001)) ;
#101986=CARTESIAN_POINT('',(0.65,0.2,-0.65)) ;
#101987=CARTESIAN_POINT('',(0.65,0.2,-0.550000000000001)) ;
#101988=CARTESIAN_POINT('',(-1.35834902761687E-32,0.2,-0.65)) ;
#101989=CARTESIAN_POINT('Origin',(3.,2.3,-2.54)) ;
#101990=CARTESIAN_POINT('',(3.,4.2,0.5)) ;
#101991=CARTESIAN_POINT('',(3.,3.4,0.5)) ;
#101992=CARTESIAN_POINT('',(3.,2.3,0.5)) ;
#101993=CARTESIAN_POINT('',(3.,4.3,0.4)) ;
#101994=CARTESIAN_POINT('Origin',(3.,4.2,0.4)) ;
#101995=CARTESIAN_POINT('',(3.,4.3,-0.4)) ;
#101996=CARTESIAN_POINT('',(3.,4.3,-2.54)) ;
#101997=CARTESIAN_POINT('',(3.,4.2,-0.5)) ;
#101998=CARTESIAN_POINT('Origin',(3.,4.2,-0.4)) ;
#101999=CARTESIAN_POINT('',(3.,3.4,-0.5)) ;
#102000=CARTESIAN_POINT('',(3.,2.3,-0.5)) ;
#102001=CARTESIAN_POINT('',(3.,3.3,-0.4)) ;
#102002=CARTESIAN_POINT('Origin',(3.,3.4,-0.4)) ;
#102003=CARTESIAN_POINT('',(3.,3.3,0.4)) ;
#102004=CARTESIAN_POINT('',(3.,3.3,-2.54)) ;
#102005=CARTESIAN_POINT('Origin',(3.,3.4,0.4)) ;
#102006=CARTESIAN_POINT('Origin',(-1.,3.8,0.)) ;
#102007=CARTESIAN_POINT('',(-1.,1.6,-1.96214168703487)) ;
#102008=CARTESIAN_POINT('',(-1.,1.55483870967742,-1.83555190077455)) ;
#102009=CARTESIAN_POINT('Origin',(-1.,1.40000000000001,-1.96214168703487)) ;
#102010=CARTESIAN_POINT('',(-1.,1.6,-2.54)) ;
#102011=CARTESIAN_POINT('',(-1.,2.95,-1.6431676725155)) ;
#102012=CARTESIAN_POINT('',(-1.,2.95,-3.80476326321452E-16)) ;
#102013=CARTESIAN_POINT('',(-1.,2.1568323274845,-0.850000000000001)) ;
#102014=CARTESIAN_POINT('Origin',(-1.,3.8,0.)) ;
#102015=CARTESIAN_POINT('',(-1.,1.02736587339765,-0.850000000000001)) ;
#102016=CARTESIAN_POINT('',(-1.,3.8,-0.85)) ;
#102017=CARTESIAN_POINT('Origin',(-1.,3.8,0.)) ;
#102018=CARTESIAN_POINT('Origin',(-1.,3.05,-2.55)) ;
#102019=CARTESIAN_POINT('',(1.15,3.05,-1.6431676725155)) ;
#102020=CARTESIAN_POINT('',(1.15,3.05,-1.58113883008419)) ;
#102021=CARTESIAN_POINT('',(-0.900000000000002,3.05,-1.6431676725155)) ;
#102022=CARTESIAN_POINT('',(-1.,3.05,-1.6431676725155)) ;
#102023=CARTESIAN_POINT('',(-0.900000000000002,3.05,-2.55)) ;
#102024=CARTESIAN_POINT('Origin',(-1.,2.21886116991581,-0.750000000000001)) ;
#102025=CARTESIAN_POINT('',(-0.900000000000002,2.1568323274845,-0.750000000000001)) ;
#102026=CARTESIAN_POINT('',(1.15,2.1568323274845,-0.750000000000001)) ;
#102027=CARTESIAN_POINT('',(1.25,2.1568323274845,-0.750000000000001)) ;
#102028=CARTESIAN_POINT('',(1.15,0.895262490344437,-0.750000000000001)) ;
#102029=CARTESIAN_POINT('',(-0.900000000000002,2.21886116991581,-0.750000000000001)) ;
#102030=CARTESIAN_POINT('Origin',(-1.,3.8,0.)) ;
#102031=CARTESIAN_POINT('',(-0.900000000000002,2.24565220167453,-0.804054054054055)) ;
#102032=CARTESIAN_POINT('',(-0.900000000000001,2.99594594594595,-1.55434779832547)) ;
#102033=CARTESIAN_POINT('Origin',(-0.900000000000001,3.8,0.)) ;
#102034=CARTESIAN_POINT('',(1.15,2.99594594594595,-1.55434779832547)) ;
#102035=CARTESIAN_POINT('',(-1.,2.99594594594595,-1.55434779832547)) ;
#102036=CARTESIAN_POINT('',(1.15,2.24565220167453,-0.804054054054055)) ;
#102037=CARTESIAN_POINT('Origin',(1.15,3.8,0.)) ;
#102038=CARTESIAN_POINT('',(-1.,2.24565220167453,-0.804054054054055)) ;
#102039=CARTESIAN_POINT('Origin',(-1.,3.8,0.)) ;
#102040=CARTESIAN_POINT('',(-0.900000000000002,2.99594594594594,1.55434779832547)) ;
#102041=CARTESIAN_POINT('',(-0.900000000000002,2.24565220167453,0.804054054054054)) ;
#102042=CARTESIAN_POINT('Origin',(-0.900000000000001,3.8,0.)) ;
#102043=CARTESIAN_POINT('',(1.15,2.24565220167453,0.804054054054054)) ;
#102044=CARTESIAN_POINT('',(-1.,2.24565220167453,0.804054054054054)) ;
#102045=CARTESIAN_POINT('',(1.15,2.99594594594594,1.55434779832547)) ;
#102046=CARTESIAN_POINT('Origin',(1.15,3.8,0.)) ;
#102047=CARTESIAN_POINT('',(-1.,2.99594594594594,1.55434779832547)) ;
#102048=CARTESIAN_POINT('Origin',(-1.,2.21886116991581,0.75)) ;
#102049=CARTESIAN_POINT('',(1.15,2.1568323274845,0.75)) ;
#102050=CARTESIAN_POINT('',(1.15,2.21886116991581,0.75)) ;
#102051=CARTESIAN_POINT('',(-0.900000000000002,2.1568323274845,0.75)) ;
#102052=CARTESIAN_POINT('',(-1.,2.1568323274845,0.75)) ;
#102053=CARTESIAN_POINT('',(-0.900000000000002,0.895262490344437,0.749999999999999)) ;
#102054=CARTESIAN_POINT('Origin',(-1.,3.05,2.55)) ;
#102055=CARTESIAN_POINT('',(-0.900000000000002,3.05,1.6431676725155)) ;
#102056=CARTESIAN_POINT('',(1.15,3.05,1.6431676725155)) ;
#102057=CARTESIAN_POINT('',(1.25,3.05,1.6431676725155)) ;
#102058=CARTESIAN_POINT('',(1.15,3.05,2.54)) ;
#102059=CARTESIAN_POINT('',(-0.900000000000002,3.05,1.58113883008419)) ;
#102060=CARTESIAN_POINT('Origin',(-1.,3.8,0.)) ;
#102061=CARTESIAN_POINT('',(-1.,2.1568323274845,0.85)) ;
#102062=CARTESIAN_POINT('',(-1.,2.95,1.6431676725155)) ;
#102063=CARTESIAN_POINT('Origin',(-1.,3.8,0.)) ;
#102064=CARTESIAN_POINT('',(-1.,2.95,2.54)) ;
#102065=CARTESIAN_POINT('',(-1.,1.6,1.96214168703487)) ;
#102066=CARTESIAN_POINT('',(-1.,1.6,0.)) ;
#102067=CARTESIAN_POINT('',(-1.,1.55483870967743,1.83555190077455)) ;
#102068=CARTESIAN_POINT('Origin',(-1.,1.40000000000001,1.96214168703487)) ;
#102069=CARTESIAN_POINT('',(-1.,1.02736587339765,0.849999999999999)) ;
#102070=CARTESIAN_POINT('Origin',(-1.,3.8,0.)) ;
#102071=CARTESIAN_POINT('',(-1.,2.21886116991581,0.850000000000001)) ;
#102072=CARTESIAN_POINT('Origin',(-1.,3.8,0.)) ;
#102073=CARTESIAN_POINT('',(-1.,5.4431676725155,-0.850000000000001)) ;
#102074=CARTESIAN_POINT('',(-1.,4.65,-1.6431676725155)) ;
#102075=CARTESIAN_POINT('Origin',(-1.,3.8,0.)) ;
#102076=CARTESIAN_POINT('',(-1.,4.65,0.)) ;
#102077=CARTESIAN_POINT('',(-1.,6.45,-0.85)) ;
#102078=CARTESIAN_POINT('',(-1.,6.45,-0.75)) ;
#102079=CARTESIAN_POINT('',(-1.,3.8,-0.850000000000001)) ;
#102080=CARTESIAN_POINT('Origin',(-1.,4.55,-1.58113883008419)) ;
#102081=CARTESIAN_POINT('',(-0.900000000000001,4.55,-1.6431676725155)) ;
#102082=CARTESIAN_POINT('',(1.15,4.55,-1.6431676725155)) ;
#102083=CARTESIAN_POINT('',(1.25,4.55,-1.6431676725155)) ;
#102084=CARTESIAN_POINT('',(1.15,4.55,-2.54)) ;
#102085=CARTESIAN_POINT('',(-0.900000000000001,4.55,-1.58113883008419)) ;
#102086=CARTESIAN_POINT('Origin',(-1.,3.8,0.)) ;
#102087=CARTESIAN_POINT('',(-0.900000000000001,4.60405405405406,-1.55434779832547)) ;
#102088=CARTESIAN_POINT('',(-0.900000000000001,5.35434779832547,-0.804054054054054)) ;
#102089=CARTESIAN_POINT('Origin',(-0.900000000000001,3.8,0.)) ;
#102090=CARTESIAN_POINT('',(1.15,5.35434779832547,-0.804054054054055)) ;
#102091=CARTESIAN_POINT('',(-1.,5.35434779832547,-0.804054054054055)) ;
#102092=CARTESIAN_POINT('',(1.15,4.60405405405405,-1.55434779832547)) ;
#102093=CARTESIAN_POINT('Origin',(1.15,3.8,0.)) ;
#102094=CARTESIAN_POINT('',(-1.,4.60405405405406,-1.55434779832547)) ;
#102095=CARTESIAN_POINT('Origin',(-1.,6.55,-0.75)) ;
#102096=CARTESIAN_POINT('',(-0.900000000000001,5.4431676725155,-0.75)) ;
#102097=CARTESIAN_POINT('',(-0.9,6.45,-0.75)) ;
#102098=CARTESIAN_POINT('',(-0.9,6.55,-0.75)) ;
#102099=CARTESIAN_POINT('',(1.15,6.45,-0.75)) ;
#102100=CARTESIAN_POINT('',(-1.,6.45,-0.75)) ;
#102101=CARTESIAN_POINT('',(1.15,5.4431676725155,-0.75)) ;
#102102=CARTESIAN_POINT('',(1.15,5.38113883008419,-0.75)) ;
#102103=CARTESIAN_POINT('',(-1.,5.4431676725155,-0.75)) ;
#102104=CARTESIAN_POINT('Origin',(-1.,3.8,0.)) ;
#102105=CARTESIAN_POINT('',(-0.900000000000001,5.35434779832547,0.804054054054056)) ;
#102106=CARTESIAN_POINT('',(-0.900000000000001,4.60405405405405,1.55434779832547)) ;
#102107=CARTESIAN_POINT('Origin',(-0.900000000000001,3.8,0.)) ;
#102108=CARTESIAN_POINT('',(1.15,4.60405405405405,1.55434779832547)) ;
#102109=CARTESIAN_POINT('',(-1.,4.60405405405405,1.55434779832547)) ;
#102110=CARTESIAN_POINT('',(1.15,5.35434779832547,0.804054054054056)) ;
#102111=CARTESIAN_POINT('Origin',(1.15,3.8,0.)) ;
#102112=CARTESIAN_POINT('',(-1.,5.35434779832547,0.804054054054056)) ;
#102113=CARTESIAN_POINT('Origin',(-1.,4.55,1.58113883008419)) ;
#102114=CARTESIAN_POINT('',(1.15,4.55,1.6431676725155)) ;
#102115=CARTESIAN_POINT('',(1.15,4.55,1.58113883008419)) ;
#102116=CARTESIAN_POINT('',(-0.900000000000001,4.55,1.6431676725155)) ;
#102117=CARTESIAN_POINT('',(-1.,4.55,1.6431676725155)) ;
#102118=CARTESIAN_POINT('',(-0.900000000000001,4.55,2.54)) ;
#102119=CARTESIAN_POINT('Origin',(-1.,6.55,0.750000000000003)) ;
#102120=CARTESIAN_POINT('',(1.15,5.4431676725155,0.750000000000002)) ;
#102121=CARTESIAN_POINT('',(1.15,6.45,0.750000000000003)) ;
#102122=CARTESIAN_POINT('',(1.15,6.55,0.750000000000003)) ;
#102123=CARTESIAN_POINT('',(-0.9,6.45,0.750000000000003)) ;
#102124=CARTESIAN_POINT('',(-1.,6.45,0.750000000000003)) ;
#102125=CARTESIAN_POINT('',(-0.900000000000001,5.4431676725155,0.750000000000002)) ;
#102126=CARTESIAN_POINT('',(-0.900000000000001,5.38113883008419,0.750000000000002)) ;
#102127=CARTESIAN_POINT('',(1.25,5.4431676725155,0.750000000000002)) ;
#102128=CARTESIAN_POINT('Origin',(-1.,3.8,0.)) ;
#102129=CARTESIAN_POINT('',(-1.,5.4431676725155,0.850000000000002)) ;
#102130=CARTESIAN_POINT('',(-1.,6.45,0.850000000000003)) ;
#102131=CARTESIAN_POINT('',(-1.,6.55,0.850000000000003)) ;
#102132=CARTESIAN_POINT('',(-1.,6.45,0.)) ;
#102133=CARTESIAN_POINT('',(-1.,4.65,1.6431676725155)) ;
#102134=CARTESIAN_POINT('',(-1.,4.65,1.58113883008419)) ;
#102135=CARTESIAN_POINT('Origin',(-1.,3.8,0.)) ;
#102136=CARTESIAN_POINT('Origin',(10.,4.35421736843756,-0.875)) ;
#102137=CARTESIAN_POINT('',(9.91643989873054,7.72792407799439,-0.86107331645509)) ;
#102138=CARTESIAN_POINT('',(8.58356010126947,8.17221734381475,-0.638926683544911)) ;
#102139=CARTESIAN_POINT('',(8.47075240319158,8.20981990984071,-0.62012540053193)) ;
#102140=CARTESIAN_POINT('',(8.58356010126947,6.66256607592813,-0.638926683544911)) ;
#102141=CARTESIAN_POINT('',(8.58356010126947,6.64863939238321,-0.638926683544911)) ;
#102142=CARTESIAN_POINT('',(9.91643989873054,6.8847127088383,-0.86107331645509)) ;
#102143=CARTESIAN_POINT('',(9.98442535909739,6.89604361889945,-0.872404226516232)) ;
#102144=CARTESIAN_POINT('',(9.91643989873054,7.8,-0.86107331645509)) ;
#102145=CARTESIAN_POINT('Origin',(8.5,4.35421736843756,-0.625)) ;
#102146=CARTESIAN_POINT('',(8.5,8.17221734381475,-0.540287291161696)) ;
#102147=CARTESIAN_POINT('',(8.50000000129681,8.20000000266558,-0.542105625353022)) ;
#102148=CARTESIAN_POINT('Origin',(8.5,8.17870774541185,-0.729037639375355)) ;
#102149=CARTESIAN_POINT('',(8.5,8.2,0.583654556300909)) ;
#102150=CARTESIAN_POINT('',(8.5,6.66256607592813,0.540287291161697)) ;
#102151=CARTESIAN_POINT('',(8.5,6.64863939238321,0.540287291161696)) ;
#102152=CARTESIAN_POINT('',(8.50000000002143,6.64999999935441,0.540682155673763)) ;
#102153=CARTESIAN_POINT('Origin',(8.5,6.65811550095888,0.736811514826147)) ;
#102154=CARTESIAN_POINT('',(8.49999999999933,6.65000073218972,-0.540689690963651)) ;
#102155=CARTESIAN_POINT('',(8.5,6.65,-0.723639392383214)) ;
#102156=CARTESIAN_POINT('',(8.5,6.66256607592813,-0.540287291161696)) ;
#102157=CARTESIAN_POINT('Origin',(8.5,6.65133313751723,-0.737010066702972)) ;
#102158=CARTESIAN_POINT('',(8.5,8.20007071090457,-0.540287291161696)) ;
#102159=CARTESIAN_POINT('Origin',(8.5,4.35421736843756,0.625)) ;
#102160=CARTESIAN_POINT('',(9.91643989873054,6.8847127088383,0.86107331645509)) ;
#102161=CARTESIAN_POINT('',(8.58356010126947,6.66256607592813,0.638926683544911)) ;
#102162=CARTESIAN_POINT('',(8.48442535909739,6.64604361889945,0.622404226516231)) ;
#102163=CARTESIAN_POINT('',(8.58356010126947,8.20007071090456,0.638926683544911)) ;
#102164=CARTESIAN_POINT('',(9.91643989873054,7.72792407799439,0.86107331645509)) ;
#102165=CARTESIAN_POINT('',(9.97075240319158,7.70981990984071,0.87012540053193)) ;
#102166=CARTESIAN_POINT('',(9.91643989873054,6.8,0.86107331645509)) ;
#102167=CARTESIAN_POINT('Origin',(8.5,3.65,0.5)) ;
#102168=CARTESIAN_POINT('',(8.45734623443633,3.62014236410543,0.0979344438426624)) ;
#102169=CARTESIAN_POINT('',(8.02582401135442,3.3180768079481,0.4)) ;
#102170=CARTESIAN_POINT('',(8.34729988159781,3.54310991711847,0.174966890829628)) ;
#102171=CARTESIAN_POINT('',(8.02582401135442,3.31807680794809,-0.4)) ;
#102172=CARTESIAN_POINT('',(8.02582401135442,3.3180768079481,0.5)) ;
#102173=CARTESIAN_POINT('',(8.45734623443633,3.62014236410543,-0.0979344438426621)) ;
#102174=CARTESIAN_POINT('',(8.70083523513316,3.79058466459322,0.0725078566451196)) ;
#102175=CARTESIAN_POINT('',(8.45734623443633,3.62014236410543,0.5)) ;
#102176=CARTESIAN_POINT('Origin',(8.5,3.95,0.5)) ;
#102177=CARTESIAN_POINT('',(8.5,3.89793444384266,-0.0979344438426626)) ;
#102178=CARTESIAN_POINT('',(8.5,3.89793444384266,0.0979344438426625)) ;
#102179=CARTESIAN_POINT('',(8.5,3.89793444384266,0.5)) ;
#102180=CARTESIAN_POINT('',(8.5,3.70206555615734,0.0979344438426625)) ;
#102181=CARTESIAN_POINT('',(8.5,3.95,0.0979344438426625)) ;
#102182=CARTESIAN_POINT('',(8.5,3.70206555615734,-0.0979344438426626)) ;
#102183=CARTESIAN_POINT('',(8.5,3.70206555615734,0.5)) ;
#102184=CARTESIAN_POINT('',(8.5,3.95,-0.0979344438426626)) ;
#102185=CARTESIAN_POINT('Origin',(8.,4.3,0.5)) ;
#102186=CARTESIAN_POINT('',(8.45734623443633,3.97985763589457,-0.0979344438426625)) ;
#102187=CARTESIAN_POINT('',(8.02582401135442,4.2819231920519,-0.4)) ;
#102188=CARTESIAN_POINT('',(8.32457260887054,4.07279917379062,-0.190875981738719)) ;
#102189=CARTESIAN_POINT('',(8.02582401135442,4.2819231920519,0.4)) ;
#102190=CARTESIAN_POINT('',(8.02582401135442,4.2819231920519,0.5)) ;
#102191=CARTESIAN_POINT('',(8.45734623443633,3.97985763589457,0.0979344438426624)) ;
#102192=CARTESIAN_POINT('',(7.97103725533518,4.32027392126537,0.438350729213466)) ;
#102193=CARTESIAN_POINT('',(8.45734623443633,3.97985763589457,0.5)) ;
#102194=CARTESIAN_POINT('Origin',(1.5,2.3,0.5)) ;
#102195=CARTESIAN_POINT('',(7.96847777691809,3.4,0.5)) ;
#102196=CARTESIAN_POINT('',(8.,3.4,0.5)) ;
#102197=CARTESIAN_POINT('',(7.96847777691809,4.2,0.5)) ;
#102198=CARTESIAN_POINT('',(7.96847777691809,4.2,0.5)) ;
#102199=CARTESIAN_POINT('',(3.,4.2,0.5)) ;
#102200=CARTESIAN_POINT('Origin',(1.5,2.3,-0.5)) ;
#102201=CARTESIAN_POINT('',(7.96847777691809,4.2,-0.5)) ;
#102202=CARTESIAN_POINT('',(1.5,4.2,-0.5)) ;
#102203=CARTESIAN_POINT('',(7.96847777691809,3.4,-0.5)) ;
#102204=CARTESIAN_POINT('',(7.96847777691809,2.3,-0.5)) ;
#102205=CARTESIAN_POINT('',(1.5,3.4,-0.5)) ;
#102206=CARTESIAN_POINT('Origin',(8.,3.3,0.5)) ;
#102207=CARTESIAN_POINT('',(7.96847777691809,3.3,-0.4)) ;
#102208=CARTESIAN_POINT('',(8.,3.3,-0.4)) ;
#102209=CARTESIAN_POINT('',(7.96847777691809,3.3,0.4)) ;
#102210=CARTESIAN_POINT('',(7.96847777691809,3.3,0.5)) ;
#102211=CARTESIAN_POINT('',(3.,3.3,0.4)) ;
#102212=CARTESIAN_POINT('Origin',(1.5,4.3,0.5)) ;
#102213=CARTESIAN_POINT('',(7.96847777691809,4.3,0.4)) ;
#102214=CARTESIAN_POINT('',(8.,4.3,0.4)) ;
#102215=CARTESIAN_POINT('',(7.96847777691809,4.3,-0.4)) ;
#102216=CARTESIAN_POINT('',(7.96847777691809,4.3,0.5)) ;
#102217=CARTESIAN_POINT('',(1.5,4.3,-0.4)) ;
#102218=CARTESIAN_POINT('Origin',(1.5,2.3,0.5)) ;
#102219=CARTESIAN_POINT('',(-0.4,2.3,0.5)) ;
#102220=CARTESIAN_POINT('',(-0.4,-3.36847777691809,0.5)) ;
#102221=CARTESIAN_POINT('',(-0.4,-3.4,0.5)) ;
#102222=CARTESIAN_POINT('',(0.4,-3.36847777691809,0.5)) ;
#102223=CARTESIAN_POINT('',(0.4,-3.36847777691809,0.5)) ;
#102224=CARTESIAN_POINT('',(0.4,2.29999999999999,0.5)) ;
#102225=CARTESIAN_POINT('',(0.4,2.29999999999999,0.5)) ;
#102226=CARTESIAN_POINT('',(0.536602540378444,2.83090991212703,0.5)) ;
#102227=CARTESIAN_POINT('Origin',(1.5,2.3,0.5)) ;
#102228=CARTESIAN_POINT('',(0.536602540378444,3.93764017256378,0.5)) ;
#102229=CARTESIAN_POINT('',(0.536602540378444,2.83090991212703,0.5)) ;
#102230=CARTESIAN_POINT('Origin',(1.5,2.3,0.5)) ;
#102231=CARTESIAN_POINT('Origin',(1.5,2.3,-0.5)) ;
#102232=CARTESIAN_POINT('',(0.4,2.29999999999999,-0.5)) ;
#102233=CARTESIAN_POINT('',(0.4,-3.36847777691809,-0.5)) ;
#102234=CARTESIAN_POINT('',(0.4,2.3,-0.5)) ;
#102235=CARTESIAN_POINT('',(-0.4,-3.36847777691809,-0.5)) ;
#102236=CARTESIAN_POINT('',(1.5,-3.36847777691809,-0.5)) ;
#102237=CARTESIAN_POINT('',(-0.4,2.3,-0.5)) ;
#102238=CARTESIAN_POINT('',(-0.4,2.3,-0.5)) ;
#102239=CARTESIAN_POINT('',(0.536602540378444,3.93764017256378,-0.5)) ;
#102240=CARTESIAN_POINT('Origin',(1.5,2.3,-0.5)) ;
#102241=CARTESIAN_POINT('',(0.536602540378444,2.83090991212703,-0.5)) ;
#102242=CARTESIAN_POINT('',(0.536602540378444,3.93764017256378,-0.5)) ;
#102243=CARTESIAN_POINT('Origin',(1.5,2.3,-0.5)) ;
#102244=CARTESIAN_POINT('Origin',(1.5,2.3,0.5)) ;
#102245=CARTESIAN_POINT('',(-0.5,2.3,0.4)) ;
#102246=CARTESIAN_POINT('',(-0.5,2.3,-0.4)) ;
#102247=CARTESIAN_POINT('',(-0.5,2.3,0.5)) ;
#102248=CARTESIAN_POINT('Origin',(1.5,2.3,0.4)) ;
#102249=CARTESIAN_POINT('Origin',(1.5,2.3,-0.4)) ;
#102250=CARTESIAN_POINT('Origin',(-0.5,-3.4,0.5)) ;
#102251=CARTESIAN_POINT('',(-0.5,-3.36847777691809,-0.4)) ;
#102252=CARTESIAN_POINT('',(-0.5,-3.4,-0.4)) ;
#102253=CARTESIAN_POINT('',(-0.5,-3.36847777691809,0.4)) ;
#102254=CARTESIAN_POINT('',(-0.5,-3.36847777691809,0.5)) ;
#102255=CARTESIAN_POINT('',(-0.5,2.3,0.4)) ;
#102256=CARTESIAN_POINT('Origin',(-0.15,-3.9,0.5)) ;
#102257=CARTESIAN_POINT('',(-0.179857635894567,-3.85734623443633,0.0979344438426625)) ;
#102258=CARTESIAN_POINT('',(-0.481923192051905,-3.42582401135442,0.4)) ;
#102259=CARTESIAN_POINT('',(-0.256890082881532,-3.74729988159781,0.174966890829628)) ;
#102260=CARTESIAN_POINT('',(-0.481923192051905,-3.42582401135442,-0.4)) ;
#102261=CARTESIAN_POINT('',(-0.481923192051905,-3.42582401135442,0.5)) ;
#102262=CARTESIAN_POINT('',(-0.179857635894567,-3.85734623443633,-0.0979344438426628)) ;
#102263=CARTESIAN_POINT('',(-0.00941533540678435,-4.10083523513317,0.0725078566451196)) ;
#102264=CARTESIAN_POINT('',(-0.179857635894567,-3.85734623443633,0.5)) ;
#102265=CARTESIAN_POINT('Origin',(0.15,-3.9,0.5)) ;
#102266=CARTESIAN_POINT('',(0.0979344438426627,-3.9,-0.0979344438426626)) ;
#102267=CARTESIAN_POINT('',(0.0979344438426627,-3.9,0.0979344438426627)) ;
#102268=CARTESIAN_POINT('',(0.0979344438426627,-3.9,0.5)) ;
#102269=CARTESIAN_POINT('',(-0.0979344438426628,-3.9,0.0979344438426627)) ;
#102270=CARTESIAN_POINT('',(0.15,-3.9,0.0979344438426627)) ;
#102271=CARTESIAN_POINT('',(-0.0979344438426628,-3.9,-0.0979344438426626)) ;
#102272=CARTESIAN_POINT('',(-0.0979344438426628,-3.9,0.5)) ;
#102273=CARTESIAN_POINT('',(0.15,-3.9,-0.0979344438426626)) ;
#102274=CARTESIAN_POINT('Origin',(0.5,-3.4,0.5)) ;
#102275=CARTESIAN_POINT('',(0.179857635894567,-3.85734623443633,-0.0979344438426625)) ;
#102276=CARTESIAN_POINT('',(0.481923192051904,-3.42582401135442,-0.4)) ;
#102277=CARTESIAN_POINT('',(0.272799173790623,-3.72457260887054,-0.190875981738719)) ;
#102278=CARTESIAN_POINT('',(0.481923192051904,-3.42582401135442,0.4)) ;
#102279=CARTESIAN_POINT('',(0.481923192051904,-3.42582401135442,0.5)) ;
#102280=CARTESIAN_POINT('',(0.179857635894567,-3.85734623443633,0.0979344438426627)) ;
#102281=CARTESIAN_POINT('',(0.520273921265371,-3.37103725533519,0.438350729213466)) ;
#102282=CARTESIAN_POINT('',(0.179857635894567,-3.85734623443633,0.5)) ;
#102283=CARTESIAN_POINT('Origin',(0.5,2.29999999999999,0.5)) ;
#102284=CARTESIAN_POINT('',(0.500000000000001,2.29999999999999,0.4)) ;
#102285=CARTESIAN_POINT('',(0.5,-3.36847777691809,0.4)) ;
#102286=CARTESIAN_POINT('',(0.5,-3.4,0.4)) ;
#102287=CARTESIAN_POINT('',(0.5,-3.36847777691809,-0.4)) ;
#102288=CARTESIAN_POINT('',(0.5,-3.36847777691809,0.5)) ;
#102289=CARTESIAN_POINT('',(0.500000000000001,2.29999999999999,-0.4)) ;
#102290=CARTESIAN_POINT('',(0.5,2.29999999999999,-0.4)) ;
#102291=CARTESIAN_POINT('',(0.500000000000001,2.29999999999999,0.5)) ;
#102292=CARTESIAN_POINT('Origin',(1.5,2.3,0.5)) ;
#102293=CARTESIAN_POINT('Origin',(1.5,2.3,0.4)) ;
#102294=CARTESIAN_POINT('Origin',(1.5,2.3,-0.4)) ;
#102295=CARTESIAN_POINT('Origin',(8.,2.68967221921331,-0.5)) ;
#102296=CARTESIAN_POINT('',(8.45734623443633,3.70206555615734,-0.179857635894567)) ;
#102297=CARTESIAN_POINT('',(8.02582401135442,3.4,-0.481923192051904)) ;
#102298=CARTESIAN_POINT('',(7.75526480758232,3.21060855735952,-0.671314634692378)) ;
#102299=CARTESIAN_POINT('',(8.02582401135442,4.2,-0.481923192051904)) ;
#102300=CARTESIAN_POINT('',(8.02582401135442,2.68967221921331,-0.481923192051904)) ;
#102301=CARTESIAN_POINT('',(8.45734623443633,3.89793444384266,-0.179857635894567)) ;
#102302=CARTESIAN_POINT('',(8.54034505662341,3.83983526831171,-0.121758460363615)) ;
#102303=CARTESIAN_POINT('',(8.45734623443633,2.68967221921331,-0.179857635894566)) ;
#102304=CARTESIAN_POINT('Origin',(8.,2.68967221921331,0.5)) ;
#102305=CARTESIAN_POINT('',(8.45734623443633,3.89793444384266,0.179857635894567)) ;
#102306=CARTESIAN_POINT('',(8.02582401135442,4.2,0.481923192051904)) ;
#102307=CARTESIAN_POINT('',(8.54034505662341,3.83983526831171,0.121758460363615)) ;
#102308=CARTESIAN_POINT('',(8.02582401135442,3.4,0.481923192051904)) ;
#102309=CARTESIAN_POINT('',(8.02582401135442,3.4,0.481923192051904)) ;
#102310=CARTESIAN_POINT('',(8.45734623443633,3.70206555615734,0.179857635894567)) ;
#102311=CARTESIAN_POINT('',(7.75526480758232,3.21060855735952,0.671314634692378)) ;
#102312=CARTESIAN_POINT('',(8.45734623443633,2.68967221921331,0.179857635894566)) ;
#102313=CARTESIAN_POINT('Origin',(-1.11032778078669,-3.9,0.15)) ;
#102314=CARTESIAN_POINT('',(0.0979344438426626,-3.85734623443633,0.179857635894567)) ;
#102315=CARTESIAN_POINT('',(0.4,-3.42582401135442,0.481923192051904)) ;
#102316=CARTESIAN_POINT('',(-0.223548570072128,-4.31660768288603,-0.141625378020224)) ;
#102317=CARTESIAN_POINT('',(-0.400000000000001,-3.42582401135442,0.481923192051904)) ;
#102318=CARTESIAN_POINT('',(-0.400000000000001,-3.42582401135442,0.481923192051904)) ;
#102319=CARTESIAN_POINT('',(-0.0979344438426627,-3.85734623443633,0.179857635894567)) ;
#102320=CARTESIAN_POINT('',(-0.326007604256636,-3.53152743384494,0.40793079630854)) ;
#102321=CARTESIAN_POINT('',(-1.11032778078669,-3.85734623443633,0.179857635894567)) ;
#102322=CARTESIAN_POINT('Origin',(-1.11032778078669,-3.4,-0.5)) ;
#102323=CARTESIAN_POINT('',(-0.0979344438426627,-3.85734623443633,-0.179857635894567)) ;
#102324=CARTESIAN_POINT('',(-0.4,-3.42582401135442,-0.481923192051904)) ;
#102325=CARTESIAN_POINT('',(-0.589391442640475,-3.15526480758232,-0.671314634692378)) ;
#102326=CARTESIAN_POINT('',(0.400000000000001,-3.42582401135442,-0.481923192051904)) ;
#102327=CARTESIAN_POINT('',(-1.11032778078669,-3.42582401135442,-0.481923192051904)) ;
#102328=CARTESIAN_POINT('',(0.0979344438426626,-3.85734623443633,-0.179857635894567)) ;
#102329=CARTESIAN_POINT('',(0.0398352683117103,-3.94034505662341,-0.121758460363614)) ;
#102330=CARTESIAN_POINT('',(-1.11032778078669,-3.85734623443633,-0.179857635894567)) ;
#102331=CARTESIAN_POINT('Origin',(10.,1.24999999999998,-2.54)) ;
#102332=CARTESIAN_POINT('',(9.91643989873054,1.26392668354489,2.0441618801782)) ;
#102333=CARTESIAN_POINT('',(9.91643989873054,1.26392668354489,-2.54)) ;
#102334=CARTESIAN_POINT('',(8.50816364570057,1.49863939238321,1.96214168703487)) ;
#102335=CARTESIAN_POINT('Origin',(43.7052916412087,-4.36754860759459,-606.688201691247)) ;
#102336=CARTESIAN_POINT('',(8.50816364570057,1.49863939238321,-2.54)) ;
#102337=CARTESIAN_POINT('Origin',(8.49999999999985,3.8,0.)) ;
#102338=CARTESIAN_POINT('',(9.91643989873053,1.24322097942674,1.98369643580595)) ;
#102339=CARTESIAN_POINT('',(9.91643989873053,1.24322097942648,-1.98369643580562)) ;
#102340=CARTESIAN_POINT('Origin',(9.91643989873053,3.8,0.)) ;
#102341=CARTESIAN_POINT('Origin',(36.5480652843801,-40.3802619076193,572.277654833716)) ;
#102342=CARTESIAN_POINT('Origin',(36.548065291501,-40.3802618709639,-572.277654846232)) ;
#102343=CARTESIAN_POINT('Origin',(10.,1.24999999999998,-2.54)) ;
#102344=CARTESIAN_POINT('',(8.50816364570059,1.49863939238321,-1.96214168703472)) ;
#102345=CARTESIAN_POINT('',(8.50816364570057,1.49863939238321,-2.54)) ;
#102346=CARTESIAN_POINT('',(9.91643989873054,1.26392668354489,-2.04416188017819)) ;
#102347=CARTESIAN_POINT('Origin',(43.7052916405325,-4.36754860730519,606.688201680236)) ;
#102348=CARTESIAN_POINT('',(9.91643989873054,1.26392668354489,-2.54)) ;
#102349=CARTESIAN_POINT('Origin',(-0.900000000000001,4.65,0.)) ;
#102350=CARTESIAN_POINT('Origin',(-0.900000000000001,4.65,1.6431676725155)) ;
#102351=CARTESIAN_POINT('Origin',(-0.900000000000001,4.65,1.6431676725155)) ;
#102352=CARTESIAN_POINT('Origin',(-0.900000000000001,4.65,1.6431676725155)) ;
#102353=CARTESIAN_POINT('Origin',(-0.900000000000001,4.65,1.6431676725155)) ;
#102354=CARTESIAN_POINT('Origin',(1.15,4.45,1.58113883008419)) ;
#102355=CARTESIAN_POINT('Origin',(1.15,4.45,1.6431676725155)) ;
#102356=CARTESIAN_POINT('Origin',(-1.,4.65,1.6431676725155)) ;
#102357=CARTESIAN_POINT('Origin',(1.15,4.65,1.6431676725155)) ;
#102358=CARTESIAN_POINT('Origin',(-0.900000000000001,3.8,0.)) ;
#102359=CARTESIAN_POINT('Origin',(-0.900000000000001,5.4431676725155,0.850000000000002)) ;
#102360=CARTESIAN_POINT('Origin',(1.15,4.65,1.6431676725155)) ;
#102361=CARTESIAN_POINT('Origin',(1.15,4.55810810810811,1.46552792413544)) ;
#102362=CARTESIAN_POINT('Origin',(-0.900000000000001,5.4431676725155,0.850000000000002)) ;
#102363=CARTESIAN_POINT('Origin',(-0.900000000000001,5.4431676725155,0.850000000000002)) ;
#102364=CARTESIAN_POINT('Origin',(-0.900000000000001,5.4431676725155,0.850000000000002)) ;
#102365=CARTESIAN_POINT('Origin',(-0.900000000000001,4.65,0.)) ;
#102366=CARTESIAN_POINT('Origin',(-0.900000000000001,4.65,-1.6431676725155)) ;
#102367=CARTESIAN_POINT('Origin',(-1.,4.65,-1.6431676725155)) ;
#102368=CARTESIAN_POINT('Origin',(1.15,4.65,-1.6431676725155)) ;
#102369=CARTESIAN_POINT('Origin',(-0.900000000000001,4.65,-1.6431676725155)) ;
#102370=CARTESIAN_POINT('Origin',(1.15,4.45,-1.58113883008419)) ;
#102371=CARTESIAN_POINT('Origin',(1.15,4.45,-1.6431676725155)) ;
#102372=CARTESIAN_POINT('Origin',(1.15,3.8,0.)) ;
#102373=CARTESIAN_POINT('Origin',(1.15,5.26552792413544,0.75810810810811)) ;
#102374=CARTESIAN_POINT('Origin',(-1.,5.4431676725155,0.850000000000002)) ;
#102375=CARTESIAN_POINT('Origin',(1.15,5.4431676725155,0.850000000000002)) ;
#102376=CARTESIAN_POINT('Origin',(-0.900000000000001,3.8,0.850000000000001)) ;
#102377=CARTESIAN_POINT('Origin',(-0.9,6.45,0.850000000000003)) ;
#102378=CARTESIAN_POINT('Origin',(-0.9,6.45,0.)) ;
#102379=CARTESIAN_POINT('Origin',(-0.9,6.45,0.850000000000003)) ;
#102380=CARTESIAN_POINT('Origin',(-0.900000000000001,4.65,-1.6431676725155)) ;
#102381=CARTESIAN_POINT('Origin',(-0.900000000000001,4.65,-1.6431676725155)) ;
#102382=CARTESIAN_POINT('Origin',(1.15,4.65,-1.6431676725155)) ;
#102383=CARTESIAN_POINT('Origin',(1.15,4.55810810810811,-1.46552792413544)) ;
#102384=CARTESIAN_POINT('Origin',(1.15,5.4431676725155,0.850000000000002)) ;
#102385=CARTESIAN_POINT('Origin',(1.15,5.4431676725155,0.650000000000002)) ;
#102386=CARTESIAN_POINT('Origin',(-0.9,6.45,0.850000000000003)) ;
#102387=CARTESIAN_POINT('Origin',(-0.9,6.45,0.850000000000003)) ;
#102388=CARTESIAN_POINT('Origin',(-0.900000000000001,3.8,0.)) ;
#102389=CARTESIAN_POINT('Origin',(-0.900000000000001,5.4431676725155,-0.850000000000001)) ;
#102390=CARTESIAN_POINT('Origin',(-1.,5.4431676725155,-0.850000000000001)) ;
#102391=CARTESIAN_POINT('Origin',(1.15,5.4431676725155,-0.850000000000001)) ;
#102392=CARTESIAN_POINT('Origin',(-0.900000000000001,5.4431676725155,-0.850000000000001)) ;
#102393=CARTESIAN_POINT('Origin',(1.15,3.8,0.)) ;
#102394=CARTESIAN_POINT('Origin',(1.15,5.26552792413544,-0.758108108108109)) ;
#102395=CARTESIAN_POINT('Origin',(1.15,6.55,0.650000000000003)) ;
#102396=CARTESIAN_POINT('Origin',(1.15,6.45,0.650000000000003)) ;
#102397=CARTESIAN_POINT('Origin',(1.25,6.45,0.850000000000003)) ;
#102398=CARTESIAN_POINT('Origin',(1.15,6.45,0.850000000000003)) ;
#102399=CARTESIAN_POINT('Origin',(-0.900000000000001,5.4431676725155,-0.850000000000001)) ;
#102400=CARTESIAN_POINT('Origin',(-0.900000000000001,5.4431676725155,-0.850000000000001)) ;
#102401=CARTESIAN_POINT('Origin',(1.15,5.4431676725155,-0.850000000000001)) ;
#102402=CARTESIAN_POINT('Origin',(1.15,5.4431676725155,-0.65)) ;
#102403=CARTESIAN_POINT('Origin',(1.15,6.45,0.650000000000003)) ;
#102404=CARTESIAN_POINT('Origin',(1.35,6.45,0.650000000000003)) ;
#102405=CARTESIAN_POINT('Origin',(-0.9,6.45,0.)) ;
#102406=CARTESIAN_POINT('Origin',(-0.9,6.45,-0.85)) ;
#102407=CARTESIAN_POINT('Origin',(-0.900000000000001,3.8,-0.850000000000001)) ;
#102408=CARTESIAN_POINT('Origin',(-0.9,6.45,-0.85)) ;
#102409=CARTESIAN_POINT('Origin',(1.15,6.55,-0.65)) ;
#102410=CARTESIAN_POINT('Origin',(1.15,6.45,-0.65)) ;
#102411=CARTESIAN_POINT('Origin',(1.35,6.45,-2.54)) ;
#102412=CARTESIAN_POINT('Origin',(1.35,6.45,-0.65)) ;
#102413=CARTESIAN_POINT('Origin',(-0.9,6.45,-0.85)) ;
#102414=CARTESIAN_POINT('Origin',(-0.9,6.45,-0.85)) ;
#102415=CARTESIAN_POINT('Origin',(1.15,6.45,-0.65)) ;
#102416=CARTESIAN_POINT('Origin',(1.15,6.45,-0.85)) ;
#102417=CARTESIAN_POINT('Origin',(-1.,6.45,-0.85)) ;
#102418=CARTESIAN_POINT('Origin',(-1.7,0.3,-0.65)) ;
#102419=CARTESIAN_POINT('Origin',(-1.7,0.3,-0.65)) ;
#102420=CARTESIAN_POINT('Origin',(-1.7,0.3,-0.65)) ;
#102421=CARTESIAN_POINT('Origin',(-1.7,0.3,-0.65)) ;
#102422=CARTESIAN_POINT('Origin',(0.549999999999999,0.3,-0.65)) ;
#102423=CARTESIAN_POINT('',(0.50857864376269,0.229289321881345,-0.579289321881346)) ;
#102424=CARTESIAN_POINT('Ctrl Pts',(0.65,0.2,-0.650000000000001)) ;
#102425=CARTESIAN_POINT('Ctrl Pts',(0.639834283464162,0.2,-0.644917141732082)) ;
#102426=CARTESIAN_POINT('Ctrl Pts',(0.629316849080556,0.200389688120422,
-0.639657683858013)) ;
#102427=CARTESIAN_POINT('Ctrl Pts',(0.606957334719702,0.202165884217644,
-0.628467949719354)) ;
#102428=CARTESIAN_POINT('Ctrl Pts',(0.595086727401132,0.203647820493439,
-0.622522761794938)) ;
#102429=CARTESIAN_POINT('Ctrl Pts',(0.572283837380418,0.207685608831266,
-0.611106760395993)) ;
#102430=CARTESIAN_POINT('Ctrl Pts',(0.561337481650347,0.210178193248346,
-0.605629861308006)) ;
#102431=CARTESIAN_POINT('Ctrl Pts',(0.549549942885282,0.213544620665578,
-0.599740696039287)) ;
#102432=CARTESIAN_POINT('Ctrl Pts',(0.548290718945597,0.213913346522004,
-0.599111682766023)) ;
#102433=CARTESIAN_POINT('Ctrl Pts',(0.536119229732665,0.217566912232542,
-0.593032751351762)) ;
#102434=CARTESIAN_POINT('Ctrl Pts',(0.525706917362415,0.221400308602604,
-0.587842238429113)) ;
#102435=CARTESIAN_POINT('Ctrl Pts',(0.51354511002719,0.226871185484683,
-0.5817711869643)) ;
#102436=CARTESIAN_POINT('Ctrl Pts',(0.511029334128286,0.228063976698547,
-0.580514667064143)) ;
#102437=CARTESIAN_POINT('Ctrl Pts',(0.50857864376269,0.229289321881345,
-0.579289321881346)) ;
#102438=CARTESIAN_POINT('Origin',(0.664280054304529,0.302990743362704,-0.657142104251322)) ;
#102439=CARTESIAN_POINT('Origin',(-1.7,4.5,-0.65)) ;
#102440=CARTESIAN_POINT('',(-1.77071067811866,4.45857864376269,-0.579289321881345)) ;
#102441=CARTESIAN_POINT('Origin',(-1.69703459697416,4.61417009505667,-0.657086685382634)) ;
#102442=CARTESIAN_POINT('Ctrl Pts',(-1.77071067811866,4.45857864376269,
-0.579289321881348)) ;
#102443=CARTESIAN_POINT('Ctrl Pts',(-1.77521675558368,4.46759079869274,
-0.583795399346371)) ;
#102444=CARTESIAN_POINT('Ctrl Pts',(-1.77928079264423,4.47748625817287,
-0.588726481671654)) ;
#102445=CARTESIAN_POINT('Ctrl Pts',(-1.78624680748625,4.49811277056867,
-0.599020882547782)) ;
#102446=CARTESIAN_POINT('Ctrl Pts',(-1.7891803078179,4.50880509433462,-0.604363984149067)) ;
#102447=CARTESIAN_POINT('Ctrl Pts',(-1.7918598550029,4.52101859322019,-0.610474754532795)) ;
#102448=CARTESIAN_POINT('Ctrl Pts',(-1.79213045061227,4.52228751722695,
-0.611109709908939)) ;
#102449=CARTESIAN_POINT('Ctrl Pts',(-1.7947746790983,4.53504937002861,-0.617496289133973)) ;
#102450=CARTESIAN_POINT('Ctrl Pts',(-1.79657370273654,4.54677936428205,
-0.623371572406224)) ;
#102451=CARTESIAN_POINT('Ctrl Pts',(-1.79896007643137,4.569200258884,-0.634595774761239)) ;
#102452=CARTESIAN_POINT('Ctrl Pts',(-1.79963010255188,4.57990192168164,
-0.639950075945062)) ;
#102453=CARTESIAN_POINT('Ctrl Pts',(-1.79996164986963,4.59357116034304,
-0.646785573817069)) ;
#102454=CARTESIAN_POINT('Ctrl Pts',(-1.8,4.59680282631918,-0.648401413159594)) ;
#102455=CARTESIAN_POINT('Ctrl Pts',(-1.8,4.6,-0.65)) ;
#102456=CARTESIAN_POINT('Origin',(-1.7,0.3,-1.5225450639222E-32)) ;
#102457=CARTESIAN_POINT('Origin',(-1.7,0.3,-1.4)) ;
#102458=CARTESIAN_POINT('Origin',(0.65,0.3,1.72609413621187E-32)) ;
#102459=CARTESIAN_POINT('',(0.579289321881342,0.229289321881349,-0.508578643762698)) ;
#102460=CARTESIAN_POINT('Origin',(0.657086685384304,0.30296540302664,-0.664170095060029)) ;
#102461=CARTESIAN_POINT('Ctrl Pts',(0.579289321881342,0.229289321881349,
-0.508578643762698)) ;
#102462=CARTESIAN_POINT('Ctrl Pts',(0.583795399346366,0.224783244416324,
-0.517590798692747)) ;
#102463=CARTESIAN_POINT('Ctrl Pts',(0.588726481671643,0.220719207355776,
-0.527486258172869)) ;
#102464=CARTESIAN_POINT('Ctrl Pts',(0.599020882547802,0.213753192513734,
-0.548112770568737)) ;
#102465=CARTESIAN_POINT('Ctrl Pts',(0.604363984149125,0.210819692182067,
-0.558805094334768)) ;
#102466=CARTESIAN_POINT('Ctrl Pts',(0.610474754532853,0.208140144997073,
-0.571018593220337)) ;
#102467=CARTESIAN_POINT('Ctrl Pts',(0.611109709908958,0.207869549387722,
-0.572287517227017)) ;
#102468=CARTESIAN_POINT('Ctrl Pts',(0.617496289133948,0.205225320901705,
-0.585049370028594)) ;
#102469=CARTESIAN_POINT('Ctrl Pts',(0.623371572406196,0.20342629726347,
-0.596779364282033)) ;
#102470=CARTESIAN_POINT('Ctrl Pts',(0.634595774761209,0.201039923568639,
-0.619200258883972)) ;
#102471=CARTESIAN_POINT('Ctrl Pts',(0.639950075945033,0.20036989744812,
-0.629901921681599)) ;
#102472=CARTESIAN_POINT('Ctrl Pts',(0.646785573817052,0.200038350130375,
-0.643571160343016)) ;
#102473=CARTESIAN_POINT('Ctrl Pts',(0.648401413159585,0.2,-0.646802826319172)) ;
#102474=CARTESIAN_POINT('Ctrl Pts',(0.65,0.2,-0.65)) ;
#102475=CARTESIAN_POINT('',(0.579289321881342,0.229289321881349,0.508578643762698)) ;
#102476=CARTESIAN_POINT('Ctrl Pts',(0.65,0.2,0.650000000000001)) ;
#102477=CARTESIAN_POINT('Ctrl Pts',(0.644917141732077,0.2,0.639834283464156)) ;
#102478=CARTESIAN_POINT('Ctrl Pts',(0.639657683858002,0.200389688120423,
0.629316849080544)) ;
#102479=CARTESIAN_POINT('Ctrl Pts',(0.62846794971934,0.202165884217647,
0.606957334719689)) ;
#102480=CARTESIAN_POINT('Ctrl Pts',(0.622522761794926,0.203647820493443,
0.595086727401124)) ;
#102481=CARTESIAN_POINT('Ctrl Pts',(0.611106760395994,0.207685608831266,
0.572283837380437)) ;
#102482=CARTESIAN_POINT('Ctrl Pts',(0.605629861308018,0.210178193248342,
0.561337481650389)) ;
#102483=CARTESIAN_POINT('Ctrl Pts',(0.599740696039299,0.213544620665571,
0.549549942885324)) ;
#102484=CARTESIAN_POINT('Ctrl Pts',(0.599111682766026,0.213913346522003,
0.54829071894562)) ;
#102485=CARTESIAN_POINT('Ctrl Pts',(0.593032751351754,0.217566912232547,
0.536119229732666)) ;
#102486=CARTESIAN_POINT('Ctrl Pts',(0.587842238429105,0.22140030860261,
0.525706917362413)) ;
#102487=CARTESIAN_POINT('Ctrl Pts',(0.581771186964293,0.22687118548469,
0.51354511002719)) ;
#102488=CARTESIAN_POINT('Ctrl Pts',(0.580514667064138,0.228063976698553,
0.51102933412829)) ;
#102489=CARTESIAN_POINT('Ctrl Pts',(0.579289321881342,0.229289321881349,
0.508578643762698)) ;
#102490=CARTESIAN_POINT('Origin',(0.657142104251401,0.302990743362705,0.664280054304728)) ;
#102491=CARTESIAN_POINT('Origin',(-1.7,4.6,-0.549999999999999)) ;
#102492=CARTESIAN_POINT('',(-1.77071067811866,4.52928932188135,-0.508578643762691)) ;
#102493=CARTESIAN_POINT('Ctrl Pts',(-1.8,4.6,-0.65)) ;
#102494=CARTESIAN_POINT('Ctrl Pts',(-1.8,4.59491714173209,-0.639834283464162)) ;
#102495=CARTESIAN_POINT('Ctrl Pts',(-1.79961031187958,4.58965768385802,
-0.629316849080557)) ;
#102496=CARTESIAN_POINT('Ctrl Pts',(-1.79783411578236,4.57846794971937,
-0.606957334719712)) ;
#102497=CARTESIAN_POINT('Ctrl Pts',(-1.79635217950657,4.57252276179496,
-0.595086727401151)) ;
#102498=CARTESIAN_POINT('Ctrl Pts',(-1.7923143911687,4.56110676039589,-0.57228383738021)) ;
#102499=CARTESIAN_POINT('Ctrl Pts',(-1.78982180675156,4.55562986130779,
-0.561337481649912)) ;
#102500=CARTESIAN_POINT('Ctrl Pts',(-1.7864553793343,4.54974069603908,-0.549549942884871)) ;
#102501=CARTESIAN_POINT('Ctrl Pts',(-1.78608665347794,4.54911168276593,
-0.548290718945413)) ;
#102502=CARTESIAN_POINT('Ctrl Pts',(-1.78243308776747,4.54303275135178,
-0.536119229732704)) ;
#102503=CARTESIAN_POINT('Ctrl Pts',(-1.77859969139741,4.53784223842913,
-0.525706917362452)) ;
#102504=CARTESIAN_POINT('Ctrl Pts',(-1.77312881451533,4.53177118696431,
-0.513545110027213)) ;
#102505=CARTESIAN_POINT('Ctrl Pts',(-1.77193602330146,4.53051466706415,
-0.511029334128298)) ;
#102506=CARTESIAN_POINT('Ctrl Pts',(-1.77071067811866,4.52928932188135,
-0.508578643762691)) ;
#102507=CARTESIAN_POINT('Origin',(-1.69700925663759,4.60714210425063,-0.664280054303076)) ;
#102508=CARTESIAN_POINT('',(-1.77071067811866,4.52928932188135,0.508578643762691)) ;
#102509=CARTESIAN_POINT('Origin',(-1.69703459697298,4.60708668538534,0.664170095062018)) ;
#102510=CARTESIAN_POINT('Ctrl Pts',(-1.77071067811866,4.52928932188135,
0.508578643762691)) ;
#102511=CARTESIAN_POINT('Ctrl Pts',(-1.77521675558368,4.53379539934637,
0.517590798692744)) ;
#102512=CARTESIAN_POINT('Ctrl Pts',(-1.77928079264423,4.53872648167165,
0.52748625817287)) ;
#102513=CARTESIAN_POINT('Ctrl Pts',(-1.78624680748627,4.54902088254781,
0.548112770568734)) ;
#102514=CARTESIAN_POINT('Ctrl Pts',(-1.78918030781794,4.55436398414913,
0.558805094334758)) ;
#102515=CARTESIAN_POINT('Ctrl Pts',(-1.79185985500293,4.56047475453286,
0.571018593220325)) ;
#102516=CARTESIAN_POINT('Ctrl Pts',(-1.79213045061228,4.56110970990897,
0.572287517227011)) ;
#102517=CARTESIAN_POINT('Ctrl Pts',(-1.7947746790983,4.56749628913396,0.585049370028587)) ;
#102518=CARTESIAN_POINT('Ctrl Pts',(-1.79657370273653,4.5733715724062,0.596779364282017)) ;
#102519=CARTESIAN_POINT('Ctrl Pts',(-1.79896007643136,4.58459577476122,
0.619200258883955)) ;
#102520=CARTESIAN_POINT('Ctrl Pts',(-1.79963010255188,4.58995007594504,
0.629901921681588)) ;
#102521=CARTESIAN_POINT('Ctrl Pts',(-1.79996164986962,4.59678557381705,
0.643571160343013)) ;
#102522=CARTESIAN_POINT('Ctrl Pts',(-1.8,4.59840141315959,0.64680282631917)) ;
#102523=CARTESIAN_POINT('Ctrl Pts',(-1.8,4.6,0.65)) ;
#102524=CARTESIAN_POINT('Origin',(-1.7,0.3,-1.4)) ;
#102525=CARTESIAN_POINT('Origin',(-1.7,0.1,-1.4)) ;
#102526=CARTESIAN_POINT('Origin',(-1.9,0.3,-1.4)) ;
#102527=CARTESIAN_POINT('Origin',(1.9668402209837E-32,0.1,-1.4)) ;
#102528=CARTESIAN_POINT('',(0.899999999999999,0.1,-1.5)) ;
#102529=CARTESIAN_POINT('',(-1.8,0.1,-1.5)) ;
#102530=CARTESIAN_POINT('Origin',(0.899999999999999,0.1,-1.4)) ;
#102531=CARTESIAN_POINT('Origin',(0.899999999999999,0.1,-1.4)) ;
#102532=CARTESIAN_POINT('',(0.999999999999999,0.1,-1.4)) ;
#102533=CARTESIAN_POINT('Origin',(0.899999999999999,0.1,-1.4)) ;
#102534=CARTESIAN_POINT('Origin',(0.899999999999999,0.1,-1.4)) ;
#102535=CARTESIAN_POINT('Origin',(0.549999999999999,0.3,0.650000000000001)) ;
#102536=CARTESIAN_POINT('',(0.50857864376269,0.229289321881345,0.579289321881346)) ;
#102537=CARTESIAN_POINT('Origin',(0.664170095060202,0.302965403026731,0.657086685384413)) ;
#102538=CARTESIAN_POINT('Ctrl Pts',(0.50857864376269,0.229289321881345,
0.579289321881346)) ;
#102539=CARTESIAN_POINT('Ctrl Pts',(0.51759079869273,0.224783244416326,
0.583795399346365)) ;
#102540=CARTESIAN_POINT('Ctrl Pts',(0.527486258172839,0.220719207355783,
0.588726481671636)) ;
#102541=CARTESIAN_POINT('Ctrl Pts',(0.54811277056867,0.213753192513749,
0.599020882547779)) ;
#102542=CARTESIAN_POINT('Ctrl Pts',(0.558805094334679,0.210819692182086,
0.60436398414909)) ;
#102543=CARTESIAN_POINT('Ctrl Pts',(0.571018593220245,0.208140144997089,
0.610474754532817)) ;
#102544=CARTESIAN_POINT('Ctrl Pts',(0.572287517226946,0.207869549387733,
0.611109709908932)) ;
#102545=CARTESIAN_POINT('Ctrl Pts',(0.58504937002854,0.205225320901711,
0.617496289133931)) ;
#102546=CARTESIAN_POINT('Ctrl Pts',(0.596779364281974,0.203426297263476,
0.623371572406175)) ;
#102547=CARTESIAN_POINT('Ctrl Pts',(0.61920025888392,0.201039923568642,
0.634595774761189)) ;
#102548=CARTESIAN_POINT('Ctrl Pts',(0.629901921681556,0.200369897448122,
0.639950075945017)) ;
#102549=CARTESIAN_POINT('Ctrl Pts',(0.643571160342994,0.200038350130376,
0.646785573817043)) ;
#102550=CARTESIAN_POINT('Ctrl Pts',(0.646802826319161,0.2,0.648401413159581)) ;
#102551=CARTESIAN_POINT('Ctrl Pts',(0.65,0.2,0.650000000000001)) ;
#102552=CARTESIAN_POINT('Origin',(-1.7,0.3,0.650000000000001)) ;
#102553=CARTESIAN_POINT('Origin',(-1.7,4.5,0.65)) ;
#102554=CARTESIAN_POINT('',(-1.77071067811866,4.45857864376269,0.579289321881346)) ;
#102555=CARTESIAN_POINT('Ctrl Pts',(-1.8,4.6,0.65)) ;
#102556=CARTESIAN_POINT('Ctrl Pts',(-1.8,4.58983428346415,0.644917141732085)) ;
#102557=CARTESIAN_POINT('Ctrl Pts',(-1.79961031187958,4.57931684908054,
0.639657683858016)) ;
#102558=CARTESIAN_POINT('Ctrl Pts',(-1.79783411578236,4.55695733471967,
0.628467949719358)) ;
#102559=CARTESIAN_POINT('Ctrl Pts',(-1.79635217950656,4.5450867274011,0.622522761794939)) ;
#102560=CARTESIAN_POINT('Ctrl Pts',(-1.79231439116879,4.5222838373807,0.611106760396153)) ;
#102561=CARTESIAN_POINT('Ctrl Pts',(-1.7898218067518,4.51133748165095,0.605629861308319)) ;
#102562=CARTESIAN_POINT('Ctrl Pts',(-1.7864553793346,4.49954994288585,0.599740696039583)) ;
#102563=CARTESIAN_POINT('Ctrl Pts',(-1.78608665347808,4.49829071894586,
0.599111682766165)) ;
#102564=CARTESIAN_POINT('Ctrl Pts',(-1.78243308776745,4.48611922973263,
0.593032751351754)) ;
#102565=CARTESIAN_POINT('Ctrl Pts',(-1.77859969139739,4.47570691736239,
0.587842238429103)) ;
#102566=CARTESIAN_POINT('Ctrl Pts',(-1.77312881451531,4.46354511002718,
0.581771186964297)) ;
#102567=CARTESIAN_POINT('Ctrl Pts',(-1.77193602330145,4.46102933412828,
0.580514667064141)) ;
#102568=CARTESIAN_POINT('Ctrl Pts',(-1.77071067811866,4.45857864376269,
0.579289321881348)) ;
#102569=CARTESIAN_POINT('Origin',(-1.6970092566387,4.61428005429881,0.657142104248473)) ;
#102570=CARTESIAN_POINT('Origin',(-1.7,0.3,0.650000000000001)) ;
#102571=CARTESIAN_POINT('Origin',(-1.9,-4.11004745125224E-16,-1.4)) ;
#102572=CARTESIAN_POINT('',(-1.9,6.9,-1.5)) ;
#102573=CARTESIAN_POINT('Origin',(-1.9,6.9,-1.4)) ;
#102574=CARTESIAN_POINT('',(-1.9,7.,-1.5)) ;
#102575=CARTESIAN_POINT('Origin',(-2.,0.1,-1.6)) ;
#102576=CARTESIAN_POINT('Origin',(-1.89999999999999,0.100000000000007,-1.6)) ;
#102577=CARTESIAN_POINT('Origin',(0.899999999999999,0.1,-1.6)) ;
#102578=CARTESIAN_POINT('Origin',(0.899999999999999,0.1,-1.4)) ;
#102579=CARTESIAN_POINT('Origin',(1.1,0.1,-1.4)) ;
#102580=CARTESIAN_POINT('Origin',(0.899999999999999,0.1,6.50521303491302E-17)) ;
#102581=CARTESIAN_POINT('',(0.999999999999999,0.1,1.4)) ;
#102582=CARTESIAN_POINT('',(0.999999999999999,0.1,-1.5)) ;
#102583=CARTESIAN_POINT('Origin',(0.899999999999999,0.1,1.4)) ;
#102584=CARTESIAN_POINT('Origin',(-1.7,0.3,0.650000000000001)) ;
#102585=CARTESIAN_POINT('Origin',(-1.7,0.3,0.650000000000001)) ;
#102586=CARTESIAN_POINT('Origin',(-1.9,6.9,-1.4)) ;
#102587=CARTESIAN_POINT('',(-1.9,7.,-1.4)) ;
#102588=CARTESIAN_POINT('Origin',(-1.9,6.9,-1.4)) ;
#102589=CARTESIAN_POINT('Origin',(-1.9,6.9,-1.4)) ;
#102590=CARTESIAN_POINT('Origin',(-1.9,7.,-1.6)) ;
#102591=CARTESIAN_POINT('Origin',(-1.9,6.9,-1.6)) ;
#102592=CARTESIAN_POINT('Origin',(1.1,0.1,1.5)) ;
#102593=CARTESIAN_POINT('Origin',(1.1,0.1,1.4)) ;
#102594=CARTESIAN_POINT('Origin',(0.899999999999999,0.1,1.4)) ;
#102595=CARTESIAN_POINT('',(0.899999999999999,0.1,1.5)) ;
#102596=CARTESIAN_POINT('Origin',(0.899999999999999,0.1,1.4)) ;
#102597=CARTESIAN_POINT('Origin',(0.899999999999999,0.1,1.4)) ;
#102598=CARTESIAN_POINT('Origin',(-1.7,0.3,-1.5225450639222E-32)) ;
#102599=CARTESIAN_POINT('Origin',(-1.7,0.3,1.4)) ;
#102600=CARTESIAN_POINT('Origin',(-1.9,6.9,-1.88079096131566E-32)) ;
#102601=CARTESIAN_POINT('',(-1.9,7.,1.4)) ;
#102602=CARTESIAN_POINT('Origin',(-1.9,6.9,1.4)) ;
#102603=CARTESIAN_POINT('',(-1.9,7.,-1.5)) ;
#102604=CARTESIAN_POINT('Origin',(-1.9,6.9,-1.4)) ;
#102605=CARTESIAN_POINT('Origin',(-1.9,7.1,-1.4)) ;
#102606=CARTESIAN_POINT('Origin',(0.899999999999999,0.1,1.4)) ;
#102607=CARTESIAN_POINT('Origin',(0.899999999999999,0.1,1.6)) ;
#102608=CARTESIAN_POINT('Origin',(-1.9668402209837E-32,0.1,1.4)) ;
#102609=CARTESIAN_POINT('',(0.999999999999999,0.1,1.5)) ;
#102610=CARTESIAN_POINT('Origin',(-1.7,0.1,1.4)) ;
#102611=CARTESIAN_POINT('Origin',(-1.7,0.3,1.4)) ;
#102612=CARTESIAN_POINT('Origin',(-1.9,0.3,1.4)) ;
#102613=CARTESIAN_POINT('Origin',(-1.9,6.9,1.4)) ;
#102614=CARTESIAN_POINT('',(-1.9,6.9,1.5)) ;
#102615=CARTESIAN_POINT('Origin',(-1.9,6.9,1.4)) ;
#102616=CARTESIAN_POINT('Origin',(-1.9,6.9,1.4)) ;
#102617=CARTESIAN_POINT('Origin',(-1.9,7.1,-1.5)) ;
#102618=CARTESIAN_POINT('Origin',(-1.9,7.1,1.4)) ;
#102619=CARTESIAN_POINT('Origin',(-1.8,0.1,1.6)) ;
#102620=CARTESIAN_POINT('Origin',(-1.9,0.0999999999999979,1.6)) ;
#102621=CARTESIAN_POINT('Origin',(-1.9,-6.40600499298624E-17,1.4)) ;
#102622=CARTESIAN_POINT('',(-1.9,7.,1.5)) ;
#102623=CARTESIAN_POINT('Origin',(-1.9,6.9,1.4)) ;
#102624=CARTESIAN_POINT('Origin',(-1.9,6.9,1.6)) ;
#102625=CARTESIAN_POINT('Origin',(-1.9,7.,1.6)) ;
#102626=CARTESIAN_POINT('Origin',(-0.900000000000002,2.95,-3.80476326321452E-16)) ;
#102627=CARTESIAN_POINT('Origin',(-0.900000000000001,2.95,-1.6431676725155)) ;
#102628=CARTESIAN_POINT('Origin',(-0.900000000000002,2.95,-1.6431676725155)) ;
#102629=CARTESIAN_POINT('Origin',(-0.900000000000001,2.95,-1.6431676725155)) ;
#102630=CARTESIAN_POINT('Origin',(-0.900000000000002,2.95,-1.6431676725155)) ;
#102631=CARTESIAN_POINT('Origin',(1.15,3.15,-2.55)) ;
#102632=CARTESIAN_POINT('Origin',(1.15,3.15,-1.6431676725155)) ;
#102633=CARTESIAN_POINT('Origin',(-1.,2.95,-1.6431676725155)) ;
#102634=CARTESIAN_POINT('Origin',(1.15,2.95,-1.6431676725155)) ;
#102635=CARTESIAN_POINT('Origin',(-0.900000000000001,3.8,0.)) ;
#102636=CARTESIAN_POINT('Origin',(-0.900000000000002,2.1568323274845,-0.850000000000001)) ;
#102637=CARTESIAN_POINT('Origin',(-0.900000000000002,1.6,0.)) ;
#102638=CARTESIAN_POINT('Origin',(-0.900000000000002,1.6,-1.96214168703487)) ;
#102639=CARTESIAN_POINT('Origin',(13.9153543900904,1.4,-1.96214168703487)) ;
#102640=CARTESIAN_POINT('Origin',(8.49172374697002,1.4,-1.96214168703487)) ;
#102641=CARTESIAN_POINT('Origin',(-0.900000000000001,1.40000000000001,-1.96214168703487)) ;
#102642=CARTESIAN_POINT('Origin',(1.15,2.95,-1.6431676725155)) ;
#102643=CARTESIAN_POINT('Origin',(1.15,3.04189189189189,-1.46552792413544)) ;
#102644=CARTESIAN_POINT('Origin',(-0.900000000000002,2.1568323274845,-0.850000000000001)) ;
#102645=CARTESIAN_POINT('Origin',(-0.900000000000002,2.1568323274845,-0.850000000000001)) ;
#102646=CARTESIAN_POINT('Origin',(-0.900000000000002,2.1568323274845,-0.850000000000001)) ;
#102647=CARTESIAN_POINT('Origin',(-0.900000000000001,1.40000000000001,-1.96214168703487)) ;
#102648=CARTESIAN_POINT('Origin',(-0.900000000000002,1.55483870967742,-1.83555190077455)) ;
#102649=CARTESIAN_POINT('Origin',(1.15,3.8,0.)) ;
#102650=CARTESIAN_POINT('Origin',(1.15,2.33447207586456,-0.758108108108109)) ;
#102651=CARTESIAN_POINT('Origin',(-1.,2.1568323274845,-0.850000000000001)) ;
#102652=CARTESIAN_POINT('Origin',(1.15,2.1568323274845,-0.850000000000001)) ;
#102653=CARTESIAN_POINT('Origin',(-0.900000000000001,3.8,-0.85)) ;
#102654=CARTESIAN_POINT('Origin',(-0.900000000000002,1.02736587339765,-0.850000000000001)) ;
#102655=CARTESIAN_POINT('Origin',(-0.900000000000001,3.8,0.)) ;
#102656=CARTESIAN_POINT('Origin',(-0.900000000000002,1.02736587339765,-0.850000000000001)) ;
#102657=CARTESIAN_POINT('Origin',(13.9153543900904,1.4,1.96214168703487)) ;
#102658=CARTESIAN_POINT('Origin',(8.49172374697002,1.4,1.96214168703487)) ;
#102659=CARTESIAN_POINT('Origin',(-0.900000000000001,1.40000000000001,1.96214168703487)) ;
#102660=CARTESIAN_POINT('Origin',(-0.900000000000002,1.6,0.)) ;
#102661=CARTESIAN_POINT('Origin',(-0.900000000000002,1.6,1.96214168703487)) ;
#102662=CARTESIAN_POINT('Origin',(-0.900000000000002,2.95,3.80476326321453E-16)) ;
#102663=CARTESIAN_POINT('Origin',(-0.900000000000002,2.95,1.6431676725155)) ;
#102664=CARTESIAN_POINT('Origin',(1.15,2.1568323274845,-0.850000000000001)) ;
#102665=CARTESIAN_POINT('Origin',(1.15,2.1568323274845,-0.65)) ;
#102666=CARTESIAN_POINT('Origin',(-0.900000000000002,1.02736587339765,-0.850000000000001)) ;
#102667=CARTESIAN_POINT('Origin',(-0.900000000000001,1.40000000000001,1.96214168703487)) ;
#102668=CARTESIAN_POINT('Origin',(-0.900000000000002,1.55483870967743,1.83555190077455)) ;
#102669=CARTESIAN_POINT('Origin',(-0.900000000000002,2.95,1.6431676725155)) ;
#102670=CARTESIAN_POINT('Origin',(-0.900000000000002,2.95,1.6431676725155)) ;
#102671=CARTESIAN_POINT('Origin',(-0.900000000000001,2.95,1.6431676725155)) ;
#102672=CARTESIAN_POINT('Origin',(1.15,2.21886116991581,-0.65)) ;
#102673=CARTESIAN_POINT('Ctrl Pts',(1.15,1.02736587339765,-0.750000000000001)) ;
#102674=CARTESIAN_POINT('Ctrl Pts',(1.1608920328805,1.02736587339765,-0.750000000000001)) ;
#102675=CARTESIAN_POINT('Ctrl Pts',(1.17195716626105,1.02622125393927,-0.748143843925991)) ;
#102676=CARTESIAN_POINT('Ctrl Pts',(1.1820844490224,1.02414637334385,-0.74471318879084)) ;
#102677=CARTESIAN_POINT('Ctrl Pts',(1.19245005921088,1.02202266415684,-0.741201799343137)) ;
#102678=CARTESIAN_POINT('Ctrl Pts',(1.20216743701154,1.01888103823701,-0.735960198070275)) ;
#102679=CARTESIAN_POINT('Ctrl Pts',(1.21053792402812,1.01518120925307,-0.72959371680205)) ;
#102680=CARTESIAN_POINT('Ctrl Pts',(1.219343173684,1.01128921135341,-0.722896560843853)) ;
#102681=CARTESIAN_POINT('Ctrl Pts',(1.22692289939014,1.00668521903338,-0.714785161531543)) ;
#102682=CARTESIAN_POINT('Ctrl Pts',(1.23290049538659,1.00186003905466,-0.70592412596239)) ;
#102683=CARTESIAN_POINT('Ctrl Pts',(1.23922345568944,0.9967560772818,-0.696551131169983)) ;
#102684=CARTESIAN_POINT('Ctrl Pts',(1.24392209779927,0.991279542094837,
-0.68610455998969)) ;
#102685=CARTESIAN_POINT('Ctrl Pts',(1.24674870216524,0.985895902333124,
-0.675292066529666)) ;
#102686=CARTESIAN_POINT('Ctrl Pts',(1.24889292215336,0.981811953364218,
-0.667089869972722)) ;
#102687=CARTESIAN_POINT('Ctrl Pts',(1.25,0.977715885027402,-0.658549168629227)) ;
#102688=CARTESIAN_POINT('Ctrl Pts',(1.25,0.973783447787483,-0.650000000000001)) ;
#102689=CARTESIAN_POINT('Origin',(-0.900000000000001,3.8,0.)) ;
#102690=CARTESIAN_POINT('Origin',(-0.900000000000002,1.02736587339765,0.849999999999999)) ;
#102691=CARTESIAN_POINT('Origin',(-0.900000000000001,3.8,0.850000000000002)) ;
#102692=CARTESIAN_POINT('Origin',(-0.900000000000002,2.1568323274845,0.85)) ;
#102693=CARTESIAN_POINT('Origin',(-0.900000000000002,1.02736587339765,0.849999999999999)) ;
#102694=CARTESIAN_POINT('Origin',(-0.900000000000001,3.8,0.)) ;
#102695=CARTESIAN_POINT('Origin',(-0.900000000000002,2.1568323274845,0.85)) ;
#102696=CARTESIAN_POINT('Origin',(-1.,2.95,1.6431676725155)) ;
#102697=CARTESIAN_POINT('Origin',(1.15,2.95,1.6431676725155)) ;
#102698=CARTESIAN_POINT('Origin',(1.15,3.15,2.55)) ;
#102699=CARTESIAN_POINT('Origin',(1.15,3.15,1.6431676725155)) ;
#102700=CARTESIAN_POINT('Ctrl Pts',(1.110285585749,0.930383836951471,-0.87499428365811)) ;
#102701=CARTESIAN_POINT('Ctrl Pts',(1.14039000477526,0.892136466138004,
-0.749969718594225)) ;
#102702=CARTESIAN_POINT('Ctrl Pts',(1.13015013463565,1.02610337426265,-0.747851124882802)) ;
#102703=CARTESIAN_POINT('Ctrl Pts',(1.17639690652713,0.935225109827677,
-0.890125739946714)) ;
#102704=CARTESIAN_POINT('Ctrl Pts',(1.15491086542926,0.891146666106694,
-0.749276050401193)) ;
#102705=CARTESIAN_POINT('Ctrl Pts',(1.16319405445818,1.03078047702079,-0.755164874245163)) ;
#102706=CARTESIAN_POINT('Ctrl Pts',(1.24701363206613,0.927145283841823,
-0.865552203825101)) ;
#102707=CARTESIAN_POINT('Ctrl Pts',(1.17759980831448,0.893467326853883,
-0.752637312031294)) ;
#102708=CARTESIAN_POINT('Ctrl Pts',(1.19848758201045,1.02297467453102,-0.74328712255501)) ;
#102709=CARTESIAN_POINT('Ctrl Pts',(1.33816236560061,0.900022463714227,
-0.769808850614887)) ;
#102710=CARTESIAN_POINT('Ctrl Pts',(1.22862786282604,0.888037626603987,
-0.723153964324038)) ;
#102711=CARTESIAN_POINT('Ctrl Pts',(1.24403288504499,0.996768276947731,
-0.697026659413336)) ;
#102712=CARTESIAN_POINT('Ctrl Pts',(1.35959492575604,0.881455895025373,
-0.698532341229029)) ;
#102713=CARTESIAN_POINT('Ctrl Pts',(1.25320519750685,0.880428099081617,
-0.691064937827297)) ;
#102714=CARTESIAN_POINT('Ctrl Pts',(1.25473603279824,0.978811277328854,
-0.662557487150855)) ;
#102715=CARTESIAN_POINT('Ctrl Pts',(1.34615355831623,0.867571605181204,
-0.632792582533412)) ;
#102716=CARTESIAN_POINT('Ctrl Pts',(1.25176090202797,0.870950130624675,
-0.649449017057823)) ;
#102717=CARTESIAN_POINT('Ctrl Pts',(1.24801589497572,0.965423101361815,
-0.630869548163999)) ;
#102718=CARTESIAN_POINT('Origin',(1.35,0.973783447787483,-0.650000000000001)) ;
#102719=CARTESIAN_POINT('Origin',(-0.900000000000002,1.02736587339765,0.849999999999999)) ;
#102720=CARTESIAN_POINT('',(-0.957735026918965,0.969630846478688,0.792264973081036)) ;
#102721=CARTESIAN_POINT('Origin',(-0.900000000000002,1.02736587339765,0.849999999999999)) ;
#102722=CARTESIAN_POINT('Origin',(-0.900000000000002,2.1568323274845,0.85)) ;
#102723=CARTESIAN_POINT('Origin',(-0.900000000000002,2.1568323274845,0.85)) ;
#102724=CARTESIAN_POINT('Origin',(1.15,2.95,1.6431676725155)) ;
#102725=CARTESIAN_POINT('Origin',(1.15,3.04189189189189,1.46552792413544)) ;
#102726=CARTESIAN_POINT('Origin',(1.35,3.8,0.)) ;
#102727=CARTESIAN_POINT('Origin',(1.35,0.973783447787484,0.649999999999999)) ;
#102728=CARTESIAN_POINT('Origin',(-1.,2.1568323274845,0.850000000000001)) ;
#102729=CARTESIAN_POINT('Origin',(1.15,2.1568323274845,0.850000000000001)) ;
#102730=CARTESIAN_POINT('Origin',(1.15,3.8,0.)) ;
#102731=CARTESIAN_POINT('Origin',(1.15,2.33447207586456,0.758108108108108)) ;
#102732=CARTESIAN_POINT('Ctrl Pts',(1.34754079198594,0.869159571293157,
0.640251465214486)) ;
#102733=CARTESIAN_POINT('Ctrl Pts',(1.25183398383323,0.871999770424339,
0.654001348239709)) ;
#102734=CARTESIAN_POINT('Ctrl Pts',(1.24871534599026,0.966951450593888,
0.634464286926457)) ;
#102735=CARTESIAN_POINT('Ctrl Pts',(1.3578897130187,0.882932151572343,0.704222571731899)) ;
#102736=CARTESIAN_POINT('Ctrl Pts',(1.25138796519089,0.881019151005411,
0.693512718576227)) ;
#102737=CARTESIAN_POINT('Ctrl Pts',(1.25389076424432,0.980237216252359,
0.665311365740565)) ;
#102738=CARTESIAN_POINT('Ctrl Pts',(1.33642796493171,0.900551643074787,
0.771683281031192)) ;
#102739=CARTESIAN_POINT('Ctrl Pts',(1.22773025960898,0.888154519889407,
0.723697645847668)) ;
#102740=CARTESIAN_POINT('Ctrl Pts',(1.24317203399027,0.997278352451065,
0.697935541716943)) ;
#102741=CARTESIAN_POINT('Ctrl Pts',(1.24851212064761,0.926675670999746,
0.863888145813442)) ;
#102742=CARTESIAN_POINT('Ctrl Pts',(1.17855408504648,0.893378082604329,
0.752064154599799)) ;
#102743=CARTESIAN_POINT('Ctrl Pts',(1.19923947710883,1.02252144543593,0.742488815939334)) ;
#102744=CARTESIAN_POINT('Ctrl Pts',(1.18212686068544,0.934567888698255,
0.888107740099251)) ;
#102745=CARTESIAN_POINT('Ctrl Pts',(1.15690947476176,0.891342319659343,
0.749498697761042)) ;
#102746=CARTESIAN_POINT('Ctrl Pts',(1.16605892368789,1.03014681530423,0.754195876479622)) ;
#102747=CARTESIAN_POINT('Ctrl Pts',(1.11776263740947,0.930888708579169,
0.876576418083976)) ;
#102748=CARTESIAN_POINT('Ctrl Pts',(1.14197710563589,0.892059806626672,
0.749917700344492)) ;
#102749=CARTESIAN_POINT('Ctrl Pts',(1.13388624958144,1.02659206201249,0.748622143898735)) ;
#102750=CARTESIAN_POINT('Ctrl Pts',(1.15,1.02736587339764,0.749999999999999)) ;
#102751=CARTESIAN_POINT('Ctrl Pts',(1.15623005440502,1.02736587339759,0.750000000000132)) ;
#102752=CARTESIAN_POINT('Ctrl Pts',(1.16249579431471,1.02700282517053,0.749409133931021)) ;
#102753=CARTESIAN_POINT('Ctrl Pts',(1.16857840195431,1.02630083270769,0.748259060553334)) ;
#102754=CARTESIAN_POINT('Ctrl Pts',(1.1798885498395,1.02499553092934,0.746120586275334)) ;
#102755=CARTESIAN_POINT('Ctrl Pts',(1.19084787809767,1.02245621903271,0.741949303384784)) ;
#102756=CARTESIAN_POINT('Ctrl Pts',(1.20043335385463,1.01914369852331,0.736350893562102)) ;
#102757=CARTESIAN_POINT('Ctrl Pts',(1.21063893018497,1.01561688548223,0.730390313177509)) ;
#102758=CARTESIAN_POINT('Ctrl Pts',(1.21965078109605,1.01112191387731,0.722645148898142)) ;
#102759=CARTESIAN_POINT('Ctrl Pts',(1.226898722009,1.00626683908294,0.713926415145715)) ;
#102760=CARTESIAN_POINT('Ctrl Pts',(1.23435386869391,1.0012729663137,0.704958428263417)) ;
#102761=CARTESIAN_POINT('Ctrl Pts',(1.24017476602864,0.995763540409855,
0.694712973593074)) ;
#102762=CARTESIAN_POINT('Ctrl Pts',(1.24405759382605,0.990267693778535,
0.683958342769537)) ;
#102763=CARTESIAN_POINT('Ctrl Pts',(1.24795610732226,0.9847496452368,0.673160265800921)) ;
#102764=CARTESIAN_POINT('Ctrl Pts',(1.25,0.97910634898267,0.661572054972022)) ;
#102765=CARTESIAN_POINT('Ctrl Pts',(1.25,0.973783447787483,0.649999999999999)) ;
#102766=CARTESIAN_POINT('Origin',(1.15,2.1568323274845,0.850000000000001)) ;
#102767=CARTESIAN_POINT('Origin',(1.15,2.1568323274845,0.65)) ;
#102768=CARTESIAN_POINT('Origin',(1.15,2.21886116991581,0.65)) ;
#102769=CARTESIAN_POINT('Origin',(1.5,2.3,-0.4)) ;
#102770=CARTESIAN_POINT('Ctrl Pts',(0.55,4.04473197180486,-0.449999999999999)) ;
#102771=CARTESIAN_POINT('Ctrl Pts',(0.55,4.04340510574361,-0.452018391674586)) ;
#102772=CARTESIAN_POINT('Ctrl Pts',(0.549938912488053,4.04197482121868,
-0.453979909355823)) ;
#102773=CARTESIAN_POINT('Ctrl Pts',(0.549362579613731,4.03414945156067,
-0.463763201696885)) ;
#102774=CARTESIAN_POINT('Ctrl Pts',(0.548040652125116,4.02633974827564,
-0.470545826227087)) ;
#102775=CARTESIAN_POINT('Ctrl Pts',(0.544205267183646,4.00519499286859,
-0.484683942788798)) ;
#102776=CARTESIAN_POINT('Ctrl Pts',(0.541221332378524,3.99011995637992,
-0.49122511544812)) ;
#102777=CARTESIAN_POINT('Ctrl Pts',(0.537814556431593,3.96385893187685,
-0.497930592239943)) ;
#102778=CARTESIAN_POINT('Ctrl Pts',(0.536602540378443,3.95132390702873,
-0.5)) ;
#102779=CARTESIAN_POINT('Ctrl Pts',(0.536602540378443,3.93764017256378,
-0.5)) ;
#102780=CARTESIAN_POINT('Origin',(-0.4,2.3,-0.4)) ;
#102781=CARTESIAN_POINT('Origin',(-0.4,-3.4,-0.4)) ;
#102782=CARTESIAN_POINT('Origin',(-0.4,-3.36847777691809,-0.4)) ;
#102783=CARTESIAN_POINT('Origin',(1.5,2.3,-0.4)) ;
#102784=CARTESIAN_POINT('Ctrl Pts',(0.536602540378444,2.83090991212703,
-0.5)) ;
#102785=CARTESIAN_POINT('Ctrl Pts',(0.536602540378444,2.80627146475495,
-0.5)) ;
#102786=CARTESIAN_POINT('Ctrl Pts',(0.538106903229181,2.77742679387655,
-0.497952790812571)) ;
#102787=CARTESIAN_POINT('Ctrl Pts',(0.545186976568881,2.71156844363323,
-0.48208398098003)) ;
#102788=CARTESIAN_POINT('Ctrl Pts',(0.55,2.68282906082667,-0.468102055813631)) ;
#102789=CARTESIAN_POINT('Ctrl Pts',(0.55,2.65280931275608,-0.449999999999997)) ;
#102790=CARTESIAN_POINT('Origin',(0.400000000000001,2.29999999999999,-0.4)) ;
#102791=CARTESIAN_POINT('Origin',(0.0725078566451197,-4.04348900069683,
0.0725078566451195)) ;
#102792=CARTESIAN_POINT('Origin',(-0.4,-3.36847777691809,-0.4)) ;
#102793=CARTESIAN_POINT('Origin',(-0.0979344438426628,-3.8,-0.0979344438426628)) ;
#102794=CARTESIAN_POINT('Origin',(1.5,2.3,0.4)) ;
#102795=CARTESIAN_POINT('Ctrl Pts',(0.536602540378444,3.93764017256378,
0.5)) ;
#102796=CARTESIAN_POINT('Ctrl Pts',(0.536602540378444,3.93925361219656,
0.5)) ;
#102797=CARTESIAN_POINT('Ctrl Pts',(0.536619300889434,3.94087098263999,
0.499971002742215)) ;
#102798=CARTESIAN_POINT('Ctrl Pts',(0.536997639747709,3.95938954612074,
0.499314187104252)) ;
#102799=CARTESIAN_POINT('Ctrl Pts',(0.539142315171056,3.97567120869891,
0.495687938438414)) ;
#102800=CARTESIAN_POINT('Ctrl Pts',(0.544035197036655,4.00535605098085,
0.484600608334013)) ;
#102801=CARTESIAN_POINT('Ctrl Pts',(0.546989816174414,4.01946236900604,
0.476430055365021)) ;
#102802=CARTESIAN_POINT('Ctrl Pts',(0.549463062495691,4.03595536007401,
0.461452618302868)) ;
#102803=CARTESIAN_POINT('Ctrl Pts',(0.550000000000879,4.04078397701435,
0.456005579653646)) ;
#102804=CARTESIAN_POINT('Ctrl Pts',(0.549999999999999,4.04473197181449,
0.449999999985356)) ;
#102805=CARTESIAN_POINT('Origin',(-0.4,2.3,0.4)) ;
#102806=CARTESIAN_POINT('Origin',(0.4,2.29999999999999,-0.4)) ;
#102807=CARTESIAN_POINT('Origin',(0.4,-3.36847777691809,-0.4)) ;
#102808=CARTESIAN_POINT('Origin',(-0.0979344438426628,-3.8,-0.0979344438426627)) ;
#102809=CARTESIAN_POINT('Origin',(-0.0979344438426628,-3.8,-0.0979344438426626)) ;
#102810=CARTESIAN_POINT('Origin',(-0.0979344438426627,-3.8,-0.0979344438426627)) ;
#102811=CARTESIAN_POINT('Origin',(-0.4,2.3,0.4)) ;
#102812=CARTESIAN_POINT('Origin',(-0.4,-3.36847777691809,0.4)) ;
#102813=CARTESIAN_POINT('Origin',(0.190875981738719,-3.6672263744342,-0.190875981738719)) ;
#102814=CARTESIAN_POINT('Origin',(0.400000000000001,-3.36847777691809,-0.4)) ;
#102815=CARTESIAN_POINT('Origin',(0.0979344438426626,-3.8,-0.0979344438426627)) ;
#102816=CARTESIAN_POINT('Origin',(0.15,-3.8,-0.0979344438426626)) ;
#102817=CARTESIAN_POINT('Origin',(0.0979344438426627,-3.8,-0.0979344438426626)) ;
#102818=CARTESIAN_POINT('Origin',(-0.0979344438426628,-3.8,0.5)) ;
#102819=CARTESIAN_POINT('Origin',(-0.0979344438426628,-3.8,0.0979344438426625)) ;
#102820=CARTESIAN_POINT('Origin',(-0.174966890829628,-3.68995364716148,
0.174966890829628)) ;
#102821=CARTESIAN_POINT('Origin',(-0.400000000000001,-3.36847777691809,
0.4)) ;
#102822=CARTESIAN_POINT('Origin',(-0.0979344438426627,-3.8,0.0979344438426627)) ;
#102823=CARTESIAN_POINT('Origin',(0.0979344438426627,-3.8,-0.0979344438426628)) ;
#102824=CARTESIAN_POINT('Origin',(0.0979344438426628,-3.8,-0.0979344438426625)) ;
#102825=CARTESIAN_POINT('Origin',(-0.0979344438426628,-3.8,0.0979344438426627)) ;
#102826=CARTESIAN_POINT('Origin',(-0.0979344438426628,-3.8,0.0979344438426627)) ;
#102827=CARTESIAN_POINT('Origin',(0.0979344438426627,-3.8,0.5)) ;
#102828=CARTESIAN_POINT('Origin',(0.0979344438426627,-3.8,0.0979344438426627)) ;
#102829=CARTESIAN_POINT('Origin',(-1.11032778078669,-3.8,0.0979344438426627)) ;
#102830=CARTESIAN_POINT('Origin',(0.0979344438426626,-3.8,0.0979344438426627)) ;
#102831=CARTESIAN_POINT('Origin',(0.0979344438426627,-3.8,0.0979344438426627)) ;
#102832=CARTESIAN_POINT('Origin',(0.0979344438426627,-3.8,0.0979344438426626)) ;
#102833=CARTESIAN_POINT('Origin',(0.438350729213467,-3.31369102089885,0.438350729213466)) ;
#102834=CARTESIAN_POINT('Origin',(0.399999999999999,-3.36847777691809,0.399999999999999)) ;
#102835=CARTESIAN_POINT('Origin',(0.4,2.3,0.4)) ;
#102836=CARTESIAN_POINT('Origin',(0.4,-3.36847777691809,0.4)) ;
#102837=CARTESIAN_POINT('Origin',(0.4,2.29999999999999,0.4)) ;
#102838=CARTESIAN_POINT('Origin',(1.5,2.3,0.4)) ;
#102839=CARTESIAN_POINT('Ctrl Pts',(0.55,2.65280931275594,0.449999999999912)) ;
#102840=CARTESIAN_POINT('Ctrl Pts',(0.550000000000012,2.67648433237899,
0.464276153337302)) ;
#102841=CARTESIAN_POINT('Ctrl Pts',(0.546908864252786,2.69988533923264,
0.476474299152385)) ;
#102842=CARTESIAN_POINT('Ctrl Pts',(0.539540151921445,2.76165254733708,
0.495908401809885)) ;
#102843=CARTESIAN_POINT('Ctrl Pts',(0.536602540378444,2.79600904778113,
0.5)) ;
#102844=CARTESIAN_POINT('Ctrl Pts',(0.536602540378444,2.83090991212703,
0.5)) ;
#102845=CARTESIAN_POINT('Origin',(8.,3.4,-0.4)) ;
#102846=CARTESIAN_POINT('Origin',(7.96847777691809,3.4,-0.4)) ;
#102847=CARTESIAN_POINT('Origin',(1.5,4.2,-0.4)) ;
#102848=CARTESIAN_POINT('Origin',(7.96847777691809,4.2,-0.4)) ;
#102849=CARTESIAN_POINT('Origin',(8.64348900069683,3.87250785664512,0.0725078566451195)) ;
#102850=CARTESIAN_POINT('Origin',(7.96847777691809,3.4,-0.4)) ;
#102851=CARTESIAN_POINT('Origin',(8.4,3.70206555615734,-0.0979344438426621)) ;
#102852=CARTESIAN_POINT('Origin',(8.26722637443421,3.99087598173872,-0.190875981738719)) ;
#102853=CARTESIAN_POINT('Origin',(7.96847777691809,4.2,-0.4)) ;
#102854=CARTESIAN_POINT('Origin',(8.4,3.89793444384266,-0.0979344438426626)) ;
#102855=CARTESIAN_POINT('Origin',(8.4,3.95,-0.0979344438426626)) ;
#102856=CARTESIAN_POINT('Origin',(8.4,3.70206555615734,-0.0979344438426625)) ;
#102857=CARTESIAN_POINT('Origin',(8.4,3.89793444384266,-0.0979344438426626)) ;
#102858=CARTESIAN_POINT('Origin',(8.4,3.70206555615734,-0.0979344438426625)) ;
#102859=CARTESIAN_POINT('Origin',(8.4,3.70206555615734,-0.0979344438426626)) ;
#102860=CARTESIAN_POINT('Origin',(1.5,3.4,0.4)) ;
#102861=CARTESIAN_POINT('Origin',(7.96847777691809,3.4,0.4)) ;
#102862=CARTESIAN_POINT('Origin',(1.5,4.2,0.4)) ;
#102863=CARTESIAN_POINT('Origin',(7.96847777691809,4.2,0.4)) ;
#102864=CARTESIAN_POINT('Origin',(8.4,3.89793444384266,-0.0979344438426626)) ;
#102865=CARTESIAN_POINT('Origin',(8.4,3.89793444384266,-0.0979344438426625)) ;
#102866=CARTESIAN_POINT('Origin',(8.4,3.70206555615734,0.5)) ;
#102867=CARTESIAN_POINT('Origin',(8.4,3.70206555615734,0.0979344438426624)) ;
#102868=CARTESIAN_POINT('Origin',(8.28995364716148,3.62503310917037,0.174966890829628)) ;
#102869=CARTESIAN_POINT('Origin',(7.96847777691809,3.4,0.4)) ;
#102870=CARTESIAN_POINT('Origin',(8.4,3.70206555615734,0.0979344438426625)) ;
#102871=CARTESIAN_POINT('Origin',(7.91369102089885,4.23835072921347,0.438350729213466)) ;
#102872=CARTESIAN_POINT('Origin',(7.96847777691809,4.2,0.4)) ;
#102873=CARTESIAN_POINT('Origin',(8.4,3.89793444384266,0.0979344438426624)) ;
#102874=CARTESIAN_POINT('Origin',(8.4,3.89793444384266,0.5)) ;
#102875=CARTESIAN_POINT('Origin',(8.4,3.89793444384266,0.0979344438426625)) ;
#102876=CARTESIAN_POINT('Origin',(8.4,3.70206555615734,0.0979344438426625)) ;
#102877=CARTESIAN_POINT('Origin',(8.4,3.70206555615734,0.0979344438426625)) ;
#102878=CARTESIAN_POINT('Origin',(8.4,3.89793444384266,0.0979344438426626)) ;
#102879=CARTESIAN_POINT('Origin',(8.4,3.89793444384266,0.0979344438426626)) ;
#102880=CARTESIAN_POINT('Origin',(8.4,2.68967221921331,0.0979344438426624)) ;
#102881=CARTESIAN_POINT('Origin',(9.9,6.8847127088383,-2.54)) ;
#102882=CARTESIAN_POINT('Origin',(9.9,6.8847127088383,-0.959712708838304)) ;
#102883=CARTESIAN_POINT('Origin',(8.77035388141948,6.69643835574155,-0.771438355741551)) ;
#102884=CARTESIAN_POINT('Ctrl Pts',(8.58356010126947,6.66256607592813,-0.638926683544912)) ;
#102885=CARTESIAN_POINT('Ctrl Pts',(8.58266714977878,6.65676189123867,-0.638777858296464)) ;
#102886=CARTESIAN_POINT('Ctrl Pts',(8.58182526931896,6.6507714222091,-0.639114171474057)) ;
#102887=CARTESIAN_POINT('Ctrl Pts',(8.58032528754334,6.63886560514808,-0.640912735099675)) ;
#102888=CARTESIAN_POINT('Ctrl Pts',(8.57966270906106,6.63295370212158,-0.64234482433286)) ;
#102889=CARTESIAN_POINT('Ctrl Pts',(8.57906641006218,6.62681909302492,-0.644477174493837)) ;
#102890=CARTESIAN_POINT('Ctrl Pts',(8.57903375157327,6.62647998752492,-0.644597169728486)) ;
#102891=CARTESIAN_POINT('Ctrl Pts',(8.5784656962419,6.62052582174859,-0.646741731680975)) ;
#102892=CARTESIAN_POINT('Ctrl Pts',(8.57802501793962,6.61503168015214,-0.649314285855883)) ;
#102893=CARTESIAN_POINT('Ctrl Pts',(8.57766199200566,6.60925146760271,-0.652746213323561)) ;
#102894=CARTESIAN_POINT('Ctrl Pts',(8.57762821177171,6.60869602779083,-0.653083835164735)) ;
#102895=CARTESIAN_POINT('Ctrl Pts',(8.57728522755448,6.60286036001494,-0.656714798956953)) ;
#102896=CARTESIAN_POINT('Ctrl Pts',(8.57709550103274,6.59788070192403,-0.660548221055747)) ;
#102897=CARTESIAN_POINT('Ctrl Pts',(8.57703980289278,6.59299711069459,-0.665172337354183)) ;
#102898=CARTESIAN_POINT('Ctrl Pts',(8.5770367027102,6.59265952430071,-0.665496892541691)) ;
#102899=CARTESIAN_POINT('Ctrl Pts',(8.57701334129167,6.58927432516126,-0.668801381595255)) ;
#102900=CARTESIAN_POINT('Ctrl Pts',(8.57705699426433,6.58642971201548,-0.671991744408714)) ;
#102901=CARTESIAN_POINT('Ctrl Pts',(8.57735031225518,6.57961409340219,-0.680795441755407)) ;
#102902=CARTESIAN_POINT('Ctrl Pts',(8.57770856513435,6.57604383182912,-0.686668245539852)) ;
#102903=CARTESIAN_POINT('Ctrl Pts',(8.57865704971091,6.57055741297625,-0.698332219338929)) ;
#102904=CARTESIAN_POINT('Ctrl Pts',(8.57922107378972,6.5685147605043,-0.704073634908064)) ;
#102905=CARTESIAN_POINT('Ctrl Pts',(8.57993695782547,6.56687610193741,-0.710455934816734)) ;
#102906=CARTESIAN_POINT('Ctrl Pts',(8.58000419042985,6.5667300168205,-0.711047835184081)) ;
#102907=CARTESIAN_POINT('Ctrl Pts',(8.58074399738022,6.56520526212512,-0.717481251735679)) ;
#102908=CARTESIAN_POINT('Ctrl Pts',(8.58149993293357,6.56438134785765,-0.723354180094219)) ;
#102909=CARTESIAN_POINT('Ctrl Pts',(8.58236768178488,6.56403389662198,-0.729498757823986)) ;
#102910=CARTESIAN_POINT('Ctrl Pts',(8.58242358604554,6.56401394107884,-0.729892173631949)) ;
#102911=CARTESIAN_POINT('Ctrl Pts',(8.58283067264383,6.56388592662946,-0.732739423426399)) ;
#102912=CARTESIAN_POINT('Ctrl Pts',(8.5831915624065,6.56386525642004,-0.735169950582818)) ;
#102913=CARTESIAN_POINT('Ctrl Pts',(8.58356019967708,6.56392669994633,-0.737566265064708)) ;
#102914=CARTESIAN_POINT('Origin',(9.9,6.8847127088383,-0.959712708838304)) ;
#102915=CARTESIAN_POINT('Origin',(9.9,6.8847127088383,-0.959712708838304)) ;
#102916=CARTESIAN_POINT('Origin',(9.9,6.8847127088383,-0.959712708838304)) ;
#102917=CARTESIAN_POINT('Origin',(9.9,7.72792407799439,-2.54)) ;
#102918=CARTESIAN_POINT('Origin',(9.9,7.72792407799439,-0.959712708838304)) ;
#102919=CARTESIAN_POINT('Origin',(9.90000000000001,4.35421736843756,-0.959712708838305)) ;
#102920=CARTESIAN_POINT('Origin',(9.9,7.72792407799439,-0.959712708838304)) ;
#102921=CARTESIAN_POINT('Origin',(9.9,7.72792407799439,-0.959712708838304)) ;
#102922=CARTESIAN_POINT('Origin',(9.9,7.72792407799439,-0.959712708838304)) ;
#102923=CARTESIAN_POINT('Origin',(10.9628342502842,7.37364599456632,-1.13685175055234)) ;
#102924=CARTESIAN_POINT('Ctrl Pts',(8.56837732530586,8.27720755823131,-0.73250525379773)) ;
#102925=CARTESIAN_POINT('Ctrl Pts',(8.56753565030796,8.2774881236726,-0.726612992197404)) ;
#102926=CARTESIAN_POINT('Ctrl Pts',(8.56682045541688,8.27721180667909,-0.720541294439539)) ;
#102927=CARTESIAN_POINT('Ctrl Pts',(8.56575413148033,8.27538624160241,-0.708728472119804)) ;
#102928=CARTESIAN_POINT('Ctrl Pts',(8.56538426077877,8.27391165896585,-0.702990562432011)) ;
#102929=CARTESIAN_POINT('Ctrl Pts',(8.56517777855942,8.27166501362671,-0.697014775451337)) ;
#102930=CARTESIAN_POINT('Ctrl Pts',(8.56516523451685,8.27151619608678,-0.696627638285824)) ;
#102931=CARTESIAN_POINT('Ctrl Pts',(8.56497390811211,8.26902793125447,-0.69029533599113)) ;
#102932=CARTESIAN_POINT('Ctrl Pts',(8.56499903025531,8.26597630129447,-0.684535778465806)) ;
#102933=CARTESIAN_POINT('Ctrl Pts',(8.56538588200255,8.26046191593053,-0.676590672368122)) ;
#102934=CARTESIAN_POINT('Ctrl Pts',(8.56556309332504,8.25853771611454,-0.674121236455737)) ;
#102935=CARTESIAN_POINT('Ctrl Pts',(8.56628156514546,8.25214511987157,-0.666801756689111)) ;
#102936=CARTESIAN_POINT('Ctrl Pts',(8.5670074287479,8.24720216256266,-0.662305445230979)) ;
#102937=CARTESIAN_POINT('Ctrl Pts',(8.56880713798121,8.23661566152184,-0.654624494880154)) ;
#102938=CARTESIAN_POINT('Ctrl Pts',(8.5698603939131,8.23102391527008,-0.651384880725776)) ;
#102939=CARTESIAN_POINT('Ctrl Pts',(8.57116255171742,8.2245955219417,-0.648446774527188)) ;
#102940=CARTESIAN_POINT('Ctrl Pts',(8.57127495810211,8.22404408343807,-0.648200660790281)) ;
#102941=CARTESIAN_POINT('Ctrl Pts',(8.57260511146323,8.21755901312516,-0.645374915305223)) ;
#102942=CARTESIAN_POINT('Ctrl Pts',(8.57395629672867,8.21135759730777,-0.643346386427245)) ;
#102943=CARTESIAN_POINT('Ctrl Pts',(8.57552311082447,8.20452945286151,-0.641749544317012)) ;
#102944=CARTESIAN_POINT('Ctrl Pts',(8.57564505123027,8.2040002630702,-0.641629826955897)) ;
#102945=CARTESIAN_POINT('Ctrl Pts',(8.57731301559524,8.19679193622633,-0.640053462537017)) ;
#102946=CARTESIAN_POINT('Ctrl Pts',(8.57896065127871,8.19002168485358,-0.639210969344035)) ;
#102947=CARTESIAN_POINT('Ctrl Pts',(8.58161366784366,8.17959769015476,-0.638755317277183)) ;
#102948=CARTESIAN_POINT('Ctrl Pts',(8.5825836286427,8.17587911616512,-0.63876393810712)) ;
#102949=CARTESIAN_POINT('Ctrl Pts',(8.58356010126947,8.17221734381475,-0.638926683544914)) ;
#102950=CARTESIAN_POINT('Origin',(7.96824861826159,6.56275414521524,0.637754145215235)) ;
#102951=CARTESIAN_POINT('Origin',(8.59688370202641,6.66156024040334,0.728756524736636)) ;
#102952=CARTESIAN_POINT('Origin',(9.9,6.8847127088383,0.959712708838304)) ;
#102953=CARTESIAN_POINT('Origin',(9.9,6.8847127088383,-2.54)) ;
#102954=CARTESIAN_POINT('Origin',(9.9,6.8847127088383,0.959712708838305)) ;
#102955=CARTESIAN_POINT('Origin',(9.9,6.8847127088383,0.959712708838304)) ;
#102956=CARTESIAN_POINT('Origin',(9.9,6.8847127088383,0.959712708838304)) ;
#102957=CARTESIAN_POINT('Origin',(9.9,6.8,0.959712708838305)) ;
#102958=CARTESIAN_POINT('Origin',(9.9,7.72792407799439,0.959712708838304)) ;
#102959=CARTESIAN_POINT('Origin',(9.9,7.72792407799439,-2.54)) ;
#102960=CARTESIAN_POINT('Origin',(9.9,7.72792407799439,0.959712708838304)) ;
#102961=CARTESIAN_POINT('Origin',(9.9,7.72792407799439,0.959712708838304)) ;
#102962=CARTESIAN_POINT('Origin',(9.9,7.72792407799439,0.959712708838304)) ;
#102963=CARTESIAN_POINT('Origin',(9.60917571369883,7.82486550676144,0.911241994454776)) ;
#102964=CARTESIAN_POINT('Origin',(8.59099001845934,8.18966234087067,0.734839026100492)) ;
#102965=CARTESIAN_POINT('Origin',(0.45,4.4,-2.94081128943275E-32)) ;
#102966=CARTESIAN_POINT('Origin',(0.45,4.4,-0.45)) ;
#102967=CARTESIAN_POINT('Origin',(0.45,4.4,0.45)) ;
#102968=CARTESIAN_POINT('Origin',(-1.9,7.55,-2.54)) ;
#102969=CARTESIAN_POINT('Origin',(6.9,7.75,-2.54)) ;
#102970=CARTESIAN_POINT('Origin',(7.1,8.2,-2.54)) ;
#102971=CARTESIAN_POINT('Origin',(9.9,0.1,-2.54)) ;
#102972=CARTESIAN_POINT('Origin',(9.9,1.16528729116168,-2.54)) ;
#102973=CARTESIAN_POINT('Origin',(9.9,1.16528729116168,-2.04416188017819)) ;
#102974=CARTESIAN_POINT('Origin',(9.9,3.8,0.)) ;
#102975=CARTESIAN_POINT('Origin',(9.9,1.16528729116168,2.0441618801782)) ;
#102976=CARTESIAN_POINT('Origin',(9.9,1.16528729116168,-2.04416188017819)) ;
#102977=CARTESIAN_POINT('Origin',(9.9,1.16528729116168,-2.54)) ;
#102978=CARTESIAN_POINT('Origin',(9.9,1.16528729116168,2.0441618801782)) ;
#102979=CARTESIAN_POINT('Ctrl Pts',(0.55,0.3,-0.450000000000001)) ;
#102980=CARTESIAN_POINT('Ctrl Pts',(0.55,0.3,-0.55)) ;
#102981=CARTESIAN_POINT('Ctrl Pts',(0.45,0.3,-0.550000000000001)) ;
#102982=CARTESIAN_POINT('Ctrl Pts',(0.55,0.28690770353672,-0.45000000081826)) ;
#102983=CARTESIAN_POINT('Ctrl Pts',(0.549992696057548,0.30054349846765,
-0.549992696055191)) ;
#102984=CARTESIAN_POINT('Ctrl Pts',(0.450000000818259,0.286907703536719,
-0.550000000000001)) ;
#102985=CARTESIAN_POINT('Ctrl Pts',(0.552602750539093,0.273825167611082,
-0.455205501078186)) ;
#102986=CARTESIAN_POINT('Ctrl Pts',(0.546703256435901,0.299059401315788,
-0.5467032564359)) ;
#102987=CARTESIAN_POINT('Ctrl Pts',(0.455205501078185,0.273825167611082,
-0.552602750539093)) ;
#102988=CARTESIAN_POINT('Ctrl Pts',(0.56262134295865,0.249638145915901,
-0.4752426859173)) ;
#102989=CARTESIAN_POINT('Ctrl Pts',(0.544986924117067,0.282072776439537,
-0.544986924117069)) ;
#102990=CARTESIAN_POINT('Ctrl Pts',(0.4752426859173,0.2496381459159,-0.56262134295865)) ;
#102991=CARTESIAN_POINT('Ctrl Pts',(0.570033341471288,0.238545302291403,
-0.490066682942577)) ;
#102992=CARTESIAN_POINT('Ctrl Pts',(0.547116196858396,0.267914459835244,
-0.547116196858398)) ;
#102993=CARTESIAN_POINT('Ctrl Pts',(0.490066682942577,0.238545302291402,
-0.570033341471289)) ;
#102994=CARTESIAN_POINT('Ctrl Pts',(0.597801282701459,0.210777361061231,
-0.545602565402918)) ;
#102995=CARTESIAN_POINT('Ctrl Pts',(0.570853448890183,0.226374713859281,
-0.57085344889018)) ;
#102996=CARTESIAN_POINT('Ctrl Pts',(0.545602565402917,0.210777361061233,
-0.597801282701458)) ;
#102997=CARTESIAN_POINT('Ctrl Pts',(0.623746567173635,0.2,-0.597493134347285)) ;
#102998=CARTESIAN_POINT('Ctrl Pts',(0.610458667314981,0.2,-0.610458667314981)) ;
#102999=CARTESIAN_POINT('Ctrl Pts',(0.597493134347281,0.2,-0.623746567173645)) ;
#103000=CARTESIAN_POINT('Ctrl Pts',(0.65,0.2,-0.650000000000001)) ;
#103001=CARTESIAN_POINT('Ctrl Pts',(0.65,0.2,-0.650000000000001)) ;
#103002=CARTESIAN_POINT('Ctrl Pts',(0.65,0.2,-0.650000000000001)) ;
#103003=CARTESIAN_POINT('Origin',(0.45,0.3,-0.45)) ;
#103004=CARTESIAN_POINT('Origin',(0.45,1.24941393210234E-16,-0.450000000000001)) ;
#103005=CARTESIAN_POINT('Origin',(0.45,4.4,-0.45)) ;
#103006=CARTESIAN_POINT('Origin',(0.45,4.4,-0.45)) ;
#103007=CARTESIAN_POINT('Origin',(0.45,4.4,-0.45)) ;
#103008=CARTESIAN_POINT('Origin',(0.549999999999999,4.4,-0.45)) ;
#103009=CARTESIAN_POINT('Origin',(-1.7,4.4,-0.45)) ;
#103010=CARTESIAN_POINT('Ctrl Pts',(-1.8,4.6,-0.65)) ;
#103011=CARTESIAN_POINT('Ctrl Pts',(-1.8,4.6,-0.65)) ;
#103012=CARTESIAN_POINT('Ctrl Pts',(-1.8,4.6,-0.65)) ;
#103013=CARTESIAN_POINT('Ctrl Pts',(-1.8,4.57374656717367,-0.597493134347272)) ;
#103014=CARTESIAN_POINT('Ctrl Pts',(-1.8,4.56045866731613,-0.610458667316091)) ;
#103015=CARTESIAN_POINT('Ctrl Pts',(-1.8,4.54749313434727,-0.62374656717366)) ;
#103016=CARTESIAN_POINT('Ctrl Pts',(-1.78922263893876,4.54780128270145,
-0.545602565402917)) ;
#103017=CARTESIAN_POINT('Ctrl Pts',(-1.77362528614073,4.52085344889015,
-0.570853448890188)) ;
#103018=CARTESIAN_POINT('Ctrl Pts',(-1.78922263893877,4.49560256540291,
-0.597801282701462)) ;
#103019=CARTESIAN_POINT('Ctrl Pts',(-1.7614546977086,4.5200333414713,-0.490066682942577)) ;
#103020=CARTESIAN_POINT('Ctrl Pts',(-1.73208554016475,4.49711619685842,
-0.547116196858392)) ;
#103021=CARTESIAN_POINT('Ctrl Pts',(-1.7614546977086,4.44006668294258,-0.570033341471286)) ;
#103022=CARTESIAN_POINT('Ctrl Pts',(-1.7503618540841,4.51262134295865,-0.475242685917298)) ;
#103023=CARTESIAN_POINT('Ctrl Pts',(-1.71792722356046,4.49498692411707,
-0.544986924117066)) ;
#103024=CARTESIAN_POINT('Ctrl Pts',(-1.7503618540841,4.42524268591729,-0.562621342958649)) ;
#103025=CARTESIAN_POINT('Ctrl Pts',(-1.72617483238892,4.50260275053909,
-0.455205501078186)) ;
#103026=CARTESIAN_POINT('Ctrl Pts',(-1.70094059868421,4.4967032564359,-0.546703256435901)) ;
#103027=CARTESIAN_POINT('Ctrl Pts',(-1.72617483238892,4.4052055010782,-0.552602750539093)) ;
#103028=CARTESIAN_POINT('Ctrl Pts',(-1.71309229646328,4.5,-0.450000000818259)) ;
#103029=CARTESIAN_POINT('Ctrl Pts',(-1.69945650153965,4.49999269603991,
-0.549992696055229)) ;
#103030=CARTESIAN_POINT('Ctrl Pts',(-1.71309229646328,4.40000000081823,
-0.55)) ;
#103031=CARTESIAN_POINT('Ctrl Pts',(-1.7,4.5,-0.45)) ;
#103032=CARTESIAN_POINT('Ctrl Pts',(-1.7,4.5,-0.55)) ;
#103033=CARTESIAN_POINT('Ctrl Pts',(-1.7,4.4,-0.55)) ;
#103034=CARTESIAN_POINT('Ctrl Pts',(-1.8,4.6,0.65)) ;
#103035=CARTESIAN_POINT('Ctrl Pts',(-1.8,4.6,0.65)) ;
#103036=CARTESIAN_POINT('Ctrl Pts',(-1.8,4.6,0.65)) ;
#103037=CARTESIAN_POINT('Ctrl Pts',(-1.8,4.54749313434727,0.623746567173674)) ;
#103038=CARTESIAN_POINT('Ctrl Pts',(-1.8,4.56045866731613,0.61045866731609)) ;
#103039=CARTESIAN_POINT('Ctrl Pts',(-1.8,4.57374656717367,0.597493134347274)) ;
#103040=CARTESIAN_POINT('Ctrl Pts',(-1.78922263893877,4.49560256540291,
0.597801282701463)) ;
#103041=CARTESIAN_POINT('Ctrl Pts',(-1.77362528614073,4.52085344889015,
0.570853448890189)) ;
#103042=CARTESIAN_POINT('Ctrl Pts',(-1.78922263893876,4.54780128270145,
0.545602565402918)) ;
#103043=CARTESIAN_POINT('Ctrl Pts',(-1.7614546977086,4.44006668294258,0.570033341471287)) ;
#103044=CARTESIAN_POINT('Ctrl Pts',(-1.73208554016475,4.49711619685842,
0.547116196858393)) ;
#103045=CARTESIAN_POINT('Ctrl Pts',(-1.7614546977086,4.5200333414713,0.490066682942578)) ;
#103046=CARTESIAN_POINT('Ctrl Pts',(-1.7503618540841,4.42524268591729,0.56262134295865)) ;
#103047=CARTESIAN_POINT('Ctrl Pts',(-1.71792722356046,4.49498692411707,
0.544986924117068)) ;
#103048=CARTESIAN_POINT('Ctrl Pts',(-1.7503618540841,4.51262134295865,0.475242685917299)) ;
#103049=CARTESIAN_POINT('Ctrl Pts',(-1.72617483238892,4.4052055010782,0.552602750539093)) ;
#103050=CARTESIAN_POINT('Ctrl Pts',(-1.70094059868421,4.4967032564359,0.5467032564359)) ;
#103051=CARTESIAN_POINT('Ctrl Pts',(-1.72617483238892,4.50260275053909,
0.455205501078187)) ;
#103052=CARTESIAN_POINT('Ctrl Pts',(-1.71309229646328,4.40000000081823,
0.55)) ;
#103053=CARTESIAN_POINT('Ctrl Pts',(-1.69945650153893,4.4999926960399,0.549992696056988)) ;
#103054=CARTESIAN_POINT('Ctrl Pts',(-1.71309229646328,4.5,0.450000000818259)) ;
#103055=CARTESIAN_POINT('Ctrl Pts',(-1.7,4.4,0.55)) ;
#103056=CARTESIAN_POINT('Ctrl Pts',(-1.7,4.5,0.55)) ;
#103057=CARTESIAN_POINT('Ctrl Pts',(-1.7,4.5,0.45)) ;
#103058=CARTESIAN_POINT('Origin',(-1.7,4.4,0.45)) ;
#103059=CARTESIAN_POINT('Origin',(0.549999999999999,4.4,0.45)) ;
#103060=CARTESIAN_POINT('Origin',(0.45,4.4,0.45)) ;
#103061=CARTESIAN_POINT('Origin',(0.45,4.4,0.45)) ;
#103062=CARTESIAN_POINT('Origin',(0.45,4.4,0.45)) ;
#103063=CARTESIAN_POINT('Origin',(0.45,4.9047241136249E-17,0.450000000000001)) ;
#103064=CARTESIAN_POINT('Origin',(0.45,0.3,0.450000000000001)) ;
#103065=CARTESIAN_POINT('Ctrl Pts',(0.45,0.3,0.550000000000001)) ;
#103066=CARTESIAN_POINT('Ctrl Pts',(0.55,0.3,0.55)) ;
#103067=CARTESIAN_POINT('Ctrl Pts',(0.55,0.3,0.450000000000001)) ;
#103068=CARTESIAN_POINT('Ctrl Pts',(0.450000000818259,0.286907703536719,
0.550000000000001)) ;
#103069=CARTESIAN_POINT('Ctrl Pts',(0.54999269605693,0.300543498469827,
0.549992696061056)) ;
#103070=CARTESIAN_POINT('Ctrl Pts',(0.55,0.28690770353672,0.45000000081826)) ;
#103071=CARTESIAN_POINT('Ctrl Pts',(0.455205501078185,0.273825167611082,
0.552602750539094)) ;
#103072=CARTESIAN_POINT('Ctrl Pts',(0.546703256435901,0.299059401315788,
0.5467032564359)) ;
#103073=CARTESIAN_POINT('Ctrl Pts',(0.552602750539093,0.273825167611082,
0.455205501078186)) ;
#103074=CARTESIAN_POINT('Ctrl Pts',(0.4752426859173,0.2496381459159,0.56262134295865)) ;
#103075=CARTESIAN_POINT('Ctrl Pts',(0.544986924117067,0.282072776439536,
0.544986924117069)) ;
#103076=CARTESIAN_POINT('Ctrl Pts',(0.56262134295865,0.249638145915901,
0.475242685917301)) ;
#103077=CARTESIAN_POINT('Ctrl Pts',(0.490066682942577,0.238545302291402,
0.570033341471289)) ;
#103078=CARTESIAN_POINT('Ctrl Pts',(0.547116196858396,0.267914459835244,
0.547116196858399)) ;
#103079=CARTESIAN_POINT('Ctrl Pts',(0.570033341471288,0.238545302291403,
0.490066682942577)) ;
#103080=CARTESIAN_POINT('Ctrl Pts',(0.545602565402917,0.210777361061233,
0.597801282701458)) ;
#103081=CARTESIAN_POINT('Ctrl Pts',(0.570853448890183,0.226374713859281,
0.57085344889018)) ;
#103082=CARTESIAN_POINT('Ctrl Pts',(0.597801282701459,0.210777361061231,
0.545602565402918)) ;
#103083=CARTESIAN_POINT('Ctrl Pts',(0.597493134347281,0.2,0.623746567173645)) ;
#103084=CARTESIAN_POINT('Ctrl Pts',(0.610458667314981,0.2,0.610458667314981)) ;
#103085=CARTESIAN_POINT('Ctrl Pts',(0.623746567173635,0.2,0.597493134347285)) ;
#103086=CARTESIAN_POINT('Ctrl Pts',(0.65,0.2,0.650000000000001)) ;
#103087=CARTESIAN_POINT('Ctrl Pts',(0.65,0.2,0.650000000000001)) ;
#103088=CARTESIAN_POINT('Ctrl Pts',(0.65,0.2,0.650000000000001)) ;
#103089=CARTESIAN_POINT('Ctrl Pts',(8.5,8.17221734381475,-0.540287291161696)) ;
#103090=CARTESIAN_POINT('Ctrl Pts',(8.5,8.17221734381475,-0.625)) ;
#103091=CARTESIAN_POINT('Ctrl Pts',(8.58356010126947,8.17221734381475,-0.638926683544911)) ;
#103092=CARTESIAN_POINT('Ctrl Pts',(8.5,8.23335379241386,-0.540287292739054)) ;
#103093=CARTESIAN_POINT('Ctrl Pts',(8.5,8.20847425960651,-0.617457567421702)) ;
#103094=CARTESIAN_POINT('Ctrl Pts',(8.57460439031229,8.20580126077888,-0.637434065052048)) ;
#103095=CARTESIAN_POINT('Ctrl Pts',(8.5,8.29192178062155,-0.567174115078498)) ;
#103096=CARTESIAN_POINT('Ctrl Pts',(8.5,8.25010493984403,-0.629254608311669)) ;
#103097=CARTESIAN_POINT('Ctrl Pts',(8.56800970738923,8.23725302684488,-0.649778363189931)) ;
#103098=CARTESIAN_POINT('Ctrl Pts',(8.5,8.36583651094028,-0.656550623291365)) ;
#103099=CARTESIAN_POINT('Ctrl Pts',(8.5,8.29925403146167,-0.683361437036636)) ;
#103100=CARTESIAN_POINT('Ctrl Pts',(8.56373266208983,8.27563607377073,-0.693753776413148)) ;
#103101=CARTESIAN_POINT('Ctrl Pts',(8.5,8.38029241321764,-0.71795520569968)) ;
#103102=CARTESIAN_POINT('Ctrl Pts',(8.5,8.30669116589107,-0.724808849941012)) ;
#103103=CARTESIAN_POINT('Ctrl Pts',(8.56610123859386,8.28208399509953,-0.724808702406988)) ;
#103104=CARTESIAN_POINT('Ctrl Pts',(8.5,8.36719795478507,-0.776054723479883)) ;
#103105=CARTESIAN_POINT('Ctrl Pts',(8.5,8.29381262650623,-0.759515149671807)) ;
#103106=CARTESIAN_POINT('Ctrl Pts',(8.57227762885807,8.27346847343705,-0.754929987635437)) ;
#103107=CARTESIAN_POINT('Ctrl Pts',(8.54852133092351,8.28383177029354,-0.755986532733631)) ;
#103108=CARTESIAN_POINT('Ctrl Pts',(8.54913757890788,8.28625057716298,-0.742921659183987)) ;
#103109=CARTESIAN_POINT('Ctrl Pts',(8.54914636139901,8.28675781111762,-0.729264789402619)) ;
#103110=CARTESIAN_POINT('Ctrl Pts',(8.54883414737369,8.28489376483071,-0.716098869425042)) ;
#103111=CARTESIAN_POINT('Ctrl Pts',(8.54852072231757,8.28302248819127,-0.702881880842787)) ;
#103112=CARTESIAN_POINT('Ctrl Pts',(8.54791723678494,8.27865742078997,-0.689831295811734)) ;
#103113=CARTESIAN_POINT('Ctrl Pts',(8.54677696932927,8.27237937104781,-0.678102076729669)) ;
#103114=CARTESIAN_POINT('Ctrl Pts',(8.5454465495755,8.26505438658866,-0.664416879730159)) ;
#103115=CARTESIAN_POINT('Ctrl Pts',(8.54324462275112,8.25487237915563,-0.652253753338803)) ;
#103116=CARTESIAN_POINT('Ctrl Pts',(8.53884071267076,8.24480815719263,-0.64120716819918)) ;
#103117=CARTESIAN_POINT('Ctrl Pts',(8.5342440055524,8.23430333763594,-0.629676978976814)) ;
#103118=CARTESIAN_POINT('Ctrl Pts',(8.52670159721618,8.22420330618022,-0.618704260242989)) ;
#103119=CARTESIAN_POINT('Ctrl Pts',(8.51928858688475,8.21729138318396,-0.605988175465276)) ;
#103120=CARTESIAN_POINT('Ctrl Pts',(8.51327528614099,8.21168455548023,-0.595673116045033)) ;
#103121=CARTESIAN_POINT('Ctrl Pts',(8.50759525524367,8.20778929846109,-0.58398494308279)) ;
#103122=CARTESIAN_POINT('Ctrl Pts',(8.50412058850191,8.20498026622232,-0.571573948662816)) ;
#103123=CARTESIAN_POINT('Ctrl Pts',(8.50147164778345,8.20283877743224,-0.562112325169396)) ;
#103124=CARTESIAN_POINT('Ctrl Pts',(8.50000317248551,8.2012555848359,-0.552083357654996)) ;
#103125=CARTESIAN_POINT('Ctrl Pts',(8.50000000513446,8.20000405629318,-0.542105238728424)) ;
#103126=CARTESIAN_POINT('Origin',(8.6,8.17221734381475,-0.540287291161696)) ;
#103127=CARTESIAN_POINT('Origin',(8.6,4.35421736843756,-0.540287291161696)) ;
#103128=CARTESIAN_POINT('Origin',(8.6,6.66256607592813,-0.540287291161696)) ;
#103129=CARTESIAN_POINT('Ctrl Pts',(8.5,6.47083593368087,-0.784808109924428)) ;
#103130=CARTESIAN_POINT('Ctrl Pts',(8.5,6.55684090505321,-0.76438773869521)) ;
#103131=CARTESIAN_POINT('Ctrl Pts',(8.58772778625753,6.56739561896918,-0.761881707090954)) ;
#103132=CARTESIAN_POINT('Ctrl Pts',(8.5,6.45680686388583,-0.72572152971769)) ;
#103133=CARTESIAN_POINT('Ctrl Pts',(8.5000000000001,6.54406229478621,-0.732510165403657)) ;
#103134=CARTESIAN_POINT('Ctrl Pts',(8.58195196310366,6.55941415012444,-0.731357686877846)) ;
#103135=CARTESIAN_POINT('Ctrl Pts',(8.5,6.4706155658439,-0.661952456804846)) ;
#103136=CARTESIAN_POINT('Ctrl Pts',(8.5,6.54836369988887,-0.69239872740711)) ;
#103137=CARTESIAN_POINT('Ctrl Pts',(8.57801125828726,6.56566601372231,-0.698834459202782)) ;
#103138=CARTESIAN_POINT('Ctrl Pts',(8.5,6.54379299301796,-0.568626471658098)) ;
#103139=CARTESIAN_POINT('Ctrl Pts',(8.5,6.59071789516225,-0.636226515292209)) ;
#103140=CARTESIAN_POINT('Ctrl Pts',(8.57642058265787,6.60198961470444,-0.651906354024515)) ;
#103141=CARTESIAN_POINT('Ctrl Pts',(8.5,6.60220518075381,-0.540287292974651)) ;
#103142=CARTESIAN_POINT('Ctrl Pts',(8.5,6.62800697860325,-0.620917670762679)) ;
#103143=CARTESIAN_POINT('Ctrl Pts',(8.57879135173926,6.63156920211805,-0.638131891956542)) ;
#103144=CARTESIAN_POINT('Ctrl Pts',(8.5,6.66256607592813,-0.540287291161696)) ;
#103145=CARTESIAN_POINT('Ctrl Pts',(8.5,6.66256607592813,-0.625)) ;
#103146=CARTESIAN_POINT('Ctrl Pts',(8.58356010126947,6.66256607592813,-0.638926683544911)) ;
#103147=CARTESIAN_POINT('',(8.54565366748554,6.61650711946996,-0.633965318291701)) ;
#103148=CARTESIAN_POINT('Ctrl Pts',(8.54565366716104,6.61650712004131,-0.633965317813484)) ;
#103149=CARTESIAN_POINT('Ctrl Pts',(8.54527684775569,6.61717057264361,-0.63341000086369)) ;
#103150=CARTESIAN_POINT('Ctrl Pts',(8.54488909344004,6.61782772231432,-0.632855429899671)) ;
#103151=CARTESIAN_POINT('Ctrl Pts',(8.54449064961561,6.61847724592616,-0.632300871385118)) ;
#103152=CARTESIAN_POINT('Ctrl Pts',(8.54445329550707,6.61853813876477,-0.632248881524379)) ;
#103153=CARTESIAN_POINT('Ctrl Pts',(8.54441584757977,6.6185989645223,-0.632196891791653)) ;
#103154=CARTESIAN_POINT('Ctrl Pts',(8.544378306106,6.61865972207467,-0.632144901585903)) ;
#103155=CARTESIAN_POINT('Ctrl Pts',(8.54363538409149,6.6198620755966,-0.631116048306817)) ;
#103156=CARTESIAN_POINT('Ctrl Pts',(8.54285495000591,6.62104203503532,-0.630084862174671)) ;
#103157=CARTESIAN_POINT('Ctrl Pts',(8.54204093171152,6.62218056960126,-0.629051115167204)) ;
#103158=CARTESIAN_POINT('Ctrl Pts',(8.54157979215439,6.62282554690599,-0.628465499781785)) ;
#103159=CARTESIAN_POINT('Ctrl Pts',(8.54110770812188,6.62345780120147,-0.627878649906638)) ;
#103160=CARTESIAN_POINT('Ctrl Pts',(8.54062344907118,6.6240789244817,-0.627286954139643)) ;
#103161=CARTESIAN_POINT('Ctrl Pts',(8.54011932596483,6.62472552591744,-0.62667098731849)) ;
#103162=CARTESIAN_POINT('Ctrl Pts',(8.53960207832255,6.62535666566135,-0.626050990589038)) ;
#103163=CARTESIAN_POINT('Ctrl Pts',(8.53907286520405,6.62597244099098,-0.625425228811039)) ;
#103164=CARTESIAN_POINT('Ctrl Pts',(8.53887441028461,6.62620335673959,-0.62519056814429)) ;
#103165=CARTESIAN_POINT('Ctrl Pts',(8.5386742766414,6.62643211299941,-0.624955099821045)) ;
#103166=CARTESIAN_POINT('Ctrl Pts',(8.53847256319996,6.62665871795109,-0.624718764218343)) ;
#103167=CARTESIAN_POINT('Ctrl Pts',(8.53842843838465,6.62670828778427,-0.624667065805252)) ;
#103168=CARTESIAN_POINT('Ctrl Pts',(8.53838423811749,6.62675775467668,-0.624615326017445)) ;
#103169=CARTESIAN_POINT('Ctrl Pts',(8.53833996369344,6.62680711871688,-0.62456354446014)) ;
#103170=CARTESIAN_POINT('Ctrl Pts',(8.53829707284515,6.62685494013082,-0.624513381076501)) ;
#103171=CARTESIAN_POINT('Ctrl Pts',(8.53825411240223,6.6269026650202,-0.624463178493077)) ;
#103172=CARTESIAN_POINT('Ctrl Pts',(8.53821108363804,6.62695029346534,-0.624412936437729)) ;
#103173=CARTESIAN_POINT('Ctrl Pts',(8.5380357143533,6.62714440934377,-0.624208168453412)) ;
#103174=CARTESIAN_POINT('Ctrl Pts',(8.53785876035509,6.62733753498025,-0.62400218366478)) ;
#103175=CARTESIAN_POINT('Ctrl Pts',(8.53767995296707,6.62753033615253,-0.623794466565225)) ;
#103176=CARTESIAN_POINT('Ctrl Pts',(8.53649871780658,6.62880401687795,-0.622422248425076)) ;
#103177=CARTESIAN_POINT('Ctrl Pts',(8.53528300832267,6.62998038079526,-0.621038076059647)) ;
#103178=CARTESIAN_POINT('Ctrl Pts',(8.53403203676339,6.63110281535144,-0.619604486564905)) ;
#103179=CARTESIAN_POINT('Ctrl Pts',(8.53346870389682,6.63160826591215,-0.618958917867875)) ;
#103180=CARTESIAN_POINT('Ctrl Pts',(8.53289959536919,6.63209979040223,-0.618305425659429)) ;
#103181=CARTESIAN_POINT('Ctrl Pts',(8.5323266134032,6.63257735344031,-0.617643701443846)) ;
#103182=CARTESIAN_POINT('Ctrl Pts',(8.53206474273905,6.63279561467256,-0.617341272798442)) ;
#103183=CARTESIAN_POINT('Ctrl Pts',(8.53180206199566,6.63301096017663,-0.617037126080686)) ;
#103184=CARTESIAN_POINT('Ctrl Pts',(8.53153874718657,6.63322338883724,-0.616731238880717)) ;
#103185=CARTESIAN_POINT('Ctrl Pts',(8.53007363658216,6.63440536369245,-0.615029251127047)) ;
#103186=CARTESIAN_POINT('Ctrl Pts',(8.52858926277508,6.63549697414125,-0.613273083913089)) ;
#103187=CARTESIAN_POINT('Ctrl Pts',(8.52711342564664,6.63649856635112,-0.61146113930632)) ;
#103188=CARTESIAN_POINT('Ctrl Pts',(8.52634316954117,6.63702130866459,-0.610515464902798)) ;
#103189=CARTESIAN_POINT('Ctrl Pts',(8.5255761534997,6.63751985710295,-0.609555719311186)) ;
#103190=CARTESIAN_POINT('Ctrl Pts',(8.52481401823432,6.63799287689813,-0.608580326161291)) ;
#103191=CARTESIAN_POINT('Ctrl Pts',(8.52460710835823,6.63812129566007,-0.608315519525312)) ;
#103192=CARTESIAN_POINT('Ctrl Pts',(8.52440075574005,6.63824801482192,-0.608049753902253)) ;
#103193=CARTESIAN_POINT('Ctrl Pts',(8.52419502810871,6.63837284070831,-0.607783086081022)) ;
#103194=CARTESIAN_POINT('Ctrl Pts',(8.52404824365685,6.63846190263543,-0.607592821459237)) ;
#103195=CARTESIAN_POINT('Ctrl Pts',(8.52390173612804,6.63855002749203,-0.607402043734724)) ;
#103196=CARTESIAN_POINT('Ctrl Pts',(8.52375553261476,6.63863721305423,-0.607210762804845)) ;
#103197=CARTESIAN_POINT('Ctrl Pts',(8.52294204127162,6.6391223224644,-0.606146456092442)) ;
#103198=CARTESIAN_POINT('Ctrl Pts',(8.52213801365707,6.6395783474869,-0.60506653755636)) ;
#103199=CARTESIAN_POINT('Ctrl Pts',(8.52134774490512,6.6400049409798,-0.603972961446361)) ;
#103200=CARTESIAN_POINT('Ctrl Pts',(8.51876608595597,6.64139854145543,-0.600400454569433)) ;
#103201=CARTESIAN_POINT('Ctrl Pts',(8.51630176076721,6.64256282842068,-0.596624566784401)) ;
#103202=CARTESIAN_POINT('Ctrl Pts',(8.51404737801024,6.64354662431173,-0.592668758228679)) ;
#103203=CARTESIAN_POINT('Ctrl Pts',(8.5117427137702,6.64455236266853,-0.58862471979261)) ;
#103204=CARTESIAN_POINT('Ctrl Pts',(8.50965863261303,6.64536892721963,-0.584393778069628)) ;
#103205=CARTESIAN_POINT('Ctrl Pts',(8.50786496313904,6.64606338785378,-0.580044165485977)) ;
#103206=CARTESIAN_POINT('Ctrl Pts',(8.50767015284865,6.64613881316472,-0.579571754429886)) ;
#103207=CARTESIAN_POINT('Ctrl Pts',(8.50747873128294,6.64621281334902,-0.579097973687544)) ;
#103208=CARTESIAN_POINT('Ctrl Pts',(8.50729076020858,6.64628549377757,-0.578622930193838)) ;
#103209=CARTESIAN_POINT('Ctrl Pts',(8.50722027105569,6.64631274893828,-0.578444788883699)) ;
#103210=CARTESIAN_POINT('Ctrl Pts',(8.50715026706479,6.64633981850992,-0.578266470019251)) ;
#103211=CARTESIAN_POINT('Ctrl Pts',(8.50708075128543,6.64636670806329,-0.578087979359469)) ;
#103212=CARTESIAN_POINT('Ctrl Pts',(8.50659414082988,6.6465549349369,-0.576838544740993)) ;
#103213=CARTESIAN_POINT('Ctrl Pts',(8.50613147592892,6.64673434010345,-0.575580683754983)) ;
#103214=CARTESIAN_POINT('Ctrl Pts',(8.50569363751095,6.64690683932497,-0.574316427502283)) ;
#103215=CARTESIAN_POINT('Ctrl Pts',(8.50395436040214,6.64759207829661,-0.569294273507268)) ;
#103216=CARTESIAN_POINT('Ctrl Pts',(8.50258205288311,6.64816393978924,-0.564091559615236)) ;
#103217=CARTESIAN_POINT('Ctrl Pts',(8.50162662717148,6.648647209875,-0.55880412474374)) ;
#103218=CARTESIAN_POINT('Ctrl Pts',(8.50156399248221,6.64867889153406,-0.558457497228713)) ;
#103219=CARTESIAN_POINT('Ctrl Pts',(8.50150313499581,6.64871019935922,-0.558110507516074)) ;
#103220=CARTESIAN_POINT('Ctrl Pts',(8.50144406283925,6.64874114271687,-0.557763183502011)) ;
#103221=CARTESIAN_POINT('Ctrl Pts',(8.50057491246573,6.64919642372275,-0.552652877493898)) ;
#103222=CARTESIAN_POINT('Ctrl Pts',(8.50009537300581,6.64957062705847,-0.54747132905142)) ;
#103223=CARTESIAN_POINT('Ctrl Pts',(8.50001293997571,6.64989933182544,-0.542314443541065)) ;
#103224=CARTESIAN_POINT('Ctrl Pts',(8.5000043087827,6.64993374902791,-0.541774489179143)) ;
#103225=CARTESIAN_POINT('Ctrl Pts',(8.5,6.64996765698295,-0.541234814428359)) ;
#103226=CARTESIAN_POINT('Ctrl Pts',(8.5,6.65000108682384,-0.540695536105911)) ;
#103227=CARTESIAN_POINT('',(8.55245136877623,6.600979943726,-0.646780119379722)) ;
#103228=CARTESIAN_POINT('Ctrl Pts',(8.55238056475496,6.60105295171764,-0.64688861549872)) ;
#103229=CARTESIAN_POINT('Ctrl Pts',(8.551705231719,6.6030854236859,-0.645102265614611)) ;
#103230=CARTESIAN_POINT('Ctrl Pts',(8.55095829520337,6.60513808680195,-0.64336273482155)) ;
#103231=CARTESIAN_POINT('Ctrl Pts',(8.55012599030481,6.60719152980482,-0.641654444180554)) ;
#103232=CARTESIAN_POINT('Ctrl Pts',(8.54968322947851,6.60828389886605,-0.640745685650989)) ;
#103233=CARTESIAN_POINT('Ctrl Pts',(8.54921644930856,6.60937569995297,-0.639846249123207)) ;
#103234=CARTESIAN_POINT('Ctrl Pts',(8.54872481267401,6.61045954913285,-0.638955746549559)) ;
#103235=CARTESIAN_POINT('Ctrl Pts',(8.54779539897823,6.61250851009536,-0.637272297372044)) ;
#103236=CARTESIAN_POINT('Ctrl Pts',(8.54677348694556,6.61453549290059,-0.635615590886287)) ;
#103237=CARTESIAN_POINT('Ctrl Pts',(8.54565366748553,6.61650711946996,-0.6339653182917)) ;
#103238=CARTESIAN_POINT('',(8.55735473176754,6.58264207262424,-0.664955797361829)) ;
#103239=CARTESIAN_POINT('Ctrl Pts',(8.55735473168708,6.5826420730276,-0.664955796844377)) ;
#103240=CARTESIAN_POINT('Ctrl Pts',(8.55706916598062,6.58397660851238,-0.663229693371652)) ;
#103241=CARTESIAN_POINT('Ctrl Pts',(8.55678088122713,6.58528501693225,-0.661662100960593)) ;
#103242=CARTESIAN_POINT('Ctrl Pts',(8.55647408091831,6.58661569125855,-0.660171823251799)) ;
#103243=CARTESIAN_POINT('Ctrl Pts',(8.55614409617588,6.58804692262372,-0.658568927518812)) ;
#103244=CARTESIAN_POINT('Ctrl Pts',(8.55579261555197,6.58950524590079,-0.657056795017548)) ;
#103245=CARTESIAN_POINT('Ctrl Pts',(8.55539993844513,6.59102291080503,-0.655587567779556)) ;
#103246=CARTESIAN_POINT('Ctrl Pts',(8.55517214917315,6.59190329771229,-0.654735279227253)) ;
#103247=CARTESIAN_POINT('Ctrl Pts',(8.5549304988197,6.59280308289125,-0.653898397754101)) ;
#103248=CARTESIAN_POINT('Ctrl Pts',(8.55467134659055,6.5937211373212,-0.653070794642137)) ;
#103249=CARTESIAN_POINT('Ctrl Pts',(8.55434805237174,6.59486641664498,-0.65203835397031)) ;
#103250=CARTESIAN_POINT('Ctrl Pts',(8.55400737519031,6.59602723165027,-0.65103619819577)) ;
#103251=CARTESIAN_POINT('Ctrl Pts',(8.55365328858765,6.59718920061515,-0.650045215513273)) ;
#103252=CARTESIAN_POINT('Ctrl Pts',(8.55328167888691,6.598408673298,-0.649005190911051)) ;
#103253=CARTESIAN_POINT('Ctrl Pts',(8.55289390107695,6.5996354646002,-0.647973679676364)) ;
#103254=CARTESIAN_POINT('Ctrl Pts',(8.55249886556666,6.60083562835443,-0.646908149434967)) ;
#103255=CARTESIAN_POINT('Ctrl Pts',(8.55248304763322,6.60088368507309,-0.64686548368468)) ;
#103256=CARTESIAN_POINT('Ctrl Pts',(8.55246721522814,6.60093179017207,-0.646822806733157)) ;
#103257=CARTESIAN_POINT('Ctrl Pts',(8.55245136877623,6.600979943726,-0.646780119379722)) ;
#103258=CARTESIAN_POINT('Ctrl Pts',(8.56107669735261,6.56009388000089,-0.762383847222383)) ;
#103259=CARTESIAN_POINT('Ctrl Pts',(8.56115635543004,6.5597817052481,-0.760820734383275)) ;
#103260=CARTESIAN_POINT('Ctrl Pts',(8.56122592915387,6.55950119162287,-0.759250712980609)) ;
#103261=CARTESIAN_POINT('Ctrl Pts',(8.56128584055879,6.55925348717443,-0.757693391948652)) ;
#103262=CARTESIAN_POINT('Ctrl Pts',(8.56142626445293,6.55867290283846,-0.754043250811132)) ;
#103263=CARTESIAN_POINT('Ctrl Pts',(8.56152217534692,6.55825854507372,-0.750375633877455)) ;
#103264=CARTESIAN_POINT('Ctrl Pts',(8.56158081746989,6.55798577878939,-0.746670135426049)) ;
#103265=CARTESIAN_POINT('Ctrl Pts',(8.5615891784535,6.55794688875065,-0.746141818743938)) ;
#103266=CARTESIAN_POINT('Ctrl Pts',(8.56159677639835,6.55791088241233,-0.7456126452602)) ;
#103267=CARTESIAN_POINT('Ctrl Pts',(8.56160362608006,6.55787769947535,-0.745082467472401)) ;
#103268=CARTESIAN_POINT('Ctrl Pts',(8.56164117305277,6.55769580506316,-0.742176263686379)) ;
#103269=CARTESIAN_POINT('Ctrl Pts',(8.56164095204357,6.55766773657215,-0.739264011996683)) ;
#103270=CARTESIAN_POINT('Ctrl Pts',(8.56161306230089,6.55774920537473,-0.736365567258155)) ;
#103271=CARTESIAN_POINT('Ctrl Pts',(8.56157759693122,6.55785280336172,-0.732679824607675)) ;
#103272=CARTESIAN_POINT('Ctrl Pts',(8.56150275624661,6.55813669070953,-0.729004928020692)) ;
#103273=CARTESIAN_POINT('Ctrl Pts',(8.56141108129146,6.55856506509341,-0.725363292547789)) ;
#103274=CARTESIAN_POINT('Ctrl Pts',(8.56136615997221,6.55877497130415,-0.723578867680741)) ;
#103275=CARTESIAN_POINT('Ctrl Pts',(8.56131707129299,6.55902016312283,-0.721801670968291)) ;
#103276=CARTESIAN_POINT('Ctrl Pts',(8.56126585691694,6.55929956116443,-0.720031525468218)) ;
#103277=CARTESIAN_POINT('Ctrl Pts',(8.56116752027495,6.55983603289963,-0.716632671909467)) ;
#103278=CARTESIAN_POINT('Ctrl Pts',(8.56104954130218,6.56049109659199,-0.713254007575518)) ;
#103279=CARTESIAN_POINT('Ctrl Pts',(8.56091150449777,6.56129147625798,-0.709830471024781)) ;
#103280=CARTESIAN_POINT('Ctrl Pts',(8.56080235670744,6.56192434857303,-0.707123428861444)) ;
#103281=CARTESIAN_POINT('Ctrl Pts',(8.56068045333715,6.56264902401856,-0.704387266689058)) ;
#103282=CARTESIAN_POINT('Ctrl Pts',(8.56054379825318,6.56349285586908,-0.701623487720724)) ;
#103283=CARTESIAN_POINT('Ctrl Pts',(8.56050762866484,6.56371619955873,-0.70089197635173)) ;
#103284=CARTESIAN_POINT('Ctrl Pts',(8.56047042218819,6.56394794674723,-0.700158791698164)) ;
#103285=CARTESIAN_POINT('Ctrl Pts',(8.56043213901762,6.56418871538691,-0.699424623470902)) ;
#103286=CARTESIAN_POINT('Ctrl Pts',(8.56026887460242,6.56521550994361,-0.696293651179561)) ;
#103287=CARTESIAN_POINT('Ctrl Pts',(8.56008532870549,6.56636514336248,-0.693261214935318)) ;
#103288=CARTESIAN_POINT('Ctrl Pts',(8.55988915918716,6.56762686151788,-0.690471327667742)) ;
#103289=CARTESIAN_POINT('Ctrl Pts',(8.55964574654531,6.56919243680243,-0.687009557276224)) ;
#103290=CARTESIAN_POINT('Ctrl Pts',(8.55938661160135,6.57080906160851,-0.683732634051197)) ;
#103291=CARTESIAN_POINT('Ctrl Pts',(8.55911582090258,6.57246439798287,-0.680667212427968)) ;
#103292=CARTESIAN_POINT('Ctrl Pts',(8.55888928658552,6.5738491962672,-0.678102784635318)) ;
#103293=CARTESIAN_POINT('Ctrl Pts',(8.55863813502891,6.57544444689331,-0.675365345431122)) ;
#103294=CARTESIAN_POINT('Ctrl Pts',(8.55834707044209,6.57718152485399,-0.672668125822793)) ;
#103295=CARTESIAN_POINT('Ctrl Pts',(8.55828762047113,6.5775363232011,-0.672117218448187)) ;
#103296=CARTESIAN_POINT('Ctrl Pts',(8.55822651695173,6.57789694345781,-0.671567846579033)) ;
#103297=CARTESIAN_POINT('Ctrl Pts',(8.5581636495887,6.57826264684151,-0.671021571079284)) ;
#103298=CARTESIAN_POINT('Ctrl Pts',(8.55792499569725,6.57965091145826,-0.668947827764096)) ;
#103299=CARTESIAN_POINT('Ctrl Pts',(8.55766032614236,6.58110993502766,-0.66692131328784)) ;
#103300=CARTESIAN_POINT('Ctrl Pts',(8.55735473176754,6.58264207262424,-0.664955797361829)) ;
#103301=CARTESIAN_POINT('Origin',(8.49172374697018,6.65,-2.54)) ;
#103302=CARTESIAN_POINT('Origin',(8.49226931273351,6.63793757405409,-0.772988271638203)) ;
#103303=CARTESIAN_POINT('Ctrl Pts',(8.40188506081764,6.5500005341705,-0.511545830815321)) ;
#103304=CARTESIAN_POINT('Ctrl Pts',(8.50280744587445,6.54966497091124,-0.525195040754151)) ;
#103305=CARTESIAN_POINT('Ctrl Pts',(8.50109204799973,6.65199687180768,-0.525680454939853)) ;
#103306=CARTESIAN_POINT('Ctrl Pts',(8.39296932930791,6.55000052027914,-0.569675802422008)) ;
#103307=CARTESIAN_POINT('Ctrl Pts',(8.49725036372774,6.54968051003369,-0.556913602683179)) ;
#103308=CARTESIAN_POINT('Ctrl Pts',(8.4966529651636,6.64935672317807,-0.556024711463538)) ;
#103309=CARTESIAN_POINT('Ctrl Pts',(8.41146079558551,6.55000052635931,-0.629608884645994)) ;
#103310=CARTESIAN_POINT('Ctrl Pts',(8.50278789772746,6.54967384197884,-0.581014351980562)) ;
#103311=CARTESIAN_POINT('Ctrl Pts',(8.5059095425555,6.65051247736751,-0.584427212093591)) ;
#103312=CARTESIAN_POINT('Ctrl Pts',(8.45744515914178,6.55000045243509,-0.682802191882288)) ;
#103313=CARTESIAN_POINT('Ctrl Pts',(8.52023811680815,6.54973725194856,-0.621633015820999)) ;
#103314=CARTESIAN_POINT('Ctrl Pts',(8.52891723073134,6.6364300977738,-0.613475163078278)) ;
#103315=CARTESIAN_POINT('Ctrl Pts',(8.46608867121686,6.55000043643008,-0.69119509917481)) ;
#103316=CARTESIAN_POINT('Ctrl Pts',(8.5233427016762,6.54974993059826,-0.628470240078956)) ;
#103317=CARTESIAN_POINT('Ctrl Pts',(8.53324349789235,6.63337968978885,-0.618220891300047)) ;
#103318=CARTESIAN_POINT('Ctrl Pts',(8.48465388181692,6.55000038323734,-0.70657631387452)) ;
#103319=CARTESIAN_POINT('Ctrl Pts',(8.53001210036432,6.54978938646811,-0.645124595123328)) ;
#103320=CARTESIAN_POINT('Ctrl Pts',(8.54253954944039,6.62323710347992,-0.62886314626903)) ;
#103321=CARTESIAN_POINT('Ctrl Pts',(8.4946704807492,6.55000035131511,-0.713488494461478)) ;
#103322=CARTESIAN_POINT('Ctrl Pts',(8.53347884787446,6.54981166882493,-0.653059031150021)) ;
#103323=CARTESIAN_POINT('Ctrl Pts',(8.54755337534736,6.61714793548866,-0.632867688126296)) ;
#103324=CARTESIAN_POINT('Ctrl Pts',(8.50997930894014,6.55000022766094,-0.723388902785886)) ;
#103325=CARTESIAN_POINT('Ctrl Pts',(8.53869035159219,6.54988741100164,-0.678774232755077)) ;
#103326=CARTESIAN_POINT('Ctrl Pts',(8.55523846583767,6.59353839814603,-0.653527883108543)) ;
#103327=CARTESIAN_POINT('Ctrl Pts',(8.51532901080113,6.55000016113069,-0.726338967319371)) ;
#103328=CARTESIAN_POINT('Ctrl Pts',(8.54023459682693,6.54992340374043,-0.688489748387105)) ;
#103329=CARTESIAN_POINT('Ctrl Pts',(8.55790835982317,6.58082417519527,-0.661582308572545)) ;
#103330=CARTESIAN_POINT('Ctrl Pts',(8.52186010906351,6.55000005932357,-0.732792759877374)) ;
#103331=CARTESIAN_POINT('Ctrl Pts',(8.54265823247975,6.5499732773141,-0.71793164411612)) ;
#103332=CARTESIAN_POINT('Ctrl Pts',(8.56121746518605,6.56135337205696,-0.70458837007694)) ;
#103333=CARTESIAN_POINT('Ctrl Pts',(8.5235499393997,6.55000003603139,-0.735824262228055)) ;
#103334=CARTESIAN_POINT('Ctrl Pts',(8.5435076996824,6.54998394755847,-0.731423873201171)) ;
#103335=CARTESIAN_POINT('Ctrl Pts',(8.56214310615443,6.55689632415127,-0.727450133563353)) ;
#103336=CARTESIAN_POINT('Ctrl Pts',(8.52268461318103,6.55000004733862,-0.741787530415828)) ;
#103337=CARTESIAN_POINT('Ctrl Pts',(8.54305517585919,6.54997881410036,-0.752813412140242)) ;
#103338=CARTESIAN_POINT('Ctrl Pts',(8.56153259171388,6.55906016573932,-0.762790181581043)) ;
#103339=CARTESIAN_POINT('Ctrl Pts',(8.52060566253918,6.55000006807331,-0.74441380654971)) ;
#103340=CARTESIAN_POINT('Ctrl Pts',(8.54195943530534,6.54996919659462,-0.760494574886098)) ;
#103341=CARTESIAN_POINT('Ctrl Pts',(8.56058441628597,6.56302742363398,-0.774507921514082)) ;
#103342=CARTESIAN_POINT('Ctrl Pts',(8.51445291480377,6.55000012130567,-0.751232814955295)) ;
#103343=CARTESIAN_POINT('Ctrl Pts',(8.53868948987834,6.54994355920608,-0.779419181767537)) ;
#103344=CARTESIAN_POINT('Ctrl Pts',(8.55750149922672,6.57320954252663,-0.801184435306907)) ;
#103345=CARTESIAN_POINT('Ctrl Pts',(8.50953280296009,6.55000015625148,-0.755047946437262)) ;
#103346=CARTESIAN_POINT('Ctrl Pts',(8.53616288920966,6.54992588038504,-0.787764748526664)) ;
#103347=CARTESIAN_POINT('Ctrl Pts',(8.55504783006515,6.57989127253972,-0.810699316792922)) ;
#103348=CARTESIAN_POINT('Ctrl Pts',(8.49261655785708,6.55000026291039,-0.768492606568883)) ;
#103349=CARTESIAN_POINT('Ctrl Pts',(8.52778251455087,6.54986718408744,-0.815769160894697)) ;
#103350=CARTESIAN_POINT('Ctrl Pts',(8.5465866761693,6.60027178071331,-0.839353375743825)) ;
#103351=CARTESIAN_POINT('Ctrl Pts',(8.4802216582452,6.55000031608562,-0.777768534160336)) ;
#103352=CARTESIAN_POINT('Ctrl Pts',(8.52288681814197,6.5498343726202,-0.827455948929167)) ;
#103353=CARTESIAN_POINT('Ctrl Pts',(8.54045339450475,6.61042388759294,-0.846301990960487)) ;
#103354=CARTESIAN_POINT('Ctrl Pts',(8.46952991654748,6.55000035836672,-0.789095446218494)) ;
#103355=CARTESIAN_POINT('Ctrl Pts',(8.51900842894086,6.54980714069604,-0.843367684676165)) ;
#103356=CARTESIAN_POINT('Ctrl Pts',(8.53471369258652,6.61849392543648,-0.861383368442905)) ;
#103357=CARTESIAN_POINT('Origin',(8.4,6.65,-0.540678001899701)) ;
#103358=CARTESIAN_POINT('Ctrl Pts',(8.54848814460235,8.28374914930622,0.75646282522011)) ;
#103359=CARTESIAN_POINT('Ctrl Pts',(8.55964225199693,8.27720012980426,0.755032051677707)) ;
#103360=CARTESIAN_POINT('Ctrl Pts',(8.572140519951,8.27365818248462,0.754258237443071)) ;
#103361=CARTESIAN_POINT('Ctrl Pts',(8.54519582228992,8.29111303851995,0.732039621192373)) ;
#103362=CARTESIAN_POINT('Ctrl Pts',(8.55569959891144,8.28406912459879,0.731962382559104)) ;
#103363=CARTESIAN_POINT('Ctrl Pts',(8.56757951573637,8.27991709749369,0.731808366088123)) ;
#103364=CARTESIAN_POINT('Ctrl Pts',(8.54340782920287,8.28927570119138,0.706177006876757)) ;
#103365=CARTESIAN_POINT('Ctrl Pts',(8.5535505383751,8.28232618564302,0.707845355710233)) ;
#103366=CARTESIAN_POINT('Ctrl Pts',(8.56507848568419,8.27803412520749,0.708867856946723)) ;
#103367=CARTESIAN_POINT('Ctrl Pts',(8.54340835145922,8.27841951799441,0.684464988838289)) ;
#103368=CARTESIAN_POINT('Ctrl Pts',(8.55355093564017,8.27219257320284,0.687578461234078)) ;
#103369=CARTESIAN_POINT('Ctrl Pts',(8.56507848521152,8.26835005667905,0.689499719495969)) ;
#103370=CARTESIAN_POINT('Ctrl Pts',(8.54742026180266,8.27608084857564,0.685634358751393)) ;
#103371=CARTESIAN_POINT('Ctrl Pts',(8.54754672558908,8.27683897030433,0.687325426963469)) ;
#103372=CARTESIAN_POINT('Ctrl Pts',(8.54766225486892,8.27755642830995,0.689034502691608)) ;
#103373=CARTESIAN_POINT('Ctrl Pts',(8.54776713596767,8.27823455672262,0.690764983222443)) ;
#103374=CARTESIAN_POINT('Ctrl Pts',(8.54791712013337,8.27920430747292,0.693239639588089)) ;
#103375=CARTESIAN_POINT('Ctrl Pts',(8.54806168001142,8.28008011045347,0.695753662732336)) ;
#103376=CARTESIAN_POINT('Ctrl Pts',(8.54818998754193,8.28086237513953,0.69828131614101)) ;
#103377=CARTESIAN_POINT('Ctrl Pts',(8.5482419492675,8.28117917511832,0.699304960133263)) ;
#103378=CARTESIAN_POINT('Ctrl Pts',(8.54829140719363,8.28148078264965,0.700331325709524)) ;
#103379=CARTESIAN_POINT('Ctrl Pts',(8.54833813644415,8.28176759858569,0.701360370022629)) ;
#103380=CARTESIAN_POINT('Ctrl Pts',(8.54850061324771,8.2827648526819,0.704938339470869)) ;
#103381=CARTESIAN_POINT('Ctrl Pts',(8.54863339756396,8.28360845633781,0.708649876470984)) ;
#103382=CARTESIAN_POINT('Ctrl Pts',(8.54873421749657,8.28426438239343,0.712386913242184)) ;
#103383=CARTESIAN_POINT('Ctrl Pts',(8.54878752953696,8.28461122607273,0.714363001205664)) ;
#103384=CARTESIAN_POINT('Ctrl Pts',(8.54883168679925,8.28490640714037,0.716345917925883)) ;
#103385=CARTESIAN_POINT('Ctrl Pts',(8.54886500248132,8.28515040605082,0.718318140970176)) ;
#103386=CARTESIAN_POINT('Ctrl Pts',(8.5488738542235,8.28521523484357,0.718842146748514)) ;
#103387=CARTESIAN_POINT('Ctrl Pts',(8.54888411330031,8.285275121517,0.719364990807687)) ;
#103388=CARTESIAN_POINT('Ctrl Pts',(8.54889386083024,8.28533143086091,0.719887913213841)) ;
#103389=CARTESIAN_POINT('Ctrl Pts',(8.54894969070932,8.28565394783544,0.722882999653076)) ;
#103390=CARTESIAN_POINT('Ctrl Pts',(8.5489793513821,8.2858668042412,0.725901363617001)) ;
#103391=CARTESIAN_POINT('Ctrl Pts',(8.54899968230029,8.28595875954338,0.728932422198607)) ;
#103392=CARTESIAN_POINT('Ctrl Pts',(8.54900356561228,8.2859763234883,0.729511370282527)) ;
#103393=CARTESIAN_POINT('Ctrl Pts',(8.54900713937599,8.28598945835117,0.730090691195829)) ;
#103394=CARTESIAN_POINT('Ctrl Pts',(8.5490105728891,8.28599806377621,0.730670159781498)) ;
#103395=CARTESIAN_POINT('Ctrl Pts',(8.54902784271198,8.28604134718936,0.733584760524092)) ;
#103396=CARTESIAN_POINT('Ctrl Pts',(8.54901619593281,8.28598556136224,0.736484224278308)) ;
#103397=CARTESIAN_POINT('Ctrl Pts',(8.54898431260111,8.28582669412324,0.739393571324556)) ;
#103398=CARTESIAN_POINT('Ctrl Pts',(8.54893914418925,8.28560163041441,0.743515179030308)) ;
#103399=CARTESIAN_POINT('Ctrl Pts',(8.54884805310403,8.28517290646446,0.747622900033123)) ;
#103400=CARTESIAN_POINT('Ctrl Pts',(8.54869940582914,8.28455561418427,0.751692922585911)) ;
#103401=CARTESIAN_POINT('Ctrl Pts',(8.54864697316337,8.28433787538056,0.753128550197273)) ;
#103402=CARTESIAN_POINT('Ctrl Pts',(8.54858736435355,8.28409676597419,0.754559160407532)) ;
#103403=CARTESIAN_POINT('Ctrl Pts',(8.54851996240545,8.28383343043592,0.755982796914733)) ;
#103404=CARTESIAN_POINT('Origin',(8.4,6.65,-2.54)) ;
#103405=CARTESIAN_POINT('Origin',(8.4,6.65,0.540678001899701)) ;
#103406=CARTESIAN_POINT('Origin',(8.49172374697018,6.65,-2.54)) ;
#103407=CARTESIAN_POINT('Origin',(8.49225485638824,6.63809817984101,0.772991371636644)) ;
#103408=CARTESIAN_POINT('Origin',(8.6,4.35421736843756,0.540287291161696)) ;
#103409=CARTESIAN_POINT('Origin',(8.6,6.66256607592813,0.540287291161696)) ;
#103410=CARTESIAN_POINT('Ctrl Pts',(8.5013487493624,6.65217253603379,0.524014743919239)) ;
#103411=CARTESIAN_POINT('Ctrl Pts',(8.50315244876578,6.54997127577019,0.523413630741524)) ;
#103412=CARTESIAN_POINT('Ctrl Pts',(8.40269444133659,6.55000000392138,0.508403503424183)) ;
#103413=CARTESIAN_POINT('Ctrl Pts',(8.49631753783951,6.64933701877088,0.554984347604346)) ;
#103414=CARTESIAN_POINT('Ctrl Pts',(8.49707874924866,6.54997270174419,0.55603877650159)) ;
#103415=CARTESIAN_POINT('Ctrl Pts',(8.39261127161987,6.55000000381175,0.567444979189231)) ;
#103416=CARTESIAN_POINT('Ctrl Pts',(8.50556246021204,6.65075235208953,0.583988954498525)) ;
#103417=CARTESIAN_POINT('Ctrl Pts',(8.502539579467,6.54997202229483,0.580355869545521)) ;
#103418=CARTESIAN_POINT('Ctrl Pts',(8.41103525938982,6.55000000386643,0.628661650365513)) ;
#103419=CARTESIAN_POINT('Ctrl Pts',(8.52891970071471,6.63645479210452,0.613472841517229)) ;
#103420=CARTESIAN_POINT('Ctrl Pts',(8.52027792490145,6.54997752826667,0.621595060038875)) ;
#103421=CARTESIAN_POINT('Ctrl Pts',(8.4576425585103,6.5500000033157,0.682609898416985)) ;
#103422=CARTESIAN_POINT('Ctrl Pts',(8.53324635448928,6.63340383613799,0.618217934261831)) ;
#103423=CARTESIAN_POINT('Ctrl Pts',(8.52338394863778,6.54997861189313,0.62842668610914)) ;
#103424=CARTESIAN_POINT('Ctrl Pts',(8.46627109069292,6.55000000319828,0.69099525146731)) ;
#103425=CARTESIAN_POINT('Ctrl Pts',(8.5425433201124,6.62325922024828,0.62885825178222)) ;
#103426=CARTESIAN_POINT('Ctrl Pts',(8.53005572430512,6.54998198465676,0.645067357531962)) ;
#103427=CARTESIAN_POINT('Ctrl Pts',(8.48480454940901,6.55000000280808,0.706372191176904)) ;
#103428=CARTESIAN_POINT('Ctrl Pts',(8.54755771953122,6.61716872587346,0.632861456122815)) ;
#103429=CARTESIAN_POINT('Ctrl Pts',(8.53352383957147,6.54998388968238,0.652993385085483)) ;
#103430=CARTESIAN_POINT('Ctrl Pts',(8.49480263348501,6.55000000257396,0.71328272370085)) ;
#103431=CARTESIAN_POINT('Ctrl Pts',(8.55524400651031,6.59355301617591,0.653519430104509)) ;
#103432=CARTESIAN_POINT('Ctrl Pts',(8.5387355250133,6.54999036710749,0.67870514119052)) ;
#103433=CARTESIAN_POINT('Ctrl Pts',(8.51008526949052,6.55000000166752,0.723224250581485)) ;
#103434=CARTESIAN_POINT('Ctrl Pts',(8.55791451833569,6.5808349442903,0.661572932536089)) ;
#103435=CARTESIAN_POINT('Ctrl Pts',(8.54027978136634,6.54999344602542,0.688420971165681)) ;
#103436=CARTESIAN_POINT('Ctrl Pts',(8.51542462880457,6.55000000118004,0.72619365566139)) ;
#103437=CARTESIAN_POINT('Ctrl Pts',(8.56122429319342,6.56135755929244,0.704583461036361)) ;
#103438=CARTESIAN_POINT('Ctrl Pts',(8.54270214007072,6.54999771321877,0.717900094355645)) ;
#103439=CARTESIAN_POINT('Ctrl Pts',(8.52194436340203,6.55000000043436,0.732732556326117)) ;
#103440=CARTESIAN_POINT('Ctrl Pts',(8.56215003896756,6.55689889598544,0.727448655243819)) ;
#103441=CARTESIAN_POINT('Ctrl Pts',(8.54355112280983,6.54999862629018,0.731414585978538)) ;
#103442=CARTESIAN_POINT('Ctrl Pts',(8.52363168464777,6.55000000026381,0.735806239205465)) ;
#103443=CARTESIAN_POINT('Ctrl Pts',(8.56153943432816,6.55906352913392,0.762793876209075)) ;
#103444=CARTESIAN_POINT('Ctrl Pts',(8.54309854033143,6.5499981870035,0.752836831731517)) ;
#103445=CARTESIAN_POINT('Ctrl Pts',(8.52276767133745,6.5500000003466,0.74183248681998)) ;
#103446=CARTESIAN_POINT('Ctrl Pts',(8.56059123720041,6.56303220640811,0.774513053537472)) ;
#103447=CARTESIAN_POINT('Ctrl Pts',(8.54200379397877,6.54999736403672,0.760527952934338)) ;
#103448=CARTESIAN_POINT('Ctrl Pts',(8.52069177703238,6.55000000049844,0.744478656263915)) ;
#103449=CARTESIAN_POINT('Ctrl Pts',(8.55750819780171,6.5732178281489,0.801192185467493)) ;
#103450=CARTESIAN_POINT('Ctrl Pts',(8.53873610184732,6.54999517041881,0.779473140357088)) ;
#103451=CARTESIAN_POINT('Ctrl Pts',(8.5145479773404,6.55000000088831,0.751343369175894)) ;
#103452=CARTESIAN_POINT('Ctrl Pts',(8.55505442469282,6.57990173798307,0.810707325538746)) ;
#103453=CARTESIAN_POINT('Ctrl Pts',(8.53621107118181,6.54999365791211,0.787823339593337)) ;
#103454=CARTESIAN_POINT('Ctrl Pts',(8.50963525726154,6.55000000114429,0.755173817084272)) ;
#103455=CARTESIAN_POINT('Ctrl Pts',(8.55022399280472,6.59153973477785,0.82706479408145)) ;
#103456=CARTESIAN_POINT('Ctrl Pts',(8.53156015545167,6.54999086985381,0.803378832820653)) ;
#103457=CARTESIAN_POINT('Ctrl Pts',(8.49999539447557,6.55000000159032,0.762872176320595)) ;
#103458=CARTESIAN_POINT('Ctrl Pts',(8.54779538881608,6.59665349532938,0.833083808301692)) ;
#103459=CARTESIAN_POINT('Ctrl Pts',(8.52936575151139,6.54998957391998,0.810004452644074)) ;
#103460=CARTESIAN_POINT('Ctrl Pts',(8.49512741158074,6.55000000178643,0.766663584101366)) ;
#103461=CARTESIAN_POINT('Ctrl Pts',(8.54538355337155,6.60121171185026,0.838324825515742)) ;
#103462=CARTESIAN_POINT('Ctrl Pts',(8.5273341553617,6.54998837980796,0.816101642790049)) ;
#103463=CARTESIAN_POINT('Ctrl Pts',(8.49033880598513,6.55000000196131,0.770551402901284)) ;
#103464=CARTESIAN_POINT('',(8.54582344182383,6.61635369861666,0.633936348427079)) ;
#103465=CARTESIAN_POINT('Ctrl Pts',(8.54582344182383,6.61635369861666,0.633936348427079)) ;
#103466=CARTESIAN_POINT('Ctrl Pts',(8.5449359516352,6.61793460914653,0.632605923790104)) ;
#103467=CARTESIAN_POINT('Ctrl Pts',(8.54398448171071,6.61948114927953,0.631282607169297)) ;
#103468=CARTESIAN_POINT('Ctrl Pts',(8.54296332801272,6.6209780844369,0.629959263220174)) ;
#103469=CARTESIAN_POINT('Ctrl Pts',(8.53827263106763,6.62785429629763,0.623880447238088)) ;
#103470=CARTESIAN_POINT('Ctrl Pts',(8.53198779426187,6.63349037496299,0.617388431475615)) ;
#103471=CARTESIAN_POINT('Ctrl Pts',(8.5259873730411,6.63731070037229,0.6099294107578)) ;
#103472=CARTESIAN_POINT('Ctrl Pts',(8.52000560405467,6.64111915034781,0.602493576312632)) ;
#103473=CARTESIAN_POINT('Ctrl Pts',(8.51430181273566,6.64349626850742,0.593962352698589)) ;
#103474=CARTESIAN_POINT('Ctrl Pts',(8.50998586672548,6.64522349213896,0.584799013029946)) ;
#103475=CARTESIAN_POINT('Ctrl Pts',(8.50534188065424,6.64708199603772,0.574939199749866)) ;
#103476=CARTESIAN_POINT('Ctrl Pts',(8.50212992821339,6.64824261275105,0.564112456325158)) ;
#103477=CARTESIAN_POINT('Ctrl Pts',(8.50077314609738,6.64911992656046,0.553175088083247)) ;
#103478=CARTESIAN_POINT('Ctrl Pts',(8.50025986706873,6.64945181977648,0.549037414332315)) ;
#103479=CARTESIAN_POINT('Ctrl Pts',(8.50000017127792,6.64974165917873,0.544856744898765)) ;
#103480=CARTESIAN_POINT('Ctrl Pts',(8.5000000000847,6.64999974464545,0.540682132504374)) ;
#103481=CARTESIAN_POINT('',(8.55242393572495,6.6010617218254,0.646757901283908)) ;
#103482=CARTESIAN_POINT('Ctrl Pts',(8.55241775170035,6.60106807917175,0.64676718384559)) ;
#103483=CARTESIAN_POINT('Ctrl Pts',(8.55072388788562,6.60619026743357,0.642278523047584)) ;
#103484=CARTESIAN_POINT('Ctrl Pts',(8.54858294048571,6.61143812822771,0.638073075855162)) ;
#103485=CARTESIAN_POINT('Ctrl Pts',(8.54582344182383,6.61635369861666,0.633936348427079)) ;
#103486=CARTESIAN_POINT('Ctrl Pts',(8.55635360773812,6.58637108369506,0.661367609266196)) ;
#103487=CARTESIAN_POINT('Ctrl Pts',(8.55606387390183,6.58765239867385,0.659887617192456)) ;
#103488=CARTESIAN_POINT('Ctrl Pts',(8.55575324501782,6.58896823902363,0.658434058666365)) ;
#103489=CARTESIAN_POINT('Ctrl Pts',(8.55541196992768,6.59037241127509,0.656956795059579)) ;
#103490=CARTESIAN_POINT('Ctrl Pts',(8.55524290008379,6.59106804711318,0.656224949300535)) ;
#103491=CARTESIAN_POINT('Ctrl Pts',(8.55506631250719,6.59178496983024,0.655488041162307)) ;
#103492=CARTESIAN_POINT('Ctrl Pts',(8.55488049708425,6.59252693597571,0.654743722380964)) ;
#103493=CARTESIAN_POINT('Ctrl Pts',(8.55445908016384,6.59420966544518,0.653055657291086)) ;
#103494=CARTESIAN_POINT('Ctrl Pts',(8.55403589309458,6.5958403790653,0.651511622277546)) ;
#103495=CARTESIAN_POINT('Ctrl Pts',(8.55359592981647,6.59737680581848,0.650096843766778)) ;
#103496=CARTESIAN_POINT('Ctrl Pts',(8.55324292160434,6.59860957066091,0.648961684408028)) ;
#103497=CARTESIAN_POINT('Ctrl Pts',(8.55287861047125,6.59978201473819,0.647908957492877)) ;
#103498=CARTESIAN_POINT('Ctrl Pts',(8.55248933155915,6.60087815532545,0.646922873013271)) ;
#103499=CARTESIAN_POINT('Ctrl Pts',(8.55246754857565,6.60093949235549,0.646867694422083)) ;
#103500=CARTESIAN_POINT('Ctrl Pts',(8.5524457495603,6.6010006820315,0.646812703721496)) ;
#103501=CARTESIAN_POINT('Ctrl Pts',(8.55242393572495,6.6010617218254,0.646757901283908)) ;
#103502=CARTESIAN_POINT('Ctrl Pts',(8.5,6.66256607592813,0.540287291161697)) ;
#103503=CARTESIAN_POINT('Ctrl Pts',(8.5,6.66256607592813,0.625)) ;
#103504=CARTESIAN_POINT('Ctrl Pts',(8.58356010126947,6.66256607592813,0.638926683544911)) ;
#103505=CARTESIAN_POINT('Ctrl Pts',(8.5,6.61011302719823,0.540287292737137)) ;
#103506=CARTESIAN_POINT('Ctrl Pts',(8.5,6.63245216822983,0.621442763400598)) ;
#103507=CARTESIAN_POINT('Ctrl Pts',(8.57941760042979,6.63563981885128,0.638236266738299)) ;
#103508=CARTESIAN_POINT('Ctrl Pts',(8.5,6.55934573373324,0.561153090057277)) ;
#103509=CARTESIAN_POINT('Ctrl Pts',(8.5,6.60054351783569,0.631918604172277)) ;
#103510=CARTESIAN_POINT('Ctrl Pts',(8.57705842698408,6.60987578993432,0.648272471952291)) ;
#103511=CARTESIAN_POINT('Ctrl Pts',(8.5,6.52274941072028,0.597749410720281)) ;
#103512=CARTESIAN_POINT('Ctrl Pts',(8.5,6.57873105977929,0.653731059779292)) ;
#103513=CARTESIAN_POINT('Ctrl Pts',(8.57705842661295,6.59157413088145,0.66657413088145)) ;
#103514=CARTESIAN_POINT('Origin',(8.49172374697003,1.4,-2.54)) ;
#103515=CARTESIAN_POINT('Origin',(8.49172374697003,1.4,1.96214168703487)) ;
#103516=CARTESIAN_POINT('Origin',(8.49172374697002,1.4,1.96214168703487)) ;
#103517=CARTESIAN_POINT('Origin',(8.49172374697003,1.4,1.96214168703486)) ;
#103518=CARTESIAN_POINT('Ctrl Pts',(8.50816364570057,1.49863939238321,1.96214168703488)) ;
#103519=CARTESIAN_POINT('Ctrl Pts',(8.51019246767907,1.4983012553868,1.92707241592901)) ;
#103520=CARTESIAN_POINT('Ctrl Pts',(8.50816364570057,1.47636598119991,1.89970798904169)) ;
#103521=CARTESIAN_POINT('Ctrl Pts',(8.97755831131118,1.42040694811478,1.99005134884688)) ;
#103522=CARTESIAN_POINT('Ctrl Pts',(8.97879997398668,1.42020000433584,1.95543332681748)) ;
#103523=CARTESIAN_POINT('Ctrl Pts',(8.97755831689155,1.39869563385799,1.92830518304939)) ;
#103524=CARTESIAN_POINT('Ctrl Pts',(9.4469849630597,1.34216917282336,2.01736862936927)) ;
#103525=CARTESIAN_POINT('Ctrl Pts',(9.44827639615878,1.34195393397319,1.98322247139131)) ;
#103526=CARTESIAN_POINT('Ctrl Pts',(9.44698496887878,1.3209776491576,1.95627701528915)) ;
#103527=CARTESIAN_POINT('Ctrl Pts',(9.91643989873053,1.26392668354489,2.04416188017823)) ;
#103528=CARTESIAN_POINT('Ctrl Pts',(9.91830968165731,1.26361505305709,2.01049065580299)) ;
#103529=CARTESIAN_POINT('Ctrl Pts',(9.91643989873053,1.24322097942674,1.98369643580598)) ;
#103530=CARTESIAN_POINT('Origin',(9.9,1.16528729116168,2.0441618801782)) ;
#103531=CARTESIAN_POINT('Origin',(9.9,1.16528729116168,2.0441618801782)) ;
#103532=CARTESIAN_POINT('Origin',(-0.4,-3.36847777691809,-0.4)) ;
#103533=CARTESIAN_POINT('Origin',(-0.400000000000001,-3.36847777691809,
-0.4)) ;
#103534=CARTESIAN_POINT('Origin',(-0.4,-3.36847777691809,-0.4)) ;
#103535=CARTESIAN_POINT('Origin',(-0.400000000000001,-3.36847777691809,
0.5)) ;
#103536=CARTESIAN_POINT('Origin',(-0.4,-3.36847777691809,0.4)) ;
#103537=CARTESIAN_POINT('Origin',(-1.11032778078669,-3.36847777691809,-0.4)) ;
#103538=CARTESIAN_POINT('Origin',(0.4,-3.36847777691809,-0.4)) ;
#103539=CARTESIAN_POINT('Origin',(-0.400000000000001,-3.36847777691809,
0.4)) ;
#103540=CARTESIAN_POINT('Origin',(-0.4,-3.36847777691809,0.4)) ;
#103541=CARTESIAN_POINT('Origin',(0.400000000000001,-3.36847777691809,-0.4)) ;
#103542=CARTESIAN_POINT('Origin',(0.400000000000001,-3.36847777691809,-0.4)) ;
#103543=CARTESIAN_POINT('Origin',(1.5,-3.36847777691809,0.4)) ;
#103544=CARTESIAN_POINT('Origin',(0.4,-3.36847777691809,0.4)) ;
#103545=CARTESIAN_POINT('Origin',(0.4,-3.36847777691809,0.5)) ;
#103546=CARTESIAN_POINT('Origin',(0.4,-3.36847777691809,0.4)) ;
#103547=CARTESIAN_POINT('Origin',(0.4,-3.36847777691809,0.4)) ;
#103548=CARTESIAN_POINT('Origin',(7.96847777691809,3.4,-0.4)) ;
#103549=CARTESIAN_POINT('Origin',(7.96847777691809,3.4,-0.4)) ;
#103550=CARTESIAN_POINT('Origin',(7.96847777691809,3.4,-0.4)) ;
#103551=CARTESIAN_POINT('Origin',(7.96847777691809,3.4,0.5)) ;
#103552=CARTESIAN_POINT('Origin',(7.96847777691809,3.4,0.4)) ;
#103553=CARTESIAN_POINT('Origin',(7.96847777691809,2.68967221921331,-0.4)) ;
#103554=CARTESIAN_POINT('Origin',(7.96847777691809,4.2,-0.4)) ;
#103555=CARTESIAN_POINT('Origin',(7.96847777691809,3.4,0.4)) ;
#103556=CARTESIAN_POINT('Origin',(7.96847777691809,3.4,0.4)) ;
#103557=CARTESIAN_POINT('Origin',(7.96847777691809,4.2,-0.4)) ;
#103558=CARTESIAN_POINT('Origin',(7.96847777691809,4.2,-0.4)) ;
#103559=CARTESIAN_POINT('Origin',(7.96847777691809,2.3,0.4)) ;
#103560=CARTESIAN_POINT('Origin',(7.96847777691809,4.2,0.4)) ;
#103561=CARTESIAN_POINT('Origin',(7.96847777691809,4.2,0.5)) ;
#103562=CARTESIAN_POINT('Origin',(7.96847777691809,4.2,0.4)) ;
#103563=CARTESIAN_POINT('Origin',(7.96847777691809,4.2,0.4)) ;
#103564=CARTESIAN_POINT('Origin',(8.49172374697003,1.4,-2.54)) ;
#103565=CARTESIAN_POINT('Origin',(8.49172374697003,1.4,-1.96214168703487)) ;
#103566=CARTESIAN_POINT('Origin',(8.49172374697002,1.4,-1.96214168703487)) ;
#103567=CARTESIAN_POINT('Origin',(8.49172374697003,1.39999999999989,-1.96214168703472)) ;
#103568=CARTESIAN_POINT('Ctrl Pts',(8.50816364570058,1.47636598119991,-1.89970798904169)) ;
#103569=CARTESIAN_POINT('Ctrl Pts',(8.51019246767908,1.4983012553868,-1.92707241592901)) ;
#103570=CARTESIAN_POINT('Ctrl Pts',(8.50816364570058,1.49863939238321,-1.96214168703488)) ;
#103571=CARTESIAN_POINT('Ctrl Pts',(8.97755831689156,1.39869563385799,-1.92830518304939)) ;
#103572=CARTESIAN_POINT('Ctrl Pts',(8.9787999739867,1.42020000433584,-1.95543332681749)) ;
#103573=CARTESIAN_POINT('Ctrl Pts',(8.97755831131119,1.42040694811478,-1.99005134884688)) ;
#103574=CARTESIAN_POINT('Ctrl Pts',(9.44698496887878,1.32097764915769,-1.95627701528927)) ;
#103575=CARTESIAN_POINT('Ctrl Pts',(9.44827639615882,1.34195393397354,-1.98322247139135)) ;
#103576=CARTESIAN_POINT('Ctrl Pts',(9.44698496305968,1.34216917282336,-2.0173686293693)) ;
#103577=CARTESIAN_POINT('Ctrl Pts',(9.91643989873053,1.24322097942674,-1.98369643580598)) ;
#103578=CARTESIAN_POINT('Ctrl Pts',(9.91830968165732,1.26361505305709,-2.01049065580299)) ;
#103579=CARTESIAN_POINT('Ctrl Pts',(9.91643989873053,1.26392668354489,-2.04416188017823)) ;
#103580=CARTESIAN_POINT('Origin',(9.9,1.16528729116168,-2.0441618801782)) ;
#103581=CARTESIAN_POINT('Origin',(9.9,1.16528729116168,-2.04416188017819)) ;
#103582=CARTESIAN_POINT('Origin',(8.48377223398316,8.2,-2.54)) ;
#103583=CARTESIAN_POINT('Origin',(8.48238054867376,8.20007133352901,0.74682106876079)) ;
#103584=CARTESIAN_POINT('Ctrl Pts',(8.4020166297015,8.3,0.514024022078609)) ;
#103585=CARTESIAN_POINT('Ctrl Pts',(8.50299337454956,8.3,0.527325188736439)) ;
#103586=CARTESIAN_POINT('Ctrl Pts',(8.50100123624932,8.19773961376455,0.527311153882261)) ;
#103587=CARTESIAN_POINT('Ctrl Pts',(8.39454129798958,8.3,0.565501818649352)) ;
#103588=CARTESIAN_POINT('Ctrl Pts',(8.49697875237674,8.3,0.554625888665333)) ;
#103589=CARTESIAN_POINT('Ctrl Pts',(8.49727262260755,8.20135231978535,0.554932936037724)) ;
#103590=CARTESIAN_POINT('Ctrl Pts',(8.40820218948343,8.3,0.617974636475715)) ;
#103591=CARTESIAN_POINT('Ctrl Pts',(8.49818669687003,8.3,0.577528272198747)) ;
#103592=CARTESIAN_POINT('Ctrl Pts',(8.50412619268404,8.20300739730711,0.579611589975179)) ;
#103593=CARTESIAN_POINT('Ctrl Pts',(8.44304134766321,8.3,0.669003066912872)) ;
#103594=CARTESIAN_POINT('Ctrl Pts',(8.5089417438721,8.3,0.619144944619423)) ;
#103595=CARTESIAN_POINT('Ctrl Pts',(8.52157716465942,8.21896555381604,0.609833873349667)) ;
#103596=CARTESIAN_POINT('Ctrl Pts',(8.44963266995284,8.3,0.677332168021774)) ;
#103597=CARTESIAN_POINT('Ctrl Pts',(8.51095981317519,8.3,0.626250559516498)) ;
#103598=CARTESIAN_POINT('Ctrl Pts',(8.52487915500778,8.22226238914487,0.615048381948129)) ;
#103599=CARTESIAN_POINT('Ctrl Pts',(8.46372306360151,8.3,0.693045273680071)) ;
#103600=CARTESIAN_POINT('Ctrl Pts',(8.51547368264943,8.3,0.642367208944066)) ;
#103601=CARTESIAN_POINT('Ctrl Pts',(8.53193863144478,8.23129792829963,0.626682521614473)) ;
#103602=CARTESIAN_POINT('Ctrl Pts',(8.47128983770083,8.3,0.700441372853609)) ;
#103603=CARTESIAN_POINT('Ctrl Pts',(8.51796237042372,8.3,0.650753505087224)) ;
#103604=CARTESIAN_POINT('Ctrl Pts',(8.53572833262715,8.23677343862354,0.632570411492244)) ;
#103605=CARTESIAN_POINT('Ctrl Pts',(8.48287565264707,8.3,0.711269205166843)) ;
#103606=CARTESIAN_POINT('Ctrl Pts',(8.52168214469875,8.3,0.669256480570013)) ;
#103607=CARTESIAN_POINT('Ctrl Pts',(8.54153766811345,8.25077321967987,0.647955012892664)) ;
#103608=CARTESIAN_POINT('Ctrl Pts',(8.48680760428677,8.3,0.714812702597994)) ;
#103609=CARTESIAN_POINT('Ctrl Pts',(8.52287759291298,8.3,0.675856495068285)) ;
#103610=CARTESIAN_POINT('Ctrl Pts',(8.54350322705384,8.25646917637537,0.653737733396524)) ;
#103611=CARTESIAN_POINT('Ctrl Pts',(8.49230810302881,8.3,0.720504650004493)) ;
#103612=CARTESIAN_POINT('Ctrl Pts',(8.52426411271139,8.3,0.691433475366392)) ;
#103613=CARTESIAN_POINT('Ctrl Pts',(8.54627296401924,8.26866384868896,0.671447430638399)) ;
#103614=CARTESIAN_POINT('Ctrl Pts',(8.49410170711668,8.3,0.722473481065998)) ;
#103615=CARTESIAN_POINT('Ctrl Pts',(8.52463604790915,8.3,0.697594474634863)) ;
#103616=CARTESIAN_POINT('Ctrl Pts',(8.54716490137965,8.27360757863442,0.679204040517475)) ;
#103617=CARTESIAN_POINT('Ctrl Pts',(8.49698869685298,8.3,0.726926721190466)) ;
#103618=CARTESIAN_POINT('Ctrl Pts',(8.52523118911551,8.3,0.713407065561665)) ;
#103619=CARTESIAN_POINT('Ctrl Pts',(8.54862931231184,8.28262305001769,0.702158650729551)) ;
#103620=CARTESIAN_POINT('Ctrl Pts',(8.49798687771249,8.3,0.729483478843415)) ;
#103621=CARTESIAN_POINT('Ctrl Pts',(8.52551930315387,8.3,0.723093723956201)) ;
#103622=CARTESIAN_POINT('Ctrl Pts',(8.54912969489066,8.28574379441723,0.717618102506755)) ;
#103623=CARTESIAN_POINT('Ctrl Pts',(8.49821791151748,8.3,0.737420429062632)) ;
#103624=CARTESIAN_POINT('Ctrl Pts',(8.52559423327562,8.3,0.747810875295178)) ;
#103625=CARTESIAN_POINT('Ctrl Pts',(8.54922875625408,8.28635135062007,0.756761329953168)) ;
#103626=CARTESIAN_POINT('Ctrl Pts',(8.49537847603514,8.3,0.742353089154235)) ;
#103627=CARTESIAN_POINT('Ctrl Pts',(8.52439331053439,8.3,0.758526725017863)) ;
#103628=CARTESIAN_POINT('Ctrl Pts',(8.5478189041853,8.28040548672881,0.771528206627957)) ;
#103629=CARTESIAN_POINT('Ctrl Pts',(8.48955273785443,8.3,0.751088596543062)) ;
#103630=CARTESIAN_POINT('Ctrl Pts',(8.52168703568128,8.3,0.775947414871858)) ;
#103631=CARTESIAN_POINT('Ctrl Pts',(8.54489815533717,8.27194212599121,0.793832992292969)) ;
#103632=CARTESIAN_POINT('Ctrl Pts',(8.48620077197361,8.3,0.755173692495235)) ;
#103633=CARTESIAN_POINT('Ctrl Pts',(8.52012703453237,8.3,0.782892667106739)) ;
#103634=CARTESIAN_POINT('Ctrl Pts',(8.54324008387896,8.26788967346962,0.801685764361643)) ;
#103635=CARTESIAN_POINT('Ctrl Pts',(8.48280151347419,8.3,0.759208890359289)) ;
#103636=CARTESIAN_POINT('Ctrl Pts',(8.51858761497412,8.3,0.7893479742148)) ;
#103637=CARTESIAN_POINT('Ctrl Pts',(8.54152015125556,8.26408224232382,0.808661774965266)) ;
#103638=CARTESIAN_POINT('Origin',(8.4,8.2,0.542072889850983)) ;
#103639=CARTESIAN_POINT('Origin',(8.4,8.2,-0.625)) ;
#103640=CARTESIAN_POINT('Origin',(8.4,8.2,-0.542072889850983)) ;
#103641=CARTESIAN_POINT('Ctrl Pts',(8.50101530037395,8.19768718256763,-0.527201774581488)) ;
#103642=CARTESIAN_POINT('Ctrl Pts',(8.50305639000872,8.3,-0.52721981135723)) ;
#103643=CARTESIAN_POINT('Ctrl Pts',(8.40204633857705,8.3,-0.513820202125374)) ;
#103644=CARTESIAN_POINT('Ctrl Pts',(8.4972546444163,8.20131038948434,-0.554867911909504)) ;
#103645=CARTESIAN_POINT('Ctrl Pts',(8.49701391805274,8.3,-0.554560942340225)) ;
#103646=CARTESIAN_POINT('Ctrl Pts',(8.39450526457596,8.3,-0.565363291070999)) ;
#103647=CARTESIAN_POINT('Ctrl Pts',(8.50410935041313,8.20295267265882,-0.579579296811489)) ;
#103648=CARTESIAN_POINT('Ctrl Pts',(8.498207495215,8.3,-0.577464337890648)) ;
#103649=CARTESIAN_POINT('Ctrl Pts',(8.40816401923485,8.3,-0.617918729043422)) ;
#103650=CARTESIAN_POINT('Ctrl Pts',(8.52158236570989,8.21893216789649,-0.60983004077578)) ;
#103651=CARTESIAN_POINT('Ctrl Pts',(8.50896456566522,8.3,-0.619127678384042)) ;
#103652=CARTESIAN_POINT('Ctrl Pts',(8.4430413476632,8.3,-0.669003066912864)) ;
#103653=CARTESIAN_POINT('Ctrl Pts',(8.5248849650705,8.222229916312,-0.615043706178146)) ;
#103654=CARTESIAN_POINT('Ctrl Pts',(8.51098076140207,8.3,-0.626233110976269)) ;
#103655=CARTESIAN_POINT('Ctrl Pts',(8.44963266995283,8.3,-0.677332168021764)) ;
#103656=CARTESIAN_POINT('Ctrl Pts',(8.53194575580938,8.23126818558571,-0.626675734966566)) ;
#103657=CARTESIAN_POINT('Ctrl Pts',(8.51549074202138,8.3,-0.642350503135092)) ;
#103658=CARTESIAN_POINT('Ctrl Pts',(8.46372306360151,8.3,-0.693045273680065)) ;
#103659=CARTESIAN_POINT('Ctrl Pts',(8.53573618291038,8.23674548871789,-0.632562377027298)) ;
#103660=CARTESIAN_POINT('Ctrl Pts',(8.51797743940285,8.3,-0.650737462558641)) ;
#103661=CARTESIAN_POINT('Ctrl Pts',(8.47128983770083,8.3,-0.700441372853603)) ;
#103662=CARTESIAN_POINT('Ctrl Pts',(8.54154687836688,8.25075037830457,-0.647945131945504)) ;
#103663=CARTESIAN_POINT('Ctrl Pts',(8.52169408444523,8.3,-0.669243554349282)) ;
#103664=CARTESIAN_POINT('Ctrl Pts',(8.48287565264705,8.3,-0.711269205166832)) ;
#103665=CARTESIAN_POINT('Ctrl Pts',(8.54351297666181,8.25644859419422,-0.65372727801617)) ;
#103666=CARTESIAN_POINT('Ctrl Pts',(8.52288848488737,8.3,-0.675844731548773)) ;
#103667=CARTESIAN_POINT('Ctrl Pts',(8.48680760428675,8.3,-0.714812702597982)) ;
#103668=CARTESIAN_POINT('Ctrl Pts',(8.54628376412584,8.268648468274,-0.671437623160067)) ;
#103669=CARTESIAN_POINT('Ctrl Pts',(8.52427341038692,8.3,-0.691425017040316)) ;
#103670=CARTESIAN_POINT('Ctrl Pts',(8.4923081030288,8.3,-0.720504650004482)) ;
#103671=CARTESIAN_POINT('Ctrl Pts',(8.54717611873857,8.27359443500938,-0.679194883718743)) ;
#103672=CARTESIAN_POINT('Ctrl Pts',(8.52464480444821,8.3,-0.697587339914159)) ;
#103673=CARTESIAN_POINT('Ctrl Pts',(8.49410170711666,8.3,-0.722473481065988)) ;
#103674=CARTESIAN_POINT('Ctrl Pts',(8.54864126180654,8.28261417405719,-0.702152906124747)) ;
#103675=CARTESIAN_POINT('Ctrl Pts',(8.52523908688553,8.3,-0.71340328490623)) ;
#103676=CARTESIAN_POINT('Ctrl Pts',(8.49698869685298,8.3,-0.726926721190451)) ;
#103677=CARTESIAN_POINT('Ctrl Pts',(8.54914185487159,8.28573645090423,-0.717615282415987)) ;
#103678=CARTESIAN_POINT('Ctrl Pts',(8.52552693815803,8.3,-0.723091952016155)) ;
#103679=CARTESIAN_POINT('Ctrl Pts',(8.49798687771249,8.3,-0.7294834788434)) ;
#103680=CARTESIAN_POINT('Ctrl Pts',(8.54924094958849,8.28634430798887,-0.756765947598448)) ;
#103681=CARTESIAN_POINT('Ctrl Pts',(8.52560181204939,8.30000000000001,-0.74781375175313)) ;
#103682=CARTESIAN_POINT('Ctrl Pts',(8.49821791151748,8.3,-0.737420429062617)) ;
#103683=CARTESIAN_POINT('Ctrl Pts',(8.54783079466743,8.28039553911298,-0.771534805981169)) ;
#103684=CARTESIAN_POINT('Ctrl Pts',(8.52440147378976,8.3,-0.758531275432198)) ;
#103685=CARTESIAN_POINT('Ctrl Pts',(8.49537847603514,8.3,-0.742353089154222)) ;
#103686=CARTESIAN_POINT('Ctrl Pts',(8.54465883986931,8.27120119512632,-0.795757194703311)) ;
#103687=CARTESIAN_POINT('Ctrl Pts',(8.52145785975948,8.3,-0.777490278330103)) ;
#103688=CARTESIAN_POINT('Ctrl Pts',(8.48905244827038,8.3,-0.751838764714472)) ;
#103689=CARTESIAN_POINT('Ctrl Pts',(8.54267599402788,8.26648669506706,-0.804294990430303)) ;
#103690=CARTESIAN_POINT('Ctrl Pts',(8.51958784692422,8.3,-0.78526413214459)) ;
#103691=CARTESIAN_POINT('Ctrl Pts',(8.48503640902804,8.3,-0.756568597065939)) ;
#103692=CARTESIAN_POINT('Ctrl Pts',(8.54064021294342,8.26212437554838,-0.812200029823916)) ;
#103693=CARTESIAN_POINT('Ctrl Pts',(8.51779796763701,8.3,-0.792689517015178)) ;
#103694=CARTESIAN_POINT('Ctrl Pts',(8.48104783026777,8.3,-0.761284807495046)) ;
#103695=CARTESIAN_POINT('Origin',(8.48238054717662,8.2000713259188,-0.746821067394115)) ;
#103696=CARTESIAN_POINT('Origin',(8.48377223398316,8.2,-2.54)) ;
#103697=CARTESIAN_POINT('Ctrl Pts',(8.55305389383868,6.58518362856711,-4.41981637143289)) ;
#103698=CARTESIAN_POINT('Ctrl Pts',(8.56447181517253,6.58947636230805,-4.41552363769195)) ;
#103699=CARTESIAN_POINT('Ctrl Pts',(8.57705842661295,6.59157413088145,-4.41342586911855)) ;
#103700=CARTESIAN_POINT('Ctrl Pts',(8.55305102515197,6.55898702014115,-4.39362045977753)) ;
#103701=CARTESIAN_POINT('Ctrl Pts',(8.56446969712851,6.56479854221783,-4.39084652309121)) ;
#103702=CARTESIAN_POINT('Ctrl Pts',(8.57705842709767,6.56766897765924,-4.38952071573476)) ;
#103703=CARTESIAN_POINT('Ctrl Pts',(8.55608440539073,6.54967077654144,-4.35347242603462)) ;
#103704=CARTESIAN_POINT('Ctrl Pts',(8.56803673427363,6.55578248257735,-4.35313112423482)) ;
#103705=CARTESIAN_POINT('Ctrl Pts',(8.58110225049762,6.55837193275,-4.35326484665044)) ;
#103706=CARTESIAN_POINT('Ctrl Pts',(8.56106007075016,6.56033186051354,-4.3169784615962)) ;
#103707=CARTESIAN_POINT('Ctrl Pts',(8.57385418571952,6.56560017282095,-4.31820388376166)) ;
#103708=CARTESIAN_POINT('Ctrl Pts',(8.58763814880121,6.56727264871055,-4.31859290569255)) ;
#103709=CARTESIAN_POINT('',(8.56104219912065,6.56017369985344,-4.3176338509444)) ;
#103710=CARTESIAN_POINT('',(8.55704445183396,6.58320973295706,-4.41483164119205)) ;
#103711=CARTESIAN_POINT('Ctrl Pts',(8.56104219912065,6.56017369985344,-4.3176338509444)) ;
#103712=CARTESIAN_POINT('Ctrl Pts',(8.56172006948825,6.55755272988493,-4.33050998342623)) ;
#103713=CARTESIAN_POINT('Ctrl Pts',(8.56178854742204,6.55691761311389,-4.34401886345913)) ;
#103714=CARTESIAN_POINT('Ctrl Pts',(8.56147572200372,6.55855061087387,-4.35707103715452)) ;
#103715=CARTESIAN_POINT('Ctrl Pts',(8.56116227470662,6.56018685493862,-4.37014915781354)) ;
#103716=CARTESIAN_POINT('Ctrl Pts',(8.5604843297899,6.56417103596015,-4.3831290791339)) ;
#103717=CARTESIAN_POINT('Ctrl Pts',(8.55945615587251,6.57017322470283,-4.39482221269648)) ;
#103718=CARTESIAN_POINT('Ctrl Pts',(8.55883284154061,6.57381195760859,-4.40191099175523)) ;
#103719=CARTESIAN_POINT('Ctrl Pts',(8.5580718554171,6.57823677723142,-4.40863504839524)) ;
#103720=CARTESIAN_POINT('Ctrl Pts',(8.55704487707428,6.58320791316494,-4.41483246211937)) ;
#103721=CARTESIAN_POINT('',(8.5563540329117,6.58636921675996,-4.41863023217439)) ;
#103722=CARTESIAN_POINT('Origin',(8.54420290866466,6.62817328219149,-4.38194114231836)) ;
#103723=CARTESIAN_POINT('',(8.57705842661295,6.59157413088145,-4.41342586911855)) ;
#103724=CARTESIAN_POINT('Origin',(8.6,6.52274941072028,-4.48225058927972)) ;
#103725=CARTESIAN_POINT('',(8.58355189313842,6.56397635572684,-4.342433776426)) ;
#103726=CARTESIAN_POINT('Origin',(8.59777129281767,6.65641294721993,-4.34088223593214)) ;
#103727=CARTESIAN_POINT('Ctrl Pts',(8.56104311409706,6.5601737548033,-4.31763480937229)) ;
#103728=CARTESIAN_POINT('Ctrl Pts',(8.56569547918975,6.56094902085081,-4.32312238616956)) ;
#103729=CARTESIAN_POINT('Ctrl Pts',(8.57049938306349,6.56176641478981,-4.32850925134764)) ;
#103730=CARTESIAN_POINT('Ctrl Pts',(8.57538893105739,6.56259599225632,-4.33378626613879)) ;
#103731=CARTESIAN_POINT('Ctrl Pts',(8.5780877379385,6.56305388107913,-4.33669893697213)) ;
#103732=CARTESIAN_POINT('Ctrl Pts',(8.58081254036875,6.5635152101042,-4.33957937936776)) ;
#103733=CARTESIAN_POINT('Ctrl Pts',(8.58355195315297,6.56397636517831,-4.3424336197205)) ;
#103734=CARTESIAN_POINT('Ctrl Pts',(8.5,8.3521616921714,-4.43240609825021)) ;
#103735=CARTESIAN_POINT('Ctrl Pts',(8.5,8.2900428850829,-4.40134669470595)) ;
#103736=CARTESIAN_POINT('Ctrl Pts',(8.56507848521152,8.26835005667905,-4.39050028050403)) ;
#103737=CARTESIAN_POINT('Ctrl Pts',(8.5,8.31945293993532,-4.49782359726859)) ;
#103738=CARTESIAN_POINT('Ctrl Pts',(8.5,8.26922013491181,-4.44299218879635)) ;
#103739=CARTESIAN_POINT('Ctrl Pts',(8.56507848600996,8.25199117628908,-4.42321804061861)) ;
#103740=CARTESIAN_POINT('Ctrl Pts',(8.5,8.24922766844395,-4.53971270685138)) ;
#103741=CARTESIAN_POINT('Ctrl Pts',(8.5,8.21777561643094,-4.46447736982275)) ;
#103742=CARTESIAN_POINT('Ctrl Pts',(8.57228151929423,8.21451202732349,-4.44295308011763)) ;
#103743=CARTESIAN_POINT('Ctrl Pts',(8.5,8.17221734381475,-4.5397127088383)) ;
#103744=CARTESIAN_POINT('Ctrl Pts',(8.5,8.17221734381474,-4.455)) ;
#103745=CARTESIAN_POINT('Ctrl Pts',(8.58356010126947,8.17221734381475,-4.44107331645509)) ;
#103746=CARTESIAN_POINT('',(8.50000000249538,8.20000280433619,-4.53790474363842)) ;
#103747=CARTESIAN_POINT('',(8.54742025481396,8.27608084305204,-4.39436566195595)) ;
#103748=CARTESIAN_POINT('Ctrl Pts',(8.50000000249538,8.20000280433619,-4.53790474363842)) ;
#103749=CARTESIAN_POINT('Ctrl Pts',(8.50000274011724,8.2015414376578,-4.52563544845108)) ;
#103750=CARTESIAN_POINT('Ctrl Pts',(8.50225788919788,8.20358050335012,-4.51326647497958)) ;
#103751=CARTESIAN_POINT('Ctrl Pts',(8.50614710304112,8.20657022673326,-4.50191598101389)) ;
#103752=CARTESIAN_POINT('Ctrl Pts',(8.51002595055128,8.20955198129041,-4.49059574072047)) ;
#103753=CARTESIAN_POINT('Ctrl Pts',(8.51564213392183,8.21362262975068,-4.48004613352066)) ;
#103754=CARTESIAN_POINT('Ctrl Pts',(8.52129493663065,8.21921832196825,-4.47062179223395)) ;
#103755=CARTESIAN_POINT('Ctrl Pts',(8.52933132065201,8.22717351408127,-4.45722354898551)) ;
#103756=CARTESIAN_POINT('Ctrl Pts',(8.53683691159804,8.23885362788864,-4.44566244344335)) ;
#103757=CARTESIAN_POINT('Ctrl Pts',(8.54097226482464,8.25011947738646,-4.43288116961709)) ;
#103758=CARTESIAN_POINT('Ctrl Pts',(8.54447125915462,8.25965170869904,-4.42206671140824)) ;
#103759=CARTESIAN_POINT('Ctrl Pts',(8.54617119150717,8.26873789958222,-4.40993961018965)) ;
#103760=CARTESIAN_POINT('Ctrl Pts',(8.54724932284106,8.27506683274844,-4.39656646025132)) ;
#103761=CARTESIAN_POINT('Ctrl Pts',(8.54730817192851,8.27541229338911,-4.39583649568633)) ;
#103762=CARTESIAN_POINT('Ctrl Pts',(8.5473651061662,8.27575037116516,-4.39510283260601)) ;
#103763=CARTESIAN_POINT('Ctrl Pts',(8.54742024083733,8.27608084608571,-4.39436567520734)) ;
#103764=CARTESIAN_POINT('',(8.56507848521152,8.26835005667905,-4.39050028050403)) ;
#103765=CARTESIAN_POINT('Origin',(8.6,8.3521616921714,-4.43240609825021)) ;
#103766=CARTESIAN_POINT('',(8.58356010126947,8.17221734381475,-4.44107331645509)) ;
#103767=CARTESIAN_POINT('Origin',(8.59670327708554,8.1688373429969,-4.34706896951945)) ;
#103768=CARTESIAN_POINT('',(8.5,8.17221734381475,-4.5397127088383)) ;
#103769=CARTESIAN_POINT('Origin',(8.6,8.17221734381475,-4.5397127088383)) ;
#103770=CARTESIAN_POINT('Origin',(8.50000000000027,8.16642648762921,-4.31710775120157)) ;
#103771=CARTESIAN_POINT('Origin',(2.9,3.8,-5.08)) ;
#103772=CARTESIAN_POINT('',(3.,2.4,-5.08)) ;
#103773=CARTESIAN_POINT('Origin',(3.,3.8,-5.08)) ;
#103774=CARTESIAN_POINT('',(2.9,2.3,-5.08)) ;
#103775=CARTESIAN_POINT('Origin',(2.9,2.4,-5.08)) ;
#103776=CARTESIAN_POINT('Origin',(2.9,3.8,-5.08)) ;
#103777=CARTESIAN_POINT('Origin',(1.35,3.8,-5.08)) ;
#103778=CARTESIAN_POINT('',(1.35,2.3,-5.08)) ;
#103779=CARTESIAN_POINT('Origin',(1.35,3.8,-5.08)) ;
#103780=CARTESIAN_POINT('',(1.25,2.2,-5.08)) ;
#103781=CARTESIAN_POINT('Origin',(1.35,2.2,-5.08)) ;
#103782=CARTESIAN_POINT('Origin',(1.25,3.8,-5.08)) ;
#103783=CARTESIAN_POINT('Origin',(13.9153543900904,1.02736587339764,-4.23)) ;
#103784=CARTESIAN_POINT('',(1.15,1.02736587339764,-4.33)) ;
#103785=CARTESIAN_POINT('',(1.15,0.931757800066529,-4.20068965517241)) ;
#103786=CARTESIAN_POINT('Origin',(1.15,1.02736587339764,-4.23)) ;
#103787=CARTESIAN_POINT('',(-0.900000000000002,1.02736587339765,-4.33)) ;
#103788=CARTESIAN_POINT('',(-1.,1.02736587339765,-4.33)) ;
#103789=CARTESIAN_POINT('',(-0.900000000000002,0.982644513847654,-4.31944271909999)) ;
#103790=CARTESIAN_POINT('Origin',(-0.900000000000002,1.02736587339765,-4.23)) ;
#103791=CARTESIAN_POINT('',(-0.900000000000002,0.93175780006653,-4.20068965517241)) ;
#103792=CARTESIAN_POINT('Origin',(-0.900000000000002,1.02736587339765,-4.23)) ;
#103793=CARTESIAN_POINT('',(13.9153543900904,0.931757800066525,-4.20068965517241)) ;
#103794=CARTESIAN_POINT('Origin',(13.9153543900904,1.02736587339764,-5.93)) ;
#103795=CARTESIAN_POINT('',(1.15,0.93175780006653,-5.95931034482759)) ;
#103796=CARTESIAN_POINT('',(1.15,1.02736587339765,-5.83)) ;
#103797=CARTESIAN_POINT('Origin',(1.15,1.02736587339765,-5.93)) ;
#103798=CARTESIAN_POINT('',(-0.900000000000002,0.931757800066531,-5.95931034482759)) ;
#103799=CARTESIAN_POINT('',(13.9153543900904,0.931757800066525,-5.95931034482759)) ;
#103800=CARTESIAN_POINT('',(-0.900000000000002,1.02736587339765,-5.83)) ;
#103801=CARTESIAN_POINT('Origin',(-0.900000000000002,1.02736587339765,-5.93)) ;
#103802=CARTESIAN_POINT('',(-1.,1.02736587339765,-5.83)) ;
#103803=CARTESIAN_POINT('Origin',(8.49172374697003,3.8,-5.08)) ;
#103804=CARTESIAN_POINT('',(8.49172374697003,1.47741935483871,-3.18115320609529)) ;
#103805=CARTESIAN_POINT('',(8.49172374697003,1.47741935483871,-6.97884679390471)) ;
#103806=CARTESIAN_POINT('Origin',(8.49172374697003,3.8,-5.08)) ;
#103807=CARTESIAN_POINT('',(8.50816364570057,1.47636598119991,-3.18029201095833)) ;
#103808=CARTESIAN_POINT('Origin',(8.49172374697003,1.4,-3.11785831296514)) ;
#103809=CARTESIAN_POINT('',(8.50816364570057,1.47636598119991,-6.97970798904167)) ;
#103810=CARTESIAN_POINT('Origin',(8.50816364570057,3.8,-5.08)) ;
#103811=CARTESIAN_POINT('Origin',(8.49172374697003,1.4,-7.04214168703486)) ;
#103812=CARTESIAN_POINT('Origin',(1.25,3.8,-5.08)) ;
#103813=CARTESIAN_POINT('',(1.25,2.3,-5.08)) ;
#103814=CARTESIAN_POINT('Origin',(13.9153543900904,3.8,-5.08)) ;
#103815=CARTESIAN_POINT('',(-0.900000000000002,1.47741935483872,-6.97884679390471)) ;
#103816=CARTESIAN_POINT('',(13.9153543900904,1.47741935483871,-6.97884679390471)) ;
#103817=CARTESIAN_POINT('Origin',(-0.900000000000001,3.8,-5.08)) ;
#103818=CARTESIAN_POINT('',(1.35,0.876327704607742,-5.75241379310345)) ;
#103819=CARTESIAN_POINT('Ctrl Pts',(1.35,0.876327704607742,-5.75241379310345)) ;
#103820=CARTESIAN_POINT('Ctrl Pts',(1.35,0.888571289407569,-5.80564921159528)) ;
#103821=CARTESIAN_POINT('Ctrl Pts',(1.32969623836296,0.902340613578954,
-5.85792959702133)) ;
#103822=CARTESIAN_POINT('Ctrl Pts',(1.25741074236298,0.924142973728496,
-5.93501505371577)) ;
#103823=CARTESIAN_POINT('Ctrl Pts',(1.20472523187106,0.93175780006653,-5.95931034482759)) ;
#103824=CARTESIAN_POINT('Ctrl Pts',(1.15,0.93175780006653,-5.95931034482759)) ;
#103825=CARTESIAN_POINT('',(1.35,0.876327704607742,-4.40758620689655)) ;
#103826=CARTESIAN_POINT('Origin',(1.35,3.8,-5.08)) ;
#103827=CARTESIAN_POINT('Ctrl Pts',(1.15,0.931757800066529,-4.20068965517241)) ;
#103828=CARTESIAN_POINT('Ctrl Pts',(1.20475877631964,0.931757800066529,
-4.20068965517242)) ;
#103829=CARTESIAN_POINT('Ctrl Pts',(1.2574100247738,0.924155896380522,-4.22493436088835)) ;
#103830=CARTESIAN_POINT('Ctrl Pts',(1.32987646938161,0.9022735155524,-4.30231254552791)) ;
#103831=CARTESIAN_POINT('Ctrl Pts',(1.35,0.888577265820266,-4.35432480281013)) ;
#103832=CARTESIAN_POINT('Ctrl Pts',(1.35,0.876327704607742,-4.40758620689655)) ;
#103833=CARTESIAN_POINT('',(-0.900000000000002,1.47741935483872,-3.18115320609529)) ;
#103834=CARTESIAN_POINT('Origin',(-0.900000000000001,3.8,-5.08)) ;
#103835=CARTESIAN_POINT('',(13.9153543900904,1.47741935483871,-3.18115320609529)) ;
#103836=CARTESIAN_POINT('Origin',(0.55,3.09772049281573E-17,-5.08)) ;
#103837=CARTESIAN_POINT('',(0.549999999999999,4.4,-4.63)) ;
#103838=CARTESIAN_POINT('',(0.549999999999999,4.4,-5.53)) ;
#103839=CARTESIAN_POINT('',(0.549999999999999,4.4,-5.08)) ;
#103840=CARTESIAN_POINT('',(0.55,4.04473197180486,-5.53)) ;
#103841=CARTESIAN_POINT('',(0.55,1.39397422176708E-16,-5.53)) ;
#103842=CARTESIAN_POINT('',(0.55,4.05997159067981,-5.48)) ;
#103843=CARTESIAN_POINT('Ctrl Pts',(0.549999999999999,4.04473197180486,
-5.53)) ;
#103844=CARTESIAN_POINT('Ctrl Pts',(0.549999999999999,4.04764757798806,
-5.52556486112774)) ;
#103845=CARTESIAN_POINT('Ctrl Pts',(0.549999999999999,4.05014503921306,
-5.52094814486588)) ;
#103846=CARTESIAN_POINT('Ctrl Pts',(0.549999999999999,4.0569489863933,-5.50568144569025)) ;
#103847=CARTESIAN_POINT('Ctrl Pts',(0.549999999999999,4.0599715906798,-5.49182145644142)) ;
#103848=CARTESIAN_POINT('Ctrl Pts',(0.549999999999999,4.0599715906798,-5.48)) ;
#103849=CARTESIAN_POINT('',(0.55,4.05997159067981,-4.68)) ;
#103850=CARTESIAN_POINT('',(0.55,4.05997159067981,-4.58)) ;
#103851=CARTESIAN_POINT('',(0.55,4.04473197181449,-4.63000000001465)) ;
#103852=CARTESIAN_POINT('Origin',(0.550034503802618,3.93869457792365,-4.68241602969307)) ;
#103853=CARTESIAN_POINT('',(0.55,6.35032701027224E-17,-4.63)) ;
#103854=CARTESIAN_POINT('Origin',(10.,7.8,-7.62)) ;
#103855=CARTESIAN_POINT('',(9.93162277660169,7.82279240779944,-7.62)) ;
#103856=CARTESIAN_POINT('',(8.51539501058484,8.29486832980505,-7.62)) ;
#103857=CARTESIAN_POINT('',(10.,7.8,-7.62)) ;
#103858=CARTESIAN_POINT('',(8.51540095511711,8.29487265903615,-5.84906075993417)) ;
#103859=CARTESIAN_POINT('',(8.51539501058484,8.29486832980505,-7.62)) ;
#103860=CARTESIAN_POINT('',(8.54856023413468,8.28398586203113,-5.83600806656551)) ;
#103861=CARTESIAN_POINT('Ctrl Pts',(8.51540095511711,8.29487265903615,-5.84906075993417)) ;
#103862=CARTESIAN_POINT('Ctrl Pts',(8.51716444659958,8.29428466923188,-5.84964248281888)) ;
#103863=CARTESIAN_POINT('Ctrl Pts',(8.51901954868165,8.29366521079576,-5.84997045085819)) ;
#103864=CARTESIAN_POINT('Ctrl Pts',(8.52087614409667,8.2930450194617,-5.85007250257837)) ;
#103865=CARTESIAN_POINT('Ctrl Pts',(8.52171779595218,8.29276386763785,-5.85011876576471)) ;
#103866=CARTESIAN_POINT('Ctrl Pts',(8.52256005861364,8.29248252453828,-5.85011908777802)) ;
#103867=CARTESIAN_POINT('Ctrl Pts',(8.52339613191994,8.29220315552769,-5.85007944601408)) ;
#103868=CARTESIAN_POINT('Ctrl Pts',(8.52456316579569,8.29181319797644,-5.85002411201277)) ;
#103869=CARTESIAN_POINT('Ctrl Pts',(8.52573147766845,8.29142195356397,-5.84989300499575)) ;
#103870=CARTESIAN_POINT('Ctrl Pts',(8.52689074379086,8.29103442649367,-5.84969132708601)) ;
#103871=CARTESIAN_POINT('Ctrl Pts',(8.52858695132691,8.2904674071317,-5.84939623730142)) ;
#103872=CARTESIAN_POINT('Ctrl Pts',(8.53026630212626,8.28992123633279,-5.84894392181427)) ;
#103873=CARTESIAN_POINT('Ctrl Pts',(8.5319011791312,8.28939883282067,-5.8483683729162)) ;
#103874=CARTESIAN_POINT('Ctrl Pts',(8.53241671440276,8.28923410028381,-5.84818688173578)) ;
#103875=CARTESIAN_POINT('Ctrl Pts',(8.53292790037787,8.28907155799427,-5.84799339751737)) ;
#103876=CARTESIAN_POINT('Ctrl Pts',(8.53343404910736,8.28891083250768,-5.84778983795526)) ;
#103877=CARTESIAN_POINT('Ctrl Pts',(8.5352968140817,8.28831931900687,-5.84704068340757)) ;
#103878=CARTESIAN_POINT('Ctrl Pts',(8.53711612169873,8.28774836357889,-5.84613100883356)) ;
#103879=CARTESIAN_POINT('Ctrl Pts',(8.5388519216198,8.28720494689876,-5.84506126474803)) ;
#103880=CARTESIAN_POINT('Ctrl Pts',(8.54015925159107,8.28679566878773,-5.84425557943394)) ;
#103881=CARTESIAN_POINT('Ctrl Pts',(8.54141951580281,8.286401527759,-5.84335974619183)) ;
#103882=CARTESIAN_POINT('Ctrl Pts',(8.54261761299017,8.28602171215281,-5.84239271078543)) ;
#103883=CARTESIAN_POINT('Ctrl Pts',(8.54427390694791,8.28549664098143,-5.84105584519768)) ;
#103884=CARTESIAN_POINT('Ctrl Pts',(8.5458275679526,8.28499592220792,-5.83955743369619)) ;
#103885=CARTESIAN_POINT('Ctrl Pts',(8.54719190273357,8.28456181678111,-5.83791397605226)) ;
#103886=CARTESIAN_POINT('Ctrl Pts',(8.54768505754697,8.28440490428152,-5.83731992900528)) ;
#103887=CARTESIAN_POINT('Ctrl Pts',(8.54815358395156,8.28425671205376,-5.83670743230753)) ;
#103888=CARTESIAN_POINT('Ctrl Pts',(8.54859369700692,8.28411936587098,-5.83607885456179)) ;
#103889=CARTESIAN_POINT('',(8.56837597005372,8.27720399148448,-5.81250542126692)) ;
#103890=CARTESIAN_POINT('Ctrl Pts',(8.5485198670553,8.28382649282421,-5.83601405277584)) ;
#103891=CARTESIAN_POINT('Ctrl Pts',(8.55267891820636,8.28243778061537,-5.83056312730521)) ;
#103892=CARTESIAN_POINT('Ctrl Pts',(8.5570174719569,8.28096933708253,-5.82525905778143)) ;
#103893=CARTESIAN_POINT('Ctrl Pts',(8.56150853123455,8.27945301063652,-5.82011321021338)) ;
#103894=CARTESIAN_POINT('Ctrl Pts',(8.56331520072594,8.27884302075226,-5.81804313158965)) ;
#103895=CARTESIAN_POINT('Ctrl Pts',(8.56514663435534,8.27822544298232,-5.8159980022295)) ;
#103896=CARTESIAN_POINT('Ctrl Pts',(8.56700126712393,8.27760232477898,-5.81397578565849)) ;
#103897=CARTESIAN_POINT('Ctrl Pts',(8.56745273479656,8.27745064099026,-5.81348352356526)) ;
#103898=CARTESIAN_POINT('Ctrl Pts',(8.56790562999349,8.27729861980367,-5.81299519536269)) ;
#103899=CARTESIAN_POINT('Ctrl Pts',(8.56835731300612,8.27714712982918,-5.8125055965825)) ;
#103900=CARTESIAN_POINT('',(9.93162277660169,7.82279240779944,-6.03971270883831)) ;
#103901=CARTESIAN_POINT('',(9.98593528106273,7.80468823964576,-6.04876479291514)) ;
#103902=CARTESIAN_POINT('',(9.93162277660169,7.82279240779944,-7.62)) ;
#103903=CARTESIAN_POINT('Origin',(10.,6.8,-7.62)) ;
#103904=CARTESIAN_POINT('',(10.,6.8847127088383,-7.62)) ;
#103905=CARTESIAN_POINT('',(10.,7.72792407799439,-7.62)) ;
#103906=CARTESIAN_POINT('',(10.,6.8,-7.62)) ;
#103907=CARTESIAN_POINT('',(10.,7.72792407799439,-6.03971270883831)) ;
#103908=CARTESIAN_POINT('',(10.,7.72792407799439,-7.62)) ;
#103909=CARTESIAN_POINT('',(10.,6.8847127088383,-6.03971270883831)) ;
#103910=CARTESIAN_POINT('',(10.,6.8,-6.03971270883831)) ;
#103911=CARTESIAN_POINT('',(10.,6.8847127088383,-7.62)) ;
#103912=CARTESIAN_POINT('Origin',(8.5,6.55,-7.62)) ;
#103913=CARTESIAN_POINT('',(9.91643989873054,6.78607331645509,-6.03971270883831)) ;
#103914=CARTESIAN_POINT('',(8.58355805979357,6.56393854759965,-5.81756654157067)) ;
#103915=CARTESIAN_POINT('',(8.48442535909739,6.54740422651623,-5.80104361889945)) ;
#103916=CARTESIAN_POINT('',(8.56107669735261,6.56009388000089,-5.84238384722239)) ;
#103917=CARTESIAN_POINT('Ctrl Pts',(8.58354728038625,6.56400494118525,-5.81756674863513)) ;
#103918=CARTESIAN_POINT('Ctrl Pts',(8.57838853885709,6.56313097816981,-5.82293656964759)) ;
#103919=CARTESIAN_POINT('Ctrl Pts',(8.57330127946578,6.56225500583444,-5.82838816865645)) ;
#103920=CARTESIAN_POINT('Ctrl Pts',(8.56834297134842,6.5614089984297,-5.83396078378918)) ;
#103921=CARTESIAN_POINT('Ctrl Pts',(8.56587587079895,6.56098805134781,-5.83673354448305)) ;
#103922=CARTESIAN_POINT('Ctrl Pts',(8.56344049907324,6.56057499921406,-5.83953530332025)) ;
#103923=CARTESIAN_POINT('Ctrl Pts',(8.56104288133098,6.56017406260213,-5.84236503624593)) ;
#103924=CARTESIAN_POINT('',(8.508163057485,6.55136011924237,-5.85737262210526)) ;
#103925=CARTESIAN_POINT('Ctrl Pts',(8.56125813732197,6.56020968955366,-5.84255063535367)) ;
#103926=CARTESIAN_POINT('Ctrl Pts',(8.55737139916423,6.55956189986071,-5.84720859947429)) ;
#103927=CARTESIAN_POINT('Ctrl Pts',(8.55306335190085,6.55884389198347,-5.8499674660883)) ;
#103928=CARTESIAN_POINT('Ctrl Pts',(8.5412133223275,6.55686888705458,-5.8565237407831)) ;
#103929=CARTESIAN_POINT('Ctrl Pts',(8.53496267039085,6.55582711173181,-5.85796136066778)) ;
#103930=CARTESIAN_POINT('Ctrl Pts',(8.52888665184994,6.55481444197499,-5.85927955393154)) ;
#103931=CARTESIAN_POINT('Ctrl Pts',(8.52471102104564,6.55411850350761,-5.85959774940141)) ;
#103932=CARTESIAN_POINT('Ctrl Pts',(8.52011475164494,6.55335245860749,-5.85970295993519)) ;
#103933=CARTESIAN_POINT('Ctrl Pts',(8.51754797133843,6.55292466188974,-5.85971864594294)) ;
#103934=CARTESIAN_POINT('Ctrl Pts',(8.5124831787005,6.55208052978342,-5.8589638228621)) ;
#103935=CARTESIAN_POINT('Ctrl Pts',(8.51021540604904,6.55170256767484,-5.85837089611144)) ;
#103936=CARTESIAN_POINT('Ctrl Pts',(8.50816120922225,6.55136020153704,-5.85737641152605)) ;
#103937=CARTESIAN_POINT('',(8.50816364570071,6.55136060761679,-7.62)) ;
#103938=CARTESIAN_POINT('',(8.50816364570071,6.55136060761679,-7.62)) ;
#103939=CARTESIAN_POINT('',(9.91643989873054,6.78607331645509,-7.62)) ;
#103940=CARTESIAN_POINT('',(8.5,6.55,-7.62)) ;
#103941=CARTESIAN_POINT('',(9.91643989873054,6.78607331645509,-7.62)) ;
#103942=CARTESIAN_POINT('Origin',(10.,1.5,-7.62)) ;
#103943=CARTESIAN_POINT('',(-0.900000000000002,1.5,-7.04214168703487)) ;
#103944=CARTESIAN_POINT('',(8.49172374697003,1.5,-7.04214168703487)) ;
#103945=CARTESIAN_POINT('',(10.,1.5,-7.04214168703487)) ;
#103946=CARTESIAN_POINT('',(8.49172374697003,1.5,-7.62)) ;
#103947=CARTESIAN_POINT('',(8.49172374697003,1.5,-7.62)) ;
#103948=CARTESIAN_POINT('',(-0.900000000000001,1.5,-7.62)) ;
#103949=CARTESIAN_POINT('',(10.,1.5,-7.62)) ;
#103950=CARTESIAN_POINT('',(-0.900000000000002,1.5,-7.00613602842582)) ;
#103951=CARTESIAN_POINT('Origin',(10.,1.5,-7.62)) ;
#103952=CARTESIAN_POINT('',(8.49172374697003,1.5,-2.54)) ;
#103953=CARTESIAN_POINT('',(-0.900000000000001,1.5,-2.54)) ;
#103954=CARTESIAN_POINT('',(10.,1.5,-2.54)) ;
#103955=CARTESIAN_POINT('',(8.49172374697003,1.5,-3.11785831296514)) ;
#103956=CARTESIAN_POINT('',(8.49172374697003,1.5,-7.62)) ;
#103957=CARTESIAN_POINT('',(-0.900000000000002,1.5,-3.11785831296514)) ;
#103958=CARTESIAN_POINT('',(10.,1.5,-3.11785831296514)) ;
#103959=CARTESIAN_POINT('',(-0.900000000000001,1.5,-7.62)) ;
#103960=CARTESIAN_POINT('Origin',(10.,0.,-7.62)) ;
#103961=CARTESIAN_POINT('',(10.,0.1,-2.54)) ;
#103962=CARTESIAN_POINT('',(10.,1.16528729116168,-2.54)) ;
#103963=CARTESIAN_POINT('',(10.,0.,-2.54)) ;
#103964=CARTESIAN_POINT('',(10.,0.1,-7.62)) ;
#103965=CARTESIAN_POINT('',(10.,0.1,-7.62)) ;
#103966=CARTESIAN_POINT('',(10.,1.16528729116168,-7.62)) ;
#103967=CARTESIAN_POINT('',(10.,0.,-7.62)) ;
#103968=CARTESIAN_POINT('',(10.,1.16528729116168,-7.12416188017819)) ;
#103969=CARTESIAN_POINT('',(10.,1.16528729116168,-7.62)) ;
#103970=CARTESIAN_POINT('',(10.,1.16528729116168,-3.03583811982181)) ;
#103971=CARTESIAN_POINT('Origin',(10.,3.8,-5.08)) ;
#103972=CARTESIAN_POINT('',(10.,1.16528729116168,-7.62)) ;
#103973=CARTESIAN_POINT('Origin',(0.,0.,-7.62)) ;
#103974=CARTESIAN_POINT('',(8.48377223398316,8.3,-7.62)) ;
#103975=CARTESIAN_POINT('',(7.1,8.3,-7.62)) ;
#103976=CARTESIAN_POINT('',(8.5,8.3,-7.62)) ;
#103977=CARTESIAN_POINT('Origin',(8.48377223398316,8.2,-7.62)) ;
#103978=CARTESIAN_POINT('Origin',(9.9,7.72792407799439,-7.62)) ;
#103979=CARTESIAN_POINT('Origin',(9.9,6.8847127088383,-7.62)) ;
#103980=CARTESIAN_POINT('',(8.49172374697018,6.55,-7.62)) ;
#103981=CARTESIAN_POINT('Origin',(8.49172374697018,6.65,-7.62)) ;
#103982=CARTESIAN_POINT('',(-0.900000000000001,6.55,-7.62)) ;
#103983=CARTESIAN_POINT('',(1.25,6.55,-7.62)) ;
#103984=CARTESIAN_POINT('',(-1.,6.45,-7.62)) ;
#103985=CARTESIAN_POINT('Origin',(-0.9,6.45,-7.62)) ;
#103986=CARTESIAN_POINT('',(-1.,4.65,-7.62)) ;
#103987=CARTESIAN_POINT('',(-1.,3.46944695195362E-16,-7.62)) ;
#103988=CARTESIAN_POINT('',(-0.900000000000001,4.55,-7.62)) ;
#103989=CARTESIAN_POINT('Origin',(-0.900000000000001,4.65,-7.62)) ;
#103990=CARTESIAN_POINT('',(1.15,4.55,-7.62)) ;
#103991=CARTESIAN_POINT('',(1.57859836313889E-15,4.55,-7.62)) ;
#103992=CARTESIAN_POINT('',(1.25,4.45,-7.62)) ;
#103993=CARTESIAN_POINT('Origin',(1.15,4.45,-7.62)) ;
#103994=CARTESIAN_POINT('',(1.25,3.15,-7.62)) ;
#103995=CARTESIAN_POINT('',(1.25,1.5,-7.62)) ;
#103996=CARTESIAN_POINT('',(1.15,3.05,-7.62)) ;
#103997=CARTESIAN_POINT('Origin',(1.15,3.15,-7.62)) ;
#103998=CARTESIAN_POINT('',(-0.900000000000002,3.05,-7.62)) ;
#103999=CARTESIAN_POINT('',(1.05818132034585E-15,3.05,-7.62)) ;
#104000=CARTESIAN_POINT('',(-1.,2.95,-7.62)) ;
#104001=CARTESIAN_POINT('Origin',(-0.900000000000002,2.95,-7.62)) ;
#104002=CARTESIAN_POINT('',(-1.,1.6,-7.62)) ;
#104003=CARTESIAN_POINT('',(-1.,3.46944695195362E-16,-7.62)) ;
#104004=CARTESIAN_POINT('Origin',(-0.900000000000002,1.6,-7.62)) ;
#104005=CARTESIAN_POINT('',(8.50816364570057,1.49863939238321,-7.62)) ;
#104006=CARTESIAN_POINT('Origin',(8.49172374697003,1.4,-7.62)) ;
#104007=CARTESIAN_POINT('',(9.91643989873054,1.26392668354489,-7.62)) ;
#104008=CARTESIAN_POINT('',(10.,1.24999999999998,-7.62)) ;
#104009=CARTESIAN_POINT('Origin',(9.9,1.16528729116168,-7.62)) ;
#104010=CARTESIAN_POINT('',(9.9,0.,-7.62)) ;
#104011=CARTESIAN_POINT('Origin',(9.9,0.1,-7.62)) ;
#104012=CARTESIAN_POINT('',(-2.,0.,-7.62)) ;
#104013=CARTESIAN_POINT('',(-2.,0.,-7.62)) ;
#104014=CARTESIAN_POINT('',(-2.,7.55,-7.62)) ;
#104015=CARTESIAN_POINT('',(-2.,7.65,-7.62)) ;
#104016=CARTESIAN_POINT('',(-1.9,7.65,-7.62)) ;
#104017=CARTESIAN_POINT('Origin',(-1.9,7.55,-7.62)) ;
#104018=CARTESIAN_POINT('',(6.9,7.65,-7.62)) ;
#104019=CARTESIAN_POINT('',(7.,7.65,-7.62)) ;
#104020=CARTESIAN_POINT('',(7.,7.75,-7.62)) ;
#104021=CARTESIAN_POINT('Origin',(6.9,7.75,-7.62)) ;
#104022=CARTESIAN_POINT('',(7.,8.2,-7.62)) ;
#104023=CARTESIAN_POINT('',(7.,8.3,-7.62)) ;
#104024=CARTESIAN_POINT('Origin',(7.1,8.2,-7.62)) ;
#104025=CARTESIAN_POINT('Origin',(0.,0.,-2.54)) ;
#104026=CARTESIAN_POINT('',(9.93162277660169,7.82279240779944,-2.54)) ;
#104027=CARTESIAN_POINT('',(8.51539501058484,8.29486832980505,-2.54)) ;
#104028=CARTESIAN_POINT('',(10.,7.8,-2.54)) ;
#104029=CARTESIAN_POINT('',(8.48377223398316,8.3,-2.54)) ;
#104030=CARTESIAN_POINT('Origin',(8.48377223398316,8.2,-2.54)) ;
#104031=CARTESIAN_POINT('',(7.1,8.3,-2.54)) ;
#104032=CARTESIAN_POINT('',(8.5,8.3,-2.54)) ;
#104033=CARTESIAN_POINT('',(7.,8.2,-2.54)) ;
#104034=CARTESIAN_POINT('Origin',(7.1,8.2,-2.54)) ;
#104035=CARTESIAN_POINT('',(7.,7.75,-2.54)) ;
#104036=CARTESIAN_POINT('',(7.,8.3,-2.54)) ;
#104037=CARTESIAN_POINT('',(6.9,7.65,-2.54)) ;
#104038=CARTESIAN_POINT('Origin',(6.9,7.75,-2.54)) ;
#104039=CARTESIAN_POINT('',(-1.9,7.65,-2.54)) ;
#104040=CARTESIAN_POINT('',(7.,7.65,-2.54)) ;
#104041=CARTESIAN_POINT('',(-2.,7.55,-2.54)) ;
#104042=CARTESIAN_POINT('Origin',(-1.9,7.55,-2.54)) ;
#104043=CARTESIAN_POINT('',(-2.,0.,-2.54)) ;
#104044=CARTESIAN_POINT('',(-2.,7.65,-2.54)) ;
#104045=CARTESIAN_POINT('',(9.9,0.,-2.54)) ;
#104046=CARTESIAN_POINT('',(-2.,0.,-2.54)) ;
#104047=CARTESIAN_POINT('Origin',(9.9,0.1,-2.54)) ;
#104048=CARTESIAN_POINT('',(9.91643989873054,1.26392668354489,-2.54)) ;
#104049=CARTESIAN_POINT('Origin',(9.9,1.16528729116168,-2.54)) ;
#104050=CARTESIAN_POINT('',(8.50816364570057,1.49863939238321,-2.54)) ;
#104051=CARTESIAN_POINT('',(0.472972972972955,2.83783783783779,-2.54)) ;
#104052=CARTESIAN_POINT('Origin',(8.49172374697003,1.4,-2.54)) ;
#104053=CARTESIAN_POINT('',(-1.,1.6,-2.54)) ;
#104054=CARTESIAN_POINT('Origin',(-0.900000000000002,1.6,-2.54)) ;
#104055=CARTESIAN_POINT('',(-1.,2.95,-2.54)) ;
#104056=CARTESIAN_POINT('',(-1.,3.46944695195362E-16,-2.54)) ;
#104057=CARTESIAN_POINT('',(-0.900000000000002,3.05,-2.54)) ;
#104058=CARTESIAN_POINT('Origin',(-0.900000000000002,2.95,-2.54)) ;
#104059=CARTESIAN_POINT('',(1.15,3.05,-2.54)) ;
#104060=CARTESIAN_POINT('',(1.05818132034585E-15,3.05,-2.54)) ;
#104061=CARTESIAN_POINT('',(1.25,3.15,-2.54)) ;
#104062=CARTESIAN_POINT('Origin',(1.15,3.15,-2.54)) ;
#104063=CARTESIAN_POINT('',(1.25,4.45,-2.54)) ;
#104064=CARTESIAN_POINT('',(1.25,5.3,-2.54)) ;
#104065=CARTESIAN_POINT('',(1.15,4.55,-2.54)) ;
#104066=CARTESIAN_POINT('Origin',(1.15,4.45,-2.54)) ;
#104067=CARTESIAN_POINT('',(-0.900000000000001,4.55,-2.54)) ;
#104068=CARTESIAN_POINT('',(1.57859836313889E-15,4.55,-2.54)) ;
#104069=CARTESIAN_POINT('',(-1.,4.65,-2.54)) ;
#104070=CARTESIAN_POINT('Origin',(-0.900000000000001,4.65,-2.54)) ;
#104071=CARTESIAN_POINT('',(-1.,6.45,-2.54)) ;
#104072=CARTESIAN_POINT('',(-1.,3.46944695195362E-16,-2.54)) ;
#104073=CARTESIAN_POINT('',(-0.900000000000001,6.55,-2.54)) ;
#104074=CARTESIAN_POINT('Origin',(-0.9,6.45,-2.54)) ;
#104075=CARTESIAN_POINT('',(8.49172374697018,6.55,-2.54)) ;
#104076=CARTESIAN_POINT('',(1.25,6.55,-2.54)) ;
#104077=CARTESIAN_POINT('',(8.50816364570071,6.55136060761679,-2.54)) ;
#104078=CARTESIAN_POINT('Origin',(8.49172374697018,6.65,-2.54)) ;
#104079=CARTESIAN_POINT('',(9.91643989873054,6.78607331645509,-2.54)) ;
#104080=CARTESIAN_POINT('',(8.5,6.55,-2.54)) ;
#104081=CARTESIAN_POINT('',(10.,6.8847127088383,-2.54)) ;
#104082=CARTESIAN_POINT('Origin',(9.9,6.8847127088383,-2.54)) ;
#104083=CARTESIAN_POINT('',(10.,7.72792407799439,-2.54)) ;
#104084=CARTESIAN_POINT('',(10.,6.8,-2.54)) ;
#104085=CARTESIAN_POINT('Origin',(9.9,7.72792407799439,-2.54)) ;
#104086=CARTESIAN_POINT('Origin',(7.,7.65,-7.62)) ;
#104087=CARTESIAN_POINT('',(-1.9,7.65,-7.62)) ;
#104088=CARTESIAN_POINT('',(6.9,7.65,-7.62)) ;
#104089=CARTESIAN_POINT('Origin',(7.,8.3,-7.62)) ;
#104090=CARTESIAN_POINT('',(7.,7.75,-2.54)) ;
#104091=CARTESIAN_POINT('',(7.,8.2,-7.62)) ;
#104092=CARTESIAN_POINT('Origin',(8.5,8.3,-7.62)) ;
#104093=CARTESIAN_POINT('',(8.4,8.3,-5.62207288985098)) ;
#104094=CARTESIAN_POINT('',(8.48377267093845,8.29999999999968,-5.83805254500423)) ;
#104095=CARTESIAN_POINT('Ctrl Pts',(8.4,8.3,-5.62207288985098)) ;
#104096=CARTESIAN_POINT('Ctrl Pts',(8.40000007660113,8.3,-5.63922965019375)) ;
#104097=CARTESIAN_POINT('Ctrl Pts',(8.40222537906592,8.3,-5.65619623911413)) ;
#104098=CARTESIAN_POINT('Ctrl Pts',(8.40642689896074,8.3,-5.67261625649977)) ;
#104099=CARTESIAN_POINT('Ctrl Pts',(8.41084238024295,8.3,-5.68987245931085)) ;
#104100=CARTESIAN_POINT('Ctrl Pts',(8.41744096860936,8.3,-5.70652674436269)) ;
#104101=CARTESIAN_POINT('Ctrl Pts',(8.42598957610141,8.3,-5.72216220072253)) ;
#104102=CARTESIAN_POINT('Ctrl Pts',(8.42927578125638,8.3,-5.72817269042366)) ;
#104103=CARTESIAN_POINT('Ctrl Pts',(8.43285067318462,8.3,-5.73403244695937)) ;
#104104=CARTESIAN_POINT('Ctrl Pts',(8.43670279785317,8.3,-5.73971678678546)) ;
#104105=CARTESIAN_POINT('Ctrl Pts',(8.43684245837178,8.3,-5.73992287509162)) ;
#104106=CARTESIAN_POINT('Ctrl Pts',(8.43698247939111,8.3,-5.74012872682246)) ;
#104107=CARTESIAN_POINT('Ctrl Pts',(8.43712286024713,8.3,-5.74033434069405)) ;
#104108=CARTESIAN_POINT('Ctrl Pts',(8.44304092798571,8.3,-5.74900245153563)) ;
#104109=CARTESIAN_POINT('Ctrl Pts',(8.4496323269955,8.300000000002,-5.75733173136454)) ;
#104110=CARTESIAN_POINT('Ctrl Pts',(8.45667836512368,8.29999999999776,-5.76518827396423)) ;
#104111=CARTESIAN_POINT('Ctrl Pts',(8.46347186896914,8.29999999999367,-5.77276323330906)) ;
#104112=CARTESIAN_POINT('Ctrl Pts',(8.47075094334182,8.29999999998297,-5.77990986551535)) ;
#104113=CARTESIAN_POINT('Ctrl Pts',(8.47818849074308,8.29999999991001,-5.78688161282849)) ;
#104114=CARTESIAN_POINT('Ctrl Pts',(8.47846436286148,8.2999999999073,-5.78714020757706)) ;
#104115=CARTESIAN_POINT('Ctrl Pts',(8.47874045306876,8.29999999990447,-5.78739856059915)) ;
#104116=CARTESIAN_POINT('Ctrl Pts',(8.47901674447045,8.29999999990152,-5.78765668520005)) ;
#104117=CARTESIAN_POINT('Ctrl Pts',(8.48287938578322,8.29999999986032,-5.79126534888334)) ;
#104118=CARTESIAN_POINT('Ctrl Pts',(8.4868120552941,8.29999999978803,-5.79480793672782)) ;
#104119=CARTESIAN_POINT('Ctrl Pts',(8.49047938959117,8.29999999977836,-5.79860270602181)) ;
#104120=CARTESIAN_POINT('Ctrl Pts',(8.49231307405274,8.29999999977353,-5.80050010858344)) ;
#104121=CARTESIAN_POINT('Ctrl Pts',(8.49410676862313,8.29999999978935,-5.802469327125)) ;
#104122=CARTESIAN_POINT('Ctrl Pts',(8.49555027122445,8.29999999981726,-5.80469680700993)) ;
#104123=CARTESIAN_POINT('Ctrl Pts',(8.49675259850851,8.2999999998405,-5.80655212742148)) ;
#104124=CARTESIAN_POINT('Ctrl Pts',(8.49764594203226,8.29999999986456,-5.80863681574321)) ;
#104125=CARTESIAN_POINT('Ctrl Pts',(8.49795530287013,8.29999999987615,-5.8108110374494)) ;
#104126=CARTESIAN_POINT('Ctrl Pts',(8.49801735255452,8.29999999987847,-5.81124712939817)) ;
#104127=CARTESIAN_POINT('Ctrl Pts',(8.49805590844335,8.29999999988033,-5.81168682297804)) ;
#104128=CARTESIAN_POINT('Ctrl Pts',(8.49806875158487,8.29999999988168,-5.81212898966141)) ;
#104129=CARTESIAN_POINT('Ctrl Pts',(8.49822249685464,8.2999999998978,-5.81742216780677)) ;
#104130=CARTESIAN_POINT('Ctrl Pts',(8.49538250015675,8.29999999989889,-5.82235534426841)) ;
#104131=CARTESIAN_POINT('Ctrl Pts',(8.49246863081132,8.29999999993392,-5.82672286055097)) ;
#104132=CARTESIAN_POINT('Ctrl Pts',(8.48983292606215,8.29999999996562,-5.83067344379386)) ;
#104133=CARTESIAN_POINT('Ctrl Pts',(8.48683766317129,8.3,-5.83439221106978)) ;
#104134=CARTESIAN_POINT('Ctrl Pts',(8.48377316486173,8.3,-5.83805195629754)) ;
#104135=CARTESIAN_POINT('',(8.48377223398316,8.3,-7.62)) ;
#104136=CARTESIAN_POINT('',(7.1,8.3,-7.62)) ;
#104137=CARTESIAN_POINT('',(8.48377267093845,8.29999999999968,-4.32194745499577)) ;
#104138=CARTESIAN_POINT('',(8.48377223398316,8.3,-7.62)) ;
#104139=CARTESIAN_POINT('',(8.4,8.3,-4.53792711014902)) ;
#104140=CARTESIAN_POINT('Ctrl Pts',(8.48377316486179,8.3,-4.3219480437024)) ;
#104141=CARTESIAN_POINT('Ctrl Pts',(8.48683766317134,8.3,-4.32560778893017)) ;
#104142=CARTESIAN_POINT('Ctrl Pts',(8.48983292606214,8.29999999996562,-4.32932655620614)) ;
#104143=CARTESIAN_POINT('Ctrl Pts',(8.49246863081131,8.29999999993393,-4.33327713944903)) ;
#104144=CARTESIAN_POINT('Ctrl Pts',(8.49538250015675,8.29999999989889,-4.33764465573159)) ;
#104145=CARTESIAN_POINT('Ctrl Pts',(8.49822249685463,8.2999999998978,-4.34257783219323)) ;
#104146=CARTESIAN_POINT('Ctrl Pts',(8.49806875158488,8.29999999988168,-4.34787101033859)) ;
#104147=CARTESIAN_POINT('Ctrl Pts',(8.49805590844336,8.29999999988033,-4.34831317702196)) ;
#104148=CARTESIAN_POINT('Ctrl Pts',(8.49801735255452,8.29999999987847,-4.34875287060183)) ;
#104149=CARTESIAN_POINT('Ctrl Pts',(8.49795530287013,8.29999999987615,-4.3491889625506)) ;
#104150=CARTESIAN_POINT('Ctrl Pts',(8.49764594190815,8.29999999986456,-4.35136318512907)) ;
#104151=CARTESIAN_POINT('Ctrl Pts',(8.49675259754384,8.2999999998405,-4.35344787406726)) ;
#104152=CARTESIAN_POINT('Ctrl Pts',(8.49555027122432,8.29999999981726,-4.35530319298998)) ;
#104153=CARTESIAN_POINT('Ctrl Pts',(8.49410676570211,8.29999999978935,-4.35753067738161)) ;
#104154=CARTESIAN_POINT('Ctrl Pts',(8.4923130692812,8.29999999977353,-4.359499896352)) ;
#104155=CARTESIAN_POINT('Ctrl Pts',(8.49047938958768,8.29999999977836,-4.36139729397482)) ;
#104156=CARTESIAN_POINT('Ctrl Pts',(8.48681202348067,8.29999999978803,-4.36519209617395)) ;
#104157=CARTESIAN_POINT('Ctrl Pts',(8.48287934332708,8.29999999986032,-4.36873469073021)) ;
#104158=CARTESIAN_POINT('Ctrl Pts',(8.47901674443308,8.29999999990152,-4.37234331475996)) ;
#104159=CARTESIAN_POINT('Ctrl Pts',(8.47874052296043,8.29999999990447,-4.37260137402811)) ;
#104160=CARTESIAN_POINT('Ctrl Pts',(8.4784645028431,8.2999999999073,-4.37285966135654)) ;
#104161=CARTESIAN_POINT('Ctrl Pts',(8.47818870097127,8.29999999991001,-4.3731181900299)) ;
#104162=CARTESIAN_POINT('Ctrl Pts',(8.47075185325582,8.29999999998296,-4.38008927532798)) ;
#104163=CARTESIAN_POINT('Ctrl Pts',(8.46347271757077,8.29999999998104,-4.38723682100701)) ;
#104164=CARTESIAN_POINT('Ctrl Pts',(8.45667934899943,8.29999999998018,-4.39481260831541)) ;
#104165=CARTESIAN_POINT('Ctrl Pts',(8.44963335392746,8.29999999997929,-4.40267011810317)) ;
#104166=CARTESIAN_POINT('Ctrl Pts',(8.44304226791565,8.29999999996634,-4.41100025634497)) ;
#104167=CARTESIAN_POINT('Ctrl Pts',(8.43712466127421,8.29999999997622,-4.419666888942)) ;
#104168=CARTESIAN_POINT('Ctrl Pts',(8.43698358608697,8.29999999997646,-4.41987350065015)) ;
#104169=CARTESIAN_POINT('Ctrl Pts',(8.43684287437574,8.2999999999767,-4.42008035127934)) ;
#104170=CARTESIAN_POINT('Ctrl Pts',(8.43670252680326,8.29999999997696,-4.42028743949552)) ;
#104171=CARTESIAN_POINT('Ctrl Pts',(8.42665365624234,8.29999999999548,-4.43511493271378)) ;
#104172=CARTESIAN_POINT('Ctrl Pts',(8.41848789916361,8.29999999999779,-4.45113486319109)) ;
#104173=CARTESIAN_POINT('Ctrl Pts',(8.41242260582447,8.29999999999911,-4.46791805139592)) ;
#104174=CARTESIAN_POINT('Ctrl Pts',(8.40662497274242,8.30000000000037,-4.48396060065411)) ;
#104175=CARTESIAN_POINT('Ctrl Pts',(8.40274598945985,8.3,-4.50070219391449)) ;
#104176=CARTESIAN_POINT('Ctrl Pts',(8.40101973895747,8.3,-4.51777978833517)) ;
#104177=CARTESIAN_POINT('Ctrl Pts',(8.40034533497825,8.3,-4.52445158806355)) ;
#104178=CARTESIAN_POINT('Ctrl Pts',(8.40000003014814,8.3,-4.53117467303786)) ;
#104179=CARTESIAN_POINT('Ctrl Pts',(8.4,8.3,-4.53792711014902)) ;
#104180=CARTESIAN_POINT('',(8.4,8.3,-5.66365455630091)) ;
#104181=CARTESIAN_POINT('Origin',(10.,7.8,-7.62)) ;
#104182=CARTESIAN_POINT('',(8.56837722373805,8.27720759208727,-4.3474948832495)) ;
#104183=CARTESIAN_POINT('',(8.54843785958924,8.28385404680359,-4.3239803122607)) ;
#104184=CARTESIAN_POINT('Ctrl Pts',(8.56837722339832,8.27720759220056,-4.34749488336226)) ;
#104185=CARTESIAN_POINT('Ctrl Pts',(8.56792584473107,8.27735805175631,-4.34700469022775)) ;
#104186=CARTESIAN_POINT('Ctrl Pts',(8.56747319573485,8.27750893475505,-4.34651579326377)) ;
#104187=CARTESIAN_POINT('Ctrl Pts',(8.56702308739659,8.2776589708678,-4.34602430395872)) ;
#104188=CARTESIAN_POINT('Ctrl Pts',(8.56055949575605,8.27981350141465,-4.33896647833431)) ;
#104189=CARTESIAN_POINT('Ctrl Pts',(8.5543545977397,8.28188180075344,-4.33162839546916)) ;
#104190=CARTESIAN_POINT('Ctrl Pts',(8.54852002808959,8.28382665730347,-4.32398586635143)) ;
#104191=CARTESIAN_POINT('',(8.51539953939799,8.29486682020067,-4.31094033012292)) ;
#104192=CARTESIAN_POINT('Origin',(8.52916905055949,8.29027698314684,-4.330734470479)) ;
#104193=CARTESIAN_POINT('',(8.51539501058484,8.29486832980505,-7.62)) ;
#104194=CARTESIAN_POINT('',(9.93162277660169,7.82279240779944,-4.1202872911617)) ;
#104195=CARTESIAN_POINT('',(9.93162277660169,7.82279240779944,-7.62)) ;
#104196=CARTESIAN_POINT('',(8.48593528106273,8.30468823964576,-4.36123520708486)) ;
#104197=CARTESIAN_POINT('Origin',(10.,6.8,-7.62)) ;
#104198=CARTESIAN_POINT('',(10.,6.8847127088383,-4.1202872911617)) ;
#104199=CARTESIAN_POINT('',(10.,7.72792407799439,-4.1202872911617)) ;
#104200=CARTESIAN_POINT('',(10.,7.8,-4.1202872911617)) ;
#104201=CARTESIAN_POINT('',(10.,7.72792407799439,-7.62)) ;
#104202=CARTESIAN_POINT('',(10.,6.8847127088383,-7.62)) ;
#104203=CARTESIAN_POINT('Origin',(8.5,6.55,-7.62)) ;
#104204=CARTESIAN_POINT('',(8.50816305748853,6.55136011924294,-4.3026273778919)) ;
#104205=CARTESIAN_POINT('Ctrl Pts',(8.5081612092262,6.5513602015377,-4.30262358847201)) ;
#104206=CARTESIAN_POINT('Ctrl Pts',(8.50982330775196,6.55163721795866,-4.30181892781797)) ;
#104207=CARTESIAN_POINT('Ctrl Pts',(8.51162127657706,6.55193687942951,-4.30127902844118)) ;
#104208=CARTESIAN_POINT('Ctrl Pts',(8.51523682141403,6.55253947023567,-4.30057109233524)) ;
#104209=CARTESIAN_POINT('Ctrl Pts',(8.51710259142332,6.55285043190389,-4.30039346793935)) ;
#104210=CARTESIAN_POINT('Ctrl Pts',(8.52217030373161,6.55369505062194,-4.30023569112656)) ;
#104211=CARTESIAN_POINT('Ctrl Pts',(8.52587381749813,6.55431230291636,-4.30048388339438)) ;
#104212=CARTESIAN_POINT('Ctrl Pts',(8.53482421527827,6.55580403587971,-4.3017298501838)) ;
#104213=CARTESIAN_POINT('Ctrl Pts',(8.53952102462486,6.55658683673452,-4.30322044742312)) ;
#104214=CARTESIAN_POINT('Ctrl Pts',(8.54640674065651,6.55773445607313,-4.30636821224513)) ;
#104215=CARTESIAN_POINT('Ctrl Pts',(8.55013419152096,6.55835569858683,-4.30823673022989)) ;
#104216=CARTESIAN_POINT('Ctrl Pts',(8.55581906875064,6.55930317812511,-4.31204337542897)) ;
#104217=CARTESIAN_POINT('Ctrl Pts',(8.55861150732083,6.55976858455347,-4.31427755556237)) ;
#104218=CARTESIAN_POINT('Ctrl Pts',(8.5612582140973,6.56020970234955,-4.31744945665611)) ;
#104219=CARTESIAN_POINT('',(9.91643989873054,6.78607331645509,-4.1202872911617)) ;
#104220=CARTESIAN_POINT('',(9.98442535909739,6.79740422651623,-4.10895638110055)) ;
#104221=CARTESIAN_POINT('',(9.91643989873054,6.78607331645509,-7.62)) ;
#104222=CARTESIAN_POINT('',(8.50816364570071,6.55136060761679,-7.62)) ;
#104223=CARTESIAN_POINT('Origin',(1.25,6.55,-7.62)) ;
#104224=CARTESIAN_POINT('',(8.49172372711481,6.55000000000007,-5.8494558427306)) ;
#104225=CARTESIAN_POINT('',(8.49172374697018,6.55,-7.62)) ;
#104226=CARTESIAN_POINT('',(8.4,6.55,-5.6206780018997)) ;
#104227=CARTESIAN_POINT('Ctrl Pts',(8.49172374697018,6.55000000000105,-5.84945574565572)) ;
#104228=CARTESIAN_POINT('Ctrl Pts',(8.49606803673628,6.55000000001052,-5.84595058632692)) ;
#104229=CARTESIAN_POINT('Ctrl Pts',(8.50046735944504,6.54999999990302,-5.84251190424928)) ;
#104230=CARTESIAN_POINT('Ctrl Pts',(8.50920280475187,6.55000000136501,-5.83551602670204)) ;
#104231=CARTESIAN_POINT('Ctrl Pts',(8.51365366733357,6.55000000372466,-5.83201891829248)) ;
#104232=CARTESIAN_POINT('Ctrl Pts',(8.51786969589099,6.55000000840872,-5.82757405149189)) ;
#104233=CARTESIAN_POINT('Ctrl Pts',(8.51824835575334,6.5500000088438,-5.82716283435581)) ;
#104234=CARTESIAN_POINT('Ctrl Pts',(8.51893753951069,6.55000000964298,-5.82638941226416)) ;
#104235=CARTESIAN_POINT('Ctrl Pts',(8.51925555226623,6.55000001000021,-5.82602468306099)) ;
#104236=CARTESIAN_POINT('Ctrl Pts',(8.52125362518914,6.55000001218547,-5.82363696640081)) ;
#104237=CARTESIAN_POINT('Ctrl Pts',(8.52280131776513,6.55000000862055,-5.82136252157375)) ;
#104238=CARTESIAN_POINT('Ctrl Pts',(8.52354796988915,6.55000000490364,-5.8162172682012)) ;
#104239=CARTESIAN_POINT('Ctrl Pts',(8.52233587755857,6.5500000056078,-5.81356291782334)) ;
#104240=CARTESIAN_POINT('Ctrl Pts',(8.52032554216556,6.55000000470579,-5.81116101057052)) ;
#104241=CARTESIAN_POINT('Ctrl Pts',(8.52004618744961,6.55000000456892,-5.81085546722455)) ;
#104242=CARTESIAN_POINT('Ctrl Pts',(8.51943244221705,6.55000000425259,-5.81023755755062)) ;
#104243=CARTESIAN_POINT('Ctrl Pts',(8.51910103101855,6.55000000405877,-5.80991727732132)) ;
#104244=CARTESIAN_POINT('Ctrl Pts',(8.51460799223804,6.5500000014124,-5.8057349310042)) ;
#104245=CARTESIAN_POINT('Ctrl Pts',(8.50969722522559,6.55000000036127,-5.80296024115299)) ;
#104246=CARTESIAN_POINT('Ctrl Pts',(8.50463600502758,6.55000000021577,-5.79966347483879)) ;
#104247=CARTESIAN_POINT('Ctrl Pts',(8.50427412871944,6.55000000020764,-5.79942728012652)) ;
#104248=CARTESIAN_POINT('Ctrl Pts',(8.49410349041847,6.55000000002642,-5.79277433128147)) ;
#104249=CARTESIAN_POINT('Ctrl Pts',(8.48448997361522,6.54999999999179,-5.78608093896228)) ;
#104250=CARTESIAN_POINT('Ctrl Pts',(8.46629237463077,6.55000000001684,-5.77097702438866)) ;
#104251=CARTESIAN_POINT('Ctrl Pts',(8.45766562693772,6.55000000000152,-5.76259393166186)) ;
#104252=CARTESIAN_POINT('Ctrl Pts',(8.44955830666691,6.54999999999999,-5.75321233426814)) ;
#104253=CARTESIAN_POINT('Ctrl Pts',(8.44937081015217,6.54999999999999,-5.75299442831169)) ;
#104254=CARTESIAN_POINT('Ctrl Pts',(8.43720071044327,6.5500000000026,-5.7387892740207)) ;
#104255=CARTESIAN_POINT('Ctrl Pts',(8.42721384365609,6.55000000009149,-5.72325666818742)) ;
#104256=CARTESIAN_POINT('Ctrl Pts',(8.41184903642134,6.55000000007035,-5.6905950553132)) ;
#104257=CARTESIAN_POINT('Ctrl Pts',(8.40635547808108,6.5500000000232,-5.67351733252205)) ;
#104258=CARTESIAN_POINT('Ctrl Pts',(8.40108598764522,6.5499999999995,-5.6443588087486)) ;
#104259=CARTESIAN_POINT('Ctrl Pts',(8.4,6.55,-5.63255952793497)) ;
#104260=CARTESIAN_POINT('Ctrl Pts',(8.4,6.55,-5.6206780018997)) ;
#104261=CARTESIAN_POINT('',(8.4,6.55,-4.5393219981003)) ;
#104262=CARTESIAN_POINT('',(8.4,6.55,-4.35636060761679)) ;
#104263=CARTESIAN_POINT('',(8.4917237271148,6.5500000000004,-4.31054415726839)) ;
#104264=CARTESIAN_POINT('Ctrl Pts',(8.4,6.55,-4.5393219981003)) ;
#104265=CARTESIAN_POINT('Ctrl Pts',(8.4,6.55,-4.52146035159378)) ;
#104266=CARTESIAN_POINT('Ctrl Pts',(8.40245177849675,6.55000000000111,-4.50378505808852)) ;
#104267=CARTESIAN_POINT('Ctrl Pts',(8.40709634751579,6.55000000003438,-4.48675184875404)) ;
#104268=CARTESIAN_POINT('Ctrl Pts',(8.41193897064716,6.55000000006908,-4.46899230783935)) ;
#104269=CARTESIAN_POINT('Ctrl Pts',(8.41916594308319,6.55000000013771,-4.45192888813902)) ;
#104270=CARTESIAN_POINT('Ctrl Pts',(8.42853896333909,6.55000000013582,-4.43608126731276)) ;
#104271=CARTESIAN_POINT('Ctrl Pts',(8.43455058706114,6.55000000013461,-4.42591699467746)) ;
#104272=CARTESIAN_POINT('Ctrl Pts',(8.44144611055395,6.55000000009671,-4.416253000721)) ;
#104273=CARTESIAN_POINT('Ctrl Pts',(8.44917210140206,6.55000000005186,-4.40723268310165)) ;
#104274=CARTESIAN_POINT('Ctrl Pts',(8.44936219523639,6.55000000005075,-4.40701074305579)) ;
#104275=CARTESIAN_POINT('Ctrl Pts',(8.44955278293316,6.55000000004968,-4.40678920228627)) ;
#104276=CARTESIAN_POINT('Ctrl Pts',(8.44974386351697,6.55000000004865,-4.40656806301674)) ;
#104277=CARTESIAN_POINT('Ctrl Pts',(8.45766118910685,6.55000000000559,-4.39740527126338)) ;
#104278=CARTESIAN_POINT('Ctrl Pts',(8.46628870646479,6.54999999999864,-4.38902155150326)) ;
#104279=CARTESIAN_POINT('Ctrl Pts',(8.47555348469884,6.55000000000007,-4.38133527594906)) ;
#104280=CARTESIAN_POINT('Ctrl Pts',(8.48448851770303,6.55000000000144,-4.37392256470859)) ;
#104281=CARTESIAN_POINT('Ctrl Pts',(8.49410273695376,6.5500000000304,-4.36723469297055)) ;
#104282=CARTESIAN_POINT('Ctrl Pts',(8.50391213313781,6.55000000016212,-4.36082389577119)) ;
#104283=CARTESIAN_POINT('Ctrl Pts',(8.50409415224108,6.55000000016456,-4.3607049396667)) ;
#104284=CARTESIAN_POINT('Ctrl Pts',(8.50427622716234,6.55000000016576,-4.36058605979315)) ;
#104285=CARTESIAN_POINT('Ctrl Pts',(8.50445835579895,6.55000000016577,-4.36046725463206)) ;
#104286=CARTESIAN_POINT('Ctrl Pts',(8.50464048443556,6.55000000016577,-4.36034844947096)) ;
#104287=CARTESIAN_POINT('Ctrl Pts',(8.50482266678753,6.55000000016459,-4.36022971902233)) ;
#104288=CARTESIAN_POINT('Ctrl Pts',(8.50500490075221,6.55000000016234,-4.36011106176766)) ;
#104289=CARTESIAN_POINT('Ctrl Pts',(8.50970297364421,6.55000000010443,-4.35705202481731)) ;
#104290=CARTESIAN_POINT('Ctrl Pts',(8.51460443926437,6.55000000028677,-4.35427565407058)) ;
#104291=CARTESIAN_POINT('Ctrl Pts',(8.5187483092633,6.55000000038295,-4.35043698472842)) ;
#104292=CARTESIAN_POINT('Ctrl Pts',(8.51909542442958,6.550000000391,-4.35011543498209)) ;
#104293=CARTESIAN_POINT('Ctrl Pts',(8.51943721516333,6.55000000039357,-4.34978641450153)) ;
#104294=CARTESIAN_POINT('Ctrl Pts',(8.51977310187182,6.55000000039098,-4.3494491161473)) ;
#104295=CARTESIAN_POINT('Ctrl Pts',(8.52085916897636,6.5500000003826,-4.34835848458113)) ;
#104296=CARTESIAN_POINT('Ctrl Pts',(8.52182399801739,6.55000000033868,-4.347044620882)) ;
#104297=CARTESIAN_POINT('Ctrl Pts',(8.52246334063461,6.55000000029842,-4.34562676665967)) ;
#104298=CARTESIAN_POINT('Ctrl Pts',(8.52278301194322,6.55000000027829,-4.34491783954851)) ;
#104299=CARTESIAN_POINT('Ctrl Pts',(8.52302131164588,6.55000000025926,-4.34418291480655)) ;
#104300=CARTESIAN_POINT('Ctrl Pts',(8.52315270869754,6.55000000024662,-4.343436897635)) ;
#104301=CARTESIAN_POINT('Ctrl Pts',(8.5232841057492,6.55000000023398,-4.34269088046346)) ;
#104302=CARTESIAN_POINT('Ctrl Pts',(8.52330860014988,6.55000000022778,-4.34193377086234)) ;
#104303=CARTESIAN_POINT('Ctrl Pts',(8.52320066085452,6.55000000023233,-4.34118047403285)) ;
#104304=CARTESIAN_POINT('Ctrl Pts',(8.52284031330749,6.55000000024754,-4.33866564693691)) ;
#104305=CARTESIAN_POINT('Ctrl Pts',(8.52133564423351,6.55000000029586,-4.33640673801311)) ;
#104306=CARTESIAN_POINT('Ctrl Pts',(8.5196587899188,6.55000000031744,-4.33439865149543)) ;
#104307=CARTESIAN_POINT('Ctrl Pts',(8.51932554032813,6.55000000032173,-4.33399957448309)) ;
#104308=CARTESIAN_POINT('Ctrl Pts',(8.51898545723479,6.55000000032523,-4.33361037576486)) ;
#104309=CARTESIAN_POINT('Ctrl Pts',(8.51864615038492,6.55000000032769,-4.33323101231938)) ;
#104310=CARTESIAN_POINT('Ctrl Pts',(8.5145508165866,6.55000000035749,-4.32865220720328)) ;
#104311=CARTESIAN_POINT('Ctrl Pts',(8.50963987409779,6.55000000028079,-4.32482020861865)) ;
#104312=CARTESIAN_POINT('Ctrl Pts',(8.5048217738226,6.55000000018959,-4.32096887012539)) ;
#104313=CARTESIAN_POINT('Ctrl Pts',(8.5004640292375,6.5500000001071,-4.31748551600118)) ;
#104314=CARTESIAN_POINT('Ctrl Pts',(8.49606692679176,6.55000000001227,-4.31404901054623)) ;
#104315=CARTESIAN_POINT('Ctrl Pts',(8.49172374697018,6.55000000000105,-4.3105442543438)) ;
#104316=CARTESIAN_POINT('',(8.49172374697018,6.55,-7.62)) ;
#104317=CARTESIAN_POINT('',(-0.9,6.55,-4.23)) ;
#104318=CARTESIAN_POINT('',(-0.900000000000001,6.55,-7.62)) ;
#104319=CARTESIAN_POINT('',(1.15,6.55,-4.23)) ;
#104320=CARTESIAN_POINT('',(1.25,6.55,-4.23)) ;
#104321=CARTESIAN_POINT('',(1.35,6.55,-4.43)) ;
#104322=CARTESIAN_POINT('Origin',(1.15,6.55,-4.43)) ;
#104323=CARTESIAN_POINT('',(1.35,6.55,-5.73)) ;
#104324=CARTESIAN_POINT('',(1.35,6.55,-5.83)) ;
#104325=CARTESIAN_POINT('',(1.15,6.55,-5.93)) ;
#104326=CARTESIAN_POINT('Origin',(1.15,6.55,-5.73)) ;
#104327=CARTESIAN_POINT('',(-0.9,6.55,-5.93)) ;
#104328=CARTESIAN_POINT('',(1.25,6.55,-5.93)) ;
#104329=CARTESIAN_POINT('',(-0.9,6.55,-7.62)) ;
#104330=CARTESIAN_POINT('Origin',(1.25,5.3,-7.62)) ;
#104331=CARTESIAN_POINT('',(1.25,3.15,-6.7231676725155)) ;
#104332=CARTESIAN_POINT('',(1.25,3.04189189189189,-6.54552792413544)) ;
#104333=CARTESIAN_POINT('Origin',(1.25,2.95,-6.7231676725155)) ;
#104334=CARTESIAN_POINT('',(1.25,3.15,-7.62)) ;
#104335=CARTESIAN_POINT('',(1.25,4.45,-6.7231676725155)) ;
#104336=CARTESIAN_POINT('',(1.25,4.45,-6.66113883008419)) ;
#104337=CARTESIAN_POINT('',(1.25,4.55810810810811,-6.54552792413544)) ;
#104338=CARTESIAN_POINT('Origin',(1.25,4.65,-6.7231676725155)) ;
#104339=CARTESIAN_POINT('',(1.25,5.26552792413544,-5.83810810810811)) ;
#104340=CARTESIAN_POINT('Origin',(1.25,3.8,-5.08)) ;
#104341=CARTESIAN_POINT('',(1.25,5.4431676725155,-5.73)) ;
#104342=CARTESIAN_POINT('Origin',(1.25,5.4431676725155,-5.93)) ;
#104343=CARTESIAN_POINT('',(1.25,6.45,-5.73)) ;
#104344=CARTESIAN_POINT('',(1.25,6.55,-5.73)) ;
#104345=CARTESIAN_POINT('',(1.25,6.45,-4.43)) ;
#104346=CARTESIAN_POINT('',(1.25,6.45,-4.33)) ;
#104347=CARTESIAN_POINT('',(1.25,5.4431676725155,-4.43)) ;
#104348=CARTESIAN_POINT('',(1.25,5.38113883008419,-4.43)) ;
#104349=CARTESIAN_POINT('',(1.25,5.26552792413544,-4.32189189189189)) ;
#104350=CARTESIAN_POINT('Origin',(1.25,5.4431676725155,-4.23)) ;
#104351=CARTESIAN_POINT('',(1.25,4.55810810810811,-3.61447207586456)) ;
#104352=CARTESIAN_POINT('Origin',(1.25,3.8,-5.08)) ;
#104353=CARTESIAN_POINT('',(1.25,4.45,-3.4368323274845)) ;
#104354=CARTESIAN_POINT('Origin',(1.25,4.65,-3.4368323274845)) ;
#104355=CARTESIAN_POINT('',(1.25,4.45,-2.54)) ;
#104356=CARTESIAN_POINT('',(1.25,3.15,-3.4368323274845)) ;
#104357=CARTESIAN_POINT('',(1.25,3.15,-3.49886116991581)) ;
#104358=CARTESIAN_POINT('',(1.25,3.04189189189189,-3.61447207586456)) ;
#104359=CARTESIAN_POINT('Origin',(1.25,2.95,-3.4368323274845)) ;
#104360=CARTESIAN_POINT('',(1.25,2.33447207586456,-4.32189189189189)) ;
#104361=CARTESIAN_POINT('Origin',(1.25,3.8,-5.08)) ;
#104362=CARTESIAN_POINT('',(1.25,2.1568323274845,-4.43)) ;
#104363=CARTESIAN_POINT('Origin',(1.25,2.1568323274845,-4.23)) ;
#104364=CARTESIAN_POINT('',(1.25,0.973783447787483,-4.43)) ;
#104365=CARTESIAN_POINT('',(1.25,0.895262490344437,-4.43)) ;
#104366=CARTESIAN_POINT('',(1.25,0.973783447787483,-5.73)) ;
#104367=CARTESIAN_POINT('Origin',(1.25,3.8,-5.08)) ;
#104368=CARTESIAN_POINT('',(1.25,2.1568323274845,-5.73)) ;
#104369=CARTESIAN_POINT('',(1.25,2.21886116991581,-5.73)) ;
#104370=CARTESIAN_POINT('',(1.25,2.33447207586456,-5.83810810810811)) ;
#104371=CARTESIAN_POINT('Origin',(1.25,2.1568323274845,-5.93)) ;
#104372=CARTESIAN_POINT('Origin',(1.25,3.8,-5.08)) ;
#104373=CARTESIAN_POINT('Origin',(-2.,0.,-7.62)) ;
#104374=CARTESIAN_POINT('',(0.899999999999999,0.,-6.68)) ;
#104375=CARTESIAN_POINT('',(1.1,0.,-6.48)) ;
#104376=CARTESIAN_POINT('Origin',(0.899999999999999,0.,-6.48)) ;
#104377=CARTESIAN_POINT('',(-2.,0.,-6.68)) ;
#104378=CARTESIAN_POINT('',(-2.,0.,-6.68)) ;
#104379=CARTESIAN_POINT('',(-2.,0.,-7.62)) ;
#104380=CARTESIAN_POINT('',(9.9,0.,-7.62)) ;
#104381=CARTESIAN_POINT('',(-2.,0.,-3.48)) ;
#104382=CARTESIAN_POINT('',(-2.,0.,-7.62)) ;
#104383=CARTESIAN_POINT('',(0.899999999999999,0.,-3.48)) ;
#104384=CARTESIAN_POINT('',(0.999999999999999,0.,-3.48)) ;
#104385=CARTESIAN_POINT('',(1.1,0.,-3.68)) ;
#104386=CARTESIAN_POINT('Origin',(0.899999999999999,0.,-3.68)) ;
#104387=CARTESIAN_POINT('',(1.1,0.,-6.58)) ;
#104388=CARTESIAN_POINT('Origin',(-2.,7.65,-7.62)) ;
#104389=CARTESIAN_POINT('',(-2.,6.9,-3.48)) ;
#104390=CARTESIAN_POINT('',(-2.,7.1,-3.68)) ;
#104391=CARTESIAN_POINT('Origin',(-2.,6.9,-3.68)) ;
#104392=CARTESIAN_POINT('',(-2.,-1.13380619344889E-17,-3.48)) ;
#104393=CARTESIAN_POINT('',(-2.,7.55,-7.62)) ;
#104394=CARTESIAN_POINT('',(-2.,6.9,-6.68)) ;
#104395=CARTESIAN_POINT('',(-2.,7.,-6.68)) ;
#104396=CARTESIAN_POINT('',(-2.,7.1,-6.48)) ;
#104397=CARTESIAN_POINT('Origin',(-2.,6.9,-6.48)) ;
#104398=CARTESIAN_POINT('',(-2.,7.1,-3.58)) ;
#104399=CARTESIAN_POINT('Origin',(-1.8,7.,-3.58)) ;
#104400=CARTESIAN_POINT('',(-1.7,0.1,-3.58)) ;
#104401=CARTESIAN_POINT('',(-1.9,0.1,-3.58)) ;
#104402=CARTESIAN_POINT('',(-2.,0.1,-3.58)) ;
#104403=CARTESIAN_POINT('',(-1.9,0.3,-3.58)) ;
#104404=CARTESIAN_POINT('',(-1.9,7.,-3.58)) ;
#104405=CARTESIAN_POINT('Origin',(-1.7,0.3,-3.58)) ;
#104406=CARTESIAN_POINT('Origin',(-1.8,7.,-6.58)) ;
#104407=CARTESIAN_POINT('',(-1.9,0.3,-6.58)) ;
#104408=CARTESIAN_POINT('',(-1.7,0.1,-6.58)) ;
#104409=CARTESIAN_POINT('Origin',(-1.7,0.3,-6.58)) ;
#104410=CARTESIAN_POINT('',(-1.9,0.1,-6.58)) ;
#104411=CARTESIAN_POINT('',(-1.9,1.23908819712629E-17,-6.58)) ;
#104412=CARTESIAN_POINT('',(0.999999999999999,0.1,-6.58)) ;
#104413=CARTESIAN_POINT('Origin',(-1.8,-2.2514151555628E-16,-5.08)) ;
#104414=CARTESIAN_POINT('',(-1.8,4.6,-5.73)) ;
#104415=CARTESIAN_POINT('',(-1.8,4.6,-4.43)) ;
#104416=CARTESIAN_POINT('',(-1.8,4.6,-4.53)) ;
#104417=CARTESIAN_POINT('',(-1.8,0.3,-4.43)) ;
#104418=CARTESIAN_POINT('',(-1.8,0.2,-4.43)) ;
#104419=CARTESIAN_POINT('',(-1.8,0.3,-3.68)) ;
#104420=CARTESIAN_POINT('',(-1.8,0.3,-3.58)) ;
#104421=CARTESIAN_POINT('',(-1.8,6.9,-3.68)) ;
#104422=CARTESIAN_POINT('',(-1.8,-5.16691679585995E-17,-3.68)) ;
#104423=CARTESIAN_POINT('',(-1.8,6.9,-6.48)) ;
#104424=CARTESIAN_POINT('',(-1.8,6.9,-5.08)) ;
#104425=CARTESIAN_POINT('',(-1.8,0.3,-6.48)) ;
#104426=CARTESIAN_POINT('',(-1.8,-3.98613863153961E-16,-6.48)) ;
#104427=CARTESIAN_POINT('',(-1.8,0.3,-5.73)) ;
#104428=CARTESIAN_POINT('',(-1.8,0.3,-5.63)) ;
#104429=CARTESIAN_POINT('',(-1.8,4.5,-5.73)) ;
#104430=CARTESIAN_POINT('Origin',(0.549999999999999,4.5,-4.53)) ;
#104431=CARTESIAN_POINT('',(-1.7,0.3,-4.53)) ;
#104432=CARTESIAN_POINT('',(-1.7,4.4,-4.53)) ;
#104433=CARTESIAN_POINT('',(-1.7,4.5,-4.53)) ;
#104434=CARTESIAN_POINT('',(0.45,4.4,-4.53)) ;
#104435=CARTESIAN_POINT('',(0.45,4.4,-4.53)) ;
#104436=CARTESIAN_POINT('',(0.45,0.3,-4.53)) ;
#104437=CARTESIAN_POINT('',(0.45,4.5,-4.53)) ;
#104438=CARTESIAN_POINT('',(0.549999999999999,0.3,-4.53)) ;
#104439=CARTESIAN_POINT('Origin',(0.549999999999999,4.5,-5.63)) ;
#104440=CARTESIAN_POINT('',(0.45,0.3,-5.63)) ;
#104441=CARTESIAN_POINT('',(0.45,4.4,-5.63)) ;
#104442=CARTESIAN_POINT('',(0.45,4.5,-5.63)) ;
#104443=CARTESIAN_POINT('',(-1.7,4.4,-5.63)) ;
#104444=CARTESIAN_POINT('',(-1.7,4.4,-5.63)) ;
#104445=CARTESIAN_POINT('',(-1.7,0.3,-5.63)) ;
#104446=CARTESIAN_POINT('',(-1.7,0.2,-5.63)) ;
#104447=CARTESIAN_POINT('',(0.549999999999999,0.3,-5.63)) ;
#104448=CARTESIAN_POINT('Origin',(0.549999999999999,4.5,-5.63)) ;
#104449=CARTESIAN_POINT('',(-1.7,4.5,-4.63)) ;
#104450=CARTESIAN_POINT('',(-1.7,4.5,-5.53)) ;
#104451=CARTESIAN_POINT('',(-1.7,4.5,-5.63)) ;
#104452=CARTESIAN_POINT('',(0.45,4.5,-5.53)) ;
#104453=CARTESIAN_POINT('',(0.45,4.5,-5.53)) ;
#104454=CARTESIAN_POINT('',(0.45,4.5,-4.63)) ;
#104455=CARTESIAN_POINT('',(0.45,4.5,-5.63)) ;
#104456=CARTESIAN_POINT('',(-1.7,4.5,-4.63)) ;
#104457=CARTESIAN_POINT('Origin',(0.55,3.09772049281573E-17,-5.08)) ;
#104458=CARTESIAN_POINT('',(0.55,2.61224989991992,-5.48)) ;
#104459=CARTESIAN_POINT('',(0.55,2.65280931275608,-5.53)) ;
#104460=CARTESIAN_POINT('Ctrl Pts',(0.55,2.61224989991992,-5.48)) ;
#104461=CARTESIAN_POINT('Ctrl Pts',(0.55,2.61224989991992,-5.48386974416198)) ;
#104462=CARTESIAN_POINT('Ctrl Pts',(0.55,2.61317624258758,-5.48842010391569)) ;
#104463=CARTESIAN_POINT('Ctrl Pts',(0.55,2.61634258087509,-5.49663300085887)) ;
#104464=CARTESIAN_POINT('Ctrl Pts',(0.55,2.61951410407877,-5.50163042864529)) ;
#104465=CARTESIAN_POINT('Ctrl Pts',(0.55,2.63040394024853,-5.51493871907015)) ;
#104466=CARTESIAN_POINT('Ctrl Pts',(0.55,2.64148366881061,-5.52317058096742)) ;
#104467=CARTESIAN_POINT('Ctrl Pts',(0.55,2.65280931275608,-5.53)) ;
#104468=CARTESIAN_POINT('',(0.55,0.3,-5.53)) ;
#104469=CARTESIAN_POINT('',(0.55,1.39397422176708E-16,-5.53)) ;
#104470=CARTESIAN_POINT('',(0.55,0.3,-4.63)) ;
#104471=CARTESIAN_POINT('',(0.55,0.3,-4.53)) ;
#104472=CARTESIAN_POINT('',(0.55,2.65280931275594,-4.63000000000009)) ;
#104473=CARTESIAN_POINT('',(0.55,6.35032701027224E-17,-4.63)) ;
#104474=CARTESIAN_POINT('',(0.55,2.61224989991992,-4.68)) ;
#104475=CARTESIAN_POINT('Ctrl Pts',(0.55,2.65280931275594,-4.63000000000009)) ;
#104476=CARTESIAN_POINT('Ctrl Pts',(0.55,2.64148366881051,-4.63682941903265)) ;
#104477=CARTESIAN_POINT('Ctrl Pts',(0.55,2.6304039402485,-4.64506128092989)) ;
#104478=CARTESIAN_POINT('Ctrl Pts',(0.55,2.61951410407877,-4.6583695713547)) ;
#104479=CARTESIAN_POINT('Ctrl Pts',(0.55,2.61634258087509,-4.66336699914112)) ;
#104480=CARTESIAN_POINT('Ctrl Pts',(0.55,2.61317624258758,-4.67157989608431)) ;
#104481=CARTESIAN_POINT('Ctrl Pts',(0.55,2.61224989991992,-4.67613025583802)) ;
#104482=CARTESIAN_POINT('Ctrl Pts',(0.55,2.61224989991992,-4.68)) ;
#104483=CARTESIAN_POINT('',(0.55,2.61224989991992,-4.58)) ;
#104484=CARTESIAN_POINT('Origin',(0.,0.2,-5.08)) ;
#104485=CARTESIAN_POINT('',(-1.7,0.2,-5.73)) ;
#104486=CARTESIAN_POINT('',(-1.7,0.2,-6.48)) ;
#104487=CARTESIAN_POINT('',(-1.7,0.2,-6.58)) ;
#104488=CARTESIAN_POINT('',(0.899999999999999,0.2,-6.48)) ;
#104489=CARTESIAN_POINT('',(0.999999999999999,0.2,-6.48)) ;
#104490=CARTESIAN_POINT('',(0.899999999999999,0.2,-3.68)) ;
#104491=CARTESIAN_POINT('',(0.899999999999999,0.2,-3.58)) ;
#104492=CARTESIAN_POINT('',(-1.7,0.2,-3.68)) ;
#104493=CARTESIAN_POINT('',(-1.8,0.2,-3.68)) ;
#104494=CARTESIAN_POINT('',(-1.7,0.2,-4.43)) ;
#104495=CARTESIAN_POINT('',(-1.7,0.2,-4.53)) ;
#104496=CARTESIAN_POINT('',(0.65,0.2,-4.43)) ;
#104497=CARTESIAN_POINT('',(-1.16429916652874E-32,0.2,-4.43)) ;
#104498=CARTESIAN_POINT('',(0.65,0.2,-5.73)) ;
#104499=CARTESIAN_POINT('',(0.65,0.2,-5.63)) ;
#104500=CARTESIAN_POINT('',(-1.35834902761687E-32,0.2,-5.73)) ;
#104501=CARTESIAN_POINT('Origin',(3.,2.3,-7.62)) ;
#104502=CARTESIAN_POINT('',(3.,4.2,-4.58)) ;
#104503=CARTESIAN_POINT('',(3.,3.4,-4.58)) ;
#104504=CARTESIAN_POINT('',(3.,2.3,-4.58)) ;
#104505=CARTESIAN_POINT('',(3.,4.3,-4.68)) ;
#104506=CARTESIAN_POINT('Origin',(3.,4.2,-4.68)) ;
#104507=CARTESIAN_POINT('',(3.,4.3,-5.48)) ;
#104508=CARTESIAN_POINT('',(3.,4.3,-7.62)) ;
#104509=CARTESIAN_POINT('',(3.,4.2,-5.58)) ;
#104510=CARTESIAN_POINT('Origin',(3.,4.2,-5.48)) ;
#104511=CARTESIAN_POINT('',(3.,3.4,-5.58)) ;
#104512=CARTESIAN_POINT('',(3.,2.3,-5.58)) ;
#104513=CARTESIAN_POINT('',(3.,3.3,-5.48)) ;
#104514=CARTESIAN_POINT('Origin',(3.,3.4,-5.48)) ;
#104515=CARTESIAN_POINT('',(3.,3.3,-4.68)) ;
#104516=CARTESIAN_POINT('',(3.,3.3,-7.62)) ;
#104517=CARTESIAN_POINT('Origin',(3.,3.4,-4.68)) ;
#104518=CARTESIAN_POINT('Origin',(-1.,3.8,-5.08)) ;
#104519=CARTESIAN_POINT('',(-1.,1.6,-7.04214168703487)) ;
#104520=CARTESIAN_POINT('',(-1.,1.55483870967742,-6.91555190077455)) ;
#104521=CARTESIAN_POINT('Origin',(-1.,1.40000000000001,-7.04214168703487)) ;
#104522=CARTESIAN_POINT('',(-1.,1.6,-7.62)) ;
#104523=CARTESIAN_POINT('',(-1.,2.95,-6.7231676725155)) ;
#104524=CARTESIAN_POINT('',(-1.,2.95,-5.08)) ;
#104525=CARTESIAN_POINT('',(-1.,2.1568323274845,-5.93)) ;
#104526=CARTESIAN_POINT('Origin',(-1.,3.8,-5.08)) ;
#104527=CARTESIAN_POINT('',(-1.,1.02736587339765,-5.93)) ;
#104528=CARTESIAN_POINT('',(-1.,3.8,-5.93)) ;
#104529=CARTESIAN_POINT('Origin',(-1.,3.8,-5.08)) ;
#104530=CARTESIAN_POINT('Origin',(-1.,3.05,-7.63)) ;
#104531=CARTESIAN_POINT('',(1.15,3.05,-6.7231676725155)) ;
#104532=CARTESIAN_POINT('',(1.15,3.05,-6.66113883008419)) ;
#104533=CARTESIAN_POINT('',(-0.900000000000002,3.05,-6.7231676725155)) ;
#104534=CARTESIAN_POINT('',(-1.,3.05,-6.7231676725155)) ;
#104535=CARTESIAN_POINT('',(-0.900000000000002,3.05,-7.63)) ;
#104536=CARTESIAN_POINT('Origin',(-1.,2.21886116991581,-5.83)) ;
#104537=CARTESIAN_POINT('',(-0.900000000000002,2.1568323274845,-5.83)) ;
#104538=CARTESIAN_POINT('',(1.15,2.1568323274845,-5.83)) ;
#104539=CARTESIAN_POINT('',(1.25,2.1568323274845,-5.83)) ;
#104540=CARTESIAN_POINT('',(1.15,0.895262490344437,-5.83)) ;
#104541=CARTESIAN_POINT('',(-0.900000000000002,2.21886116991581,-5.83)) ;
#104542=CARTESIAN_POINT('Origin',(-1.,3.8,-5.08)) ;
#104543=CARTESIAN_POINT('',(-0.900000000000002,2.24565220167453,-5.88405405405406)) ;
#104544=CARTESIAN_POINT('',(-0.900000000000001,2.99594594594595,-6.63434779832547)) ;
#104545=CARTESIAN_POINT('Origin',(-0.900000000000001,3.8,-5.08)) ;
#104546=CARTESIAN_POINT('',(1.15,2.99594594594595,-6.63434779832547)) ;
#104547=CARTESIAN_POINT('',(-1.,2.99594594594595,-6.63434779832547)) ;
#104548=CARTESIAN_POINT('',(1.15,2.24565220167453,-5.88405405405406)) ;
#104549=CARTESIAN_POINT('Origin',(1.15,3.8,-5.08)) ;
#104550=CARTESIAN_POINT('',(-1.,2.24565220167453,-5.88405405405406)) ;
#104551=CARTESIAN_POINT('Origin',(-1.,3.8,-5.08)) ;
#104552=CARTESIAN_POINT('',(-0.900000000000002,2.99594594594594,-3.52565220167453)) ;
#104553=CARTESIAN_POINT('',(-0.900000000000002,2.24565220167453,-4.27594594594595)) ;
#104554=CARTESIAN_POINT('Origin',(-0.900000000000001,3.8,-5.08)) ;
#104555=CARTESIAN_POINT('',(1.15,2.24565220167453,-4.27594594594595)) ;
#104556=CARTESIAN_POINT('',(-1.,2.24565220167453,-4.27594594594595)) ;
#104557=CARTESIAN_POINT('',(1.15,2.99594594594594,-3.52565220167453)) ;
#104558=CARTESIAN_POINT('Origin',(1.15,3.8,-5.08)) ;
#104559=CARTESIAN_POINT('',(-1.,2.99594594594594,-3.52565220167453)) ;
#104560=CARTESIAN_POINT('Origin',(-1.,2.21886116991581,-4.33)) ;
#104561=CARTESIAN_POINT('',(1.15,2.1568323274845,-4.33)) ;
#104562=CARTESIAN_POINT('',(1.15,2.21886116991581,-4.33)) ;
#104563=CARTESIAN_POINT('',(-0.900000000000002,2.1568323274845,-4.33)) ;
#104564=CARTESIAN_POINT('',(-1.,2.1568323274845,-4.33)) ;
#104565=CARTESIAN_POINT('',(-0.900000000000002,0.895262490344437,-4.33)) ;
#104566=CARTESIAN_POINT('Origin',(-1.,3.05,-2.53)) ;
#104567=CARTESIAN_POINT('',(-0.900000000000002,3.05,-3.4368323274845)) ;
#104568=CARTESIAN_POINT('',(1.15,3.05,-3.4368323274845)) ;
#104569=CARTESIAN_POINT('',(1.25,3.05,-3.4368323274845)) ;
#104570=CARTESIAN_POINT('',(1.15,3.05,-2.54)) ;
#104571=CARTESIAN_POINT('',(-0.900000000000002,3.05,-3.49886116991581)) ;
#104572=CARTESIAN_POINT('Origin',(-1.,3.8,-5.08)) ;
#104573=CARTESIAN_POINT('',(-1.,2.1568323274845,-4.23)) ;
#104574=CARTESIAN_POINT('',(-1.,2.95,-3.4368323274845)) ;
#104575=CARTESIAN_POINT('Origin',(-1.,3.8,-5.08)) ;
#104576=CARTESIAN_POINT('',(-1.,2.95,-2.54)) ;
#104577=CARTESIAN_POINT('',(-1.,1.6,-3.11785831296514)) ;
#104578=CARTESIAN_POINT('',(-1.,1.6,-5.08)) ;
#104579=CARTESIAN_POINT('',(-1.,1.55483870967743,-3.24444809922545)) ;
#104580=CARTESIAN_POINT('Origin',(-1.,1.40000000000001,-3.11785831296514)) ;
#104581=CARTESIAN_POINT('',(-1.,1.02736587339765,-4.23)) ;
#104582=CARTESIAN_POINT('Origin',(-1.,3.8,-5.08)) ;
#104583=CARTESIAN_POINT('',(-1.,2.21886116991581,-4.23)) ;
#104584=CARTESIAN_POINT('Origin',(-1.,3.8,-5.08)) ;
#104585=CARTESIAN_POINT('',(-1.,5.4431676725155,-5.93)) ;
#104586=CARTESIAN_POINT('',(-1.,4.65,-6.7231676725155)) ;
#104587=CARTESIAN_POINT('Origin',(-1.,3.8,-5.08)) ;
#104588=CARTESIAN_POINT('',(-1.,4.65,-5.08)) ;
#104589=CARTESIAN_POINT('',(-1.,6.45,-5.93)) ;
#104590=CARTESIAN_POINT('',(-1.,6.45,-5.83)) ;
#104591=CARTESIAN_POINT('',(-1.,3.8,-5.93)) ;
#104592=CARTESIAN_POINT('Origin',(-1.,4.55,-6.66113883008419)) ;
#104593=CARTESIAN_POINT('',(-0.900000000000001,4.55,-6.7231676725155)) ;
#104594=CARTESIAN_POINT('',(1.15,4.55,-6.7231676725155)) ;
#104595=CARTESIAN_POINT('',(1.25,4.55,-6.7231676725155)) ;
#104596=CARTESIAN_POINT('',(1.15,4.55,-7.62)) ;
#104597=CARTESIAN_POINT('',(-0.900000000000001,4.55,-6.66113883008419)) ;
#104598=CARTESIAN_POINT('Origin',(-1.,3.8,-5.08)) ;
#104599=CARTESIAN_POINT('',(-0.900000000000001,4.60405405405406,-6.63434779832547)) ;
#104600=CARTESIAN_POINT('',(-0.900000000000001,5.35434779832547,-5.88405405405405)) ;
#104601=CARTESIAN_POINT('Origin',(-0.900000000000001,3.8,-5.08)) ;
#104602=CARTESIAN_POINT('',(1.15,5.35434779832547,-5.88405405405406)) ;
#104603=CARTESIAN_POINT('',(-1.,5.35434779832547,-5.88405405405406)) ;
#104604=CARTESIAN_POINT('',(1.15,4.60405405405405,-6.63434779832547)) ;
#104605=CARTESIAN_POINT('Origin',(1.15,3.8,-5.08)) ;
#104606=CARTESIAN_POINT('',(-1.,4.60405405405406,-6.63434779832547)) ;
#104607=CARTESIAN_POINT('Origin',(-1.,6.55,-5.83)) ;
#104608=CARTESIAN_POINT('',(-0.900000000000001,5.4431676725155,-5.83)) ;
#104609=CARTESIAN_POINT('',(-0.9,6.45,-5.83)) ;
#104610=CARTESIAN_POINT('',(-0.9,6.55,-5.83)) ;
#104611=CARTESIAN_POINT('',(1.15,6.45,-5.83)) ;
#104612=CARTESIAN_POINT('',(-1.,6.45,-5.83)) ;
#104613=CARTESIAN_POINT('',(1.15,5.4431676725155,-5.83)) ;
#104614=CARTESIAN_POINT('',(1.15,5.38113883008419,-5.83)) ;
#104615=CARTESIAN_POINT('',(-1.,5.4431676725155,-5.83)) ;
#104616=CARTESIAN_POINT('Origin',(-1.,3.8,-5.08)) ;
#104617=CARTESIAN_POINT('',(-0.900000000000001,5.35434779832547,-4.27594594594594)) ;
#104618=CARTESIAN_POINT('',(-0.900000000000001,4.60405405405405,-3.52565220167453)) ;
#104619=CARTESIAN_POINT('Origin',(-0.900000000000001,3.8,-5.08)) ;
#104620=CARTESIAN_POINT('',(1.15,4.60405405405405,-3.52565220167453)) ;
#104621=CARTESIAN_POINT('',(-1.,4.60405405405405,-3.52565220167453)) ;
#104622=CARTESIAN_POINT('',(1.15,5.35434779832547,-4.27594594594594)) ;
#104623=CARTESIAN_POINT('Origin',(1.15,3.8,-5.08)) ;
#104624=CARTESIAN_POINT('',(-1.,5.35434779832547,-4.27594594594594)) ;
#104625=CARTESIAN_POINT('Origin',(-1.,4.55,-3.49886116991581)) ;
#104626=CARTESIAN_POINT('',(1.15,4.55,-3.4368323274845)) ;
#104627=CARTESIAN_POINT('',(1.15,4.55,-3.49886116991581)) ;
#104628=CARTESIAN_POINT('',(-0.900000000000001,4.55,-3.4368323274845)) ;
#104629=CARTESIAN_POINT('',(-1.,4.55,-3.4368323274845)) ;
#104630=CARTESIAN_POINT('',(-0.900000000000001,4.55,-2.54)) ;
#104631=CARTESIAN_POINT('Origin',(-1.,6.55,-4.33)) ;
#104632=CARTESIAN_POINT('',(1.15,5.4431676725155,-4.33)) ;
#104633=CARTESIAN_POINT('',(1.15,6.45,-4.33)) ;
#104634=CARTESIAN_POINT('',(1.15,6.55,-4.33)) ;
#104635=CARTESIAN_POINT('',(-0.9,6.45,-4.33)) ;
#104636=CARTESIAN_POINT('',(-1.,6.45,-4.33)) ;
#104637=CARTESIAN_POINT('',(-0.900000000000001,5.4431676725155,-4.33)) ;
#104638=CARTESIAN_POINT('',(-0.900000000000001,5.38113883008419,-4.33)) ;
#104639=CARTESIAN_POINT('',(1.25,5.4431676725155,-4.33)) ;
#104640=CARTESIAN_POINT('Origin',(-1.,3.8,-5.08)) ;
#104641=CARTESIAN_POINT('',(-1.,5.4431676725155,-4.23)) ;
#104642=CARTESIAN_POINT('',(-1.,6.45,-4.23)) ;
#104643=CARTESIAN_POINT('',(-1.,6.55,-4.23)) ;
#104644=CARTESIAN_POINT('',(-1.,6.45,-5.08)) ;
#104645=CARTESIAN_POINT('',(-1.,4.65,-3.4368323274845)) ;
#104646=CARTESIAN_POINT('',(-1.,4.65,-3.49886116991581)) ;
#104647=CARTESIAN_POINT('Origin',(-1.,3.8,-5.08)) ;
#104648=CARTESIAN_POINT('Origin',(10.,4.35421736843756,-5.955)) ;
#104649=CARTESIAN_POINT('',(9.91643989873054,7.72792407799439,-5.94107331645509)) ;
#104650=CARTESIAN_POINT('',(8.58356010126947,8.17221734381475,-5.71892668354491)) ;
#104651=CARTESIAN_POINT('',(8.47075240319158,8.20981990984071,-5.70012540053193)) ;
#104652=CARTESIAN_POINT('',(8.58356010126947,6.66256607592813,-5.71892668354491)) ;
#104653=CARTESIAN_POINT('',(8.58356010126947,6.64863939238321,-5.71892668354491)) ;
#104654=CARTESIAN_POINT('',(9.91643989873054,6.8847127088383,-5.94107331645509)) ;
#104655=CARTESIAN_POINT('',(9.98442535909739,6.89604361889945,-5.95240422651623)) ;
#104656=CARTESIAN_POINT('',(9.91643989873054,7.8,-5.94107331645509)) ;
#104657=CARTESIAN_POINT('Origin',(8.5,4.35421736843756,-5.705)) ;
#104658=CARTESIAN_POINT('',(8.5,8.17221734381475,-5.6202872911617)) ;
#104659=CARTESIAN_POINT('',(8.50000000129681,8.20000000266558,-5.62210562535302)) ;
#104660=CARTESIAN_POINT('Origin',(8.5,8.17870774541385,-5.8090376393979)) ;
#104661=CARTESIAN_POINT('',(8.5,8.2,-4.49634544369909)) ;
#104662=CARTESIAN_POINT('',(8.5,6.66256607592813,-4.5397127088383)) ;
#104663=CARTESIAN_POINT('',(8.5,6.64863939238321,-4.5397127088383)) ;
#104664=CARTESIAN_POINT('',(8.50000000002143,6.64999999935441,-4.53931784432623)) ;
#104665=CARTESIAN_POINT('Origin',(8.5,6.65811550100372,-4.34318848269215)) ;
#104666=CARTESIAN_POINT('',(8.49999999999933,6.65000073218972,-5.62068969096366)) ;
#104667=CARTESIAN_POINT('',(8.5,6.65,-5.80363939238321)) ;
#104668=CARTESIAN_POINT('',(8.5,6.66256607592813,-5.6202872911617)) ;
#104669=CARTESIAN_POINT('Origin',(8.5,6.65133313742082,-5.81701007179561)) ;
#104670=CARTESIAN_POINT('',(8.5,8.20007071090457,-5.6202872911617)) ;
#104671=CARTESIAN_POINT('Origin',(8.5,4.35421736843756,-4.455)) ;
#104672=CARTESIAN_POINT('',(9.91643989873054,6.8847127088383,-4.21892668354491)) ;
#104673=CARTESIAN_POINT('',(8.58356010126947,6.66256607592813,-4.44107331645509)) ;
#104674=CARTESIAN_POINT('',(8.48442535909739,6.64604361889945,-4.45759577348377)) ;
#104675=CARTESIAN_POINT('',(8.58356010126947,8.20007071090456,-4.44107331645509)) ;
#104676=CARTESIAN_POINT('',(9.91643989873054,7.72792407799439,-4.21892668354491)) ;
#104677=CARTESIAN_POINT('',(9.97075240319158,7.70981990984071,-4.20987459946807)) ;
#104678=CARTESIAN_POINT('',(9.91643989873054,6.8,-4.21892668354491)) ;
#104679=CARTESIAN_POINT('Origin',(8.5,3.65,-4.58)) ;
#104680=CARTESIAN_POINT('',(8.45734623443633,3.62014236410543,-4.98206555615734)) ;
#104681=CARTESIAN_POINT('',(8.02582401135442,3.3180768079481,-4.68)) ;
#104682=CARTESIAN_POINT('',(8.34729988159781,3.54310991711847,-4.90503310917037)) ;
#104683=CARTESIAN_POINT('',(8.02582401135442,3.31807680794809,-5.48)) ;
#104684=CARTESIAN_POINT('',(8.02582401135442,3.3180768079481,-4.58)) ;
#104685=CARTESIAN_POINT('',(8.45734623443633,3.62014236410543,-5.17793444384266)) ;
#104686=CARTESIAN_POINT('',(8.70083523513316,3.79058466459322,-5.00749214335488)) ;
#104687=CARTESIAN_POINT('',(8.45734623443633,3.62014236410543,-4.58)) ;
#104688=CARTESIAN_POINT('Origin',(8.5,3.95,-4.58)) ;
#104689=CARTESIAN_POINT('',(8.5,3.89793444384266,-5.17793444384266)) ;
#104690=CARTESIAN_POINT('',(8.5,3.89793444384266,-4.98206555615734)) ;
#104691=CARTESIAN_POINT('',(8.5,3.89793444384266,-4.58)) ;
#104692=CARTESIAN_POINT('',(8.5,3.70206555615734,-4.98206555615734)) ;
#104693=CARTESIAN_POINT('',(8.5,3.95,-4.98206555615734)) ;
#104694=CARTESIAN_POINT('',(8.5,3.70206555615734,-5.17793444384266)) ;
#104695=CARTESIAN_POINT('',(8.5,3.70206555615734,-4.58)) ;
#104696=CARTESIAN_POINT('',(8.5,3.95,-5.17793444384266)) ;
#104697=CARTESIAN_POINT('Origin',(8.,4.3,-4.58)) ;
#104698=CARTESIAN_POINT('',(8.45734623443633,3.97985763589457,-5.17793444384266)) ;
#104699=CARTESIAN_POINT('',(8.02582401135442,4.2819231920519,-5.48)) ;
#104700=CARTESIAN_POINT('',(8.32457260887054,4.07279917379062,-5.27087598173872)) ;
#104701=CARTESIAN_POINT('',(8.02582401135442,4.2819231920519,-4.68)) ;
#104702=CARTESIAN_POINT('',(8.02582401135442,4.2819231920519,-4.58)) ;
#104703=CARTESIAN_POINT('',(8.45734623443633,3.97985763589457,-4.98206555615734)) ;
#104704=CARTESIAN_POINT('',(7.97103725533518,4.32027392126537,-4.64164927078653)) ;
#104705=CARTESIAN_POINT('',(8.45734623443633,3.97985763589457,-4.58)) ;
#104706=CARTESIAN_POINT('Origin',(1.5,2.3,-4.58)) ;
#104707=CARTESIAN_POINT('',(7.96847777691809,3.4,-4.58)) ;
#104708=CARTESIAN_POINT('',(8.,3.4,-4.58)) ;
#104709=CARTESIAN_POINT('',(7.96847777691809,4.2,-4.58)) ;
#104710=CARTESIAN_POINT('',(7.96847777691809,4.2,-4.58)) ;
#104711=CARTESIAN_POINT('',(3.,4.2,-4.58)) ;
#104712=CARTESIAN_POINT('Origin',(1.5,2.3,-5.58)) ;
#104713=CARTESIAN_POINT('',(7.96847777691809,4.2,-5.58)) ;
#104714=CARTESIAN_POINT('',(1.5,4.2,-5.58)) ;
#104715=CARTESIAN_POINT('',(7.96847777691809,3.4,-5.58)) ;
#104716=CARTESIAN_POINT('',(7.96847777691809,2.3,-5.58)) ;
#104717=CARTESIAN_POINT('',(1.5,3.4,-5.58)) ;
#104718=CARTESIAN_POINT('Origin',(8.,3.3,-4.58)) ;
#104719=CARTESIAN_POINT('',(7.96847777691809,3.3,-5.48)) ;
#104720=CARTESIAN_POINT('',(8.,3.3,-5.48)) ;
#104721=CARTESIAN_POINT('',(7.96847777691809,3.3,-4.68)) ;
#104722=CARTESIAN_POINT('',(7.96847777691809,3.3,-4.58)) ;
#104723=CARTESIAN_POINT('',(3.,3.3,-4.68)) ;
#104724=CARTESIAN_POINT('Origin',(1.5,4.3,-4.58)) ;
#104725=CARTESIAN_POINT('',(7.96847777691809,4.3,-4.68)) ;
#104726=CARTESIAN_POINT('',(8.,4.3,-4.68)) ;
#104727=CARTESIAN_POINT('',(7.96847777691809,4.3,-5.48)) ;
#104728=CARTESIAN_POINT('',(7.96847777691809,4.3,-4.58)) ;
#104729=CARTESIAN_POINT('',(1.5,4.3,-5.48)) ;
#104730=CARTESIAN_POINT('Origin',(1.5,2.3,-4.58)) ;
#104731=CARTESIAN_POINT('',(-0.4,2.3,-4.58)) ;
#104732=CARTESIAN_POINT('',(-0.4,-3.36847777691809,-4.58)) ;
#104733=CARTESIAN_POINT('',(-0.4,-3.4,-4.58)) ;
#104734=CARTESIAN_POINT('',(0.4,-3.36847777691809,-4.58)) ;
#104735=CARTESIAN_POINT('',(0.4,-3.36847777691809,-4.58)) ;
#104736=CARTESIAN_POINT('',(0.4,2.29999999999999,-4.58)) ;
#104737=CARTESIAN_POINT('',(0.4,2.29999999999999,-4.58)) ;
#104738=CARTESIAN_POINT('',(0.536602540378444,2.83090991212703,-4.58)) ;
#104739=CARTESIAN_POINT('Origin',(1.5,2.3,-4.58)) ;
#104740=CARTESIAN_POINT('',(0.536602540378444,3.93764017256378,-4.58)) ;
#104741=CARTESIAN_POINT('',(0.536602540378444,2.83090991212703,-4.58)) ;
#104742=CARTESIAN_POINT('Origin',(1.5,2.3,-4.58)) ;
#104743=CARTESIAN_POINT('Origin',(1.5,2.3,-5.58)) ;
#104744=CARTESIAN_POINT('',(0.4,2.29999999999999,-5.58)) ;
#104745=CARTESIAN_POINT('',(0.4,-3.36847777691809,-5.58)) ;
#104746=CARTESIAN_POINT('',(0.4,2.3,-5.58)) ;
#104747=CARTESIAN_POINT('',(-0.4,-3.36847777691809,-5.58)) ;
#104748=CARTESIAN_POINT('',(1.5,-3.36847777691809,-5.58)) ;
#104749=CARTESIAN_POINT('',(-0.4,2.3,-5.58)) ;
#104750=CARTESIAN_POINT('',(-0.4,2.3,-5.58)) ;
#104751=CARTESIAN_POINT('',(0.536602540378444,3.93764017256378,-5.58)) ;
#104752=CARTESIAN_POINT('Origin',(1.5,2.3,-5.58)) ;
#104753=CARTESIAN_POINT('',(0.536602540378444,2.83090991212703,-5.58)) ;
#104754=CARTESIAN_POINT('',(0.536602540378444,3.93764017256378,-5.58)) ;
#104755=CARTESIAN_POINT('Origin',(1.5,2.3,-5.58)) ;
#104756=CARTESIAN_POINT('Origin',(1.5,2.3,-4.58)) ;
#104757=CARTESIAN_POINT('',(-0.5,2.3,-4.68)) ;
#104758=CARTESIAN_POINT('',(-0.5,2.3,-5.48)) ;
#104759=CARTESIAN_POINT('',(-0.5,2.3,-4.58)) ;
#104760=CARTESIAN_POINT('Origin',(1.5,2.3,-4.68)) ;
#104761=CARTESIAN_POINT('Origin',(1.5,2.3,-5.48)) ;
#104762=CARTESIAN_POINT('Origin',(-0.5,-3.4,-4.58)) ;
#104763=CARTESIAN_POINT('',(-0.5,-3.36847777691809,-5.48)) ;
#104764=CARTESIAN_POINT('',(-0.5,-3.4,-5.48)) ;
#104765=CARTESIAN_POINT('',(-0.5,-3.36847777691809,-4.68)) ;
#104766=CARTESIAN_POINT('',(-0.5,-3.36847777691809,-4.58)) ;
#104767=CARTESIAN_POINT('',(-0.5,2.3,-4.68)) ;
#104768=CARTESIAN_POINT('Origin',(-0.15,-3.9,-4.58)) ;
#104769=CARTESIAN_POINT('',(-0.179857635894567,-3.85734623443633,-4.98206555615734)) ;
#104770=CARTESIAN_POINT('',(-0.481923192051905,-3.42582401135442,-4.68)) ;
#104771=CARTESIAN_POINT('',(-0.256890082881532,-3.74729988159781,-4.90503310917037)) ;
#104772=CARTESIAN_POINT('',(-0.481923192051905,-3.42582401135442,-5.48)) ;
#104773=CARTESIAN_POINT('',(-0.481923192051905,-3.42582401135442,-4.58)) ;
#104774=CARTESIAN_POINT('',(-0.179857635894567,-3.85734623443633,-5.17793444384266)) ;
#104775=CARTESIAN_POINT('',(-0.00941533540678435,-4.10083523513317,-5.00749214335488)) ;
#104776=CARTESIAN_POINT('',(-0.179857635894567,-3.85734623443633,-4.58)) ;
#104777=CARTESIAN_POINT('Origin',(0.15,-3.9,-4.58)) ;
#104778=CARTESIAN_POINT('',(0.0979344438426627,-3.9,-5.17793444384266)) ;
#104779=CARTESIAN_POINT('',(0.0979344438426627,-3.9,-4.98206555615734)) ;
#104780=CARTESIAN_POINT('',(0.0979344438426627,-3.9,-4.58)) ;
#104781=CARTESIAN_POINT('',(-0.0979344438426628,-3.9,-4.98206555615734)) ;
#104782=CARTESIAN_POINT('',(0.15,-3.9,-4.98206555615734)) ;
#104783=CARTESIAN_POINT('',(-0.0979344438426628,-3.9,-5.17793444384266)) ;
#104784=CARTESIAN_POINT('',(-0.0979344438426628,-3.9,-4.58)) ;
#104785=CARTESIAN_POINT('',(0.15,-3.9,-5.17793444384266)) ;
#104786=CARTESIAN_POINT('Origin',(0.5,-3.4,-4.58)) ;
#104787=CARTESIAN_POINT('',(0.179857635894567,-3.85734623443633,-5.17793444384266)) ;
#104788=CARTESIAN_POINT('',(0.481923192051904,-3.42582401135442,-5.48)) ;
#104789=CARTESIAN_POINT('',(0.272799173790623,-3.72457260887054,-5.27087598173872)) ;
#104790=CARTESIAN_POINT('',(0.481923192051904,-3.42582401135442,-4.68)) ;
#104791=CARTESIAN_POINT('',(0.481923192051904,-3.42582401135442,-4.58)) ;
#104792=CARTESIAN_POINT('',(0.179857635894567,-3.85734623443633,-4.98206555615734)) ;
#104793=CARTESIAN_POINT('',(0.520273921265371,-3.37103725533519,-4.64164927078653)) ;
#104794=CARTESIAN_POINT('',(0.179857635894567,-3.85734623443633,-4.58)) ;
#104795=CARTESIAN_POINT('Origin',(0.5,2.29999999999999,-4.58)) ;
#104796=CARTESIAN_POINT('',(0.500000000000001,2.29999999999999,-4.68)) ;
#104797=CARTESIAN_POINT('',(0.5,-3.36847777691809,-4.68)) ;
#104798=CARTESIAN_POINT('',(0.5,-3.4,-4.68)) ;
#104799=CARTESIAN_POINT('',(0.5,-3.36847777691809,-5.48)) ;
#104800=CARTESIAN_POINT('',(0.5,-3.36847777691809,-4.58)) ;
#104801=CARTESIAN_POINT('',(0.500000000000001,2.29999999999999,-5.48)) ;
#104802=CARTESIAN_POINT('',(0.5,2.29999999999999,-5.48)) ;
#104803=CARTESIAN_POINT('',(0.500000000000001,2.29999999999999,-4.58)) ;
#104804=CARTESIAN_POINT('Origin',(1.5,2.3,-4.58)) ;
#104805=CARTESIAN_POINT('Origin',(1.5,2.3,-4.68)) ;
#104806=CARTESIAN_POINT('Origin',(1.5,2.3,-5.48)) ;
#104807=CARTESIAN_POINT('Origin',(8.,2.68967221921331,-5.58)) ;
#104808=CARTESIAN_POINT('',(8.45734623443633,3.70206555615734,-5.25985763589457)) ;
#104809=CARTESIAN_POINT('',(8.02582401135442,3.4,-5.5619231920519)) ;
#104810=CARTESIAN_POINT('',(7.75526480758232,3.21060855735952,-5.75131463469238)) ;
#104811=CARTESIAN_POINT('',(8.02582401135442,4.2,-5.5619231920519)) ;
#104812=CARTESIAN_POINT('',(8.02582401135442,2.68967221921331,-5.5619231920519)) ;
#104813=CARTESIAN_POINT('',(8.45734623443633,3.89793444384266,-5.25985763589457)) ;
#104814=CARTESIAN_POINT('',(8.54034505662341,3.83983526831171,-5.20175846036362)) ;
#104815=CARTESIAN_POINT('',(8.45734623443633,2.68967221921331,-5.25985763589457)) ;
#104816=CARTESIAN_POINT('Origin',(8.,2.68967221921331,-4.58)) ;
#104817=CARTESIAN_POINT('',(8.45734623443633,3.89793444384266,-4.90014236410543)) ;
#104818=CARTESIAN_POINT('',(8.02582401135442,4.2,-4.5980768079481)) ;
#104819=CARTESIAN_POINT('',(8.54034505662341,3.83983526831171,-4.95824153963639)) ;
#104820=CARTESIAN_POINT('',(8.02582401135442,3.4,-4.5980768079481)) ;
#104821=CARTESIAN_POINT('',(8.02582401135442,3.4,-4.5980768079481)) ;
#104822=CARTESIAN_POINT('',(8.45734623443633,3.70206555615734,-4.90014236410543)) ;
#104823=CARTESIAN_POINT('',(7.75526480758232,3.21060855735952,-4.40868536530762)) ;
#104824=CARTESIAN_POINT('',(8.45734623443633,2.68967221921331,-4.90014236410543)) ;
#104825=CARTESIAN_POINT('Origin',(-1.11032778078669,-3.9,-4.93)) ;
#104826=CARTESIAN_POINT('',(0.0979344438426626,-3.85734623443633,-4.90014236410543)) ;
#104827=CARTESIAN_POINT('',(0.4,-3.42582401135442,-4.5980768079481)) ;
#104828=CARTESIAN_POINT('',(-0.223548570072128,-4.31660768288603,-5.22162537802022)) ;
#104829=CARTESIAN_POINT('',(-0.400000000000001,-3.42582401135442,-4.5980768079481)) ;
#104830=CARTESIAN_POINT('',(-0.400000000000001,-3.42582401135442,-4.5980768079481)) ;
#104831=CARTESIAN_POINT('',(-0.0979344438426627,-3.85734623443633,-4.90014236410543)) ;
#104832=CARTESIAN_POINT('',(-0.326007604256636,-3.53152743384494,-4.67206920369146)) ;
#104833=CARTESIAN_POINT('',(-1.11032778078669,-3.85734623443633,-4.90014236410543)) ;
#104834=CARTESIAN_POINT('Origin',(-1.11032778078669,-3.4,-5.58)) ;
#104835=CARTESIAN_POINT('',(-0.0979344438426627,-3.85734623443633,-5.25985763589457)) ;
#104836=CARTESIAN_POINT('',(-0.4,-3.42582401135442,-5.5619231920519)) ;
#104837=CARTESIAN_POINT('',(-0.589391442640475,-3.15526480758232,-5.75131463469238)) ;
#104838=CARTESIAN_POINT('',(0.400000000000001,-3.42582401135442,-5.5619231920519)) ;
#104839=CARTESIAN_POINT('',(-1.11032778078669,-3.42582401135442,-5.5619231920519)) ;
#104840=CARTESIAN_POINT('',(0.0979344438426626,-3.85734623443633,-5.25985763589457)) ;
#104841=CARTESIAN_POINT('',(0.0398352683117103,-3.94034505662341,-5.20175846036361)) ;
#104842=CARTESIAN_POINT('',(-1.11032778078669,-3.85734623443633,-5.25985763589457)) ;
#104843=CARTESIAN_POINT('Origin',(10.,1.24999999999998,-7.62)) ;
#104844=CARTESIAN_POINT('',(9.91643989873054,1.26392668354489,-3.0358381198218)) ;
#104845=CARTESIAN_POINT('',(9.91643989873054,1.26392668354489,-7.62)) ;
#104846=CARTESIAN_POINT('',(8.50816364570057,1.49863939238321,-3.11785831296514)) ;
#104847=CARTESIAN_POINT('Origin',(43.7052916416609,-4.36754860786629,-611.768201693183)) ;
#104848=CARTESIAN_POINT('',(8.50816364570057,1.49863939238321,-7.62)) ;
#104849=CARTESIAN_POINT('Origin',(8.49999999999985,3.8,-5.08)) ;
#104850=CARTESIAN_POINT('',(9.91643989873053,1.24322097942674,-3.09630356419405)) ;
#104851=CARTESIAN_POINT('',(9.91643989873053,1.24322097942648,-7.06369643580562)) ;
#104852=CARTESIAN_POINT('Origin',(9.91643989873053,3.8,-5.08)) ;
#104853=CARTESIAN_POINT('Origin',(36.5480653059678,-40.380261828241,567.197654967682)) ;
#104854=CARTESIAN_POINT('Origin',(36.5480653017837,-40.3802618313523,-577.357654913403)) ;
#104855=CARTESIAN_POINT('Origin',(10.,1.24999999999998,-7.62)) ;
#104856=CARTESIAN_POINT('',(8.50816364570059,1.49863939238321,-7.04214168703472)) ;
#104857=CARTESIAN_POINT('',(8.50816364570057,1.49863939238321,-7.62)) ;
#104858=CARTESIAN_POINT('',(9.91643989873054,1.26392668354489,-7.12416188017819)) ;
#104859=CARTESIAN_POINT('Origin',(43.7052916530562,-4.3675486096968,601.608201900582)) ;
#104860=CARTESIAN_POINT('',(9.91643989873054,1.26392668354489,-7.62)) ;
#104861=CARTESIAN_POINT('Origin',(-0.900000000000001,4.65,-5.08)) ;
#104862=CARTESIAN_POINT('Origin',(-0.900000000000001,4.65,-3.4368323274845)) ;
#104863=CARTESIAN_POINT('Origin',(-0.900000000000001,4.65,-3.4368323274845)) ;
#104864=CARTESIAN_POINT('Origin',(-0.900000000000001,4.65,-3.4368323274845)) ;
#104865=CARTESIAN_POINT('Origin',(-0.900000000000001,4.65,-3.4368323274845)) ;
#104866=CARTESIAN_POINT('Origin',(1.15,4.45,-3.49886116991581)) ;
#104867=CARTESIAN_POINT('Origin',(1.15,4.45,-3.4368323274845)) ;
#104868=CARTESIAN_POINT('Origin',(-1.,4.65,-3.4368323274845)) ;
#104869=CARTESIAN_POINT('Origin',(1.15,4.65,-3.4368323274845)) ;
#104870=CARTESIAN_POINT('Origin',(-0.900000000000001,3.8,-5.08)) ;
#104871=CARTESIAN_POINT('Origin',(-0.900000000000001,5.4431676725155,-4.23)) ;
#104872=CARTESIAN_POINT('Origin',(1.15,4.65,-3.4368323274845)) ;
#104873=CARTESIAN_POINT('Origin',(1.15,4.55810810810811,-3.61447207586456)) ;
#104874=CARTESIAN_POINT('Origin',(-0.900000000000001,5.4431676725155,-4.23)) ;
#104875=CARTESIAN_POINT('Origin',(-0.900000000000001,5.4431676725155,-4.23)) ;
#104876=CARTESIAN_POINT('Origin',(-0.900000000000001,5.4431676725155,-4.23)) ;
#104877=CARTESIAN_POINT('Origin',(-0.900000000000001,4.65,-5.08)) ;
#104878=CARTESIAN_POINT('Origin',(-0.900000000000001,4.65,-6.7231676725155)) ;
#104879=CARTESIAN_POINT('Origin',(-1.,4.65,-6.7231676725155)) ;
#104880=CARTESIAN_POINT('Origin',(1.15,4.65,-6.7231676725155)) ;
#104881=CARTESIAN_POINT('Origin',(-0.900000000000001,4.65,-6.7231676725155)) ;
#104882=CARTESIAN_POINT('Origin',(1.15,4.45,-6.66113883008419)) ;
#104883=CARTESIAN_POINT('Origin',(1.15,4.45,-6.7231676725155)) ;
#104884=CARTESIAN_POINT('Origin',(1.15,3.8,-5.08)) ;
#104885=CARTESIAN_POINT('Origin',(1.15,5.26552792413544,-4.32189189189189)) ;
#104886=CARTESIAN_POINT('Origin',(-1.,5.4431676725155,-4.23)) ;
#104887=CARTESIAN_POINT('Origin',(1.15,5.4431676725155,-4.23)) ;
#104888=CARTESIAN_POINT('Origin',(-0.900000000000001,3.8,-4.23)) ;
#104889=CARTESIAN_POINT('Origin',(-0.9,6.45,-4.23)) ;
#104890=CARTESIAN_POINT('Origin',(-0.9,6.45,-5.08)) ;
#104891=CARTESIAN_POINT('Origin',(-0.9,6.45,-4.23)) ;
#104892=CARTESIAN_POINT('Origin',(-0.900000000000001,4.65,-6.7231676725155)) ;
#104893=CARTESIAN_POINT('Origin',(-0.900000000000001,4.65,-6.7231676725155)) ;
#104894=CARTESIAN_POINT('Origin',(1.15,4.65,-6.7231676725155)) ;
#104895=CARTESIAN_POINT('Origin',(1.15,4.55810810810811,-6.54552792413544)) ;
#104896=CARTESIAN_POINT('Origin',(1.15,5.4431676725155,-4.23)) ;
#104897=CARTESIAN_POINT('Origin',(1.15,5.4431676725155,-4.43)) ;
#104898=CARTESIAN_POINT('Origin',(-0.9,6.45,-4.23)) ;
#104899=CARTESIAN_POINT('Origin',(-0.9,6.45,-4.23)) ;
#104900=CARTESIAN_POINT('Origin',(-0.900000000000001,3.8,-5.08)) ;
#104901=CARTESIAN_POINT('Origin',(-0.900000000000001,5.4431676725155,-5.93)) ;
#104902=CARTESIAN_POINT('Origin',(-1.,5.4431676725155,-5.93)) ;
#104903=CARTESIAN_POINT('Origin',(1.15,5.4431676725155,-5.93)) ;
#104904=CARTESIAN_POINT('Origin',(-0.900000000000001,5.4431676725155,-5.93)) ;
#104905=CARTESIAN_POINT('Origin',(1.15,3.8,-5.08)) ;
#104906=CARTESIAN_POINT('Origin',(1.15,5.26552792413544,-5.83810810810811)) ;
#104907=CARTESIAN_POINT('Origin',(1.15,6.55,-4.43)) ;
#104908=CARTESIAN_POINT('Origin',(1.15,6.45,-4.43)) ;
#104909=CARTESIAN_POINT('Origin',(1.25,6.45,-4.23)) ;
#104910=CARTESIAN_POINT('Origin',(1.15,6.45,-4.23)) ;
#104911=CARTESIAN_POINT('Origin',(-0.900000000000001,5.4431676725155,-5.93)) ;
#104912=CARTESIAN_POINT('Origin',(-0.900000000000001,5.4431676725155,-5.93)) ;
#104913=CARTESIAN_POINT('Origin',(1.15,5.4431676725155,-5.93)) ;
#104914=CARTESIAN_POINT('Origin',(1.15,5.4431676725155,-5.73)) ;
#104915=CARTESIAN_POINT('Origin',(1.15,6.45,-4.43)) ;
#104916=CARTESIAN_POINT('Origin',(1.35,6.45,-4.43)) ;
#104917=CARTESIAN_POINT('Origin',(-0.9,6.45,-5.08)) ;
#104918=CARTESIAN_POINT('Origin',(-0.9,6.45,-5.93)) ;
#104919=CARTESIAN_POINT('Origin',(-0.900000000000001,3.8,-5.93)) ;
#104920=CARTESIAN_POINT('Origin',(-0.9,6.45,-5.93)) ;
#104921=CARTESIAN_POINT('Origin',(1.15,6.55,-5.73)) ;
#104922=CARTESIAN_POINT('Origin',(1.15,6.45,-5.73)) ;
#104923=CARTESIAN_POINT('Origin',(1.35,6.45,-7.62)) ;
#104924=CARTESIAN_POINT('Origin',(1.35,6.45,-5.73)) ;
#104925=CARTESIAN_POINT('Origin',(-0.9,6.45,-5.93)) ;
#104926=CARTESIAN_POINT('Origin',(-0.9,6.45,-5.93)) ;
#104927=CARTESIAN_POINT('Origin',(1.15,6.45,-5.73)) ;
#104928=CARTESIAN_POINT('Origin',(1.15,6.45,-5.93)) ;
#104929=CARTESIAN_POINT('Origin',(-1.,6.45,-5.93)) ;
#104930=CARTESIAN_POINT('Origin',(-1.7,0.3,-5.73)) ;
#104931=CARTESIAN_POINT('Origin',(-1.7,0.3,-5.73)) ;
#104932=CARTESIAN_POINT('Origin',(-1.7,0.3,-5.73)) ;
#104933=CARTESIAN_POINT('Origin',(-1.7,0.3,-5.73)) ;
#104934=CARTESIAN_POINT('Origin',(0.549999999999999,0.3,-5.73)) ;
#104935=CARTESIAN_POINT('',(0.50857864376269,0.229289321881345,-5.65928932188135)) ;
#104936=CARTESIAN_POINT('Ctrl Pts',(0.65,0.2,-5.73)) ;
#104937=CARTESIAN_POINT('Ctrl Pts',(0.639834283464151,0.2,-5.72491714173208)) ;
#104938=CARTESIAN_POINT('Ctrl Pts',(0.629316849080535,0.200389688120422,
-5.71965768385801)) ;
#104939=CARTESIAN_POINT('Ctrl Pts',(0.606957334719669,0.202165884217645,
-5.70846794971935)) ;
#104940=CARTESIAN_POINT('Ctrl Pts',(0.595086727401099,0.203647820493442,
-5.70252276179493)) ;
#104941=CARTESIAN_POINT('Ctrl Pts',(0.572283837380409,0.207685608831265,
-5.691106760396)) ;
#104942=CARTESIAN_POINT('Ctrl Pts',(0.561337481650365,0.21017819324834,
-5.68562986130802)) ;
#104943=CARTESIAN_POINT('Ctrl Pts',(0.549549942885299,0.213544620665569,
-5.6797406960393)) ;
#104944=CARTESIAN_POINT('Ctrl Pts',(0.548290718945592,0.213913346522002,
-5.67911168276603)) ;
#104945=CARTESIAN_POINT('Ctrl Pts',(0.536119229732643,0.217566912232546,
-5.67303275135176)) ;
#104946=CARTESIAN_POINT('Ctrl Pts',(0.525706917362398,0.221400308602611,
-5.66784223842911)) ;
#104947=CARTESIAN_POINT('Ctrl Pts',(0.513545110027183,0.226871185484688,
-5.6617711869643)) ;
#104948=CARTESIAN_POINT('Ctrl Pts',(0.511029334128283,0.22806397669855,
-5.66051466706414)) ;
#104949=CARTESIAN_POINT('Ctrl Pts',(0.50857864376269,0.229289321881343,
-5.65928932188135)) ;
#104950=CARTESIAN_POINT('Origin',(0.664280054301624,0.302990743362135,-5.73714210424988)) ;
#104951=CARTESIAN_POINT('Origin',(-1.7,4.5,-5.73)) ;
#104952=CARTESIAN_POINT('',(-1.77071067811863,4.45857864376274,-5.65928932188132)) ;
#104953=CARTESIAN_POINT('Origin',(-1.69703459697506,4.61417009505288,-5.73708668538063)) ;
#104954=CARTESIAN_POINT('Ctrl Pts',(-1.77071067811863,4.45857864376274,
-5.65928932188132)) ;
#104955=CARTESIAN_POINT('Ctrl Pts',(-1.77521675558366,4.46759079869281,
-5.66379539934635)) ;
#104956=CARTESIAN_POINT('Ctrl Pts',(-1.77928079264422,4.47748625817296,
-5.66872648167164)) ;
#104957=CARTESIAN_POINT('Ctrl Pts',(-1.78624680748626,4.49811277056884,
-5.6790208825478)) ;
#104958=CARTESIAN_POINT('Ctrl Pts',(-1.78918030781792,4.50880509433485,
-5.68436398414911)) ;
#104959=CARTESIAN_POINT('Ctrl Pts',(-1.79185985500292,4.52101859322041,
-5.69047475453283)) ;
#104960=CARTESIAN_POINT('Ctrl Pts',(-1.79213045061227,4.52228751722709,
-5.69110970990894)) ;
#104961=CARTESIAN_POINT('Ctrl Pts',(-1.79477467909828,4.53504937002863,
-5.69749628913391)) ;
#104962=CARTESIAN_POINT('Ctrl Pts',(-1.79657370273651,4.54677936428202,
-5.70337157240614)) ;
#104963=CARTESIAN_POINT('Ctrl Pts',(-1.79896007643135,4.56920025888388,
-5.71459577476113)) ;
#104964=CARTESIAN_POINT('Ctrl Pts',(-1.79963010255187,4.57990192168148,
-5.71995007594496)) ;
#104965=CARTESIAN_POINT('Ctrl Pts',(-1.79996164986962,4.59357116034292,
-5.726785573817)) ;
#104966=CARTESIAN_POINT('Ctrl Pts',(-1.8,4.59680282631912,-5.72840141315956)) ;
#104967=CARTESIAN_POINT('Ctrl Pts',(-1.8,4.6,-5.73)) ;
#104968=CARTESIAN_POINT('Origin',(-1.7,0.3,-5.08)) ;
#104969=CARTESIAN_POINT('Origin',(-1.7,0.3,-6.48)) ;
#104970=CARTESIAN_POINT('Origin',(0.65,0.3,-5.08)) ;
#104971=CARTESIAN_POINT('',(0.579289321881328,0.229289321881363,-5.58857864376273)) ;
#104972=CARTESIAN_POINT('Origin',(0.657086685378504,0.302965403023971,-5.74417009504855)) ;
#104973=CARTESIAN_POINT('Ctrl Pts',(0.579289321881328,0.229289321881363,
-5.58857864376273)) ;
#104974=CARTESIAN_POINT('Ctrl Pts',(0.583795399346357,0.224783244416332,
-5.59759079869279)) ;
#104975=CARTESIAN_POINT('Ctrl Pts',(0.588726481671639,0.220719207355779,
-5.60748625817292)) ;
#104976=CARTESIAN_POINT('Ctrl Pts',(0.599020882547819,0.213753192513722,
-5.62811277056884)) ;
#104977=CARTESIAN_POINT('Ctrl Pts',(0.604363984149159,0.210819692182048,
-5.6388050943349)) ;
#104978=CARTESIAN_POINT('Ctrl Pts',(0.610474754532884,0.20814014499706,
-5.65101859322046)) ;
#104979=CARTESIAN_POINT('Ctrl Pts',(0.611109709908967,0.207869549387718,
-5.65228751722709)) ;
#104980=CARTESIAN_POINT('Ctrl Pts',(0.617496289133925,0.205225320901714,
-5.6650493700286)) ;
#104981=CARTESIAN_POINT('Ctrl Pts',(0.62337157240616,0.203426297263481,
-5.67677936428201)) ;
#104982=CARTESIAN_POINT('Ctrl Pts',(0.634595774761163,0.201039923568647,
-5.69920025888391)) ;
#104983=CARTESIAN_POINT('Ctrl Pts',(0.639950075944988,0.200369897448124,
-5.70990192168153)) ;
#104984=CARTESIAN_POINT('Ctrl Pts',(0.646785573817023,0.200038350130376,
-5.72357116034297)) ;
#104985=CARTESIAN_POINT('Ctrl Pts',(0.648401413159571,0.2,-5.72680282631915)) ;
#104986=CARTESIAN_POINT('Ctrl Pts',(0.65,0.2,-5.73)) ;
#104987=CARTESIAN_POINT('',(0.579289321881328,0.229289321881363,-4.57142135623727)) ;
#104988=CARTESIAN_POINT('Ctrl Pts',(0.65,0.2,-4.43)) ;
#104989=CARTESIAN_POINT('Ctrl Pts',(0.644917141732079,0.2,-4.44016571653583)) ;
#104990=CARTESIAN_POINT('Ctrl Pts',(0.639657683858008,0.200389688120423,
-4.45068315091942)) ;
#104991=CARTESIAN_POINT('Ctrl Pts',(0.628467949719361,0.202165884217643,
-4.47304266528023)) ;
#104992=CARTESIAN_POINT('Ctrl Pts',(0.622522761794958,0.203647820493435,
-4.48491327259876)) ;
#104993=CARTESIAN_POINT('Ctrl Pts',(0.611106760396026,0.207685608831252,
-4.50771616261944)) ;
#104994=CARTESIAN_POINT('Ctrl Pts',(0.60562986130804,0.21017819324833,-4.51866251834951)) ;
#104995=CARTESIAN_POINT('Ctrl Pts',(0.59974069603932,0.213544620665559,
-4.53045005711458)) ;
#104996=CARTESIAN_POINT('Ctrl Pts',(0.599111682766055,0.213913346521986,
-4.53170928105426)) ;
#104997=CARTESIAN_POINT('Ctrl Pts',(0.593032751351781,0.217566912232528,
-4.54388077026722)) ;
#104998=CARTESIAN_POINT('Ctrl Pts',(0.587842238429123,0.221400308602595,
-4.55429308263749)) ;
#104999=CARTESIAN_POINT('Ctrl Pts',(0.581771186964295,0.226871185484688,
-4.56645488997275)) ;
#105000=CARTESIAN_POINT('Ctrl Pts',(0.580514667064132,0.228063976698558,
-4.56897066587167)) ;
#105001=CARTESIAN_POINT('Ctrl Pts',(0.579289321881328,0.229289321881363,
-4.57142135623728)) ;
#105002=CARTESIAN_POINT('Origin',(0.657142104246849,0.302990743360512,-4.41571994570428)) ;
#105003=CARTESIAN_POINT('Origin',(-1.7,4.6,-5.63)) ;
#105004=CARTESIAN_POINT('',(-1.77071067811866,4.52928932188135,-5.58857864376269)) ;
#105005=CARTESIAN_POINT('Ctrl Pts',(-1.8,4.6,-5.73)) ;
#105006=CARTESIAN_POINT('Ctrl Pts',(-1.8,4.59491714173209,-5.71983428346416)) ;
#105007=CARTESIAN_POINT('Ctrl Pts',(-1.79961031187958,4.58965768385802,
-5.70931684908055)) ;
#105008=CARTESIAN_POINT('Ctrl Pts',(-1.79783411578236,4.57846794971937,
-5.68695733471969)) ;
#105009=CARTESIAN_POINT('Ctrl Pts',(-1.79635217950657,4.57252276179496,
-5.67508672740113)) ;
#105010=CARTESIAN_POINT('Ctrl Pts',(-1.79231439116882,4.56110676039622,
-5.65228383738084)) ;
#105011=CARTESIAN_POINT('Ctrl Pts',(-1.78982180675185,4.55562986130843,
-5.64133748165119)) ;
#105012=CARTESIAN_POINT('Ctrl Pts',(-1.78645537933466,4.54974069603969,
-5.62954994288609)) ;
#105013=CARTESIAN_POINT('Ctrl Pts',(-1.78608665347812,4.54911168276623,
-5.628290718946)) ;
#105014=CARTESIAN_POINT('Ctrl Pts',(-1.78243308776746,4.54303275135176,
-5.61611922973268)) ;
#105015=CARTESIAN_POINT('Ctrl Pts',(-1.7785996913974,4.53784223842911,-5.60570691736243)) ;
#105016=CARTESIAN_POINT('Ctrl Pts',(-1.77312881451532,4.5317711869643,-5.5935451100272)) ;
#105017=CARTESIAN_POINT('Ctrl Pts',(-1.77193602330145,4.53051466706415,
-5.59102933412829)) ;
#105018=CARTESIAN_POINT('Ctrl Pts',(-1.77071067811866,4.52928932188135,
-5.58857864376269)) ;
#105019=CARTESIAN_POINT('Origin',(-1.6970092566394,4.60714210424635,-5.74428005429455)) ;
#105020=CARTESIAN_POINT('',(-1.77071067811866,4.52928932188135,-4.57142135623731)) ;
#105021=CARTESIAN_POINT('Origin',(-1.69703459697486,4.6070866853807,-4.41582990494723)) ;
#105022=CARTESIAN_POINT('Ctrl Pts',(-1.77071067811866,4.52928932188135,
-4.57142135623731)) ;
#105023=CARTESIAN_POINT('Ctrl Pts',(-1.77521675558368,4.53379539934637,
-4.56240920130726)) ;
#105024=CARTESIAN_POINT('Ctrl Pts',(-1.77928079264423,4.53872648167164,
-4.55251374182714)) ;
#105025=CARTESIAN_POINT('Ctrl Pts',(-1.78624680748632,4.54902088254787,
-4.53188722943115)) ;
#105026=CARTESIAN_POINT('Ctrl Pts',(-1.78918030781801,4.55436398414927,
-4.52119490566499)) ;
#105027=CARTESIAN_POINT('Ctrl Pts',(-1.79185985500299,4.560474754533,-4.50898140677941)) ;
#105028=CARTESIAN_POINT('Ctrl Pts',(-1.79213045061231,4.56110970990904,
-4.50771248277287)) ;
#105029=CARTESIAN_POINT('Ctrl Pts',(-1.7947746790983,4.56749628913397,-4.49495062997143)) ;
#105030=CARTESIAN_POINT('Ctrl Pts',(-1.79657370273653,4.57337157240621,
-4.483220635718)) ;
#105031=CARTESIAN_POINT('Ctrl Pts',(-1.79896007643136,4.58459577476122,
-4.46079974111606)) ;
#105032=CARTESIAN_POINT('Ctrl Pts',(-1.79963010255188,4.58995007594504,
-4.45009807831843)) ;
#105033=CARTESIAN_POINT('Ctrl Pts',(-1.79996164986962,4.59678557381705,
-4.436428839657)) ;
#105034=CARTESIAN_POINT('Ctrl Pts',(-1.8,4.59840141315958,-4.43319717368084)) ;
#105035=CARTESIAN_POINT('Ctrl Pts',(-1.8,4.6,-4.43)) ;
#105036=CARTESIAN_POINT('Origin',(-1.7,0.3,-6.48)) ;
#105037=CARTESIAN_POINT('Origin',(-1.7,0.1,-6.48)) ;
#105038=CARTESIAN_POINT('Origin',(-1.9,0.3,-6.48)) ;
#105039=CARTESIAN_POINT('Origin',(1.9668402209837E-32,0.1,-6.48)) ;
#105040=CARTESIAN_POINT('',(0.899999999999999,0.1,-6.58)) ;
#105041=CARTESIAN_POINT('',(-1.8,0.1,-6.58)) ;
#105042=CARTESIAN_POINT('Origin',(0.899999999999999,0.1,-6.48)) ;
#105043=CARTESIAN_POINT('Origin',(0.899999999999999,0.1,-6.48)) ;
#105044=CARTESIAN_POINT('',(0.999999999999999,0.1,-6.48)) ;
#105045=CARTESIAN_POINT('Origin',(0.899999999999999,0.1,-6.48)) ;
#105046=CARTESIAN_POINT('Origin',(0.899999999999999,0.1,-6.48)) ;
#105047=CARTESIAN_POINT('Origin',(0.549999999999999,0.3,-4.43)) ;
#105048=CARTESIAN_POINT('',(0.508578643762691,0.229289321881345,-4.50071067811866)) ;
#105049=CARTESIAN_POINT('Origin',(0.664170095058604,0.302965403026464,-4.42291331461641)) ;
#105050=CARTESIAN_POINT('Ctrl Pts',(0.50857864376269,0.229289321881348,
-4.50071067811866)) ;
#105051=CARTESIAN_POINT('Ctrl Pts',(0.517590798692739,0.224783244416321,
-4.49620460065363)) ;
#105052=CARTESIAN_POINT('Ctrl Pts',(0.527486258172858,0.220719207355774,
-4.49127351832835)) ;
#105053=CARTESIAN_POINT('Ctrl Pts',(0.548112770568679,0.213753192513746,
-4.48097911745222)) ;
#105054=CARTESIAN_POINT('Ctrl Pts',(0.558805094334662,0.210819692182089,
-4.47563601585092)) ;
#105055=CARTESIAN_POINT('Ctrl Pts',(0.571018593220227,0.20814014499709,
-4.46952524546719)) ;
#105056=CARTESIAN_POINT('Ctrl Pts',(0.572287517226953,0.207869549387729,
-4.46889029009106)) ;
#105057=CARTESIAN_POINT('Ctrl Pts',(0.585049370028579,0.205225320901701,
-4.46250371086604)) ;
#105058=CARTESIAN_POINT('Ctrl Pts',(0.59677936428202,0.203426297263468,
-4.45662842759379)) ;
#105059=CARTESIAN_POINT('Ctrl Pts',(0.619200258883963,0.201039923568638,
-4.44540422523878)) ;
#105060=CARTESIAN_POINT('Ctrl Pts',(0.62990192168159,0.20036989744812,-4.44004992405496)) ;
#105061=CARTESIAN_POINT('Ctrl Pts',(0.64357116034301,0.200038350130375,
-4.43321442618295)) ;
#105062=CARTESIAN_POINT('Ctrl Pts',(0.646802826319169,0.2,-4.43159858684041)) ;
#105063=CARTESIAN_POINT('Ctrl Pts',(0.65,0.2,-4.43)) ;
#105064=CARTESIAN_POINT('Origin',(-1.7,0.3,-4.43)) ;
#105065=CARTESIAN_POINT('Origin',(-1.7,4.5,-4.43)) ;
#105066=CARTESIAN_POINT('',(-1.77071067811863,4.45857864376274,-4.50071067811868)) ;
#105067=CARTESIAN_POINT('Ctrl Pts',(-1.8,4.6,-4.43)) ;
#105068=CARTESIAN_POINT('Ctrl Pts',(-1.8,4.58983428346418,-4.43508285826792)) ;
#105069=CARTESIAN_POINT('Ctrl Pts',(-1.79961031187958,4.5793168490806,-4.44034231614199)) ;
#105070=CARTESIAN_POINT('Ctrl Pts',(-1.79783411578236,4.55695733471983,
-4.45153205028063)) ;
#105071=CARTESIAN_POINT('Ctrl Pts',(-1.79635217950657,4.54508672740132,
-4.45747723820502)) ;
#105072=CARTESIAN_POINT('Ctrl Pts',(-1.79231439116875,4.52228383738059,
-4.46889323960399)) ;
#105073=CARTESIAN_POINT('Ctrl Pts',(-1.78982180675165,4.51133748165043,
-4.47437013869202)) ;
#105074=CARTESIAN_POINT('Ctrl Pts',(-1.78645537933441,4.49954994288537,
-4.48025930396073)) ;
#105075=CARTESIAN_POINT('Ctrl Pts',(-1.78608665347801,4.49829071894577,
-4.48088831723395)) ;
#105076=CARTESIAN_POINT('Ctrl Pts',(-1.78243308776749,4.48611922973289,
-4.48696724864819)) ;
#105077=CARTESIAN_POINT('Ctrl Pts',(-1.77859969139742,4.4757069173626,-4.49215776157085)) ;
#105078=CARTESIAN_POINT('Ctrl Pts',(-1.77312881451532,4.46354511002731,
-4.49822881303569)) ;
#105079=CARTESIAN_POINT('Ctrl Pts',(-1.77193602330144,4.46102933412837,
-4.49948533293587)) ;
#105080=CARTESIAN_POINT('Ctrl Pts',(-1.77071067811863,4.45857864376274,
-4.50071067811868)) ;
#105081=CARTESIAN_POINT('Origin',(-1.6970092566383,4.61428005430142,-4.42285789575035)) ;
#105082=CARTESIAN_POINT('Origin',(-1.7,0.3,-4.43)) ;
#105083=CARTESIAN_POINT('Origin',(-1.9,-4.11004745125224E-16,-6.48)) ;
#105084=CARTESIAN_POINT('',(-1.9,6.9,-6.58)) ;
#105085=CARTESIAN_POINT('Origin',(-1.9,6.9,-6.48)) ;
#105086=CARTESIAN_POINT('',(-1.9,7.,-6.58)) ;
#105087=CARTESIAN_POINT('Origin',(-2.,0.1,-6.68)) ;
#105088=CARTESIAN_POINT('Origin',(-1.89999999999995,0.100000000000053,-6.68000000000005)) ;
#105089=CARTESIAN_POINT('Origin',(0.899999999999999,0.1,-6.68)) ;
#105090=CARTESIAN_POINT('Origin',(0.899999999999999,0.1,-6.48)) ;
#105091=CARTESIAN_POINT('Origin',(1.1,0.1,-6.48)) ;
#105092=CARTESIAN_POINT('Origin',(0.899999999999999,0.1,-5.08)) ;
#105093=CARTESIAN_POINT('',(0.999999999999999,0.1,-3.68)) ;
#105094=CARTESIAN_POINT('',(0.999999999999999,0.1,-6.58)) ;
#105095=CARTESIAN_POINT('Origin',(0.899999999999999,0.1,-3.68)) ;
#105096=CARTESIAN_POINT('Origin',(-1.7,0.3,-4.43)) ;
#105097=CARTESIAN_POINT('Origin',(-1.7,0.3,-4.43)) ;
#105098=CARTESIAN_POINT('Origin',(-1.9,6.9,-6.48)) ;
#105099=CARTESIAN_POINT('',(-1.9,7.,-6.48)) ;
#105100=CARTESIAN_POINT('Origin',(-1.9,6.9,-6.48)) ;
#105101=CARTESIAN_POINT('Origin',(-1.9,6.9,-6.48)) ;
#105102=CARTESIAN_POINT('Origin',(-1.9,7.,-6.68)) ;
#105103=CARTESIAN_POINT('Origin',(-1.9,6.9,-6.68)) ;
#105104=CARTESIAN_POINT('Origin',(1.1,0.1,-3.58)) ;
#105105=CARTESIAN_POINT('Origin',(1.1,0.1,-3.68)) ;
#105106=CARTESIAN_POINT('Origin',(0.899999999999999,0.1,-3.68)) ;
#105107=CARTESIAN_POINT('',(0.899999999999999,0.1,-3.58)) ;
#105108=CARTESIAN_POINT('Origin',(0.899999999999999,0.1,-3.68)) ;
#105109=CARTESIAN_POINT('Origin',(0.899999999999999,0.1,-3.68)) ;
#105110=CARTESIAN_POINT('Origin',(-1.7,0.3,-5.08)) ;
#105111=CARTESIAN_POINT('Origin',(-1.7,0.3,-3.68)) ;
#105112=CARTESIAN_POINT('Origin',(-1.9,6.9,-5.08)) ;
#105113=CARTESIAN_POINT('',(-1.9,7.,-3.68)) ;
#105114=CARTESIAN_POINT('Origin',(-1.9,6.9,-3.68)) ;
#105115=CARTESIAN_POINT('',(-1.9,7.,-6.58)) ;
#105116=CARTESIAN_POINT('Origin',(-1.9,6.9,-6.48)) ;
#105117=CARTESIAN_POINT('Origin',(-1.9,7.1,-6.48)) ;
#105118=CARTESIAN_POINT('Origin',(0.899999999999999,0.1,-3.68)) ;
#105119=CARTESIAN_POINT('Origin',(0.899999999999999,0.1,-3.48)) ;
#105120=CARTESIAN_POINT('Origin',(-1.9668402209837E-32,0.1,-3.68)) ;
#105121=CARTESIAN_POINT('',(0.999999999999999,0.1,-3.58)) ;
#105122=CARTESIAN_POINT('Origin',(-1.7,0.1,-3.68)) ;
#105123=CARTESIAN_POINT('Origin',(-1.7,0.3,-3.68)) ;
#105124=CARTESIAN_POINT('Origin',(-1.9,0.3,-3.68)) ;
#105125=CARTESIAN_POINT('Origin',(-1.9,6.9,-3.68)) ;
#105126=CARTESIAN_POINT('',(-1.9,6.9,-3.58)) ;
#105127=CARTESIAN_POINT('Origin',(-1.9,6.9,-3.68)) ;
#105128=CARTESIAN_POINT('Origin',(-1.9,6.9,-3.68)) ;
#105129=CARTESIAN_POINT('Origin',(-1.9,7.1,-6.58)) ;
#105130=CARTESIAN_POINT('Origin',(-1.9,7.1,-3.68)) ;
#105131=CARTESIAN_POINT('Origin',(-1.8,0.1,-3.48)) ;
#105132=CARTESIAN_POINT('Origin',(-1.89999999999997,0.100000000000027,-3.47999999999998)) ;
#105133=CARTESIAN_POINT('Origin',(-1.9,-6.40600499298624E-17,-3.68)) ;
#105134=CARTESIAN_POINT('',(-1.9,7.,-3.58)) ;
#105135=CARTESIAN_POINT('Origin',(-1.9,6.9,-3.68)) ;
#105136=CARTESIAN_POINT('Origin',(-1.9,6.9,-3.48)) ;
#105137=CARTESIAN_POINT('Origin',(-1.9,7.,-3.48)) ;
#105138=CARTESIAN_POINT('Origin',(-0.900000000000002,2.95,-5.08)) ;
#105139=CARTESIAN_POINT('Origin',(-0.900000000000001,2.95,-6.7231676725155)) ;
#105140=CARTESIAN_POINT('Origin',(-0.900000000000002,2.95,-6.7231676725155)) ;
#105141=CARTESIAN_POINT('Origin',(-0.900000000000001,2.95,-6.7231676725155)) ;
#105142=CARTESIAN_POINT('Origin',(-0.900000000000002,2.95,-6.7231676725155)) ;
#105143=CARTESIAN_POINT('Origin',(1.15,3.15,-7.63)) ;
#105144=CARTESIAN_POINT('Origin',(1.15,3.15,-6.7231676725155)) ;
#105145=CARTESIAN_POINT('Origin',(-1.,2.95,-6.7231676725155)) ;
#105146=CARTESIAN_POINT('Origin',(1.15,2.95,-6.7231676725155)) ;
#105147=CARTESIAN_POINT('Origin',(-0.900000000000001,3.8,-5.08)) ;
#105148=CARTESIAN_POINT('Origin',(-0.900000000000002,2.1568323274845,-5.93)) ;
#105149=CARTESIAN_POINT('Origin',(-0.900000000000002,1.6,-5.08)) ;
#105150=CARTESIAN_POINT('Origin',(-0.900000000000002,1.6,-7.04214168703487)) ;
#105151=CARTESIAN_POINT('Origin',(13.9153543900904,1.4,-7.04214168703487)) ;
#105152=CARTESIAN_POINT('Origin',(8.49172374697002,1.4,-7.04214168703487)) ;
#105153=CARTESIAN_POINT('Origin',(-0.900000000000001,1.40000000000001,-7.04214168703487)) ;
#105154=CARTESIAN_POINT('Origin',(1.15,2.95,-6.7231676725155)) ;
#105155=CARTESIAN_POINT('Origin',(1.15,3.04189189189189,-6.54552792413544)) ;
#105156=CARTESIAN_POINT('Origin',(-0.900000000000002,2.1568323274845,-5.93)) ;
#105157=CARTESIAN_POINT('Origin',(-0.900000000000002,2.1568323274845,-5.93)) ;
#105158=CARTESIAN_POINT('Origin',(-0.900000000000002,2.1568323274845,-5.93)) ;
#105159=CARTESIAN_POINT('Origin',(-0.900000000000001,1.40000000000001,-7.04214168703487)) ;
#105160=CARTESIAN_POINT('Origin',(-0.900000000000002,1.55483870967742,-6.91555190077455)) ;
#105161=CARTESIAN_POINT('Origin',(1.15,3.8,-5.08)) ;
#105162=CARTESIAN_POINT('Origin',(1.15,2.33447207586456,-5.83810810810811)) ;
#105163=CARTESIAN_POINT('Origin',(-1.,2.1568323274845,-5.93)) ;
#105164=CARTESIAN_POINT('Origin',(1.15,2.1568323274845,-5.93)) ;
#105165=CARTESIAN_POINT('Origin',(-0.900000000000001,3.8,-5.93)) ;
#105166=CARTESIAN_POINT('Origin',(-0.900000000000002,1.02736587339765,-5.93)) ;
#105167=CARTESIAN_POINT('Origin',(-0.900000000000001,3.8,-5.08)) ;
#105168=CARTESIAN_POINT('Origin',(-0.900000000000002,1.02736587339765,-5.93)) ;
#105169=CARTESIAN_POINT('Origin',(13.9153543900904,1.4,-3.11785831296514)) ;
#105170=CARTESIAN_POINT('Origin',(8.49172374697002,1.4,-3.11785831296514)) ;
#105171=CARTESIAN_POINT('Origin',(-0.900000000000001,1.40000000000001,-3.11785831296514)) ;
#105172=CARTESIAN_POINT('Origin',(-0.900000000000002,1.6,-5.08)) ;
#105173=CARTESIAN_POINT('Origin',(-0.900000000000002,1.6,-3.11785831296514)) ;
#105174=CARTESIAN_POINT('Origin',(-0.900000000000002,2.95,-5.08)) ;
#105175=CARTESIAN_POINT('Origin',(-0.900000000000002,2.95,-3.4368323274845)) ;
#105176=CARTESIAN_POINT('Origin',(1.15,2.1568323274845,-5.93)) ;
#105177=CARTESIAN_POINT('Origin',(1.15,2.1568323274845,-5.73)) ;
#105178=CARTESIAN_POINT('Origin',(-0.900000000000002,1.02736587339765,-5.93)) ;
#105179=CARTESIAN_POINT('Origin',(-0.900000000000001,1.40000000000001,-3.11785831296514)) ;
#105180=CARTESIAN_POINT('Origin',(-0.900000000000002,1.55483870967743,-3.24444809922545)) ;
#105181=CARTESIAN_POINT('Origin',(-0.900000000000002,2.95,-3.4368323274845)) ;
#105182=CARTESIAN_POINT('Origin',(-0.900000000000002,2.95,-3.4368323274845)) ;
#105183=CARTESIAN_POINT('Origin',(-0.900000000000001,2.95,-3.4368323274845)) ;
#105184=CARTESIAN_POINT('Origin',(1.15,2.21886116991581,-5.73)) ;
#105185=CARTESIAN_POINT('Ctrl Pts',(1.15,1.02736587339765,-5.83)) ;
#105186=CARTESIAN_POINT('Ctrl Pts',(1.1608920328805,1.02736587339765,-5.83)) ;
#105187=CARTESIAN_POINT('Ctrl Pts',(1.17195716626105,1.02622125393927,-5.82814384392599)) ;
#105188=CARTESIAN_POINT('Ctrl Pts',(1.1820844490224,1.02414637334385,-5.82471318879084)) ;
#105189=CARTESIAN_POINT('Ctrl Pts',(1.19245005921088,1.02202266415684,-5.82120179934314)) ;
#105190=CARTESIAN_POINT('Ctrl Pts',(1.20216743701154,1.01888103823701,-5.81596019807028)) ;
#105191=CARTESIAN_POINT('Ctrl Pts',(1.21053792402812,1.01518120925307,-5.80959371680205)) ;
#105192=CARTESIAN_POINT('Ctrl Pts',(1.219343173684,1.01128921135341,-5.80289656084385)) ;
#105193=CARTESIAN_POINT('Ctrl Pts',(1.22692289939014,1.00668521903338,-5.79478516153154)) ;
#105194=CARTESIAN_POINT('Ctrl Pts',(1.23290049538659,1.00186003905466,-5.78592412596239)) ;
#105195=CARTESIAN_POINT('Ctrl Pts',(1.23922345568944,0.9967560772818,-5.77655113116998)) ;
#105196=CARTESIAN_POINT('Ctrl Pts',(1.24392209779927,0.991279542094837,
-5.76610455998969)) ;
#105197=CARTESIAN_POINT('Ctrl Pts',(1.24674870216524,0.985895902333124,
-5.75529206652967)) ;
#105198=CARTESIAN_POINT('Ctrl Pts',(1.24889292215336,0.981811953364218,
-5.74708986997272)) ;
#105199=CARTESIAN_POINT('Ctrl Pts',(1.25,0.977715885027402,-5.73854916862923)) ;
#105200=CARTESIAN_POINT('Ctrl Pts',(1.25,0.973783447787483,-5.73)) ;
#105201=CARTESIAN_POINT('Origin',(-0.900000000000001,3.8,-5.08)) ;
#105202=CARTESIAN_POINT('Origin',(-0.900000000000002,1.02736587339765,-4.23)) ;
#105203=CARTESIAN_POINT('Origin',(-0.900000000000001,3.8,-4.23)) ;
#105204=CARTESIAN_POINT('Origin',(-0.900000000000002,2.1568323274845,-4.23)) ;
#105205=CARTESIAN_POINT('Origin',(-0.900000000000002,1.02736587339765,-4.23)) ;
#105206=CARTESIAN_POINT('Origin',(-0.900000000000001,3.8,-5.08)) ;
#105207=CARTESIAN_POINT('Origin',(-0.900000000000002,2.1568323274845,-4.23)) ;
#105208=CARTESIAN_POINT('Origin',(-1.,2.95,-3.4368323274845)) ;
#105209=CARTESIAN_POINT('Origin',(1.15,2.95,-3.4368323274845)) ;
#105210=CARTESIAN_POINT('Origin',(1.15,3.15,-2.53)) ;
#105211=CARTESIAN_POINT('Origin',(1.15,3.15,-3.4368323274845)) ;
#105212=CARTESIAN_POINT('Ctrl Pts',(1.110285585749,0.930383836951459,-5.95499428365807)) ;
#105213=CARTESIAN_POINT('Ctrl Pts',(1.14039000477524,0.892136466137966,
-5.82996971859421)) ;
#105214=CARTESIAN_POINT('Ctrl Pts',(1.13015013463564,1.02610337426259,-5.82785112488281)) ;
#105215=CARTESIAN_POINT('Ctrl Pts',(1.17639690652714,0.935225109827694,
-5.97012573994677)) ;
#105216=CARTESIAN_POINT('Ctrl Pts',(1.15491086542928,0.891146666106776,
-5.82927605040126)) ;
#105217=CARTESIAN_POINT('Ctrl Pts',(1.16319405445818,1.03078047702086,-5.83516487424516)) ;
#105218=CARTESIAN_POINT('Ctrl Pts',(1.24701363206612,0.927145283841818,
-5.94555220382508)) ;
#105219=CARTESIAN_POINT('Ctrl Pts',(1.17759980831448,0.893467326853881,
-5.83263731203129)) ;
#105220=CARTESIAN_POINT('Ctrl Pts',(1.19848758201044,1.02297467453099,-5.82328712255501)) ;
#105221=CARTESIAN_POINT('Ctrl Pts',(1.33816236560061,0.900022463714231,
-5.8498088506149)) ;
#105222=CARTESIAN_POINT('Ctrl Pts',(1.22862786282608,0.888037626604003,
-5.80315396432406)) ;
#105223=CARTESIAN_POINT('Ctrl Pts',(1.24403288504499,0.996768276947733,
-5.77702665941333)) ;
#105224=CARTESIAN_POINT('Ctrl Pts',(1.35959492575603,0.881455895025369,
-5.77853234122901)) ;
#105225=CARTESIAN_POINT('Ctrl Pts',(1.25320519750694,0.880428099081613,
-5.77106493782729)) ;
#105226=CARTESIAN_POINT('Ctrl Pts',(1.25473603279823,0.978811277328813,
-5.74255748715087)) ;
#105227=CARTESIAN_POINT('Ctrl Pts',(1.34615355831622,0.867571605181207,
-5.71279258253342)) ;
#105228=CARTESIAN_POINT('Ctrl Pts',(1.25176090202793,0.87095013062468,-5.72944901705783)) ;
#105229=CARTESIAN_POINT('Ctrl Pts',(1.24801589497572,0.965423101361823,
-5.710869548164)) ;
#105230=CARTESIAN_POINT('Origin',(1.35,0.973783447787483,-5.73)) ;
#105231=CARTESIAN_POINT('Origin',(-0.900000000000002,1.02736587339765,-4.23)) ;
#105232=CARTESIAN_POINT('',(-0.957735026918965,0.969630846478687,-4.28773502691896)) ;
#105233=CARTESIAN_POINT('Origin',(-0.900000000000002,1.02736587339765,-4.23)) ;
#105234=CARTESIAN_POINT('Origin',(-0.900000000000002,2.1568323274845,-4.23)) ;
#105235=CARTESIAN_POINT('Origin',(-0.900000000000002,2.1568323274845,-4.23)) ;
#105236=CARTESIAN_POINT('Origin',(1.15,2.95,-3.4368323274845)) ;
#105237=CARTESIAN_POINT('Origin',(1.15,3.04189189189189,-3.61447207586456)) ;
#105238=CARTESIAN_POINT('Origin',(1.35,3.8,-5.08)) ;
#105239=CARTESIAN_POINT('Origin',(1.35,0.973783447787484,-4.43)) ;
#105240=CARTESIAN_POINT('Origin',(-1.,2.1568323274845,-4.23)) ;
#105241=CARTESIAN_POINT('Origin',(1.15,2.1568323274845,-4.23)) ;
#105242=CARTESIAN_POINT('Origin',(1.15,3.8,-5.08)) ;
#105243=CARTESIAN_POINT('Origin',(1.15,2.33447207586456,-4.32189189189189)) ;
#105244=CARTESIAN_POINT('Ctrl Pts',(1.34754079198594,0.869159571293155,
-4.43974853478553)) ;
#105245=CARTESIAN_POINT('Ctrl Pts',(1.25183398383321,0.87199977042434,-4.4259986517603)) ;
#105246=CARTESIAN_POINT('Ctrl Pts',(1.24871534599026,0.966951450593901,
-4.44553571307355)) ;
#105247=CARTESIAN_POINT('Ctrl Pts',(1.35788971301869,0.882932151572348,
-4.37577742826808)) ;
#105248=CARTESIAN_POINT('Ctrl Pts',(1.2513879651909,0.881019151005419,-4.38648728142376)) ;
#105249=CARTESIAN_POINT('Ctrl Pts',(1.25389076424432,0.980237216252362,
-4.41468863425942)) ;
#105250=CARTESIAN_POINT('Ctrl Pts',(1.33642796493172,0.900551643074782,
-4.30831671896883)) ;
#105251=CARTESIAN_POINT('Ctrl Pts',(1.22773025960899,0.888154519889423,
-4.35630235415234)) ;
#105252=CARTESIAN_POINT('Ctrl Pts',(1.24317203399028,0.997278352451075,
-4.38206445828307)) ;
#105253=CARTESIAN_POINT('Ctrl Pts',(1.24851212064759,0.92667567099975,-4.21611185418655)) ;
#105254=CARTESIAN_POINT('Ctrl Pts',(1.17855408504645,0.893378082604316,
-4.32793584540021)) ;
#105255=CARTESIAN_POINT('Ctrl Pts',(1.19923947710882,1.02252144543594,-4.33751118406066)) ;
#105256=CARTESIAN_POINT('Ctrl Pts',(1.18212686068546,0.934567888698244,
-4.19189225990079)) ;
#105257=CARTESIAN_POINT('Ctrl Pts',(1.15690947476179,0.891342319659344,
-4.33050130223878)) ;
#105258=CARTESIAN_POINT('Ctrl Pts',(1.1660589236879,1.03014681530414,-4.32580412352038)) ;
#105259=CARTESIAN_POINT('Ctrl Pts',(1.11776263740946,0.930888708579174,
-4.20342358191601)) ;
#105260=CARTESIAN_POINT('Ctrl Pts',(1.14197710563588,0.892059806626676,
-4.33008229965564)) ;
#105261=CARTESIAN_POINT('Ctrl Pts',(1.13388624958144,1.02659206201256,-4.33137785610126)) ;
#105262=CARTESIAN_POINT('Ctrl Pts',(1.15,1.02736587339764,-4.33)) ;
#105263=CARTESIAN_POINT('Ctrl Pts',(1.15623005440502,1.02736587339759,-4.32999999999987)) ;
#105264=CARTESIAN_POINT('Ctrl Pts',(1.16249579431471,1.02700282517053,-4.33059086606898)) ;
#105265=CARTESIAN_POINT('Ctrl Pts',(1.16857840195431,1.02630083270769,-4.33174093944667)) ;
#105266=CARTESIAN_POINT('Ctrl Pts',(1.1798885498395,1.02499553092934,-4.33387941372467)) ;
#105267=CARTESIAN_POINT('Ctrl Pts',(1.19084787809767,1.02245621903271,-4.33805069661522)) ;
#105268=CARTESIAN_POINT('Ctrl Pts',(1.20043335385463,1.01914369852331,-4.3436491064379)) ;
#105269=CARTESIAN_POINT('Ctrl Pts',(1.21063893018497,1.01561688548223,-4.34960968682249)) ;
#105270=CARTESIAN_POINT('Ctrl Pts',(1.21965078109605,1.01112191387731,-4.35735485110186)) ;
#105271=CARTESIAN_POINT('Ctrl Pts',(1.226898722009,1.00626683908294,-4.36607358485428)) ;
#105272=CARTESIAN_POINT('Ctrl Pts',(1.23435386869391,1.0012729663137,-4.37504157173658)) ;
#105273=CARTESIAN_POINT('Ctrl Pts',(1.24017476602864,0.995763540409855,
-4.38528702640693)) ;
#105274=CARTESIAN_POINT('Ctrl Pts',(1.24405759382605,0.990267693778535,
-4.39604165723046)) ;
#105275=CARTESIAN_POINT('Ctrl Pts',(1.24795610732226,0.9847496452368,-4.40683973419908)) ;
#105276=CARTESIAN_POINT('Ctrl Pts',(1.25,0.97910634898267,-4.41842794502798)) ;
#105277=CARTESIAN_POINT('Ctrl Pts',(1.25,0.973783447787483,-4.43)) ;
#105278=CARTESIAN_POINT('Origin',(1.15,2.1568323274845,-4.23)) ;
#105279=CARTESIAN_POINT('Origin',(1.15,2.1568323274845,-4.43)) ;
#105280=CARTESIAN_POINT('Origin',(1.15,2.21886116991581,-4.43)) ;
#105281=CARTESIAN_POINT('Origin',(1.5,2.3,-5.48)) ;
#105282=CARTESIAN_POINT('Ctrl Pts',(0.55,4.04473197180486,-5.53)) ;
#105283=CARTESIAN_POINT('Ctrl Pts',(0.55,4.04340510574361,-5.53201839167459)) ;
#105284=CARTESIAN_POINT('Ctrl Pts',(0.549938912488052,4.04197482121868,
-5.53397990935583)) ;
#105285=CARTESIAN_POINT('Ctrl Pts',(0.549362579613729,4.03414945156065,
-5.5437632016969)) ;
#105286=CARTESIAN_POINT('Ctrl Pts',(0.54804065212511,4.02633974827561,-5.5505458262271)) ;
#105287=CARTESIAN_POINT('Ctrl Pts',(0.544205267183641,4.00519499286857,
-5.56468394278881)) ;
#105288=CARTESIAN_POINT('Ctrl Pts',(0.54122133237852,3.9901199563799,-5.57122511544813)) ;
#105289=CARTESIAN_POINT('Ctrl Pts',(0.537814556431591,3.96385893187682,
-5.57793059223995)) ;
#105290=CARTESIAN_POINT('Ctrl Pts',(0.536602540378443,3.95132390702871,
-5.58)) ;
#105291=CARTESIAN_POINT('Ctrl Pts',(0.536602540378443,3.93764017256378,
-5.58)) ;
#105292=CARTESIAN_POINT('Origin',(-0.4,2.3,-5.48)) ;
#105293=CARTESIAN_POINT('Origin',(-0.4,-3.4,-5.48)) ;
#105294=CARTESIAN_POINT('Origin',(-0.4,-3.36847777691809,-5.48)) ;
#105295=CARTESIAN_POINT('Origin',(1.5,2.3,-5.48)) ;
#105296=CARTESIAN_POINT('Ctrl Pts',(0.536602540378443,2.83090991212703,
-5.58)) ;
#105297=CARTESIAN_POINT('Ctrl Pts',(0.536602540378443,2.80627146475523,
-5.58)) ;
#105298=CARTESIAN_POINT('Ctrl Pts',(0.538106903229135,2.77742679387697,
-5.57795279081267)) ;
#105299=CARTESIAN_POINT('Ctrl Pts',(0.545186976568789,2.7115684436341,-5.56208398098024)) ;
#105300=CARTESIAN_POINT('Ctrl Pts',(0.55,2.6828290608274,-5.54810205581407)) ;
#105301=CARTESIAN_POINT('Ctrl Pts',(0.55,2.65280931275608,-5.53)) ;
#105302=CARTESIAN_POINT('Origin',(0.400000000000001,2.29999999999999,-5.48)) ;
#105303=CARTESIAN_POINT('Origin',(0.0725078566451197,-4.04348900069683,
-5.00749214335488)) ;
#105304=CARTESIAN_POINT('Origin',(-0.4,-3.36847777691809,-5.48)) ;
#105305=CARTESIAN_POINT('Origin',(-0.0979344438426628,-3.8,-5.17793444384266)) ;
#105306=CARTESIAN_POINT('Origin',(1.5,2.3,-4.68)) ;
#105307=CARTESIAN_POINT('Ctrl Pts',(0.536602540378443,3.93764017256378,
-4.58)) ;
#105308=CARTESIAN_POINT('Ctrl Pts',(0.536602540378443,3.93925361219655,
-4.58)) ;
#105309=CARTESIAN_POINT('Ctrl Pts',(0.536619300889434,3.94087098263999,
-4.58002899725778)) ;
#105310=CARTESIAN_POINT('Ctrl Pts',(0.536997639747708,3.95938954612073,
-4.58068581289575)) ;
#105311=CARTESIAN_POINT('Ctrl Pts',(0.539142315171053,3.9756712086989,-4.58431206156158)) ;
#105312=CARTESIAN_POINT('Ctrl Pts',(0.544035197036652,4.00535605098083,
-4.59539939166598)) ;
#105313=CARTESIAN_POINT('Ctrl Pts',(0.546989816174412,4.01946236900603,
-4.60356994463497)) ;
#105314=CARTESIAN_POINT('Ctrl Pts',(0.54946306249569,4.035955360074,-4.61854738169713)) ;
#105315=CARTESIAN_POINT('Ctrl Pts',(0.550000000000879,4.04078397701435,
-4.62399442034635)) ;
#105316=CARTESIAN_POINT('Ctrl Pts',(0.549999999999999,4.04473197181449,
-4.63000000001465)) ;
#105317=CARTESIAN_POINT('Origin',(-0.4,2.3,-4.68)) ;
#105318=CARTESIAN_POINT('Origin',(0.4,2.29999999999999,-5.48)) ;
#105319=CARTESIAN_POINT('Origin',(0.4,-3.36847777691809,-5.48)) ;
#105320=CARTESIAN_POINT('Origin',(-0.0979344438426628,-3.8,-5.17793444384266)) ;
#105321=CARTESIAN_POINT('Origin',(-0.0979344438426628,-3.8,-5.17793444384266)) ;
#105322=CARTESIAN_POINT('Origin',(-0.0979344438426627,-3.8,-5.17793444384266)) ;
#105323=CARTESIAN_POINT('Origin',(-0.4,2.3,-4.68)) ;
#105324=CARTESIAN_POINT('Origin',(-0.4,-3.36847777691809,-4.68)) ;
#105325=CARTESIAN_POINT('Origin',(0.190875981738719,-3.6672263744342,-5.27087598173872)) ;
#105326=CARTESIAN_POINT('Origin',(0.400000000000001,-3.36847777691809,-5.48)) ;
#105327=CARTESIAN_POINT('Origin',(0.0979344438426626,-3.8,-5.17793444384266)) ;
#105328=CARTESIAN_POINT('Origin',(0.15,-3.8,-5.17793444384266)) ;
#105329=CARTESIAN_POINT('Origin',(0.0979344438426627,-3.8,-5.17793444384266)) ;
#105330=CARTESIAN_POINT('Origin',(-0.0979344438426628,-3.8,-4.58)) ;
#105331=CARTESIAN_POINT('Origin',(-0.0979344438426628,-3.8,-4.98206555615734)) ;
#105332=CARTESIAN_POINT('Origin',(-0.174966890829628,-3.68995364716148,
-4.90503310917037)) ;
#105333=CARTESIAN_POINT('Origin',(-0.400000000000001,-3.36847777691809,
-4.68)) ;
#105334=CARTESIAN_POINT('Origin',(-0.0979344438426627,-3.8,-4.98206555615734)) ;
#105335=CARTESIAN_POINT('Origin',(0.0979344438426627,-3.8,-5.17793444384266)) ;
#105336=CARTESIAN_POINT('Origin',(0.0979344438426628,-3.8,-5.17793444384266)) ;
#105337=CARTESIAN_POINT('Origin',(-0.0979344438426628,-3.8,-4.98206555615734)) ;
#105338=CARTESIAN_POINT('Origin',(-0.0979344438426628,-3.8,-4.98206555615734)) ;
#105339=CARTESIAN_POINT('Origin',(0.0979344438426627,-3.8,-4.58)) ;
#105340=CARTESIAN_POINT('Origin',(0.0979344438426627,-3.8,-4.98206555615734)) ;
#105341=CARTESIAN_POINT('Origin',(-1.11032778078669,-3.8,-4.98206555615734)) ;
#105342=CARTESIAN_POINT('Origin',(0.0979344438426626,-3.8,-4.98206555615734)) ;
#105343=CARTESIAN_POINT('Origin',(0.0979344438426627,-3.8,-4.98206555615734)) ;
#105344=CARTESIAN_POINT('Origin',(0.0979344438426627,-3.8,-4.98206555615734)) ;
#105345=CARTESIAN_POINT('Origin',(0.438350729213467,-3.31369102089885,-4.64164927078653)) ;
#105346=CARTESIAN_POINT('Origin',(0.399999999999999,-3.36847777691809,-4.68)) ;
#105347=CARTESIAN_POINT('Origin',(0.4,2.3,-4.68)) ;
#105348=CARTESIAN_POINT('Origin',(0.4,-3.36847777691809,-4.68)) ;
#105349=CARTESIAN_POINT('Origin',(0.4,2.29999999999999,-4.68)) ;
#105350=CARTESIAN_POINT('Origin',(1.5,2.3,-4.68)) ;
#105351=CARTESIAN_POINT('Ctrl Pts',(0.55,2.65280931275594,-4.63000000000009)) ;
#105352=CARTESIAN_POINT('Ctrl Pts',(0.550000000000012,2.67648433237898,
-4.6157238466627)) ;
#105353=CARTESIAN_POINT('Ctrl Pts',(0.546908864252786,2.69988533923263,
-4.60352570084762)) ;
#105354=CARTESIAN_POINT('Ctrl Pts',(0.539540151921445,2.76165254733708,
-4.58409159819012)) ;
#105355=CARTESIAN_POINT('Ctrl Pts',(0.536602540378443,2.79600904778112,
-4.58)) ;
#105356=CARTESIAN_POINT('Ctrl Pts',(0.536602540378443,2.83090991212703,
-4.58)) ;
#105357=CARTESIAN_POINT('Origin',(8.,3.4,-5.48)) ;
#105358=CARTESIAN_POINT('Origin',(7.96847777691809,3.4,-5.48)) ;
#105359=CARTESIAN_POINT('Origin',(1.5,4.2,-5.48)) ;
#105360=CARTESIAN_POINT('Origin',(7.96847777691809,4.2,-5.48)) ;
#105361=CARTESIAN_POINT('Origin',(8.64348900069683,3.87250785664512,-5.00749214335488)) ;
#105362=CARTESIAN_POINT('Origin',(7.96847777691809,3.4,-5.48)) ;
#105363=CARTESIAN_POINT('Origin',(8.4,3.70206555615734,-5.17793444384266)) ;
#105364=CARTESIAN_POINT('Origin',(8.26722637443421,3.99087598173872,-5.27087598173872)) ;
#105365=CARTESIAN_POINT('Origin',(7.96847777691809,4.2,-5.48)) ;
#105366=CARTESIAN_POINT('Origin',(8.4,3.89793444384266,-5.17793444384266)) ;
#105367=CARTESIAN_POINT('Origin',(8.4,3.95,-5.17793444384266)) ;
#105368=CARTESIAN_POINT('Origin',(8.4,3.70206555615734,-5.17793444384266)) ;
#105369=CARTESIAN_POINT('Origin',(8.4,3.89793444384266,-5.17793444384266)) ;
#105370=CARTESIAN_POINT('Origin',(8.4,3.70206555615734,-5.17793444384266)) ;
#105371=CARTESIAN_POINT('Origin',(8.4,3.70206555615734,-5.17793444384266)) ;
#105372=CARTESIAN_POINT('Origin',(1.5,3.4,-4.68)) ;
#105373=CARTESIAN_POINT('Origin',(7.96847777691809,3.4,-4.68)) ;
#105374=CARTESIAN_POINT('Origin',(1.5,4.2,-4.68)) ;
#105375=CARTESIAN_POINT('Origin',(7.96847777691809,4.2,-4.68)) ;
#105376=CARTESIAN_POINT('Origin',(8.4,3.89793444384266,-5.17793444384266)) ;
#105377=CARTESIAN_POINT('Origin',(8.4,3.89793444384266,-5.17793444384266)) ;
#105378=CARTESIAN_POINT('Origin',(8.4,3.70206555615734,-4.58)) ;
#105379=CARTESIAN_POINT('Origin',(8.4,3.70206555615734,-4.98206555615734)) ;
#105380=CARTESIAN_POINT('Origin',(8.28995364716148,3.62503310917037,-4.90503310917037)) ;
#105381=CARTESIAN_POINT('Origin',(7.96847777691809,3.4,-4.68)) ;
#105382=CARTESIAN_POINT('Origin',(8.4,3.70206555615734,-4.98206555615734)) ;
#105383=CARTESIAN_POINT('Origin',(7.91369102089885,4.23835072921347,-4.64164927078653)) ;
#105384=CARTESIAN_POINT('Origin',(7.96847777691809,4.2,-4.68)) ;
#105385=CARTESIAN_POINT('Origin',(8.4,3.89793444384266,-4.98206555615734)) ;
#105386=CARTESIAN_POINT('Origin',(8.4,3.89793444384266,-4.58)) ;
#105387=CARTESIAN_POINT('Origin',(8.4,3.89793444384266,-4.98206555615734)) ;
#105388=CARTESIAN_POINT('Origin',(8.4,3.70206555615734,-4.98206555615734)) ;
#105389=CARTESIAN_POINT('Origin',(8.4,3.70206555615734,-4.98206555615734)) ;
#105390=CARTESIAN_POINT('Origin',(8.4,3.89793444384266,-4.98206555615734)) ;
#105391=CARTESIAN_POINT('Origin',(8.4,3.89793444384266,-4.98206555615734)) ;
#105392=CARTESIAN_POINT('Origin',(8.4,2.68967221921331,-4.98206555615734)) ;
#105393=CARTESIAN_POINT('Origin',(9.9,6.8847127088383,-7.62)) ;
#105394=CARTESIAN_POINT('Origin',(9.9,6.8847127088383,-6.03971270883831)) ;
#105395=CARTESIAN_POINT('Origin',(8.77035388141948,6.69643835574155,-5.85143835574155)) ;
#105396=CARTESIAN_POINT('Ctrl Pts',(8.58356010126947,6.66256607592813,-5.71892668354491)) ;
#105397=CARTESIAN_POINT('Ctrl Pts',(8.58266714977878,6.65676189123867,-5.71877785829646)) ;
#105398=CARTESIAN_POINT('Ctrl Pts',(8.58182526931896,6.6507714222091,-5.71911417147406)) ;
#105399=CARTESIAN_POINT('Ctrl Pts',(8.58032528754339,6.63886560514846,-5.72091273509962)) ;
#105400=CARTESIAN_POINT('Ctrl Pts',(8.57966270906115,6.63295370212233,-5.72234482433268)) ;
#105401=CARTESIAN_POINT('Ctrl Pts',(8.57906641006225,6.62681909302566,-5.72447717449357)) ;
#105402=CARTESIAN_POINT('Ctrl Pts',(8.57903375157331,6.62647998752528,-5.72459716972835)) ;
#105403=CARTESIAN_POINT('Ctrl Pts',(8.57846569624192,6.62052582174872,-5.72674173168093)) ;
#105404=CARTESIAN_POINT('Ctrl Pts',(8.57802501793963,6.61503168015239,-5.72931428585577)) ;
#105405=CARTESIAN_POINT('Ctrl Pts',(8.57766199200567,6.60925146760294,-5.73274621332342)) ;
#105406=CARTESIAN_POINT('Ctrl Pts',(8.57762821177171,6.60869602779095,-5.73308383516466)) ;
#105407=CARTESIAN_POINT('Ctrl Pts',(8.57728522755448,6.60286036001487,-5.736714798957)) ;
#105408=CARTESIAN_POINT('Ctrl Pts',(8.57709550103272,6.59788070192389,-5.74054822105585)) ;
#105409=CARTESIAN_POINT('Ctrl Pts',(8.57703980289277,6.59299711069447,-5.7451723373543)) ;
#105410=CARTESIAN_POINT('Ctrl Pts',(8.5770367027102,6.59265952430066,-5.74549689254174)) ;
#105411=CARTESIAN_POINT('Ctrl Pts',(8.57701334129167,6.58927432516127,-5.74880138159525)) ;
#105412=CARTESIAN_POINT('Ctrl Pts',(8.57705699426433,6.58642971201549,-5.75199174440871)) ;
#105413=CARTESIAN_POINT('Ctrl Pts',(8.57735031225518,6.57961409340219,-5.76079544175541)) ;
#105414=CARTESIAN_POINT('Ctrl Pts',(8.57770856513435,6.57604383182912,-5.76666824553985)) ;
#105415=CARTESIAN_POINT('Ctrl Pts',(8.5786570497109,6.57055741297632,-5.77833221933877)) ;
#105416=CARTESIAN_POINT('Ctrl Pts',(8.57922107378969,6.56851476050442,-5.78407363490774)) ;
#105417=CARTESIAN_POINT('Ctrl Pts',(8.57993695782544,6.5668761019375,-5.79045593481641)) ;
#105418=CARTESIAN_POINT('Ctrl Pts',(8.58000419042984,6.56673001682054,-5.79104783518392)) ;
#105419=CARTESIAN_POINT('Ctrl Pts',(8.58074399738023,6.56520526212514,-5.7974812517356)) ;
#105420=CARTESIAN_POINT('Ctrl Pts',(8.58149993293355,6.56438134785768,-5.80335418009406)) ;
#105421=CARTESIAN_POINT('Ctrl Pts',(8.58236768178486,6.56403389662199,-5.80949875782384)) ;
#105422=CARTESIAN_POINT('Ctrl Pts',(8.58242358604552,6.56401394107884,-5.80989217363188)) ;
#105423=CARTESIAN_POINT('Ctrl Pts',(8.58283067264383,6.56388592662946,-5.81273942342641)) ;
#105424=CARTESIAN_POINT('Ctrl Pts',(8.5831915624065,6.56386525642004,-5.81516995058283)) ;
#105425=CARTESIAN_POINT('Ctrl Pts',(8.58356019967708,6.56392669994633,-5.81756626506471)) ;
#105426=CARTESIAN_POINT('Origin',(9.9,6.8847127088383,-6.03971270883831)) ;
#105427=CARTESIAN_POINT('Origin',(9.9,6.8847127088383,-6.03971270883831)) ;
#105428=CARTESIAN_POINT('Origin',(9.9,6.8847127088383,-6.03971270883831)) ;
#105429=CARTESIAN_POINT('Origin',(9.9,7.72792407799439,-7.62)) ;
#105430=CARTESIAN_POINT('Origin',(9.9,7.72792407799439,-6.03971270883831)) ;
#105431=CARTESIAN_POINT('Origin',(9.90000000000001,4.35421736843756,-6.03971270883831)) ;
#105432=CARTESIAN_POINT('Origin',(9.9,7.72792407799439,-6.03971270883831)) ;
#105433=CARTESIAN_POINT('Origin',(9.9,7.72792407799439,-6.03971270883831)) ;
#105434=CARTESIAN_POINT('Origin',(9.9,7.72792407799439,-6.03971270883831)) ;
#105435=CARTESIAN_POINT('Origin',(10.9628342502842,7.37364599456632,-6.21685175055234)) ;
#105436=CARTESIAN_POINT('Ctrl Pts',(8.56837732530586,8.27720755823131,-5.81250525379773)) ;
#105437=CARTESIAN_POINT('Ctrl Pts',(8.56753565030796,8.2774881236726,-5.80661299219742)) ;
#105438=CARTESIAN_POINT('Ctrl Pts',(8.5668204554169,8.27721180667909,-5.80054129443957)) ;
#105439=CARTESIAN_POINT('Ctrl Pts',(8.56575413148036,8.2753862416024,-5.78872847211981)) ;
#105440=CARTESIAN_POINT('Ctrl Pts',(8.56538426077881,8.27391165896583,-5.78299056243199)) ;
#105441=CARTESIAN_POINT('Ctrl Pts',(8.56517777855947,8.27166501362668,-5.77701477545133)) ;
#105442=CARTESIAN_POINT('Ctrl Pts',(8.56516523451691,8.27151619608676,-5.77662763828585)) ;
#105443=CARTESIAN_POINT('Ctrl Pts',(8.56497390811218,8.26902793125447,-5.77029533599119)) ;
#105444=CARTESIAN_POINT('Ctrl Pts',(8.56499903025539,8.26597630129447,-5.76453577846586)) ;
#105445=CARTESIAN_POINT('Ctrl Pts',(8.56538588200264,8.26046191593052,-5.75659067236816)) ;
#105446=CARTESIAN_POINT('Ctrl Pts',(8.56556309332513,8.25853771611453,-5.75412123645577)) ;
#105447=CARTESIAN_POINT('Ctrl Pts',(8.56628156514555,8.25214511987154,-5.74680175668912)) ;
#105448=CARTESIAN_POINT('Ctrl Pts',(8.56700742874798,8.24720216256262,-5.74230544523098)) ;
#105449=CARTESIAN_POINT('Ctrl Pts',(8.5688071379813,8.23661566152166,-5.73462449488006)) ;
#105450=CARTESIAN_POINT('Ctrl Pts',(8.56986039391321,8.23102391526976,-5.73138488072561)) ;
#105451=CARTESIAN_POINT('Ctrl Pts',(8.57116255171754,8.22459552194136,-5.72844677452705)) ;
#105452=CARTESIAN_POINT('Ctrl Pts',(8.5712749581022,8.22404408343787,-5.72820066079021)) ;
#105453=CARTESIAN_POINT('Ctrl Pts',(8.57260511146326,8.21755901312516,-5.72537491530524)) ;
#105454=CARTESIAN_POINT('Ctrl Pts',(8.57395629672869,8.21135759730784,-5.72334638642728)) ;
#105455=CARTESIAN_POINT('Ctrl Pts',(8.57552311082448,8.20452945286157,-5.72174954431703)) ;
#105456=CARTESIAN_POINT('Ctrl Pts',(8.57564505123029,8.20400026307019,-5.7216298269559)) ;
#105457=CARTESIAN_POINT('Ctrl Pts',(8.57731301559527,8.19679193622625,-5.72005346253701)) ;
#105458=CARTESIAN_POINT('Ctrl Pts',(8.57896065127873,8.1900216848535,-5.71921096934403)) ;
#105459=CARTESIAN_POINT('Ctrl Pts',(8.58161366784367,8.17959769015469,-5.71875531727718)) ;
#105460=CARTESIAN_POINT('Ctrl Pts',(8.58258362864271,8.17587911616509,-5.71876393810712)) ;
#105461=CARTESIAN_POINT('Ctrl Pts',(8.58356010126947,8.17221734381475,-5.71892668354492)) ;
#105462=CARTESIAN_POINT('Origin',(7.96824861826159,6.56275414521524,-4.44224585478477)) ;
#105463=CARTESIAN_POINT('Origin',(8.59688370202654,6.66156024040368,-4.35124347526272)) ;
#105464=CARTESIAN_POINT('Origin',(9.9,6.8847127088383,-4.1202872911617)) ;
#105465=CARTESIAN_POINT('Origin',(9.9,6.8847127088383,-7.62)) ;
#105466=CARTESIAN_POINT('Origin',(9.9,6.8847127088383,-4.1202872911617)) ;
#105467=CARTESIAN_POINT('Origin',(9.9,6.8847127088383,-4.1202872911617)) ;
#105468=CARTESIAN_POINT('Origin',(9.9,6.8847127088383,-4.1202872911617)) ;
#105469=CARTESIAN_POINT('Origin',(9.9,6.8,-4.1202872911617)) ;
#105470=CARTESIAN_POINT('Origin',(9.9,7.72792407799439,-4.1202872911617)) ;
#105471=CARTESIAN_POINT('Origin',(9.9,7.72792407799439,-7.62)) ;
#105472=CARTESIAN_POINT('Origin',(9.9,7.72792407799439,-4.1202872911617)) ;
#105473=CARTESIAN_POINT('Origin',(9.9,7.72792407799439,-4.1202872911617)) ;
#105474=CARTESIAN_POINT('Origin',(9.9,7.72792407799439,-4.1202872911617)) ;
#105475=CARTESIAN_POINT('Origin',(9.60917571369883,7.82486550676144,-4.16875800554523)) ;
#105476=CARTESIAN_POINT('Origin',(8.5909900184595,8.18966234087008,-4.34516097389893)) ;
#105477=CARTESIAN_POINT('Origin',(0.45,4.4,-5.08)) ;
#105478=CARTESIAN_POINT('Origin',(0.45,4.4,-5.53)) ;
#105479=CARTESIAN_POINT('Origin',(0.45,4.4,-4.63)) ;
#105480=CARTESIAN_POINT('Origin',(-1.9,7.55,-7.62)) ;
#105481=CARTESIAN_POINT('Origin',(6.9,7.75,-7.62)) ;
#105482=CARTESIAN_POINT('Origin',(7.1,8.2,-7.62)) ;
#105483=CARTESIAN_POINT('Origin',(9.9,0.1,-7.62)) ;
#105484=CARTESIAN_POINT('Origin',(9.9,1.16528729116168,-7.62)) ;
#105485=CARTESIAN_POINT('Origin',(9.9,1.16528729116168,-7.12416188017819)) ;
#105486=CARTESIAN_POINT('Origin',(9.9,3.8,-5.08)) ;
#105487=CARTESIAN_POINT('Origin',(9.9,1.16528729116168,-3.0358381198218)) ;
#105488=CARTESIAN_POINT('Origin',(9.9,1.16528729116168,-7.12416188017819)) ;
#105489=CARTESIAN_POINT('Origin',(9.9,1.16528729116168,-7.62)) ;
#105490=CARTESIAN_POINT('Origin',(9.9,1.16528729116168,-3.0358381198218)) ;
#105491=CARTESIAN_POINT('Ctrl Pts',(0.55,0.3,-5.53)) ;
#105492=CARTESIAN_POINT('Ctrl Pts',(0.55,0.3,-5.63)) ;
#105493=CARTESIAN_POINT('Ctrl Pts',(0.45,0.3,-5.63)) ;
#105494=CARTESIAN_POINT('Ctrl Pts',(0.55,0.28690770353672,-5.53000000081823)) ;
#105495=CARTESIAN_POINT('Ctrl Pts',(0.549992696052345,0.300543498459179,
-5.62999269603997)) ;
#105496=CARTESIAN_POINT('Ctrl Pts',(0.450000000818259,0.286907703536718,
-5.63)) ;
#105497=CARTESIAN_POINT('Ctrl Pts',(0.552602750539093,0.273825167611082,
-5.53520550107818)) ;
#105498=CARTESIAN_POINT('Ctrl Pts',(0.546703256435892,0.299059401315782,
-5.62670325643589)) ;
#105499=CARTESIAN_POINT('Ctrl Pts',(0.455205501078185,0.273825167611084,
-5.63260275053909)) ;
#105500=CARTESIAN_POINT('Ctrl Pts',(0.56262134295865,0.249638145915901,
-5.5552426859173)) ;
#105501=CARTESIAN_POINT('Ctrl Pts',(0.544986924117075,0.282072776439542,
-5.62498692411708)) ;
#105502=CARTESIAN_POINT('Ctrl Pts',(0.4752426859173,0.249638145915898,-5.64262134295865)) ;
#105503=CARTESIAN_POINT('Ctrl Pts',(0.570033341471288,0.238545302291403,
-5.57006668294258)) ;
#105504=CARTESIAN_POINT('Ctrl Pts',(0.547116196858396,0.267914459835244,
-5.6271161968584)) ;
#105505=CARTESIAN_POINT('Ctrl Pts',(0.490066682942577,0.238545302291402,
-5.65003334147129)) ;
#105506=CARTESIAN_POINT('Ctrl Pts',(0.597801282701459,0.210777361061231,
-5.62560256540292)) ;
#105507=CARTESIAN_POINT('Ctrl Pts',(0.570853448890183,0.226374713859281,
-5.65085344889018)) ;
#105508=CARTESIAN_POINT('Ctrl Pts',(0.545602565402917,0.210777361061233,
-5.67780128270146)) ;
#105509=CARTESIAN_POINT('Ctrl Pts',(0.623746567173609,0.2,-5.6774931343473)) ;
#105510=CARTESIAN_POINT('Ctrl Pts',(0.610458667315046,0.2,-5.69045866731505)) ;
#105511=CARTESIAN_POINT('Ctrl Pts',(0.59749313434727,0.2,-5.70374656717367)) ;
#105512=CARTESIAN_POINT('Ctrl Pts',(0.65,0.2,-5.73)) ;
#105513=CARTESIAN_POINT('Ctrl Pts',(0.65,0.2,-5.73)) ;
#105514=CARTESIAN_POINT('Ctrl Pts',(0.65,0.2,-5.73)) ;
#105515=CARTESIAN_POINT('Origin',(0.45,0.3,-5.53)) ;
#105516=CARTESIAN_POINT('Origin',(0.45,1.24941393210234E-16,-5.53)) ;
#105517=CARTESIAN_POINT('Origin',(0.45,4.4,-5.53)) ;
#105518=CARTESIAN_POINT('Origin',(0.45,4.4,-5.53)) ;
#105519=CARTESIAN_POINT('Origin',(0.45,4.4,-5.53)) ;
#105520=CARTESIAN_POINT('Origin',(0.549999999999999,4.4,-5.53)) ;
#105521=CARTESIAN_POINT('Origin',(-1.7,4.4,-5.53)) ;
#105522=CARTESIAN_POINT('Ctrl Pts',(-1.8,4.6,-5.73)) ;
#105523=CARTESIAN_POINT('Ctrl Pts',(-1.8,4.6,-5.73)) ;
#105524=CARTESIAN_POINT('Ctrl Pts',(-1.8,4.6,-5.73)) ;
#105525=CARTESIAN_POINT('Ctrl Pts',(-1.8,4.5737465671737,-5.67749313434726)) ;
#105526=CARTESIAN_POINT('Ctrl Pts',(-1.8,4.56045866731625,-5.69045866731612)) ;
#105527=CARTESIAN_POINT('Ctrl Pts',(-1.8,4.54749313434731,-5.70374656717359)) ;
#105528=CARTESIAN_POINT('Ctrl Pts',(-1.78922263893876,4.54780128270145,
-5.62560256540292)) ;
#105529=CARTESIAN_POINT('Ctrl Pts',(-1.77362528614073,4.52085344889015,
-5.65085344889015)) ;
#105530=CARTESIAN_POINT('Ctrl Pts',(-1.78922263893876,4.49560256540291,
-5.67780128270145)) ;
#105531=CARTESIAN_POINT('Ctrl Pts',(-1.7614546977086,4.5200333414713,-5.57006668294258)) ;
#105532=CARTESIAN_POINT('Ctrl Pts',(-1.73208554016475,4.49711619685841,
-5.62711619685841)) ;
#105533=CARTESIAN_POINT('Ctrl Pts',(-1.7614546977086,4.44006668294258,-5.6500333414713)) ;
#105534=CARTESIAN_POINT('Ctrl Pts',(-1.7503618540841,4.51262134295865,-5.55524268591729)) ;
#105535=CARTESIAN_POINT('Ctrl Pts',(-1.71792722356046,4.49498692411707,
-5.62498692411707)) ;
#105536=CARTESIAN_POINT('Ctrl Pts',(-1.7503618540841,4.42524268591729,-5.64262134295865)) ;
#105537=CARTESIAN_POINT('Ctrl Pts',(-1.72617483238892,4.50260275053909,
-5.5352055010782)) ;
#105538=CARTESIAN_POINT('Ctrl Pts',(-1.70094059868422,4.4967032564359,-5.6267032564359)) ;
#105539=CARTESIAN_POINT('Ctrl Pts',(-1.72617483238892,4.4052055010782,-5.63260275053909)) ;
#105540=CARTESIAN_POINT('Ctrl Pts',(-1.71309229646328,4.5,-5.53000000081823)) ;
#105541=CARTESIAN_POINT('Ctrl Pts',(-1.69945650154594,4.49999269603999,
-5.62999269603999)) ;
#105542=CARTESIAN_POINT('Ctrl Pts',(-1.71309229646328,4.40000000081823,
-5.63)) ;
#105543=CARTESIAN_POINT('Ctrl Pts',(-1.7,4.5,-5.53)) ;
#105544=CARTESIAN_POINT('Ctrl Pts',(-1.7,4.5,-5.63)) ;
#105545=CARTESIAN_POINT('Ctrl Pts',(-1.7,4.4,-5.63)) ;
#105546=CARTESIAN_POINT('Ctrl Pts',(-1.8,4.6,-4.43)) ;
#105547=CARTESIAN_POINT('Ctrl Pts',(-1.8,4.6,-4.43)) ;
#105548=CARTESIAN_POINT('Ctrl Pts',(-1.8,4.6,-4.43)) ;
#105549=CARTESIAN_POINT('Ctrl Pts',(-1.8,4.54749313434731,-4.45625343282641)) ;
#105550=CARTESIAN_POINT('Ctrl Pts',(-1.8,4.56045866731625,-4.46954133268388)) ;
#105551=CARTESIAN_POINT('Ctrl Pts',(-1.8,4.57374656717369,-4.48250686565274)) ;
#105552=CARTESIAN_POINT('Ctrl Pts',(-1.78922263893876,4.49560256540291,
-4.48219871729855)) ;
#105553=CARTESIAN_POINT('Ctrl Pts',(-1.77362528614073,4.52085344889015,
-4.50914655110985)) ;
#105554=CARTESIAN_POINT('Ctrl Pts',(-1.78922263893876,4.54780128270145,
-4.53439743459709)) ;
#105555=CARTESIAN_POINT('Ctrl Pts',(-1.7614546977086,4.44006668294258,-4.5099666585287)) ;
#105556=CARTESIAN_POINT('Ctrl Pts',(-1.73208554016475,4.49711619685842,
-4.53288380314159)) ;
#105557=CARTESIAN_POINT('Ctrl Pts',(-1.7614546977086,4.5200333414713,-4.58993331705742)) ;
#105558=CARTESIAN_POINT('Ctrl Pts',(-1.7503618540841,4.42524268591729,-4.51737865704135)) ;
#105559=CARTESIAN_POINT('Ctrl Pts',(-1.71792722356046,4.49498692411707,
-4.53501307588293)) ;
#105560=CARTESIAN_POINT('Ctrl Pts',(-1.7503618540841,4.51262134295865,-4.60475731408271)) ;
#105561=CARTESIAN_POINT('Ctrl Pts',(-1.72617483238892,4.4052055010782,-4.52739724946091)) ;
#105562=CARTESIAN_POINT('Ctrl Pts',(-1.70094059868422,4.4967032564359,-4.5332967435641)) ;
#105563=CARTESIAN_POINT('Ctrl Pts',(-1.72617483238892,4.50260275053909,
-4.6247944989218)) ;
#105564=CARTESIAN_POINT('Ctrl Pts',(-1.71309229646328,4.40000000081823,
-4.53)) ;
#105565=CARTESIAN_POINT('Ctrl Pts',(-1.69945650154594,4.49999269603999,
-4.53000730396001)) ;
#105566=CARTESIAN_POINT('Ctrl Pts',(-1.71309229646328,4.5,-4.62999999918177)) ;
#105567=CARTESIAN_POINT('Ctrl Pts',(-1.7,4.4,-4.53)) ;
#105568=CARTESIAN_POINT('Ctrl Pts',(-1.7,4.5,-4.53)) ;
#105569=CARTESIAN_POINT('Ctrl Pts',(-1.7,4.5,-4.63)) ;
#105570=CARTESIAN_POINT('Origin',(-1.7,4.4,-4.63)) ;
#105571=CARTESIAN_POINT('Origin',(0.549999999999999,4.4,-4.63)) ;
#105572=CARTESIAN_POINT('Origin',(0.45,4.4,-4.63)) ;
#105573=CARTESIAN_POINT('Origin',(0.45,4.4,-4.63)) ;
#105574=CARTESIAN_POINT('Origin',(0.45,4.4,-4.63)) ;
#105575=CARTESIAN_POINT('Origin',(0.45,4.9047241136249E-17,-4.63)) ;
#105576=CARTESIAN_POINT('Origin',(0.45,0.3,-4.63)) ;
#105577=CARTESIAN_POINT('Ctrl Pts',(0.45,0.3,-4.53)) ;
#105578=CARTESIAN_POINT('Ctrl Pts',(0.55,0.3,-4.53)) ;
#105579=CARTESIAN_POINT('Ctrl Pts',(0.55,0.3,-4.63)) ;
#105580=CARTESIAN_POINT('Ctrl Pts',(0.450000000818259,0.286907703536718,
-4.53)) ;
#105581=CARTESIAN_POINT('Ctrl Pts',(0.549992696057035,0.30054349846111,
-4.53000730396006)) ;
#105582=CARTESIAN_POINT('Ctrl Pts',(0.55,0.28690770353672,-4.62999999918177)) ;
#105583=CARTESIAN_POINT('Ctrl Pts',(0.455205501078185,0.273825167611084,
-4.52739724946091)) ;
#105584=CARTESIAN_POINT('Ctrl Pts',(0.5467032564359,0.299059401315787,-4.53329674356411)) ;
#105585=CARTESIAN_POINT('Ctrl Pts',(0.552602750539093,0.273825167611082,
-4.62479449892182)) ;
#105586=CARTESIAN_POINT('Ctrl Pts',(0.4752426859173,0.249638145915898,-4.51737865704135)) ;
#105587=CARTESIAN_POINT('Ctrl Pts',(0.544986924117068,0.282072776439538,
-4.53501307588292)) ;
#105588=CARTESIAN_POINT('Ctrl Pts',(0.56262134295865,0.249638145915901,
-4.6047573140827)) ;
#105589=CARTESIAN_POINT('Ctrl Pts',(0.490066682942577,0.238545302291402,
-4.50996665852871)) ;
#105590=CARTESIAN_POINT('Ctrl Pts',(0.547116196858396,0.267914459835244,
-4.5328838031416)) ;
#105591=CARTESIAN_POINT('Ctrl Pts',(0.570033341471288,0.238545302291403,
-4.58993331705742)) ;
#105592=CARTESIAN_POINT('Ctrl Pts',(0.545602565402917,0.210777361061233,
-4.48219871729854)) ;
#105593=CARTESIAN_POINT('Ctrl Pts',(0.570853448890183,0.226374713859281,
-4.50914655110982)) ;
#105594=CARTESIAN_POINT('Ctrl Pts',(0.597801282701459,0.210777361061231,
-4.53439743459709)) ;
#105595=CARTESIAN_POINT('Ctrl Pts',(0.59749313434727,0.2,-4.45625343282633)) ;
#105596=CARTESIAN_POINT('Ctrl Pts',(0.610458667315046,0.2,-4.46954133268495)) ;
#105597=CARTESIAN_POINT('Ctrl Pts',(0.62374656717361,0.2,-4.4825068656527)) ;
#105598=CARTESIAN_POINT('Ctrl Pts',(0.65,0.2,-4.43)) ;
#105599=CARTESIAN_POINT('Ctrl Pts',(0.65,0.2,-4.43)) ;
#105600=CARTESIAN_POINT('Ctrl Pts',(0.65,0.2,-4.43)) ;
#105601=CARTESIAN_POINT('Ctrl Pts',(8.5,8.17221734381475,-5.6202872911617)) ;
#105602=CARTESIAN_POINT('Ctrl Pts',(8.5,8.17221734381474,-5.705)) ;
#105603=CARTESIAN_POINT('Ctrl Pts',(8.58356010126947,8.17221734381475,-5.71892668354491)) ;
#105604=CARTESIAN_POINT('Ctrl Pts',(8.5,8.23335379241386,-5.62028729273906)) ;
#105605=CARTESIAN_POINT('Ctrl Pts',(8.5,8.20847425960651,-5.69745756742167)) ;
#105606=CARTESIAN_POINT('Ctrl Pts',(8.57460439031225,8.20580126077887,-5.71743406505204)) ;
#105607=CARTESIAN_POINT('Ctrl Pts',(8.5,8.29192178062155,-5.64717411507849)) ;
#105608=CARTESIAN_POINT('Ctrl Pts',(8.5,8.25010493984404,-5.70925460831168)) ;
#105609=CARTESIAN_POINT('Ctrl Pts',(8.56800970738923,8.23725302684488,-5.72977836318993)) ;
#105610=CARTESIAN_POINT('Ctrl Pts',(8.5,8.36583651094028,-5.73655062329137)) ;
#105611=CARTESIAN_POINT('Ctrl Pts',(8.5,8.29925403146167,-5.76336143703663)) ;
#105612=CARTESIAN_POINT('Ctrl Pts',(8.56373266208983,8.27563607377073,-5.77375377641315)) ;
#105613=CARTESIAN_POINT('Ctrl Pts',(8.5,8.38029241321763,-5.79795520569967)) ;
#105614=CARTESIAN_POINT('Ctrl Pts',(8.5,8.30669116589123,-5.80480884994108)) ;
#105615=CARTESIAN_POINT('Ctrl Pts',(8.56610123859368,8.28208399509958,-5.80480870240703)) ;
#105616=CARTESIAN_POINT('Ctrl Pts',(8.5,8.36719795478507,-5.85605472347988)) ;
#105617=CARTESIAN_POINT('Ctrl Pts',(8.5,8.29381262650623,-5.83951514967181)) ;
#105618=CARTESIAN_POINT('Ctrl Pts',(8.57227762885807,8.27346847343705,-5.83492998763544)) ;
#105619=CARTESIAN_POINT('Ctrl Pts',(8.5485213309235,8.28383177029354,-5.83598653273363)) ;
#105620=CARTESIAN_POINT('Ctrl Pts',(8.54913757890789,8.28625057716299,-5.82292165918399)) ;
#105621=CARTESIAN_POINT('Ctrl Pts',(8.549146361399,8.28675781111762,-5.80926478940262)) ;
#105622=CARTESIAN_POINT('Ctrl Pts',(8.54883414737369,8.28489376483071,-5.79609886942504)) ;
#105623=CARTESIAN_POINT('Ctrl Pts',(8.54852072231757,8.28302248819127,-5.78288188084279)) ;
#105624=CARTESIAN_POINT('Ctrl Pts',(8.54791723678494,8.27865742078997,-5.76983129581174)) ;
#105625=CARTESIAN_POINT('Ctrl Pts',(8.54677696932927,8.27237937104781,-5.75810207672967)) ;
#105626=CARTESIAN_POINT('Ctrl Pts',(8.5454465495755,8.26505438658866,-5.74441687973016)) ;
#105627=CARTESIAN_POINT('Ctrl Pts',(8.54324462275112,8.25487237915563,-5.7322537533388)) ;
#105628=CARTESIAN_POINT('Ctrl Pts',(8.53884071267076,8.24480815719263,-5.72120716819918)) ;
#105629=CARTESIAN_POINT('Ctrl Pts',(8.5342440055524,8.23430333763594,-5.70967697897682)) ;
#105630=CARTESIAN_POINT('Ctrl Pts',(8.52670159721618,8.22420330618022,-5.69870426024299)) ;
#105631=CARTESIAN_POINT('Ctrl Pts',(8.51928858688475,8.21729138318396,-5.68598817546528)) ;
#105632=CARTESIAN_POINT('Ctrl Pts',(8.51327528614099,8.21168455548023,-5.67567311604503)) ;
#105633=CARTESIAN_POINT('Ctrl Pts',(8.50759525524367,8.20778929846109,-5.66398494308279)) ;
#105634=CARTESIAN_POINT('Ctrl Pts',(8.50412058850191,8.20498026622232,-5.65157394866282)) ;
#105635=CARTESIAN_POINT('Ctrl Pts',(8.50147164778346,8.20283877743224,-5.6421123251694)) ;
#105636=CARTESIAN_POINT('Ctrl Pts',(8.50000317248551,8.2012555848359,-5.632083357655)) ;
#105637=CARTESIAN_POINT('Ctrl Pts',(8.50000000513446,8.20000405629318,-5.62210523872843)) ;
#105638=CARTESIAN_POINT('Origin',(8.6,8.17221734381475,-5.6202872911617)) ;
#105639=CARTESIAN_POINT('Origin',(8.6,4.35421736843756,-5.6202872911617)) ;
#105640=CARTESIAN_POINT('Origin',(8.6,6.66256607592813,-5.6202872911617)) ;
#105641=CARTESIAN_POINT('Ctrl Pts',(8.5,6.47083593368087,-5.86480810992443)) ;
#105642=CARTESIAN_POINT('Ctrl Pts',(8.5,6.55684090505321,-5.84438773869521)) ;
#105643=CARTESIAN_POINT('Ctrl Pts',(8.58772778625753,6.56739561896918,-5.84188170709095)) ;
#105644=CARTESIAN_POINT('Ctrl Pts',(8.5,6.45680686388573,-5.80572152971771)) ;
#105645=CARTESIAN_POINT('Ctrl Pts',(8.5000000000001,6.54406229478618,-5.81251016540367)) ;
#105646=CARTESIAN_POINT('Ctrl Pts',(8.58195196310365,6.55941415012444,-5.81135768687784)) ;
#105647=CARTESIAN_POINT('Ctrl Pts',(8.5,6.4706155658439,-5.74195245680485)) ;
#105648=CARTESIAN_POINT('Ctrl Pts',(8.5,6.5483636998889,-5.7723987274071)) ;
#105649=CARTESIAN_POINT('Ctrl Pts',(8.57801125828726,6.56566601372231,-5.77883445920279)) ;
#105650=CARTESIAN_POINT('Ctrl Pts',(8.5,6.54379299301796,-5.6486264716581)) ;
#105651=CARTESIAN_POINT('Ctrl Pts',(8.5,6.59071789516222,-5.71622651529222)) ;
#105652=CARTESIAN_POINT('Ctrl Pts',(8.57642058265786,6.60198961470444,-5.73190635402451)) ;
#105653=CARTESIAN_POINT('Ctrl Pts',(8.5,6.6022051807538,-5.6202872929747)) ;
#105654=CARTESIAN_POINT('Ctrl Pts',(8.5,6.62800697860326,-5.70091767076279)) ;
#105655=CARTESIAN_POINT('Ctrl Pts',(8.57879135173926,6.63156920211804,-5.71813189195654)) ;
#105656=CARTESIAN_POINT('Ctrl Pts',(8.5,6.66256607592813,-5.6202872911617)) ;
#105657=CARTESIAN_POINT('Ctrl Pts',(8.5,6.66256607592813,-5.705)) ;
#105658=CARTESIAN_POINT('Ctrl Pts',(8.58356010126947,6.66256607592813,-5.71892668354491)) ;
#105659=CARTESIAN_POINT('',(8.5456536674855,6.61650711947,-5.71396531829168)) ;
#105660=CARTESIAN_POINT('Ctrl Pts',(8.545653667161,6.61650712004134,-5.71396531781346)) ;
#105661=CARTESIAN_POINT('Ctrl Pts',(8.54527684775566,6.61717057264364,-5.71341000086367)) ;
#105662=CARTESIAN_POINT('Ctrl Pts',(8.54488909344002,6.61782772231436,-5.71285542989966)) ;
#105663=CARTESIAN_POINT('Ctrl Pts',(8.54449064961559,6.61847724592619,-5.7123008713851)) ;
#105664=CARTESIAN_POINT('Ctrl Pts',(8.54445329550705,6.6185381387648,-5.71224888152437)) ;
#105665=CARTESIAN_POINT('Ctrl Pts',(8.54441584757974,6.61859896452233,-5.71219689179164)) ;
#105666=CARTESIAN_POINT('Ctrl Pts',(8.54437830610597,6.6186597220747,-5.71214490158589)) ;
#105667=CARTESIAN_POINT('Ctrl Pts',(8.54363538409146,6.61986207559664,-5.7111160483068)) ;
#105668=CARTESIAN_POINT('Ctrl Pts',(8.54285495000587,6.62104203503536,-5.71008486217465)) ;
#105669=CARTESIAN_POINT('Ctrl Pts',(8.54204093171147,6.62218056960131,-5.70905111516717)) ;
#105670=CARTESIAN_POINT('Ctrl Pts',(8.54157979215435,6.62282554690603,-5.70846549978176)) ;
#105671=CARTESIAN_POINT('Ctrl Pts',(8.54110770812185,6.62345780120148,-5.70787864990663)) ;
#105672=CARTESIAN_POINT('Ctrl Pts',(8.54062344907116,6.62407892448169,-5.70728695413965)) ;
#105673=CARTESIAN_POINT('Ctrl Pts',(8.54011932596481,6.62472552591744,-5.7066709873185)) ;
#105674=CARTESIAN_POINT('Ctrl Pts',(8.53960207832254,6.62535666566135,-5.70605099058905)) ;
#105675=CARTESIAN_POINT('Ctrl Pts',(8.53907286520404,6.62597244099099,-5.70542522881105)) ;
#105676=CARTESIAN_POINT('Ctrl Pts',(8.53887441028459,6.6262033567396,-5.7051905681443)) ;
#105677=CARTESIAN_POINT('Ctrl Pts',(8.53867427664139,6.62643211299942,-5.70495509982106)) ;
#105678=CARTESIAN_POINT('Ctrl Pts',(8.53847256319995,6.6266587179511,-5.70471876421835)) ;
#105679=CARTESIAN_POINT('Ctrl Pts',(8.53842843838463,6.62670828778428,-5.70466706580526)) ;
#105680=CARTESIAN_POINT('Ctrl Pts',(8.53838423811747,6.62675775467668,-5.70461532601745)) ;
#105681=CARTESIAN_POINT('Ctrl Pts',(8.53833996369343,6.62680711871688,-5.70456354446015)) ;
#105682=CARTESIAN_POINT('Ctrl Pts',(8.53829707284513,6.62685494013081,-5.70451338107651)) ;
#105683=CARTESIAN_POINT('Ctrl Pts',(8.53825411240222,6.62690266502019,-5.70446317849309)) ;
#105684=CARTESIAN_POINT('Ctrl Pts',(8.53821108363803,6.62695029346533,-5.70441293643774)) ;
#105685=CARTESIAN_POINT('Ctrl Pts',(8.53803571435328,6.62714440934378,-5.70420816845341)) ;
#105686=CARTESIAN_POINT('Ctrl Pts',(8.53785876035506,6.62733753498028,-5.70400218366477)) ;
#105687=CARTESIAN_POINT('Ctrl Pts',(8.53767995296703,6.62753033615257,-5.7037944665652)) ;
#105688=CARTESIAN_POINT('Ctrl Pts',(8.53649871780654,6.62880401687798,-5.70242224842506)) ;
#105689=CARTESIAN_POINT('Ctrl Pts',(8.53528300832265,6.62998038079526,-5.70103807605966)) ;
#105690=CARTESIAN_POINT('Ctrl Pts',(8.53403203676338,6.63110281535143,-5.69960448656493)) ;
#105691=CARTESIAN_POINT('Ctrl Pts',(8.53346870389682,6.63160826591214,-5.6989589178679)) ;
#105692=CARTESIAN_POINT('Ctrl Pts',(8.53289959536919,6.63209979040222,-5.69830542565945)) ;
#105693=CARTESIAN_POINT('Ctrl Pts',(8.53232661340319,6.6325773534403,-5.69764370144387)) ;
#105694=CARTESIAN_POINT('Ctrl Pts',(8.53206474273905,6.63279561467254,-5.69734127279847)) ;
#105695=CARTESIAN_POINT('Ctrl Pts',(8.53180206199566,6.63301096017663,-5.69703712608071)) ;
#105696=CARTESIAN_POINT('Ctrl Pts',(8.53153874718657,6.63322338883724,-5.69673123888074)) ;
#105697=CARTESIAN_POINT('Ctrl Pts',(8.53007363658217,6.63440536369244,-5.69502925112708)) ;
#105698=CARTESIAN_POINT('Ctrl Pts',(8.52858926277508,6.63549697414123,-5.69327308391312)) ;
#105699=CARTESIAN_POINT('Ctrl Pts',(8.52711342564664,6.6364985663511,-5.69146113930635)) ;
#105700=CARTESIAN_POINT('Ctrl Pts',(8.52634316954116,6.63702130866459,-5.69051546490281)) ;
#105701=CARTESIAN_POINT('Ctrl Pts',(8.52557615349968,6.63751985710295,-5.68955571931119)) ;
#105702=CARTESIAN_POINT('Ctrl Pts',(8.52481401823429,6.63799287689814,-5.68858032616127)) ;
#105703=CARTESIAN_POINT('Ctrl Pts',(8.5246071083582,6.63812129566007,-5.68831551952531)) ;
#105704=CARTESIAN_POINT('Ctrl Pts',(8.52440075574004,6.63824801482192,-5.68804975390226)) ;
#105705=CARTESIAN_POINT('Ctrl Pts',(8.5241950281087,6.63837284070829,-5.68778308608104)) ;
#105706=CARTESIAN_POINT('Ctrl Pts',(8.52404824365684,6.63846190263542,-5.68759282145926)) ;
#105707=CARTESIAN_POINT('Ctrl Pts',(8.52390173612804,6.63855002749203,-5.68740204373474)) ;
#105708=CARTESIAN_POINT('Ctrl Pts',(8.52375553261475,6.63863721305423,-5.68721076280486)) ;
#105709=CARTESIAN_POINT('Ctrl Pts',(8.5229420412716,6.63912232246441,-5.68614645609245)) ;
#105710=CARTESIAN_POINT('Ctrl Pts',(8.52213801365706,6.63957834748689,-5.68506653755637)) ;
#105711=CARTESIAN_POINT('Ctrl Pts',(8.52134774490511,6.64000494097979,-5.68397296144637)) ;
#105712=CARTESIAN_POINT('Ctrl Pts',(8.51876608595595,6.64139854145543,-5.68040045456944)) ;
#105713=CARTESIAN_POINT('Ctrl Pts',(8.51630176076719,6.64256282842068,-5.6766245667844)) ;
#105714=CARTESIAN_POINT('Ctrl Pts',(8.51404737801022,6.64354662431173,-5.67266875822867)) ;
#105715=CARTESIAN_POINT('Ctrl Pts',(8.51174271377018,6.64455236266853,-5.66862471979259)) ;
#105716=CARTESIAN_POINT('Ctrl Pts',(8.50965863261302,6.64536892721963,-5.66439377806961)) ;
#105717=CARTESIAN_POINT('Ctrl Pts',(8.50786496313902,6.64606338785378,-5.66004416548596)) ;
#105718=CARTESIAN_POINT('Ctrl Pts',(8.50767015284864,6.64613881316472,-5.65957175442987)) ;
#105719=CARTESIAN_POINT('Ctrl Pts',(8.50747873128293,6.64621281334902,-5.65909797368753)) ;
#105720=CARTESIAN_POINT('Ctrl Pts',(8.50729076020857,6.64628549377757,-5.65862293019382)) ;
#105721=CARTESIAN_POINT('Ctrl Pts',(8.50722027105568,6.64631274893828,-5.65844478888368)) ;
#105722=CARTESIAN_POINT('Ctrl Pts',(8.50715026706477,6.64633981850992,-5.65826647001924)) ;
#105723=CARTESIAN_POINT('Ctrl Pts',(8.50708075128541,6.64636670806329,-5.65808797935946)) ;
#105724=CARTESIAN_POINT('Ctrl Pts',(8.50659414082988,6.6465549349369,-5.65683854474099)) ;
#105725=CARTESIAN_POINT('Ctrl Pts',(8.50613147592891,6.64673434010344,-5.65558068375498)) ;
#105726=CARTESIAN_POINT('Ctrl Pts',(8.50569363751094,6.64690683932496,-5.65431642750228)) ;
#105727=CARTESIAN_POINT('Ctrl Pts',(8.5039543604021,6.64759207829661,-5.64929427350717)) ;
#105728=CARTESIAN_POINT('Ctrl Pts',(8.50258205288306,6.64816393978926,-5.64409155961505)) ;
#105729=CARTESIAN_POINT('Ctrl Pts',(8.50162662717143,6.64864720987502,-5.63880412474346)) ;
#105730=CARTESIAN_POINT('Ctrl Pts',(8.50156399248218,6.64867889153407,-5.63845749722853)) ;
#105731=CARTESIAN_POINT('Ctrl Pts',(8.50150313499579,6.64871019935924,-5.63811050751598)) ;
#105732=CARTESIAN_POINT('Ctrl Pts',(8.50144406283925,6.64874114271688,-5.63776318350201)) ;
#105733=CARTESIAN_POINT('Ctrl Pts',(8.50057491246572,6.64919642372276,-5.63265287749383)) ;
#105734=CARTESIAN_POINT('Ctrl Pts',(8.5000953730058,6.64957062705848,-5.62747132905128)) ;
#105735=CARTESIAN_POINT('Ctrl Pts',(8.50001293997571,6.64989933182545,-5.62231444354085)) ;
#105736=CARTESIAN_POINT('Ctrl Pts',(8.5000043087827,6.64993374902791,-5.621774489179)) ;
#105737=CARTESIAN_POINT('Ctrl Pts',(8.5,6.64996765698296,-5.62123481442829)) ;
#105738=CARTESIAN_POINT('Ctrl Pts',(8.5,6.65000108682384,-5.62069553610592)) ;
#105739=CARTESIAN_POINT('',(8.55245136877619,6.60097994372612,-5.72678011937962)) ;
#105740=CARTESIAN_POINT('Ctrl Pts',(8.55238056475491,6.60105295171776,-5.72688861549862)) ;
#105741=CARTESIAN_POINT('Ctrl Pts',(8.55170523171898,6.60308542368594,-5.72510226561458)) ;
#105742=CARTESIAN_POINT('Ctrl Pts',(8.55095829520339,6.60513808680191,-5.72336273482159)) ;
#105743=CARTESIAN_POINT('Ctrl Pts',(8.55012599030486,6.60719152980469,-5.72165444418067)) ;
#105744=CARTESIAN_POINT('Ctrl Pts',(8.54968322947853,6.60828389886601,-5.72074568565103)) ;
#105745=CARTESIAN_POINT('Ctrl Pts',(8.54921644930854,6.609375699953,-5.71984624912318)) ;
#105746=CARTESIAN_POINT('Ctrl Pts',(8.54872481267395,6.61045954913296,-5.71895574654947)) ;
#105747=CARTESIAN_POINT('Ctrl Pts',(8.54779539897818,6.61250851009545,-5.71727229737198)) ;
#105748=CARTESIAN_POINT('Ctrl Pts',(8.54677348694552,6.61453549290067,-5.71561559088624)) ;
#105749=CARTESIAN_POINT('Ctrl Pts',(8.5456536674855,6.61650711947,-5.71396531829168)) ;
#105750=CARTESIAN_POINT('',(8.55735473176751,6.58264207262433,-5.74495579736184)) ;
#105751=CARTESIAN_POINT('Ctrl Pts',(8.55735473168706,6.58264207302769,-5.74495579684439)) ;
#105752=CARTESIAN_POINT('Ctrl Pts',(8.55706916598059,6.58397660851249,-5.74322969337166)) ;
#105753=CARTESIAN_POINT('Ctrl Pts',(8.55678088122709,6.58528501693236,-5.74166210096059)) ;
#105754=CARTESIAN_POINT('Ctrl Pts',(8.55647408091827,6.58661569125868,-5.74017182325178)) ;
#105755=CARTESIAN_POINT('Ctrl Pts',(8.55614409617586,6.58804692262381,-5.73856892751883)) ;
#105756=CARTESIAN_POINT('Ctrl Pts',(8.55579261555195,6.58950524590085,-5.73705679501759)) ;
#105757=CARTESIAN_POINT('Ctrl Pts',(8.55539993844513,6.59102291080506,-5.73558756777962)) ;
#105758=CARTESIAN_POINT('Ctrl Pts',(8.55517214917315,6.59190329771233,-5.7347352792273)) ;
#105759=CARTESIAN_POINT('Ctrl Pts',(8.55493049881969,6.5928030828913,-5.73389839775413)) ;
#105760=CARTESIAN_POINT('Ctrl Pts',(8.55467134659054,6.59372113732125,-5.73307079464215)) ;
#105761=CARTESIAN_POINT('Ctrl Pts',(8.55434805237174,6.59486641664501,-5.73203835397032)) ;
#105762=CARTESIAN_POINT('Ctrl Pts',(8.55400737519031,6.59602723165029,-5.73103619819578)) ;
#105763=CARTESIAN_POINT('Ctrl Pts',(8.55365328858765,6.59718920061515,-5.73004521551328)) ;
#105764=CARTESIAN_POINT('Ctrl Pts',(8.55328167888689,6.59840867329803,-5.72900519091102)) ;
#105765=CARTESIAN_POINT('Ctrl Pts',(8.55289390107692,6.59963546460028,-5.7279736796763)) ;
#105766=CARTESIAN_POINT('Ctrl Pts',(8.55249886556662,6.60083562835454,-5.72690814943487)) ;
#105767=CARTESIAN_POINT('Ctrl Pts',(8.55248304763318,6.60088368507321,-5.72686548368458)) ;
#105768=CARTESIAN_POINT('Ctrl Pts',(8.5524672152281,6.60093179017218,-5.72682280673305)) ;
#105769=CARTESIAN_POINT('Ctrl Pts',(8.55245136877619,6.60097994372612,-5.72678011937962)) ;
#105770=CARTESIAN_POINT('Ctrl Pts',(8.56107669735261,6.56009388000089,-5.84238384722239)) ;
#105771=CARTESIAN_POINT('Ctrl Pts',(8.56115635543004,6.5597817052481,-5.84082073438328)) ;
#105772=CARTESIAN_POINT('Ctrl Pts',(8.56122592915387,6.55950119162287,-5.83925071298061)) ;
#105773=CARTESIAN_POINT('Ctrl Pts',(8.56128584055879,6.55925348717442,-5.83769339194866)) ;
#105774=CARTESIAN_POINT('Ctrl Pts',(8.56142626445293,6.55867290283846,-5.83404325081112)) ;
#105775=CARTESIAN_POINT('Ctrl Pts',(8.56152217534692,6.55825854507371,-5.83037563387743)) ;
#105776=CARTESIAN_POINT('Ctrl Pts',(8.56158081746989,6.55798577878939,-5.82667013542601)) ;
#105777=CARTESIAN_POINT('Ctrl Pts',(8.5615891784535,6.55794688875063,-5.82614181874374)) ;
#105778=CARTESIAN_POINT('Ctrl Pts',(8.56159677639836,6.5579108824123,-5.82561264525984)) ;
#105779=CARTESIAN_POINT('Ctrl Pts',(8.56160362608007,6.55787769947532,-5.82508246747188)) ;
#105780=CARTESIAN_POINT('Ctrl Pts',(8.56164117305277,6.55769580506315,-5.82217626368602)) ;
#105781=CARTESIAN_POINT('Ctrl Pts',(8.56164095204357,6.55766773657215,-5.81926401199649)) ;
#105782=CARTESIAN_POINT('Ctrl Pts',(8.56161306230089,6.55774920537472,-5.81636556725813)) ;
#105783=CARTESIAN_POINT('Ctrl Pts',(8.56157759693122,6.55785280336172,-5.81267982460765)) ;
#105784=CARTESIAN_POINT('Ctrl Pts',(8.56150275624661,6.55813669070952,-5.80900492802066)) ;
#105785=CARTESIAN_POINT('Ctrl Pts',(8.56141108129146,6.55856506509341,-5.80536329254776)) ;
#105786=CARTESIAN_POINT('Ctrl Pts',(8.56136615997221,6.55877497130415,-5.80357886768072)) ;
#105787=CARTESIAN_POINT('Ctrl Pts',(8.56131707129299,6.55902016312283,-5.80180167096828)) ;
#105788=CARTESIAN_POINT('Ctrl Pts',(8.56126585691693,6.55929956116443,-5.80003152546822)) ;
#105789=CARTESIAN_POINT('Ctrl Pts',(8.56116752027494,6.55983603289964,-5.79663267190947)) ;
#105790=CARTESIAN_POINT('Ctrl Pts',(8.56104954130217,6.56049109659201,-5.79325400757552)) ;
#105791=CARTESIAN_POINT('Ctrl Pts',(8.56091150449776,6.561291476258,-5.78983047102478)) ;
#105792=CARTESIAN_POINT('Ctrl Pts',(8.56080235670743,6.56192434857303,-5.7871234288615)) ;
#105793=CARTESIAN_POINT('Ctrl Pts',(8.56068045333715,6.56264902401855,-5.78438726668918)) ;
#105794=CARTESIAN_POINT('Ctrl Pts',(8.56054379825318,6.56349285586905,-5.7816234877209)) ;
#105795=CARTESIAN_POINT('Ctrl Pts',(8.56050762866483,6.56371619955872,-5.78089197635184)) ;
#105796=CARTESIAN_POINT('Ctrl Pts',(8.56047042218818,6.56394794674723,-5.78015879169821)) ;
#105797=CARTESIAN_POINT('Ctrl Pts',(8.5604321390176,6.56418871538693,-5.77942462347088)) ;
#105798=CARTESIAN_POINT('Ctrl Pts',(8.5602688746024,6.56521550994367,-5.77629365117944)) ;
#105799=CARTESIAN_POINT('Ctrl Pts',(8.56008532870547,6.56636514336257,-5.77326121493511)) ;
#105800=CARTESIAN_POINT('Ctrl Pts',(8.55988915918713,6.567626861518,-5.77047132766748)) ;
#105801=CARTESIAN_POINT('Ctrl Pts',(8.55964574654529,6.56919243680251,-5.76700955727607)) ;
#105802=CARTESIAN_POINT('Ctrl Pts',(8.55938661160133,6.57080906160856,-5.76373263405113)) ;
#105803=CARTESIAN_POINT('Ctrl Pts',(8.55911582090256,6.57246439798288,-5.76066721242798)) ;
#105804=CARTESIAN_POINT('Ctrl Pts',(8.55888928658551,6.57384919626718,-5.75810278463541)) ;
#105805=CARTESIAN_POINT('Ctrl Pts',(8.5586381350289,6.57544444689325,-5.7553653454313)) ;
#105806=CARTESIAN_POINT('Ctrl Pts',(8.55834707044209,6.57718152485387,-5.75266812582306)) ;
#105807=CARTESIAN_POINT('Ctrl Pts',(8.55828762047113,6.57753632320103,-5.75211721844838)) ;
#105808=CARTESIAN_POINT('Ctrl Pts',(8.55822651695171,6.5778969434578,-5.75156784657914)) ;
#105809=CARTESIAN_POINT('Ctrl Pts',(8.55816364958868,6.57826264684156,-5.75102157107932)) ;
#105810=CARTESIAN_POINT('Ctrl Pts',(8.55792499569723,6.57965091145832,-5.74894782776412)) ;
#105811=CARTESIAN_POINT('Ctrl Pts',(8.55766032614232,6.58110993502773,-5.74692131328785)) ;
#105812=CARTESIAN_POINT('Ctrl Pts',(8.55735473176751,6.58264207262433,-5.74495579736184)) ;
#105813=CARTESIAN_POINT('Origin',(8.49172374697018,6.65,-7.62)) ;
#105814=CARTESIAN_POINT('Origin',(8.49226931268683,6.63793757459679,-5.85298827163609)) ;
#105815=CARTESIAN_POINT('Ctrl Pts',(8.40188506081772,6.5500005341705,-5.59154583081534)) ;
#105816=CARTESIAN_POINT('Ctrl Pts',(8.50280744587447,6.54966497091134,-5.60519504075416)) ;
#105817=CARTESIAN_POINT('Ctrl Pts',(8.50109204799972,6.6519968718077,-5.60568045493985)) ;
#105818=CARTESIAN_POINT('Ctrl Pts',(8.39296932930804,6.55000052027914,-5.649675802422)) ;
#105819=CARTESIAN_POINT('Ctrl Pts',(8.49725036372775,6.54968051003378,-5.63691360268317)) ;
#105820=CARTESIAN_POINT('Ctrl Pts',(8.49665296516361,6.6493567231781,-5.63602471146354)) ;
#105821=CARTESIAN_POINT('Ctrl Pts',(8.41146079558552,6.55000052635931,-5.7096088846459)) ;
#105822=CARTESIAN_POINT('Ctrl Pts',(8.50278789772753,6.54967384197893,-5.66101435198054)) ;
#105823=CARTESIAN_POINT('Ctrl Pts',(8.50590954255548,6.65051247736752,-5.66442721209356)) ;
#105824=CARTESIAN_POINT('Ctrl Pts',(8.4574451591418,6.55000045243508,-5.76280219188218)) ;
#105825=CARTESIAN_POINT('Ctrl Pts',(8.52023811680814,6.54973725194865,-5.70163301582095)) ;
#105826=CARTESIAN_POINT('Ctrl Pts',(8.52891723073132,6.63643009777383,-5.69347516307825)) ;
#105827=CARTESIAN_POINT('Ctrl Pts',(8.46608867121686,6.55000043643008,-5.7711950991747)) ;
#105828=CARTESIAN_POINT('Ctrl Pts',(8.52334270167619,6.54974993059834,-5.7084702400789)) ;
#105829=CARTESIAN_POINT('Ctrl Pts',(8.53324349789233,6.63337968978889,-5.69822089130001)) ;
#105830=CARTESIAN_POINT('Ctrl Pts',(8.48465388181691,6.55000038323734,-5.78657631387441)) ;
#105831=CARTESIAN_POINT('Ctrl Pts',(8.53001210036432,6.54978938646817,-5.72512459512324)) ;
#105832=CARTESIAN_POINT('Ctrl Pts',(8.54253954944035,6.62323710347999,-5.70886314626898)) ;
#105833=CARTESIAN_POINT('Ctrl Pts',(8.49467048074916,6.55000035131511,-5.79348849446136)) ;
#105834=CARTESIAN_POINT('Ctrl Pts',(8.53347884787439,6.549811668825,-5.73305903115006)) ;
#105835=CARTESIAN_POINT('Ctrl Pts',(8.54755337534732,6.6171479354886,-5.71286768812636)) ;
#105836=CARTESIAN_POINT('Ctrl Pts',(8.5099793089401,6.55000022766094,-5.80338890278579)) ;
#105837=CARTESIAN_POINT('Ctrl Pts',(8.53869035159221,6.54988741100167,-5.75877423275484)) ;
#105838=CARTESIAN_POINT('Ctrl Pts',(8.55523846583764,6.59353839814626,-5.73352788310835)) ;
#105839=CARTESIAN_POINT('Ctrl Pts',(8.51532901080107,6.55000016113069,-5.80633896731928)) ;
#105840=CARTESIAN_POINT('Ctrl Pts',(8.54023459682687,6.54992340374045,-5.76848974838733)) ;
#105841=CARTESIAN_POINT('Ctrl Pts',(8.55790835982317,6.58082417519513,-5.741582308573)) ;
#105842=CARTESIAN_POINT('Ctrl Pts',(8.52186010906347,6.55000005932357,-5.81279275987727)) ;
#105843=CARTESIAN_POINT('Ctrl Pts',(8.54265823247975,6.5499732773141,-5.79793164411572)) ;
#105844=CARTESIAN_POINT('Ctrl Pts',(8.561217465186,6.56135337205721,-5.78458837007632)) ;
#105845=CARTESIAN_POINT('Ctrl Pts',(8.52354993939971,6.55000003603139,-5.81582426222795)) ;
#105846=CARTESIAN_POINT('Ctrl Pts',(8.54350769968241,6.54998394755847,-5.81142387320079)) ;
#105847=CARTESIAN_POINT('Ctrl Pts',(8.56214310615443,6.55689632415131,-5.8074501335627)) ;
#105848=CARTESIAN_POINT('Ctrl Pts',(8.5226846131811,6.55000004733863,-5.82178753041577)) ;
#105849=CARTESIAN_POINT('Ctrl Pts',(8.54305517585924,6.54997881410037,-5.83281341214)) ;
#105850=CARTESIAN_POINT('Ctrl Pts',(8.5615325917139,6.55906016573922,-5.84279018158066)) ;
#105851=CARTESIAN_POINT('Ctrl Pts',(8.52060566253926,6.55000006807331,-5.82441380654967)) ;
#105852=CARTESIAN_POINT('Ctrl Pts',(8.54195943530538,6.54996919659462,-5.84049457488593)) ;
#105853=CARTESIAN_POINT('Ctrl Pts',(8.560584416286,6.5630274236339,-5.85450792151382)) ;
#105854=CARTESIAN_POINT('Ctrl Pts',(8.51445291480386,6.55000012130567,-5.8312328149553)) ;
#105855=CARTESIAN_POINT('Ctrl Pts',(8.53868948987839,6.54994355920609,-5.85941918176749)) ;
#105856=CARTESIAN_POINT('Ctrl Pts',(8.55750149922674,6.57320954252657,-5.88118443530683)) ;
#105857=CARTESIAN_POINT('Ctrl Pts',(8.50953280296015,6.55000015625148,-5.83504794643728)) ;
#105858=CARTESIAN_POINT('Ctrl Pts',(8.5361628892097,6.54992588038506,-5.86776474852663)) ;
#105859=CARTESIAN_POINT('Ctrl Pts',(8.55504783006517,6.57989127253968,-5.89069931679286)) ;
#105860=CARTESIAN_POINT('Ctrl Pts',(8.49261655785714,6.55000026291039,-5.84849260656893)) ;
#105861=CARTESIAN_POINT('Ctrl Pts',(8.5277825145509,6.54986718408749,-5.89576916089473)) ;
#105862=CARTESIAN_POINT('Ctrl Pts',(8.54658667616931,6.60027178071332,-5.91935337574384)) ;
#105863=CARTESIAN_POINT('Ctrl Pts',(8.48022165824512,6.55000031608562,-5.85776853416037)) ;
#105864=CARTESIAN_POINT('Ctrl Pts',(8.52288681814166,6.54983437262025,-5.90745594892907)) ;
#105865=CARTESIAN_POINT('Ctrl Pts',(8.5404533945046,6.61042388759286,-5.92630199096054)) ;
#105866=CARTESIAN_POINT('Ctrl Pts',(8.46952991654791,6.55000035836672,-5.86909544621882)) ;
#105867=CARTESIAN_POINT('Ctrl Pts',(8.51900842894237,6.54980714069607,-5.92336768467695)) ;
#105868=CARTESIAN_POINT('Ctrl Pts',(8.53471369258715,6.61849392543707,-5.94138336844284)) ;
#105869=CARTESIAN_POINT('Origin',(8.4,6.65,-5.6206780018997)) ;
#105870=CARTESIAN_POINT('Ctrl Pts',(8.54848814460235,8.28374914930622,-4.32353717477989)) ;
#105871=CARTESIAN_POINT('Ctrl Pts',(8.55964225199693,8.27720012980426,-4.32496794832229)) ;
#105872=CARTESIAN_POINT('Ctrl Pts',(8.572140519951,8.27365818248462,-4.32574176255693)) ;
#105873=CARTESIAN_POINT('Ctrl Pts',(8.54519582228991,8.29111303851995,-4.34796037880762)) ;
#105874=CARTESIAN_POINT('Ctrl Pts',(8.55569959891143,8.2840691245988,-4.34803761744089)) ;
#105875=CARTESIAN_POINT('Ctrl Pts',(8.56757951573636,8.27991709749369,-4.34819163391188)) ;
#105876=CARTESIAN_POINT('Ctrl Pts',(8.54340782920288,8.28927570119137,-4.37382299312324)) ;
#105877=CARTESIAN_POINT('Ctrl Pts',(8.5535505383751,8.28232618564302,-4.37215464428977)) ;
#105878=CARTESIAN_POINT('Ctrl Pts',(8.5650784856842,8.27803412520748,-4.37113214305328)) ;
#105879=CARTESIAN_POINT('Ctrl Pts',(8.54340835145922,8.27841951799442,-4.39553501116171)) ;
#105880=CARTESIAN_POINT('Ctrl Pts',(8.55355093564017,8.27219257320284,-4.39242153876592)) ;
#105881=CARTESIAN_POINT('Ctrl Pts',(8.56507848521152,8.26835005667905,-4.39050028050403)) ;
#105882=CARTESIAN_POINT('Ctrl Pts',(8.54742026180266,8.27608084857565,-4.3943656412486)) ;
#105883=CARTESIAN_POINT('Ctrl Pts',(8.54754672558908,8.27683897030433,-4.39267457303653)) ;
#105884=CARTESIAN_POINT('Ctrl Pts',(8.54766225486892,8.27755642830995,-4.39096549730839)) ;
#105885=CARTESIAN_POINT('Ctrl Pts',(8.54776713596767,8.27823455672262,-4.38923501677756)) ;
#105886=CARTESIAN_POINT('Ctrl Pts',(8.54791712013337,8.27920430747291,-4.38676036041194)) ;
#105887=CARTESIAN_POINT('Ctrl Pts',(8.54806168001142,8.28008011045346,-4.38424633726772)) ;
#105888=CARTESIAN_POINT('Ctrl Pts',(8.54818998754192,8.28086237513951,-4.38171868385907)) ;
#105889=CARTESIAN_POINT('Ctrl Pts',(8.5482419492675,8.28117917511831,-4.38069503986677)) ;
#105890=CARTESIAN_POINT('Ctrl Pts',(8.54829140719362,8.28148078264966,-4.37966867429046)) ;
#105891=CARTESIAN_POINT('Ctrl Pts',(8.54833813644415,8.28176759858571,-4.3786396299773)) ;
#105892=CARTESIAN_POINT('Ctrl Pts',(8.54850061324771,8.28276485268192,-4.37506166052903)) ;
#105893=CARTESIAN_POINT('Ctrl Pts',(8.54863339756396,8.28360845633784,-4.37135012352888)) ;
#105894=CARTESIAN_POINT('Ctrl Pts',(8.54873421749658,8.28426438239345,-4.36761308675765)) ;
#105895=CARTESIAN_POINT('Ctrl Pts',(8.54878752953697,8.28461122607275,-4.36563699879419)) ;
#105896=CARTESIAN_POINT('Ctrl Pts',(8.54883168679926,8.28490640714038,-4.36365408207398)) ;
#105897=CARTESIAN_POINT('Ctrl Pts',(8.54886500248133,8.28515040605083,-4.3616818590297)) ;
#105898=CARTESIAN_POINT('Ctrl Pts',(8.54887385422351,8.28521523484357,-4.3611578532514)) ;
#105899=CARTESIAN_POINT('Ctrl Pts',(8.54888411330031,8.285275121517,-4.36063500919228)) ;
#105900=CARTESIAN_POINT('Ctrl Pts',(8.54889386083024,8.28533143086091,-4.36011208678616)) ;
#105901=CARTESIAN_POINT('Ctrl Pts',(8.54894969070932,8.28565394783545,-4.35711700034689)) ;
#105902=CARTESIAN_POINT('Ctrl Pts',(8.5489793513821,8.28586680424121,-4.35409863638292)) ;
#105903=CARTESIAN_POINT('Ctrl Pts',(8.54899968230028,8.28595875954338,-4.35106757780128)) ;
#105904=CARTESIAN_POINT('Ctrl Pts',(8.54900356561227,8.28597632348831,-4.3504886297174)) ;
#105905=CARTESIAN_POINT('Ctrl Pts',(8.54900713937599,8.28598945835117,-4.34990930880415)) ;
#105906=CARTESIAN_POINT('Ctrl Pts',(8.54901057288909,8.28599806377621,-4.34932984021852)) ;
#105907=CARTESIAN_POINT('Ctrl Pts',(8.54902784271198,8.28604134718936,-4.34641523947593)) ;
#105908=CARTESIAN_POINT('Ctrl Pts',(8.54901619593281,8.28598556136224,-4.34351577572171)) ;
#105909=CARTESIAN_POINT('Ctrl Pts',(8.54898431260111,8.28582669412323,-4.34060642867547)) ;
#105910=CARTESIAN_POINT('Ctrl Pts',(8.54893914418926,8.2856016304144,-4.33648482096958)) ;
#105911=CARTESIAN_POINT('Ctrl Pts',(8.54884805310403,8.28517290646443,-4.33237709996661)) ;
#105912=CARTESIAN_POINT('Ctrl Pts',(8.54869940582912,8.28455561418421,-4.32830707741367)) ;
#105913=CARTESIAN_POINT('Ctrl Pts',(8.54864697316336,8.28433787538052,-4.32687144980245)) ;
#105914=CARTESIAN_POINT('Ctrl Pts',(8.54858736435354,8.28409676597416,-4.32544083959233)) ;
#105915=CARTESIAN_POINT('Ctrl Pts',(8.54851996240544,8.28383343043593,-4.32401720308527)) ;
#105916=CARTESIAN_POINT('Origin',(8.4,6.65,-7.62)) ;
#105917=CARTESIAN_POINT('Origin',(8.4,6.65,-4.5393219981003)) ;
#105918=CARTESIAN_POINT('Origin',(8.49172374697018,6.65,-7.62)) ;
#105919=CARTESIAN_POINT('Origin',(8.49225485648112,6.63809817882833,-4.30700862835662)) ;
#105920=CARTESIAN_POINT('Origin',(8.6,4.35421736843756,-4.5397127088383)) ;
#105921=CARTESIAN_POINT('Origin',(8.6,6.66256607592813,-4.5397127088383)) ;
#105922=CARTESIAN_POINT('Ctrl Pts',(8.5013487493624,6.65217253603376,-4.55598525608077)) ;
#105923=CARTESIAN_POINT('Ctrl Pts',(8.50315244876574,6.54997127577019,-4.55658636925847)) ;
#105924=CARTESIAN_POINT('Ctrl Pts',(8.40269444133658,6.55000000392136,-4.57159649657583)) ;
#105925=CARTESIAN_POINT('Ctrl Pts',(8.4963175378395,6.64933701877085,-4.52501565239563)) ;
#105926=CARTESIAN_POINT('Ctrl Pts',(8.49707874924865,6.5499727017442,-4.52396122349841)) ;
#105927=CARTESIAN_POINT('Ctrl Pts',(8.39261127161987,6.55000000381175,-4.51255502081071)) ;
#105928=CARTESIAN_POINT('Ctrl Pts',(8.50556246021204,6.65075235208947,-4.4960110455015)) ;
#105929=CARTESIAN_POINT('Ctrl Pts',(8.50253957946693,6.54997202229481,-4.49964413045446)) ;
#105930=CARTESIAN_POINT('Ctrl Pts',(8.41103525938983,6.55000000386643,-4.45133834963453)) ;
#105931=CARTESIAN_POINT('Ctrl Pts',(8.52891970071471,6.63645479210449,-4.46652715848277)) ;
#105932=CARTESIAN_POINT('Ctrl Pts',(8.52027792490144,6.54997752826668,-4.45840493996111)) ;
#105933=CARTESIAN_POINT('Ctrl Pts',(8.4576425585103,6.5500000033157,-4.39739010158301)) ;
#105934=CARTESIAN_POINT('Ctrl Pts',(8.53324635448928,6.63340383613797,-4.46178206573816)) ;
#105935=CARTESIAN_POINT('Ctrl Pts',(8.52338394863778,6.54997861189313,-4.45157331389085)) ;
#105936=CARTESIAN_POINT('Ctrl Pts',(8.46627109069292,6.55000000319827,-4.38900474853269)) ;
#105937=CARTESIAN_POINT('Ctrl Pts',(8.54254332011239,6.62325922024825,-4.45114174821778)) ;
#105938=CARTESIAN_POINT('Ctrl Pts',(8.53005572430509,6.54998198465676,-4.43493264246801)) ;
#105939=CARTESIAN_POINT('Ctrl Pts',(8.48480454940901,6.55000000280808,-4.3736278088231)) ;
#105940=CARTESIAN_POINT('Ctrl Pts',(8.54755771953121,6.61716872587346,-4.44713854387719)) ;
#105941=CARTESIAN_POINT('Ctrl Pts',(8.53352383957147,6.54998388968238,-4.42700661491452)) ;
#105942=CARTESIAN_POINT('Ctrl Pts',(8.49480263348501,6.55000000257396,-4.36671727629915)) ;
#105943=CARTESIAN_POINT('Ctrl Pts',(8.5552440065103,6.59355301617591,-4.42648056989549)) ;
#105944=CARTESIAN_POINT('Ctrl Pts',(8.53873552501329,6.54999036710749,-4.40129485880948)) ;
#105945=CARTESIAN_POINT('Ctrl Pts',(8.51008526949052,6.55000000166752,-4.35677574941852)) ;
#105946=CARTESIAN_POINT('Ctrl Pts',(8.55791451833571,6.58083494429015,-4.41842706746372)) ;
#105947=CARTESIAN_POINT('Ctrl Pts',(8.54027978136633,6.54999344602542,-4.39157902883419)) ;
#105948=CARTESIAN_POINT('Ctrl Pts',(8.51542462880457,6.55000000118004,-4.35380634433862)) ;
#105949=CARTESIAN_POINT('Ctrl Pts',(8.5612242931934,6.5613575592924,-4.37541653896351)) ;
#105950=CARTESIAN_POINT('Ctrl Pts',(8.54270214007071,6.54999771321876,-4.36209990564428)) ;
#105951=CARTESIAN_POINT('Ctrl Pts',(8.52194436340204,6.55000000043436,-4.34726744367388)) ;
#105952=CARTESIAN_POINT('Ctrl Pts',(8.56215003896755,6.55689889598543,-4.35255134475617)) ;
#105953=CARTESIAN_POINT('Ctrl Pts',(8.54355112280983,6.54999862629018,-4.34858541402145)) ;
#105954=CARTESIAN_POINT('Ctrl Pts',(8.52363168464777,6.55000000026381,-4.34419376079453)) ;
#105955=CARTESIAN_POINT('Ctrl Pts',(8.56153943432815,6.55906352913392,-4.31720612379092)) ;
#105956=CARTESIAN_POINT('Ctrl Pts',(8.54309854033142,6.5499981870035,-4.32716316826848)) ;
#105957=CARTESIAN_POINT('Ctrl Pts',(8.52276767133745,6.5500000003466,-4.33816751318002)) ;
#105958=CARTESIAN_POINT('Ctrl Pts',(8.5605912372004,6.56303220640811,-4.30548694646253)) ;
#105959=CARTESIAN_POINT('Ctrl Pts',(8.54200379397877,6.54999736403672,-4.31947204706566)) ;
#105960=CARTESIAN_POINT('Ctrl Pts',(8.52069177703238,6.55000000049844,-4.33552134373608)) ;
#105961=CARTESIAN_POINT('Ctrl Pts',(8.5575081978017,6.5732178281489,-4.27880781453251)) ;
#105962=CARTESIAN_POINT('Ctrl Pts',(8.53873610184731,6.54999517041881,-4.30052685964291)) ;
#105963=CARTESIAN_POINT('Ctrl Pts',(8.5145479773404,6.55000000088831,-4.3286566308241)) ;
#105964=CARTESIAN_POINT('Ctrl Pts',(8.55505442469281,6.57990173798307,-4.26929267446125)) ;
#105965=CARTESIAN_POINT('Ctrl Pts',(8.53621107118181,6.54999365791211,-4.29217666040666)) ;
#105966=CARTESIAN_POINT('Ctrl Pts',(8.50963525726155,6.5500000011443,-4.32482618291572)) ;
#105967=CARTESIAN_POINT('Ctrl Pts',(8.55022399280471,6.59153973477783,-4.25293520591856)) ;
#105968=CARTESIAN_POINT('Ctrl Pts',(8.53156015545166,6.54999086985382,-4.27662116717936)) ;
#105969=CARTESIAN_POINT('Ctrl Pts',(8.49999539447557,6.55000000159032,-4.3171278236794)) ;
#105970=CARTESIAN_POINT('Ctrl Pts',(8.54779538881607,6.59665349532936,-4.24691619169831)) ;
#105971=CARTESIAN_POINT('Ctrl Pts',(8.52936575151138,6.54998957391998,-4.26999554735594)) ;
#105972=CARTESIAN_POINT('Ctrl Pts',(8.49512741158075,6.55000000178643,-4.31333641589864)) ;
#105973=CARTESIAN_POINT('Ctrl Pts',(8.54538355337154,6.60121171185025,-4.24167517448427)) ;
#105974=CARTESIAN_POINT('Ctrl Pts',(8.52733415536169,6.54998837980796,-4.26389835720996)) ;
#105975=CARTESIAN_POINT('Ctrl Pts',(8.49033880598513,6.55000000196131,-4.30944859709871)) ;
#105976=CARTESIAN_POINT('',(8.54582344182383,6.61635369861666,-4.44606365157292)) ;
#105977=CARTESIAN_POINT('Ctrl Pts',(8.54582344182383,6.61635369861666,-4.44606365157292)) ;
#105978=CARTESIAN_POINT('Ctrl Pts',(8.5449359516352,6.61793460914653,-4.4473940762099)) ;
#105979=CARTESIAN_POINT('Ctrl Pts',(8.54398448171071,6.61948114927953,-4.4487173928307)) ;
#105980=CARTESIAN_POINT('Ctrl Pts',(8.54296332801272,6.6209780844369,-4.45004073677983)) ;
#105981=CARTESIAN_POINT('Ctrl Pts',(8.53827263106763,6.62785429629763,-4.45611955276191)) ;
#105982=CARTESIAN_POINT('Ctrl Pts',(8.53198779426187,6.63349037496299,-4.46261156852438)) ;
#105983=CARTESIAN_POINT('Ctrl Pts',(8.5259873730411,6.63731070037229,-4.4700705892422)) ;
#105984=CARTESIAN_POINT('Ctrl Pts',(8.52000560405467,6.64111915034781,-4.47750642368737)) ;
#105985=CARTESIAN_POINT('Ctrl Pts',(8.51430181273566,6.64349626850742,-4.48603764730141)) ;
#105986=CARTESIAN_POINT('Ctrl Pts',(8.50998586672548,6.64522349213896,-4.49520098697005)) ;
#105987=CARTESIAN_POINT('Ctrl Pts',(8.50534188065424,6.64708199603772,-4.50506080025013)) ;
#105988=CARTESIAN_POINT('Ctrl Pts',(8.50212992821339,6.64824261275105,-4.51588754367484)) ;
#105989=CARTESIAN_POINT('Ctrl Pts',(8.50077314609738,6.64911992656046,-4.52682491191675)) ;
#105990=CARTESIAN_POINT('Ctrl Pts',(8.50025986706873,6.64945181977648,-4.53096258566768)) ;
#105991=CARTESIAN_POINT('Ctrl Pts',(8.50000017127793,6.64974165917873,-4.53514325510123)) ;
#105992=CARTESIAN_POINT('Ctrl Pts',(8.5000000000847,6.64999974464545,-4.53931786749562)) ;
#105993=CARTESIAN_POINT('',(8.55242393572496,6.60106172182542,-4.4332420987161)) ;
#105994=CARTESIAN_POINT('Ctrl Pts',(8.55241775170035,6.60106807917176,-4.43323281615442)) ;
#105995=CARTESIAN_POINT('Ctrl Pts',(8.55072388788562,6.60619026743357,-4.43772147695242)) ;
#105996=CARTESIAN_POINT('Ctrl Pts',(8.54858294048571,6.61143812822772,-4.44192692414484)) ;
#105997=CARTESIAN_POINT('Ctrl Pts',(8.54582344182383,6.61635369861666,-4.44606365157292)) ;
#105998=CARTESIAN_POINT('Ctrl Pts',(8.55635360773813,6.58637108369506,-4.4186323907338)) ;
#105999=CARTESIAN_POINT('Ctrl Pts',(8.55606387390183,6.58765239867385,-4.42011238280755)) ;
#106000=CARTESIAN_POINT('Ctrl Pts',(8.55575324501781,6.58896823902363,-4.42156594133364)) ;
#106001=CARTESIAN_POINT('Ctrl Pts',(8.55541196992767,6.5903724112751,-4.42304320494043)) ;
#106002=CARTESIAN_POINT('Ctrl Pts',(8.55524290008378,6.59106804711319,-4.42377505069948)) ;
#106003=CARTESIAN_POINT('Ctrl Pts',(8.5550663125072,6.59178496983024,-4.4245119588377)) ;
#106004=CARTESIAN_POINT('Ctrl Pts',(8.55488049708426,6.59252693597571,-4.42525627761904)) ;
#106005=CARTESIAN_POINT('Ctrl Pts',(8.55445908016385,6.59420966544518,-4.42694434270892)) ;
#106006=CARTESIAN_POINT('Ctrl Pts',(8.55403589309457,6.5958403790653,-4.42848837772246)) ;
#106007=CARTESIAN_POINT('Ctrl Pts',(8.55359592981647,6.59737680581848,-4.42990315623323)) ;
#106008=CARTESIAN_POINT('Ctrl Pts',(8.55324292160435,6.59860957066092,-4.43103831559198)) ;
#106009=CARTESIAN_POINT('Ctrl Pts',(8.55287861047124,6.59978201473819,-4.43209104250714)) ;
#106010=CARTESIAN_POINT('Ctrl Pts',(8.55248933155915,6.60087815532546,-4.43307712698674)) ;
#106011=CARTESIAN_POINT('Ctrl Pts',(8.55246754857565,6.6009394923555,-4.43313230557793)) ;
#106012=CARTESIAN_POINT('Ctrl Pts',(8.5524457495603,6.60100068203151,-4.43318729627852)) ;
#106013=CARTESIAN_POINT('Ctrl Pts',(8.55242393572496,6.60106172182542,-4.4332420987161)) ;
#106014=CARTESIAN_POINT('Ctrl Pts',(8.5,6.66256607592813,-4.5397127088383)) ;
#106015=CARTESIAN_POINT('Ctrl Pts',(8.5,6.66256607592813,-4.455)) ;
#106016=CARTESIAN_POINT('Ctrl Pts',(8.58356010126947,6.66256607592813,-4.44107331645509)) ;
#106017=CARTESIAN_POINT('Ctrl Pts',(8.5,6.6101130271982,-4.53971270726282)) ;
#106018=CARTESIAN_POINT('Ctrl Pts',(8.5,6.63245216822986,-4.4585572365994)) ;
#106019=CARTESIAN_POINT('Ctrl Pts',(8.5794176004298,6.63563981885127,-4.4417637332617)) ;
#106020=CARTESIAN_POINT('Ctrl Pts',(8.5,6.55934573373329,-4.51884690994274)) ;
#106021=CARTESIAN_POINT('Ctrl Pts',(8.5,6.60054351783565,-4.44808139582774)) ;
#106022=CARTESIAN_POINT('Ctrl Pts',(8.57705842698408,6.60987578993432,-4.43172752804771)) ;
#106023=CARTESIAN_POINT('Ctrl Pts',(8.5,6.52274941072028,-4.48225058927972)) ;
#106024=CARTESIAN_POINT('Ctrl Pts',(8.5,6.57873105977929,-4.42626894022071)) ;
#106025=CARTESIAN_POINT('Ctrl Pts',(8.57705842661295,6.59157413088145,-4.41342586911855)) ;
#106026=CARTESIAN_POINT('Origin',(8.49172374697003,1.4,-7.62)) ;
#106027=CARTESIAN_POINT('Origin',(8.49172374697003,1.4,-3.11785831296514)) ;
#106028=CARTESIAN_POINT('Origin',(8.49172374697002,1.4,-3.11785831296514)) ;
#106029=CARTESIAN_POINT('Origin',(8.49172374697003,1.4,-3.11785831296514)) ;
#106030=CARTESIAN_POINT('Ctrl Pts',(8.50816364570057,1.49863939238321,-3.11785831296512)) ;
#106031=CARTESIAN_POINT('Ctrl Pts',(8.51019246767907,1.4983012553868,-3.15292758407099)) ;
#106032=CARTESIAN_POINT('Ctrl Pts',(8.50816364570057,1.47636598119991,-3.18029201095831)) ;
#106033=CARTESIAN_POINT('Ctrl Pts',(8.97755831131119,1.42040694811478,-3.08994865115312)) ;
#106034=CARTESIAN_POINT('Ctrl Pts',(8.97879997398671,1.42020000433583,-3.12456667318282)) ;
#106035=CARTESIAN_POINT('Ctrl Pts',(8.97755831689154,1.39869563385789,-3.15169481695074)) ;
#106036=CARTESIAN_POINT('Ctrl Pts',(9.44698496305969,1.34216917282336,-3.06263137063073)) ;
#106037=CARTESIAN_POINT('Ctrl Pts',(9.44827639615875,1.34195393397299,-3.0967775286091)) ;
#106038=CARTESIAN_POINT('Ctrl Pts',(9.44698496887878,1.3209776491576,-3.12372298471085)) ;
#106039=CARTESIAN_POINT('Ctrl Pts',(9.91643989873053,1.26392668354489,-3.03583811982177)) ;
#106040=CARTESIAN_POINT('Ctrl Pts',(9.91830968165731,1.26361505305709,-3.06950934419701)) ;
#106041=CARTESIAN_POINT('Ctrl Pts',(9.91643989873053,1.24322097942674,-3.09630356419402)) ;
#106042=CARTESIAN_POINT('Origin',(9.9,1.16528729116168,-3.0358381198218)) ;
#106043=CARTESIAN_POINT('Origin',(9.9,1.16528729116168,-3.0358381198218)) ;
#106044=CARTESIAN_POINT('Origin',(-0.4,-3.36847777691809,-5.48)) ;
#106045=CARTESIAN_POINT('Origin',(-0.400000000000001,-3.36847777691809,
-5.48)) ;
#106046=CARTESIAN_POINT('Origin',(-0.4,-3.36847777691809,-5.48)) ;
#106047=CARTESIAN_POINT('Origin',(-0.400000000000001,-3.36847777691809,
-4.58)) ;
#106048=CARTESIAN_POINT('Origin',(-0.4,-3.36847777691809,-4.68)) ;
#106049=CARTESIAN_POINT('Origin',(-1.11032778078669,-3.36847777691809,-5.48)) ;
#106050=CARTESIAN_POINT('Origin',(0.4,-3.36847777691809,-5.48)) ;
#106051=CARTESIAN_POINT('Origin',(-0.400000000000001,-3.36847777691809,
-4.68)) ;
#106052=CARTESIAN_POINT('Origin',(-0.4,-3.36847777691809,-4.68)) ;
#106053=CARTESIAN_POINT('Origin',(0.400000000000001,-3.36847777691809,-5.48)) ;
#106054=CARTESIAN_POINT('Origin',(0.400000000000001,-3.36847777691809,-5.48)) ;
#106055=CARTESIAN_POINT('Origin',(1.5,-3.36847777691809,-4.68)) ;
#106056=CARTESIAN_POINT('Origin',(0.4,-3.36847777691809,-4.68)) ;
#106057=CARTESIAN_POINT('Origin',(0.4,-3.36847777691809,-4.58)) ;
#106058=CARTESIAN_POINT('Origin',(0.4,-3.36847777691809,-4.68)) ;
#106059=CARTESIAN_POINT('Origin',(0.4,-3.36847777691809,-4.68)) ;
#106060=CARTESIAN_POINT('Origin',(7.96847777691809,3.4,-5.48)) ;
#106061=CARTESIAN_POINT('Origin',(7.96847777691809,3.4,-5.48)) ;
#106062=CARTESIAN_POINT('Origin',(7.96847777691809,3.4,-5.48)) ;
#106063=CARTESIAN_POINT('Origin',(7.96847777691809,3.4,-4.58)) ;
#106064=CARTESIAN_POINT('Origin',(7.96847777691809,3.4,-4.68)) ;
#106065=CARTESIAN_POINT('Origin',(7.96847777691809,2.68967221921331,-5.48)) ;
#106066=CARTESIAN_POINT('Origin',(7.96847777691809,4.2,-5.48)) ;
#106067=CARTESIAN_POINT('Origin',(7.96847777691809,3.4,-4.68)) ;
#106068=CARTESIAN_POINT('Origin',(7.96847777691809,3.4,-4.68)) ;
#106069=CARTESIAN_POINT('Origin',(7.96847777691809,4.2,-5.48)) ;
#106070=CARTESIAN_POINT('Origin',(7.96847777691809,4.2,-5.48)) ;
#106071=CARTESIAN_POINT('Origin',(7.96847777691809,2.3,-4.68)) ;
#106072=CARTESIAN_POINT('Origin',(7.96847777691809,4.2,-4.68)) ;
#106073=CARTESIAN_POINT('Origin',(7.96847777691809,4.2,-4.58)) ;
#106074=CARTESIAN_POINT('Origin',(7.96847777691809,4.2,-4.68)) ;
#106075=CARTESIAN_POINT('Origin',(7.96847777691809,4.2,-4.68)) ;
#106076=CARTESIAN_POINT('Origin',(8.49172374697003,1.4,-7.62)) ;
#106077=CARTESIAN_POINT('Origin',(8.49172374697003,1.4,-7.04214168703487)) ;
#106078=CARTESIAN_POINT('Origin',(8.49172374697002,1.4,-7.04214168703487)) ;
#106079=CARTESIAN_POINT('Origin',(8.49172374697003,1.39999999999989,-7.04214168703472)) ;
#106080=CARTESIAN_POINT('Ctrl Pts',(8.50816364570058,1.47636598119991,-6.97970798904169)) ;
#106081=CARTESIAN_POINT('Ctrl Pts',(8.51019246767908,1.4983012553868,-7.00707241592901)) ;
#106082=CARTESIAN_POINT('Ctrl Pts',(8.50816364570058,1.49863939238321,-7.04214168703488)) ;
#106083=CARTESIAN_POINT('Ctrl Pts',(8.97755831689153,1.39869563385779,-7.00830518304914)) ;
#106084=CARTESIAN_POINT('Ctrl Pts',(8.97879997398671,1.42020000433583,-7.03543332681677)) ;
#106085=CARTESIAN_POINT('Ctrl Pts',(8.97755831131121,1.42040694811478,-7.07005134884647)) ;
#106086=CARTESIAN_POINT('Ctrl Pts',(9.44698496887879,1.32097764915769,-7.03627701528927)) ;
#106087=CARTESIAN_POINT('Ctrl Pts',(9.44827639615876,1.34195393397361,-7.063222471393)) ;
#106088=CARTESIAN_POINT('Ctrl Pts',(9.44698496305971,1.34216917282336,-7.09736862936899)) ;
#106089=CARTESIAN_POINT('Ctrl Pts',(9.91643989873053,1.24322097942674,-7.06369643580598)) ;
#106090=CARTESIAN_POINT('Ctrl Pts',(9.91830968165732,1.26361505305709,-7.09049065580299)) ;
#106091=CARTESIAN_POINT('Ctrl Pts',(9.91643989873053,1.26392668354489,-7.12416188017823)) ;
#106092=CARTESIAN_POINT('Origin',(9.9,1.16528729116168,-7.1241618801782)) ;
#106093=CARTESIAN_POINT('Origin',(9.9,1.16528729116168,-7.12416188017819)) ;
#106094=CARTESIAN_POINT('Origin',(8.48377223398316,8.2,-7.62)) ;
#106095=CARTESIAN_POINT('Origin',(8.48238054865791,8.20007133344167,-4.3331789312541)) ;
#106096=CARTESIAN_POINT('Ctrl Pts',(8.40201662970151,8.3,-4.56597597792137)) ;
#106097=CARTESIAN_POINT('Ctrl Pts',(8.50299337454953,8.3,-4.55267481126356)) ;
#106098=CARTESIAN_POINT('Ctrl Pts',(8.50100123624933,8.19773961376458,-4.55268884611771)) ;
#106099=CARTESIAN_POINT('Ctrl Pts',(8.39454129798956,8.3,-4.51449818135068)) ;
#106100=CARTESIAN_POINT('Ctrl Pts',(8.4969787523767,8.3,-4.52537411133468)) ;
#106101=CARTESIAN_POINT('Ctrl Pts',(8.49727262260754,8.20135231978537,-4.52506706396232)) ;
#106102=CARTESIAN_POINT('Ctrl Pts',(8.40820218948348,8.3,-4.46202536352427)) ;
#106103=CARTESIAN_POINT('Ctrl Pts',(8.49818669687006,8.3,-4.50247172780123)) ;
#106104=CARTESIAN_POINT('Ctrl Pts',(8.50412619268406,8.20300739730712,-4.50038841002479)) ;
#106105=CARTESIAN_POINT('Ctrl Pts',(8.4430413476632,8.3,-4.41099693308713)) ;
#106106=CARTESIAN_POINT('Ctrl Pts',(8.50894174387208,8.3,-4.46085505538057)) ;
#106107=CARTESIAN_POINT('Ctrl Pts',(8.52157716465941,8.21896555381606,-4.47016612665034)) ;
#106108=CARTESIAN_POINT('Ctrl Pts',(8.44963266995283,8.3,-4.40266783197822)) ;
#106109=CARTESIAN_POINT('Ctrl Pts',(8.51095981317517,8.3,-4.45374944048349)) ;
#106110=CARTESIAN_POINT('Ctrl Pts',(8.52487915500778,8.22226238914488,-4.46495161805187)) ;
#106111=CARTESIAN_POINT('Ctrl Pts',(8.46372306360152,8.3,-4.38695472631993)) ;
#106112=CARTESIAN_POINT('Ctrl Pts',(8.51547368264943,8.3,-4.43763279105593)) ;
#106113=CARTESIAN_POINT('Ctrl Pts',(8.53193863144478,8.23129792829966,-4.45331747838552)) ;
#106114=CARTESIAN_POINT('Ctrl Pts',(8.47128983770084,8.3,-4.37955862714639)) ;
#106115=CARTESIAN_POINT('Ctrl Pts',(8.51796237042372,8.3,-4.42924649491277)) ;
#106116=CARTESIAN_POINT('Ctrl Pts',(8.53572833262714,8.23677343862356,-4.44742958850775)) ;
#106117=CARTESIAN_POINT('Ctrl Pts',(8.48287565264706,8.3,-4.36873079483316)) ;
#106118=CARTESIAN_POINT('Ctrl Pts',(8.52168214469874,8.3,-4.41074351942997)) ;
#106119=CARTESIAN_POINT('Ctrl Pts',(8.54153766811345,8.25077321967989,-4.43204498710732)) ;
#106120=CARTESIAN_POINT('Ctrl Pts',(8.48680760428677,8.3,-4.365187297402)) ;
#106121=CARTESIAN_POINT('Ctrl Pts',(8.52287759291297,8.3,-4.40414350493168)) ;
#106122=CARTESIAN_POINT('Ctrl Pts',(8.54350322705384,8.25646917637541,-4.42626226660343)) ;
#106123=CARTESIAN_POINT('Ctrl Pts',(8.49230810302881,8.3,-4.35949534999551)) ;
#106124=CARTESIAN_POINT('Ctrl Pts',(8.52426411271137,8.3,-4.38856652463359)) ;
#106125=CARTESIAN_POINT('Ctrl Pts',(8.54627296401923,8.26866384868897,-4.40855256936158)) ;
#106126=CARTESIAN_POINT('Ctrl Pts',(8.49410170711667,8.3,-4.357526518934)) ;
#106127=CARTESIAN_POINT('Ctrl Pts',(8.52463604790914,8.3,-4.38240552536515)) ;
#106128=CARTESIAN_POINT('Ctrl Pts',(8.54716490137964,8.27360757863442,-4.40079595948255)) ;
#106129=CARTESIAN_POINT('Ctrl Pts',(8.49698869685298,8.3,-4.35307327880953)) ;
#106130=CARTESIAN_POINT('Ctrl Pts',(8.5252311891155,8.3,-4.36659293443832)) ;
#106131=CARTESIAN_POINT('Ctrl Pts',(8.54862931231183,8.28262305001771,-4.37784134927042)) ;
#106132=CARTESIAN_POINT('Ctrl Pts',(8.49798687771249,8.3,-4.35051652115659)) ;
#106133=CARTESIAN_POINT('Ctrl Pts',(8.52551930315387,8.3,-4.3569062760438)) ;
#106134=CARTESIAN_POINT('Ctrl Pts',(8.54912969489065,8.28574379441723,-4.36238189749325)) ;
#106135=CARTESIAN_POINT('Ctrl Pts',(8.49821791151748,8.3,-4.34257957093737)) ;
#106136=CARTESIAN_POINT('Ctrl Pts',(8.52559423327562,8.3,-4.33218912470485)) ;
#106137=CARTESIAN_POINT('Ctrl Pts',(8.54922875625408,8.28635135062007,-4.32323867004689)) ;
#106138=CARTESIAN_POINT('Ctrl Pts',(8.49537847603514,8.3,-4.33764691084577)) ;
#106139=CARTESIAN_POINT('Ctrl Pts',(8.5243933105344,8.3,-4.32147327498212)) ;
#106140=CARTESIAN_POINT('Ctrl Pts',(8.54781890418529,8.28040548672881,-4.30847179337202)) ;
#106141=CARTESIAN_POINT('Ctrl Pts',(8.48955273785442,8.3,-4.32891140345694)) ;
#106142=CARTESIAN_POINT('Ctrl Pts',(8.52168703568126,8.3,-4.30405258512816)) ;
#106143=CARTESIAN_POINT('Ctrl Pts',(8.54489815533715,8.27194212599122,-4.28616700770705)) ;
#106144=CARTESIAN_POINT('Ctrl Pts',(8.4862007719736,8.3,-4.32482630750477)) ;
#106145=CARTESIAN_POINT('Ctrl Pts',(8.52012703453234,8.3,-4.29710733289327)) ;
#106146=CARTESIAN_POINT('Ctrl Pts',(8.54324008387893,8.26788967346965,-4.27831423563835)) ;
#106147=CARTESIAN_POINT('Ctrl Pts',(8.48280151347419,8.3,-4.32079110964071)) ;
#106148=CARTESIAN_POINT('Ctrl Pts',(8.51858761497411,8.3,-4.2906520257852)) ;
#106149=CARTESIAN_POINT('Ctrl Pts',(8.54152015125555,8.26408224232383,-4.27133822503473)) ;
#106150=CARTESIAN_POINT('Origin',(8.4,8.2,-4.53792711014902)) ;
#106151=CARTESIAN_POINT('Origin',(8.4,8.2,-5.705)) ;
#106152=CARTESIAN_POINT('Origin',(8.4,8.2,-5.62207288985098)) ;
#106153=CARTESIAN_POINT('Ctrl Pts',(8.50101530037395,8.19768718256759,-5.60720177458148)) ;
#106154=CARTESIAN_POINT('Ctrl Pts',(8.50305639000875,8.3,-5.60721981135723)) ;
#106155=CARTESIAN_POINT('Ctrl Pts',(8.40204633857705,8.3,-5.59382020212539)) ;
#106156=CARTESIAN_POINT('Ctrl Pts',(8.49725464441629,8.20131038948434,-5.63486791190954)) ;
#106157=CARTESIAN_POINT('Ctrl Pts',(8.49701391805276,8.3,-5.63456094234022)) ;
#106158=CARTESIAN_POINT('Ctrl Pts',(8.39450526457597,8.3,-5.645363291071)) ;
#106159=CARTESIAN_POINT('Ctrl Pts',(8.50410935041313,8.20295267265876,-5.65957929681148)) ;
#106160=CARTESIAN_POINT('Ctrl Pts',(8.49820749521502,8.3,-5.65746433789065)) ;
#106161=CARTESIAN_POINT('Ctrl Pts',(8.40816401923481,8.3,-5.69791872904343)) ;
#106162=CARTESIAN_POINT('Ctrl Pts',(8.52158236570989,8.21893216789648,-5.68983004077579)) ;
#106163=CARTESIAN_POINT('Ctrl Pts',(8.50896456566523,8.3,-5.69912767838404)) ;
#106164=CARTESIAN_POINT('Ctrl Pts',(8.44304134766321,8.3,-5.74900306691287)) ;
#106165=CARTESIAN_POINT('Ctrl Pts',(8.5248849650705,8.22222991631198,-5.69504370617815)) ;
#106166=CARTESIAN_POINT('Ctrl Pts',(8.51098076140209,8.3,-5.70623311097626)) ;
#106167=CARTESIAN_POINT('Ctrl Pts',(8.44963266995283,8.3,-5.75733216802178)) ;
#106168=CARTESIAN_POINT('Ctrl Pts',(8.53194575580939,8.23126818558571,-5.70667573496657)) ;
#106169=CARTESIAN_POINT('Ctrl Pts',(8.51549074202139,8.3,-5.7223505031351)) ;
#106170=CARTESIAN_POINT('Ctrl Pts',(8.46372306360152,8.3,-5.77304527368007)) ;
#106171=CARTESIAN_POINT('Ctrl Pts',(8.53573618291038,8.23674548871784,-5.71256237702727)) ;
#106172=CARTESIAN_POINT('Ctrl Pts',(8.51797743940286,8.3,-5.73073746255862)) ;
#106173=CARTESIAN_POINT('Ctrl Pts',(8.47128983770083,8.3,-5.78044137285362)) ;
#106174=CARTESIAN_POINT('Ctrl Pts',(8.54154687836689,8.25075037830459,-5.72794513194553)) ;
#106175=CARTESIAN_POINT('Ctrl Pts',(8.52169408444525,8.3,-5.74924355434931)) ;
#106176=CARTESIAN_POINT('Ctrl Pts',(8.48287565264707,8.3,-5.79126920516684)) ;
#106177=CARTESIAN_POINT('Ctrl Pts',(8.54351297666182,8.25644859419425,-5.73372727801621)) ;
#106178=CARTESIAN_POINT('Ctrl Pts',(8.52288848488738,8.3,-5.75584473154881)) ;
#106179=CARTESIAN_POINT('Ctrl Pts',(8.48680760428677,8.3,-5.79481270259799)) ;
#106180=CARTESIAN_POINT('Ctrl Pts',(8.54628376412585,8.26864846827403,-5.75143762316011)) ;
#106181=CARTESIAN_POINT('Ctrl Pts',(8.52427341038692,8.3,-5.77142501704035)) ;
#106182=CARTESIAN_POINT('Ctrl Pts',(8.49230810302881,8.3,-5.80050465000449)) ;
#106183=CARTESIAN_POINT('Ctrl Pts',(8.54717611873858,8.2735944350094,-5.75919488371877)) ;
#106184=CARTESIAN_POINT('Ctrl Pts',(8.52464480444821,8.3,-5.77758733991419)) ;
#106185=CARTESIAN_POINT('Ctrl Pts',(8.49410170711667,8.3,-5.802473481066)) ;
#106186=CARTESIAN_POINT('Ctrl Pts',(8.54864126180655,8.28261417405722,-5.78215290612485)) ;
#106187=CARTESIAN_POINT('Ctrl Pts',(8.52523908688554,8.3,-5.7934032849063)) ;
#106188=CARTESIAN_POINT('Ctrl Pts',(8.49698869685298,8.3,-5.80692672119047)) ;
#106189=CARTESIAN_POINT('Ctrl Pts',(8.54914185487161,8.28573645090424,-5.79761528241614)) ;
#106190=CARTESIAN_POINT('Ctrl Pts',(8.52552693815804,8.3,-5.80309195201625)) ;
#106191=CARTESIAN_POINT('Ctrl Pts',(8.49798687771249,8.3,-5.80948347884342)) ;
#106192=CARTESIAN_POINT('Ctrl Pts',(8.54924094958849,8.28634430798884,-5.8367659475985)) ;
#106193=CARTESIAN_POINT('Ctrl Pts',(8.5256018120494,8.3,-5.82781375175316)) ;
#106194=CARTESIAN_POINT('Ctrl Pts',(8.49821791151748,8.3,-5.81742042906263)) ;
#106195=CARTESIAN_POINT('Ctrl Pts',(8.54783079466744,8.28039553911293,-5.85153480598126)) ;
#106196=CARTESIAN_POINT('Ctrl Pts',(8.52440147378977,8.3,-5.83853127543226)) ;
#106197=CARTESIAN_POINT('Ctrl Pts',(8.49537847603514,8.3,-5.82235308915424)) ;
#106198=CARTESIAN_POINT('Ctrl Pts',(8.54465883986932,8.27120119512635,-5.87575719470323)) ;
#106199=CARTESIAN_POINT('Ctrl Pts',(8.52145785975948,8.3,-5.85749027833005)) ;
#106200=CARTESIAN_POINT('Ctrl Pts',(8.48905244827037,8.3,-5.83183876471446)) ;
#106201=CARTESIAN_POINT('Ctrl Pts',(8.54267599402787,8.26648669506702,-5.88429499043038)) ;
#106202=CARTESIAN_POINT('Ctrl Pts',(8.51958784692424,8.3,-5.86526413214463)) ;
#106203=CARTESIAN_POINT('Ctrl Pts',(8.48503640902806,8.3,-5.83656859706595)) ;
#106204=CARTESIAN_POINT('Ctrl Pts',(8.54064021294344,8.26212437554838,-5.89220002982386)) ;
#106205=CARTESIAN_POINT('Ctrl Pts',(8.51779796763702,8.3,-5.87268951701513)) ;
#106206=CARTESIAN_POINT('Ctrl Pts',(8.48104783026778,8.3,-5.84128480749502)) ;
#106207=CARTESIAN_POINT('Origin',(8.48238054717179,8.20007132587459,-5.82682106738604)) ;
#106208=CARTESIAN_POINT('Origin',(8.48377223398316,8.2,-7.62)) ;
#106209=CARTESIAN_POINT('Ctrl Pts',(8.55305389383868,6.58518362856711,-9.49981637143289)) ;
#106210=CARTESIAN_POINT('Ctrl Pts',(8.56447181517253,6.58947636230805,-9.49552363769195)) ;
#106211=CARTESIAN_POINT('Ctrl Pts',(8.57705842661295,6.59157413088145,-9.49342586911855)) ;
#106212=CARTESIAN_POINT('Ctrl Pts',(8.553051025152,6.55898702014118,-9.47362045977747)) ;
#106213=CARTESIAN_POINT('Ctrl Pts',(8.56446969712854,6.56479854221785,-9.47084652309117)) ;
#106214=CARTESIAN_POINT('Ctrl Pts',(8.5770584270977,6.56766897765924,-9.46952071573475)) ;
#106215=CARTESIAN_POINT('Ctrl Pts',(8.55608440539074,6.54967077654143,-9.43347242603467)) ;
#106216=CARTESIAN_POINT('Ctrl Pts',(8.56803673427363,6.55578248257735,-9.43313112423485)) ;
#106217=CARTESIAN_POINT('Ctrl Pts',(8.58110225049763,6.55837193275,-9.43326484665045)) ;
#106218=CARTESIAN_POINT('Ctrl Pts',(8.56106007075017,6.56033186051355,-9.3969784615962)) ;
#106219=CARTESIAN_POINT('Ctrl Pts',(8.57385418571953,6.56560017282096,-9.39820388376167)) ;
#106220=CARTESIAN_POINT('Ctrl Pts',(8.58763814880121,6.56727264871055,-9.39859290569255)) ;
#106221=CARTESIAN_POINT('',(8.56104219912065,6.56017369985344,-9.39763385094441)) ;
#106222=CARTESIAN_POINT('',(8.55704445183394,6.5832097329571,-9.49483164119209)) ;
#106223=CARTESIAN_POINT('Ctrl Pts',(8.56104219912065,6.56017369985344,-9.39763385094441)) ;
#106224=CARTESIAN_POINT('Ctrl Pts',(8.56172006948825,6.55755272988493,-9.41050998342623)) ;
#106225=CARTESIAN_POINT('Ctrl Pts',(8.56178854742204,6.55691761311389,-9.42401886345913)) ;
#106226=CARTESIAN_POINT('Ctrl Pts',(8.56147572200372,6.55855061087387,-9.43707103715452)) ;
#106227=CARTESIAN_POINT('Ctrl Pts',(8.56116227470662,6.56018685493861,-9.45014915781355)) ;
#106228=CARTESIAN_POINT('Ctrl Pts',(8.5604843297899,6.56417103596015,-9.4631290791339)) ;
#106229=CARTESIAN_POINT('Ctrl Pts',(8.55945615587251,6.57017322470283,-9.47482221269648)) ;
#106230=CARTESIAN_POINT('Ctrl Pts',(8.55883284154061,6.5738119576086,-9.48191099175524)) ;
#106231=CARTESIAN_POINT('Ctrl Pts',(8.5580718554171,6.57823677723143,-9.48863504839527)) ;
#106232=CARTESIAN_POINT('Ctrl Pts',(8.55704487707427,6.58320791316498,-9.49483246211941)) ;
#106233=CARTESIAN_POINT('',(8.55635403291171,6.58636921675996,-9.4986302321744)) ;
#106234=CARTESIAN_POINT('Origin',(8.5442029138841,6.62817326403372,-9.46194115684657)) ;
#106235=CARTESIAN_POINT('',(8.57705842661295,6.59157413088145,-9.49342586911855)) ;
#106236=CARTESIAN_POINT('Origin',(8.6,6.52274941072028,-9.56225058927972)) ;
#106237=CARTESIAN_POINT('',(8.58355189313841,6.56397635572685,-9.422433776426)) ;
#106238=CARTESIAN_POINT('Origin',(8.59777129281774,6.65641294722022,-9.42088223593215)) ;
#106239=CARTESIAN_POINT('Ctrl Pts',(8.56104311409705,6.56017375480331,-9.3976348093723)) ;
#106240=CARTESIAN_POINT('Ctrl Pts',(8.56569547918967,6.5609490208508,-9.40312238616949)) ;
#106241=CARTESIAN_POINT('Ctrl Pts',(8.57049938306336,6.56176641478979,-9.40850925134749)) ;
#106242=CARTESIAN_POINT('Ctrl Pts',(8.5753889310572,6.56259599225629,-9.41378626613857)) ;
#106243=CARTESIAN_POINT('Ctrl Pts',(8.57808773793837,6.56305388107911,-9.41669893697199)) ;
#106244=CARTESIAN_POINT('Ctrl Pts',(8.58081254036868,6.5635152101042,-9.41957937936769)) ;
#106245=CARTESIAN_POINT('Ctrl Pts',(8.58355195315299,6.56397636517832,-9.4224336197205)) ;
#106246=CARTESIAN_POINT('Ctrl Pts',(8.5,8.35216169217141,-9.51240609825021)) ;
#106247=CARTESIAN_POINT('Ctrl Pts',(8.5,8.2900428850829,-9.48134669470595)) ;
#106248=CARTESIAN_POINT('Ctrl Pts',(8.56507848521152,8.26835005667906,-9.47050028050403)) ;
#106249=CARTESIAN_POINT('Ctrl Pts',(8.5,8.31945293993511,-9.57782359726851)) ;
#106250=CARTESIAN_POINT('Ctrl Pts',(8.5,8.2692201349117,-9.52299218879621)) ;
#106251=CARTESIAN_POINT('Ctrl Pts',(8.56507848601002,8.25199117628906,-9.50321804061861)) ;
#106252=CARTESIAN_POINT('Ctrl Pts',(8.5,8.24922766844411,-9.61971270685141)) ;
#106253=CARTESIAN_POINT('Ctrl Pts',(8.5,8.21777561643101,-9.54447736982289)) ;
#106254=CARTESIAN_POINT('Ctrl Pts',(8.57228151929421,8.21451202732351,-9.52295308011763)) ;
#106255=CARTESIAN_POINT('Ctrl Pts',(8.5,8.17221734381475,-9.61971270883831)) ;
#106256=CARTESIAN_POINT('Ctrl Pts',(8.5,8.17221734381475,-9.535)) ;
#106257=CARTESIAN_POINT('Ctrl Pts',(8.58356010126947,8.17221734381475,-9.52107331645509)) ;
#106258=CARTESIAN_POINT('',(8.50000000249538,8.20000280433619,-9.61790474363843)) ;
#106259=CARTESIAN_POINT('',(8.54742025481395,8.27608084305204,-9.47436566195595)) ;
#106260=CARTESIAN_POINT('Ctrl Pts',(8.50000000249538,8.20000280433619,-9.61790474363843)) ;
#106261=CARTESIAN_POINT('Ctrl Pts',(8.50000274011724,8.20154143765779,-9.60563544845108)) ;
#106262=CARTESIAN_POINT('Ctrl Pts',(8.50225788919788,8.20358050335012,-9.59326647497958)) ;
#106263=CARTESIAN_POINT('Ctrl Pts',(8.50614710304112,8.20657022673326,-9.58191598101389)) ;
#106264=CARTESIAN_POINT('Ctrl Pts',(8.51002595055128,8.20955198129041,-9.57059574072047)) ;
#106265=CARTESIAN_POINT('Ctrl Pts',(8.51564213392183,8.21362262975068,-9.56004613352066)) ;
#106266=CARTESIAN_POINT('Ctrl Pts',(8.52129493663065,8.21921832196825,-9.55062179223395)) ;
#106267=CARTESIAN_POINT('Ctrl Pts',(8.52933132065201,8.22717351408127,-9.53722354898551)) ;
#106268=CARTESIAN_POINT('Ctrl Pts',(8.53683691159804,8.23885362788864,-9.52566244344335)) ;
#106269=CARTESIAN_POINT('Ctrl Pts',(8.54097226482464,8.25011947738646,-9.51288116961709)) ;
#106270=CARTESIAN_POINT('Ctrl Pts',(8.54447125915462,8.25965170869904,-9.50206671140824)) ;
#106271=CARTESIAN_POINT('Ctrl Pts',(8.54617119150717,8.26873789958222,-9.48993961018965)) ;
#106272=CARTESIAN_POINT('Ctrl Pts',(8.54724932284106,8.27506683274844,-9.47656646025131)) ;
#106273=CARTESIAN_POINT('Ctrl Pts',(8.54730817192851,8.27541229338911,-9.47583649568633)) ;
#106274=CARTESIAN_POINT('Ctrl Pts',(8.5473651061662,8.27575037116516,-9.47510283260602)) ;
#106275=CARTESIAN_POINT('Ctrl Pts',(8.54742024083733,8.27608084608571,-9.47436567520734)) ;
#106276=CARTESIAN_POINT('',(8.56507848521152,8.26835005667905,-9.47050028050403)) ;
#106277=CARTESIAN_POINT('Origin',(8.6,8.3521616921714,-9.51240609825021)) ;
#106278=CARTESIAN_POINT('',(8.58356010126947,8.17221734381475,-9.52107331645509)) ;
#106279=CARTESIAN_POINT('Origin',(8.59670327708553,8.16883734299696,-9.42706896951949)) ;
#106280=CARTESIAN_POINT('',(8.5,8.17221734381475,-9.61971270883831)) ;
#106281=CARTESIAN_POINT('Origin',(8.6,8.17221734381475,-9.61971270883831)) ;
#106282=CARTESIAN_POINT('Origin',(8.5,8.16642648793215,-9.39710775449589)) ;
#106283=CARTESIAN_POINT('Origin',(2.9,3.8,-10.16)) ;
#106284=CARTESIAN_POINT('',(3.,2.4,-10.16)) ;
#106285=CARTESIAN_POINT('Origin',(3.,3.8,-10.16)) ;
#106286=CARTESIAN_POINT('',(2.9,2.3,-10.16)) ;
#106287=CARTESIAN_POINT('Origin',(2.9,2.4,-10.16)) ;
#106288=CARTESIAN_POINT('Origin',(2.9,3.8,-10.16)) ;
#106289=CARTESIAN_POINT('Origin',(1.35,3.8,-10.16)) ;
#106290=CARTESIAN_POINT('',(1.35,2.3,-10.16)) ;
#106291=CARTESIAN_POINT('Origin',(1.35,3.8,-10.16)) ;
#106292=CARTESIAN_POINT('',(1.25,2.2,-10.16)) ;
#106293=CARTESIAN_POINT('Origin',(1.35,2.2,-10.16)) ;
#106294=CARTESIAN_POINT('Origin',(1.25,3.8,-10.16)) ;
#106295=CARTESIAN_POINT('Origin',(13.9153543900904,1.02736587339764,-9.31)) ;
#106296=CARTESIAN_POINT('',(1.15,1.02736587339764,-9.41)) ;
#106297=CARTESIAN_POINT('',(1.15,0.931757800066529,-9.28068965517241)) ;
#106298=CARTESIAN_POINT('Origin',(1.15,1.02736587339764,-9.31)) ;
#106299=CARTESIAN_POINT('',(-0.900000000000002,1.02736587339765,-9.41)) ;
#106300=CARTESIAN_POINT('',(-1.,1.02736587339765,-9.41)) ;
#106301=CARTESIAN_POINT('',(-0.900000000000002,0.982644513847654,-9.39944271909999)) ;
#106302=CARTESIAN_POINT('Origin',(-0.900000000000002,1.02736587339765,-9.31)) ;
#106303=CARTESIAN_POINT('',(-0.900000000000002,0.93175780006653,-9.28068965517241)) ;
#106304=CARTESIAN_POINT('Origin',(-0.900000000000002,1.02736587339765,-9.31)) ;
#106305=CARTESIAN_POINT('',(13.9153543900904,0.931757800066525,-9.28068965517241)) ;
#106306=CARTESIAN_POINT('Origin',(13.9153543900904,1.02736587339764,-11.01)) ;
#106307=CARTESIAN_POINT('',(1.15,0.93175780006653,-11.0393103448276)) ;
#106308=CARTESIAN_POINT('',(1.15,1.02736587339765,-10.91)) ;
#106309=CARTESIAN_POINT('Origin',(1.15,1.02736587339765,-11.01)) ;
#106310=CARTESIAN_POINT('',(-0.900000000000002,0.931757800066531,-11.0393103448276)) ;
#106311=CARTESIAN_POINT('',(13.9153543900904,0.931757800066525,-11.0393103448276)) ;
#106312=CARTESIAN_POINT('',(-0.900000000000002,1.02736587339765,-10.91)) ;
#106313=CARTESIAN_POINT('Origin',(-0.900000000000002,1.02736587339765,-11.01)) ;
#106314=CARTESIAN_POINT('',(-1.,1.02736587339765,-10.91)) ;
#106315=CARTESIAN_POINT('Origin',(8.49172374697003,3.8,-10.16)) ;
#106316=CARTESIAN_POINT('',(8.49172374697003,1.47741935483871,-8.26115320609529)) ;
#106317=CARTESIAN_POINT('',(8.49172374697003,1.47741935483871,-12.0588467939047)) ;
#106318=CARTESIAN_POINT('Origin',(8.49172374697003,3.8,-10.16)) ;
#106319=CARTESIAN_POINT('',(8.50816364570057,1.47636598119991,-8.26029201095833)) ;
#106320=CARTESIAN_POINT('Origin',(8.49172374697003,1.4,-8.19785831296514)) ;
#106321=CARTESIAN_POINT('',(8.50816364570057,1.47636598119991,-12.0597079890417)) ;
#106322=CARTESIAN_POINT('Origin',(8.50816364570057,3.8,-10.16)) ;
#106323=CARTESIAN_POINT('Origin',(8.49172374697003,1.4,-12.1221416870349)) ;
#106324=CARTESIAN_POINT('Origin',(1.25,3.8,-10.16)) ;
#106325=CARTESIAN_POINT('',(1.25,2.3,-10.16)) ;
#106326=CARTESIAN_POINT('Origin',(13.9153543900904,3.8,-10.16)) ;
#106327=CARTESIAN_POINT('',(-0.900000000000002,1.47741935483872,-12.0588467939047)) ;
#106328=CARTESIAN_POINT('',(13.9153543900904,1.47741935483871,-12.0588467939047)) ;
#106329=CARTESIAN_POINT('Origin',(-0.900000000000001,3.8,-10.16)) ;
#106330=CARTESIAN_POINT('',(1.35,0.876327704607742,-10.8324137931035)) ;
#106331=CARTESIAN_POINT('Ctrl Pts',(1.35,0.876327704607742,-10.8324137931035)) ;
#106332=CARTESIAN_POINT('Ctrl Pts',(1.35,0.888571289407569,-10.8856492115953)) ;
#106333=CARTESIAN_POINT('Ctrl Pts',(1.32969623836296,0.902340613578954,
-10.9379295970213)) ;
#106334=CARTESIAN_POINT('Ctrl Pts',(1.25741074236298,0.924142973728496,
-11.0150150537158)) ;
#106335=CARTESIAN_POINT('Ctrl Pts',(1.20472523187106,0.93175780006653,-11.0393103448276)) ;
#106336=CARTESIAN_POINT('Ctrl Pts',(1.15,0.93175780006653,-11.0393103448276)) ;
#106337=CARTESIAN_POINT('',(1.35,0.876327704607742,-9.48758620689656)) ;
#106338=CARTESIAN_POINT('Origin',(1.35,3.8,-10.16)) ;
#106339=CARTESIAN_POINT('Ctrl Pts',(1.15,0.931757800066529,-9.28068965517241)) ;
#106340=CARTESIAN_POINT('Ctrl Pts',(1.20475877631964,0.931757800066529,
-9.28068965517241)) ;
#106341=CARTESIAN_POINT('Ctrl Pts',(1.2574100247738,0.924155896380522,-9.30493436088835)) ;
#106342=CARTESIAN_POINT('Ctrl Pts',(1.32987646938161,0.9022735155524,-9.3823125455279)) ;
#106343=CARTESIAN_POINT('Ctrl Pts',(1.35,0.888577265820266,-9.43432480281013)) ;
#106344=CARTESIAN_POINT('Ctrl Pts',(1.35,0.876327704607742,-9.48758620689656)) ;
#106345=CARTESIAN_POINT('',(-0.900000000000002,1.47741935483872,-8.26115320609529)) ;
#106346=CARTESIAN_POINT('Origin',(-0.900000000000001,3.8,-10.16)) ;
#106347=CARTESIAN_POINT('',(13.9153543900904,1.47741935483871,-8.26115320609529)) ;
#106348=CARTESIAN_POINT('Origin',(0.55,3.09772049281573E-17,-10.16)) ;
#106349=CARTESIAN_POINT('',(0.549999999999999,4.4,-9.71)) ;
#106350=CARTESIAN_POINT('',(0.549999999999999,4.4,-10.61)) ;
#106351=CARTESIAN_POINT('',(0.549999999999999,4.4,-10.16)) ;
#106352=CARTESIAN_POINT('',(0.55,4.04473197180486,-10.61)) ;
#106353=CARTESIAN_POINT('',(0.55,1.39397422176708E-16,-10.61)) ;
#106354=CARTESIAN_POINT('',(0.55,4.05997159067981,-10.56)) ;
#106355=CARTESIAN_POINT('Ctrl Pts',(0.549999999999999,4.04473197180486,
-10.61)) ;
#106356=CARTESIAN_POINT('Ctrl Pts',(0.549999999999999,4.04764757798806,
-10.6055648611277)) ;
#106357=CARTESIAN_POINT('Ctrl Pts',(0.549999999999999,4.05014503921306,
-10.6009481448659)) ;
#106358=CARTESIAN_POINT('Ctrl Pts',(0.549999999999999,4.0569489863933,-10.5856814456903)) ;
#106359=CARTESIAN_POINT('Ctrl Pts',(0.549999999999999,4.0599715906798,-10.5718214564414)) ;
#106360=CARTESIAN_POINT('Ctrl Pts',(0.549999999999999,4.0599715906798,-10.56)) ;
#106361=CARTESIAN_POINT('',(0.55,4.05997159067981,-9.76)) ;
#106362=CARTESIAN_POINT('',(0.55,4.05997159067981,-9.66)) ;
#106363=CARTESIAN_POINT('',(0.55,4.04473197181449,-9.71000000001465)) ;
#106364=CARTESIAN_POINT('Origin',(0.550034503802642,3.93869457791256,-9.76241602969578)) ;
#106365=CARTESIAN_POINT('',(0.55,6.35032701027224E-17,-9.71)) ;
#106366=CARTESIAN_POINT('Origin',(10.,7.8,-12.7)) ;
#106367=CARTESIAN_POINT('',(9.93162277660169,7.82279240779944,-12.7)) ;
#106368=CARTESIAN_POINT('',(8.51539501058484,8.29486832980505,-12.7)) ;
#106369=CARTESIAN_POINT('',(10.,7.8,-12.7)) ;
#106370=CARTESIAN_POINT('',(8.51540095511712,8.29487265903615,-10.9290607599342)) ;
#106371=CARTESIAN_POINT('',(8.51539501058484,8.29486832980505,-12.7)) ;
#106372=CARTESIAN_POINT('',(8.54856023413467,8.28398586203111,-10.9160080665656)) ;
#106373=CARTESIAN_POINT('Ctrl Pts',(8.51540095511712,8.29487265903615,-10.9290607599342)) ;
#106374=CARTESIAN_POINT('Ctrl Pts',(8.51716444659958,8.29428466923189,-10.9296424828188)) ;
#106375=CARTESIAN_POINT('Ctrl Pts',(8.51901954868166,8.29366521079575,-10.9299704508582)) ;
#106376=CARTESIAN_POINT('Ctrl Pts',(8.52087614409666,8.29304501946169,-10.9300725025784)) ;
#106377=CARTESIAN_POINT('Ctrl Pts',(8.52171779595217,8.29276386763785,-10.9301187657647)) ;
#106378=CARTESIAN_POINT('Ctrl Pts',(8.52256005861363,8.29248252453827,-10.930119087778)) ;
#106379=CARTESIAN_POINT('Ctrl Pts',(8.52339613191993,8.29220315552769,-10.9300794460141)) ;
#106380=CARTESIAN_POINT('Ctrl Pts',(8.5245631657957,8.29181319797643,-10.9300241120128)) ;
#106381=CARTESIAN_POINT('Ctrl Pts',(8.52573147766849,8.29142195356395,-10.9298930049957)) ;
#106382=CARTESIAN_POINT('Ctrl Pts',(8.52689074379091,8.29103442649364,-10.929691327086)) ;
#106383=CARTESIAN_POINT('Ctrl Pts',(8.52858695132695,8.29046740713167,-10.9293962373014)) ;
#106384=CARTESIAN_POINT('Ctrl Pts',(8.53026630212631,8.28992123633276,-10.9289439218143)) ;
#106385=CARTESIAN_POINT('Ctrl Pts',(8.53190117913125,8.28939883282065,-10.9283683729162)) ;
#106386=CARTESIAN_POINT('Ctrl Pts',(8.53241671440279,8.2892341002838,-10.9281868817357)) ;
#106387=CARTESIAN_POINT('Ctrl Pts',(8.53292790037789,8.28907155799426,-10.9279933975174)) ;
#106388=CARTESIAN_POINT('Ctrl Pts',(8.53343404910735,8.28891083250767,-10.9277898379553)) ;
#106389=CARTESIAN_POINT('Ctrl Pts',(8.5352968140817,8.28831931900686,-10.9270406834076)) ;
#106390=CARTESIAN_POINT('Ctrl Pts',(8.5371161216987,8.28774836357891,-10.9261310088335)) ;
#106391=CARTESIAN_POINT('Ctrl Pts',(8.53885192161978,8.28720494689878,-10.925061264748)) ;
#106392=CARTESIAN_POINT('Ctrl Pts',(8.54015925159107,8.28679566878774,-10.9242555794339)) ;
#106393=CARTESIAN_POINT('Ctrl Pts',(8.54141951580281,8.28640152775902,-10.9233597461918)) ;
#106394=CARTESIAN_POINT('Ctrl Pts',(8.54261761299018,8.28602171215282,-10.9223927107854)) ;
#106395=CARTESIAN_POINT('Ctrl Pts',(8.54427390694789,8.28549664098145,-10.9210558451977)) ;
#106396=CARTESIAN_POINT('Ctrl Pts',(8.54582756795257,8.28499592220795,-10.9195574336962)) ;
#106397=CARTESIAN_POINT('Ctrl Pts',(8.54719190273352,8.28456181678114,-10.9179139760523)) ;
#106398=CARTESIAN_POINT('Ctrl Pts',(8.54768505754694,8.28440490428155,-10.9173199290053)) ;
#106399=CARTESIAN_POINT('Ctrl Pts',(8.54815358395155,8.28425671205378,-10.9167074323076)) ;
#106400=CARTESIAN_POINT('Ctrl Pts',(8.54859369700693,8.284119365871,-10.9160788545618)) ;
#106401=CARTESIAN_POINT('',(8.56837597005373,8.27720399148446,-10.8925054212669)) ;
#106402=CARTESIAN_POINT('Ctrl Pts',(8.5485198670553,8.28382649282421,-10.9160140527758)) ;
#106403=CARTESIAN_POINT('Ctrl Pts',(8.55267891820639,8.28243778061536,-10.9105631273052)) ;
#106404=CARTESIAN_POINT('Ctrl Pts',(8.55701747195698,8.28096933708251,-10.9052590577814)) ;
#106405=CARTESIAN_POINT('Ctrl Pts',(8.56150853123466,8.27945301063649,-10.9001132102133)) ;
#106406=CARTESIAN_POINT('Ctrl Pts',(8.56331520072601,8.27884302075224,-10.8980431315896)) ;
#106407=CARTESIAN_POINT('Ctrl Pts',(8.56514663435538,8.27822544298231,-10.8959980022295)) ;
#106408=CARTESIAN_POINT('Ctrl Pts',(8.56700126712394,8.27760232477898,-10.8939757856585)) ;
#106409=CARTESIAN_POINT('Ctrl Pts',(8.56745273479657,8.27745064099026,-10.8934835235653)) ;
#106410=CARTESIAN_POINT('Ctrl Pts',(8.56790562999348,8.27729861980367,-10.8929951953627)) ;
#106411=CARTESIAN_POINT('Ctrl Pts',(8.56835731300612,8.27714712982918,-10.8925055965825)) ;
#106412=CARTESIAN_POINT('',(9.93162277660169,7.82279240779944,-11.1197127088383)) ;
#106413=CARTESIAN_POINT('',(9.98593528106273,7.80468823964576,-11.1287647929151)) ;
#106414=CARTESIAN_POINT('',(9.93162277660169,7.82279240779944,-12.7)) ;
#106415=CARTESIAN_POINT('Origin',(10.,6.8,-12.7)) ;
#106416=CARTESIAN_POINT('',(10.,6.8847127088383,-12.7)) ;
#106417=CARTESIAN_POINT('',(10.,7.72792407799439,-12.7)) ;
#106418=CARTESIAN_POINT('',(10.,6.8,-12.7)) ;
#106419=CARTESIAN_POINT('',(10.,7.72792407799439,-11.1197127088383)) ;
#106420=CARTESIAN_POINT('',(10.,7.72792407799439,-12.7)) ;
#106421=CARTESIAN_POINT('',(10.,6.8847127088383,-11.1197127088383)) ;
#106422=CARTESIAN_POINT('',(10.,6.8,-11.1197127088383)) ;
#106423=CARTESIAN_POINT('',(10.,6.8847127088383,-12.7)) ;
#106424=CARTESIAN_POINT('Origin',(8.5,6.55,-12.7)) ;
#106425=CARTESIAN_POINT('',(9.91643989873054,6.78607331645509,-11.1197127088383)) ;
#106426=CARTESIAN_POINT('',(8.58355805979355,6.56393854759964,-10.8975665415707)) ;
#106427=CARTESIAN_POINT('',(8.48442535909739,6.54740422651623,-10.8810436188994)) ;
#106428=CARTESIAN_POINT('',(8.56107669735261,6.5600938800009,-10.9223838472224)) ;
#106429=CARTESIAN_POINT('Ctrl Pts',(8.58354728038623,6.56400494118526,-10.8975667486351)) ;
#106430=CARTESIAN_POINT('Ctrl Pts',(8.57838853885701,6.56313097816979,-10.9029365696477)) ;
#106431=CARTESIAN_POINT('Ctrl Pts',(8.57330127946562,6.56225500583441,-10.9083881686566)) ;
#106432=CARTESIAN_POINT('Ctrl Pts',(8.56834297134819,6.56140899842965,-10.9139607837894)) ;
#106433=CARTESIAN_POINT('Ctrl Pts',(8.5658758707988,6.56098805134778,-10.9167335444832)) ;
#106434=CARTESIAN_POINT('Ctrl Pts',(8.56344049907318,6.56057499921404,-10.9195353033203)) ;
#106435=CARTESIAN_POINT('Ctrl Pts',(8.56104288133097,6.56017406260212,-10.9223650362459)) ;
#106436=CARTESIAN_POINT('',(8.50816305748499,6.55136011924236,-10.9373726221052)) ;
#106437=CARTESIAN_POINT('Ctrl Pts',(8.56125813732195,6.56020968955366,-10.9225506353537)) ;
#106438=CARTESIAN_POINT('Ctrl Pts',(8.55737139916546,6.55956189986091,-10.9272085994728)) ;
#106439=CARTESIAN_POINT('Ctrl Pts',(8.55306335190366,6.55884389198394,-10.9299674660865)) ;
#106440=CARTESIAN_POINT('Ctrl Pts',(8.54121332232485,6.55686888705414,-10.9365237407852)) ;
#106441=CARTESIAN_POINT('Ctrl Pts',(8.53496267037859,6.55582711172976,-10.9379613606703)) ;
#106442=CARTESIAN_POINT('Ctrl Pts',(8.52888665185255,6.55481444197543,-10.9392795539312)) ;
#106443=CARTESIAN_POINT('Ctrl Pts',(8.52471102104795,6.55411850350799,-10.9395977494013)) ;
#106444=CARTESIAN_POINT('Ctrl Pts',(8.52011475164576,6.55335245860763,-10.9397029599352)) ;
#106445=CARTESIAN_POINT('Ctrl Pts',(8.51754797133926,6.55292466188988,-10.939718645943)) ;
#106446=CARTESIAN_POINT('Ctrl Pts',(8.51248317870107,6.55208052978351,-10.9389638228623)) ;
#106447=CARTESIAN_POINT('Ctrl Pts',(8.51021540604929,6.55170256767488,-10.9383708961116)) ;
#106448=CARTESIAN_POINT('Ctrl Pts',(8.50816120922223,6.55136020153704,-10.9373764115261)) ;
#106449=CARTESIAN_POINT('',(8.50816364570071,6.55136060761679,-12.7)) ;
#106450=CARTESIAN_POINT('',(8.50816364570071,6.55136060761679,-12.7)) ;
#106451=CARTESIAN_POINT('',(9.91643989873054,6.78607331645509,-12.7)) ;
#106452=CARTESIAN_POINT('',(8.5,6.55,-12.7)) ;
#106453=CARTESIAN_POINT('',(9.91643989873054,6.78607331645509,-12.7)) ;
#106454=CARTESIAN_POINT('Origin',(10.,1.5,-12.7)) ;
#106455=CARTESIAN_POINT('',(-0.900000000000002,1.5,-12.1221416870349)) ;
#106456=CARTESIAN_POINT('',(8.49172374697003,1.5,-12.1221416870349)) ;
#106457=CARTESIAN_POINT('',(10.,1.5,-12.1221416870349)) ;
#106458=CARTESIAN_POINT('',(8.49172374697003,1.5,-12.7)) ;
#106459=CARTESIAN_POINT('',(8.49172374697003,1.5,-12.7)) ;
#106460=CARTESIAN_POINT('',(-0.900000000000001,1.5,-12.7)) ;
#106461=CARTESIAN_POINT('',(10.,1.5,-12.7)) ;
#106462=CARTESIAN_POINT('',(-0.900000000000002,1.5,-12.0861360284258)) ;
#106463=CARTESIAN_POINT('Origin',(10.,1.5,-12.7)) ;
#106464=CARTESIAN_POINT('',(8.49172374697003,1.5,-7.62)) ;
#106465=CARTESIAN_POINT('',(-0.900000000000001,1.5,-7.62)) ;
#106466=CARTESIAN_POINT('',(10.,1.5,-7.62)) ;
#106467=CARTESIAN_POINT('',(8.49172374697003,1.5,-8.19785831296513)) ;
#106468=CARTESIAN_POINT('',(8.49172374697003,1.5,-12.7)) ;
#106469=CARTESIAN_POINT('',(-0.900000000000002,1.5,-8.19785831296513)) ;
#106470=CARTESIAN_POINT('',(10.,1.5,-8.19785831296513)) ;
#106471=CARTESIAN_POINT('',(-0.900000000000001,1.5,-12.7)) ;
#106472=CARTESIAN_POINT('Origin',(10.,0.,-12.7)) ;
#106473=CARTESIAN_POINT('',(10.,0.1,-7.62)) ;
#106474=CARTESIAN_POINT('',(10.,1.16528729116168,-7.62)) ;
#106475=CARTESIAN_POINT('',(10.,0.,-7.62)) ;
#106476=CARTESIAN_POINT('',(10.,0.1,-12.7)) ;
#106477=CARTESIAN_POINT('',(10.,0.1,-12.7)) ;
#106478=CARTESIAN_POINT('',(10.,1.16528729116168,-12.7)) ;
#106479=CARTESIAN_POINT('',(10.,0.,-12.7)) ;
#106480=CARTESIAN_POINT('',(10.,1.16528729116168,-12.2041618801782)) ;
#106481=CARTESIAN_POINT('',(10.,1.16528729116168,-12.7)) ;
#106482=CARTESIAN_POINT('',(10.,1.16528729116168,-8.11583811982181)) ;
#106483=CARTESIAN_POINT('Origin',(10.,3.8,-10.16)) ;
#106484=CARTESIAN_POINT('',(10.,1.16528729116168,-12.7)) ;
#106485=CARTESIAN_POINT('Origin',(0.,0.,-12.7)) ;
#106486=CARTESIAN_POINT('',(8.48377223398316,8.3,-12.7)) ;
#106487=CARTESIAN_POINT('',(7.1,8.3,-12.7)) ;
#106488=CARTESIAN_POINT('',(8.5,8.3,-12.7)) ;
#106489=CARTESIAN_POINT('Origin',(8.48377223398316,8.2,-12.7)) ;
#106490=CARTESIAN_POINT('Origin',(9.9,7.72792407799439,-12.7)) ;
#106491=CARTESIAN_POINT('Origin',(9.9,6.8847127088383,-12.7)) ;
#106492=CARTESIAN_POINT('',(8.49172374697018,6.55,-12.7)) ;
#106493=CARTESIAN_POINT('Origin',(8.49172374697018,6.65,-12.7)) ;
#106494=CARTESIAN_POINT('',(-0.900000000000001,6.55,-12.7)) ;
#106495=CARTESIAN_POINT('',(1.25,6.55,-12.7)) ;
#106496=CARTESIAN_POINT('',(-1.,6.45,-12.7)) ;
#106497=CARTESIAN_POINT('Origin',(-0.9,6.45,-12.7)) ;
#106498=CARTESIAN_POINT('',(-1.,4.65,-12.7)) ;
#106499=CARTESIAN_POINT('',(-1.,3.46944695195362E-16,-12.7)) ;
#106500=CARTESIAN_POINT('',(-0.900000000000001,4.55,-12.7)) ;
#106501=CARTESIAN_POINT('Origin',(-0.900000000000001,4.65,-12.7)) ;
#106502=CARTESIAN_POINT('',(1.15,4.55,-12.7)) ;
#106503=CARTESIAN_POINT('',(1.57859836313889E-15,4.55,-12.7)) ;
#106504=CARTESIAN_POINT('',(1.25,4.45,-12.7)) ;
#106505=CARTESIAN_POINT('Origin',(1.15,4.45,-12.7)) ;
#106506=CARTESIAN_POINT('',(1.25,3.15,-12.7)) ;
#106507=CARTESIAN_POINT('',(1.25,1.5,-12.7)) ;
#106508=CARTESIAN_POINT('',(1.15,3.05,-12.7)) ;
#106509=CARTESIAN_POINT('Origin',(1.15,3.15,-12.7)) ;
#106510=CARTESIAN_POINT('',(-0.900000000000002,3.05,-12.7)) ;
#106511=CARTESIAN_POINT('',(1.05818132034585E-15,3.05,-12.7)) ;
#106512=CARTESIAN_POINT('',(-1.,2.95,-12.7)) ;
#106513=CARTESIAN_POINT('Origin',(-0.900000000000002,2.95,-12.7)) ;
#106514=CARTESIAN_POINT('',(-1.,1.6,-12.7)) ;
#106515=CARTESIAN_POINT('',(-1.,3.46944695195362E-16,-12.7)) ;
#106516=CARTESIAN_POINT('Origin',(-0.900000000000002,1.6,-12.7)) ;
#106517=CARTESIAN_POINT('',(8.50816364570057,1.49863939238321,-12.7)) ;
#106518=CARTESIAN_POINT('Origin',(8.49172374697003,1.4,-12.7)) ;
#106519=CARTESIAN_POINT('',(9.91643989873054,1.26392668354489,-12.7)) ;
#106520=CARTESIAN_POINT('',(10.,1.24999999999998,-12.7)) ;
#106521=CARTESIAN_POINT('Origin',(9.9,1.16528729116168,-12.7)) ;
#106522=CARTESIAN_POINT('',(9.9,0.,-12.7)) ;
#106523=CARTESIAN_POINT('Origin',(9.9,0.1,-12.7)) ;
#106524=CARTESIAN_POINT('',(-2.,0.,-12.7)) ;
#106525=CARTESIAN_POINT('',(-2.,0.,-12.7)) ;
#106526=CARTESIAN_POINT('',(-2.,7.55,-12.7)) ;
#106527=CARTESIAN_POINT('',(-2.,7.65,-12.7)) ;
#106528=CARTESIAN_POINT('',(-1.9,7.65,-12.7)) ;
#106529=CARTESIAN_POINT('Origin',(-1.9,7.55,-12.7)) ;
#106530=CARTESIAN_POINT('',(6.9,7.65,-12.7)) ;
#106531=CARTESIAN_POINT('',(7.,7.65,-12.7)) ;
#106532=CARTESIAN_POINT('',(7.,7.75,-12.7)) ;
#106533=CARTESIAN_POINT('Origin',(6.9,7.75,-12.7)) ;
#106534=CARTESIAN_POINT('',(7.,8.2,-12.7)) ;
#106535=CARTESIAN_POINT('',(7.,8.3,-12.7)) ;
#106536=CARTESIAN_POINT('Origin',(7.1,8.2,-12.7)) ;
#106537=CARTESIAN_POINT('Origin',(0.,0.,-7.62)) ;
#106538=CARTESIAN_POINT('',(9.93162277660169,7.82279240779944,-7.62)) ;
#106539=CARTESIAN_POINT('',(8.51539501058484,8.29486832980505,-7.62)) ;
#106540=CARTESIAN_POINT('',(10.,7.8,-7.62)) ;
#106541=CARTESIAN_POINT('',(8.48377223398316,8.3,-7.62)) ;
#106542=CARTESIAN_POINT('Origin',(8.48377223398316,8.2,-7.62)) ;
#106543=CARTESIAN_POINT('',(7.1,8.3,-7.62)) ;
#106544=CARTESIAN_POINT('',(8.5,8.3,-7.62)) ;
#106545=CARTESIAN_POINT('',(7.,8.2,-7.62)) ;
#106546=CARTESIAN_POINT('Origin',(7.1,8.2,-7.62)) ;
#106547=CARTESIAN_POINT('',(7.,7.75,-7.62)) ;
#106548=CARTESIAN_POINT('',(7.,8.3,-7.62)) ;
#106549=CARTESIAN_POINT('',(6.9,7.65,-7.62)) ;
#106550=CARTESIAN_POINT('Origin',(6.9,7.75,-7.62)) ;
#106551=CARTESIAN_POINT('',(-1.9,7.65,-7.62)) ;
#106552=CARTESIAN_POINT('',(7.,7.65,-7.62)) ;
#106553=CARTESIAN_POINT('',(-2.,7.55,-7.62)) ;
#106554=CARTESIAN_POINT('Origin',(-1.9,7.55,-7.62)) ;
#106555=CARTESIAN_POINT('',(-2.,0.,-7.62)) ;
#106556=CARTESIAN_POINT('',(-2.,7.65,-7.62)) ;
#106557=CARTESIAN_POINT('',(9.9,0.,-7.62)) ;
#106558=CARTESIAN_POINT('',(-2.,0.,-7.62)) ;
#106559=CARTESIAN_POINT('Origin',(9.9,0.1,-7.62)) ;
#106560=CARTESIAN_POINT('',(9.91643989873054,1.26392668354489,-7.62)) ;
#106561=CARTESIAN_POINT('Origin',(9.9,1.16528729116168,-7.62)) ;
#106562=CARTESIAN_POINT('',(8.50816364570057,1.49863939238321,-7.62)) ;
#106563=CARTESIAN_POINT('',(0.472972972972955,2.83783783783779,-7.62)) ;
#106564=CARTESIAN_POINT('Origin',(8.49172374697003,1.4,-7.62)) ;
#106565=CARTESIAN_POINT('',(-1.,1.6,-7.62)) ;
#106566=CARTESIAN_POINT('Origin',(-0.900000000000002,1.6,-7.62)) ;
#106567=CARTESIAN_POINT('',(-1.,2.95,-7.62)) ;
#106568=CARTESIAN_POINT('',(-1.,3.46944695195362E-16,-7.62)) ;
#106569=CARTESIAN_POINT('',(-0.900000000000002,3.05,-7.62)) ;
#106570=CARTESIAN_POINT('Origin',(-0.900000000000002,2.95,-7.62)) ;
#106571=CARTESIAN_POINT('',(1.15,3.05,-7.62)) ;
#106572=CARTESIAN_POINT('',(1.05818132034585E-15,3.05,-7.62)) ;
#106573=CARTESIAN_POINT('',(1.25,3.15,-7.62)) ;
#106574=CARTESIAN_POINT('Origin',(1.15,3.15,-7.62)) ;
#106575=CARTESIAN_POINT('',(1.25,4.45,-7.62)) ;
#106576=CARTESIAN_POINT('',(1.25,5.3,-7.62)) ;
#106577=CARTESIAN_POINT('',(1.15,4.55,-7.62)) ;
#106578=CARTESIAN_POINT('Origin',(1.15,4.45,-7.62)) ;
#106579=CARTESIAN_POINT('',(-0.900000000000001,4.55,-7.62)) ;
#106580=CARTESIAN_POINT('',(1.57859836313889E-15,4.55,-7.62)) ;
#106581=CARTESIAN_POINT('',(-1.,4.65,-7.62)) ;
#106582=CARTESIAN_POINT('Origin',(-0.900000000000001,4.65,-7.62)) ;
#106583=CARTESIAN_POINT('',(-1.,6.45,-7.62)) ;
#106584=CARTESIAN_POINT('',(-1.,3.46944695195362E-16,-7.62)) ;
#106585=CARTESIAN_POINT('',(-0.900000000000001,6.55,-7.62)) ;
#106586=CARTESIAN_POINT('Origin',(-0.9,6.45,-7.62)) ;
#106587=CARTESIAN_POINT('',(8.49172374697018,6.55,-7.62)) ;
#106588=CARTESIAN_POINT('',(1.25,6.55,-7.62)) ;
#106589=CARTESIAN_POINT('',(8.50816364570071,6.55136060761679,-7.62)) ;
#106590=CARTESIAN_POINT('Origin',(8.49172374697018,6.65,-7.62)) ;
#106591=CARTESIAN_POINT('',(9.91643989873054,6.78607331645509,-7.62)) ;
#106592=CARTESIAN_POINT('',(8.5,6.55,-7.62)) ;
#106593=CARTESIAN_POINT('',(10.,6.8847127088383,-7.62)) ;
#106594=CARTESIAN_POINT('Origin',(9.9,6.8847127088383,-7.62)) ;
#106595=CARTESIAN_POINT('',(10.,7.72792407799439,-7.62)) ;
#106596=CARTESIAN_POINT('',(10.,6.8,-7.62)) ;
#106597=CARTESIAN_POINT('Origin',(9.9,7.72792407799439,-7.62)) ;
#106598=CARTESIAN_POINT('Origin',(7.,7.65,-12.7)) ;
#106599=CARTESIAN_POINT('',(-1.9,7.65,-12.7)) ;
#106600=CARTESIAN_POINT('',(6.9,7.65,-12.7)) ;
#106601=CARTESIAN_POINT('Origin',(7.,8.3,-12.7)) ;
#106602=CARTESIAN_POINT('',(7.,7.75,-7.62)) ;
#106603=CARTESIAN_POINT('',(7.,8.2,-12.7)) ;
#106604=CARTESIAN_POINT('Origin',(8.5,8.3,-12.7)) ;
#106605=CARTESIAN_POINT('',(8.4,8.3,-10.702072889851)) ;
#106606=CARTESIAN_POINT('',(8.48377267093844,8.29999999999968,-10.9180525450042)) ;
#106607=CARTESIAN_POINT('Ctrl Pts',(8.4,8.3,-10.702072889851)) ;
#106608=CARTESIAN_POINT('Ctrl Pts',(8.40000007660114,8.3,-10.7192296501939)) ;
#106609=CARTESIAN_POINT('Ctrl Pts',(8.40222537906598,8.3,-10.7361962391145)) ;
#106610=CARTESIAN_POINT('Ctrl Pts',(8.40642689896089,8.3,-10.7526162565003)) ;
#106611=CARTESIAN_POINT('Ctrl Pts',(8.4108423802432,8.3,-10.7698724593116)) ;
#106612=CARTESIAN_POINT('Ctrl Pts',(8.41744096860975,8.3,-10.7865267443636)) ;
#106613=CARTESIAN_POINT('Ctrl Pts',(8.42598957610198,8.3,-10.8021622007235)) ;
#106614=CARTESIAN_POINT('Ctrl Pts',(8.42927578125679,8.3,-10.8081726904243)) ;
#106615=CARTESIAN_POINT('Ctrl Pts',(8.43285067318485,8.3,-10.8140324469597)) ;
#106616=CARTESIAN_POINT('Ctrl Pts',(8.43670279785317,8.3,-10.8197167867854)) ;
#106617=CARTESIAN_POINT('Ctrl Pts',(8.43684245837178,8.3,-10.8199228750916)) ;
#106618=CARTESIAN_POINT('Ctrl Pts',(8.43698247939112,8.3,-10.8201287268225)) ;
#106619=CARTESIAN_POINT('Ctrl Pts',(8.43712286024714,8.3,-10.8203343406941)) ;
#106620=CARTESIAN_POINT('Ctrl Pts',(8.4430409279857,8.3,-10.8290024515356)) ;
#106621=CARTESIAN_POINT('Ctrl Pts',(8.44963232699551,8.300000000002,-10.8373317313645)) ;
#106622=CARTESIAN_POINT('Ctrl Pts',(8.45667836512368,8.29999999999776,-10.8451882739642)) ;
#106623=CARTESIAN_POINT('Ctrl Pts',(8.46347186896913,8.29999999999368,-10.8527632333091)) ;
#106624=CARTESIAN_POINT('Ctrl Pts',(8.47075094334182,8.29999999998296,-10.8599098655153)) ;
#106625=CARTESIAN_POINT('Ctrl Pts',(8.47818849074308,8.29999999991001,-10.8668816128285)) ;
#106626=CARTESIAN_POINT('Ctrl Pts',(8.47846436286148,8.2999999999073,-10.8671402075771)) ;
#106627=CARTESIAN_POINT('Ctrl Pts',(8.47874045306876,8.29999999990447,-10.8673985605991)) ;
#106628=CARTESIAN_POINT('Ctrl Pts',(8.47901674447045,8.29999999990152,-10.8676566852)) ;
#106629=CARTESIAN_POINT('Ctrl Pts',(8.48287938578321,8.29999999986032,-10.8712653488833)) ;
#106630=CARTESIAN_POINT('Ctrl Pts',(8.4868120552941,8.29999999978804,-10.8748079367278)) ;
#106631=CARTESIAN_POINT('Ctrl Pts',(8.49047938959117,8.29999999977837,-10.8786027060218)) ;
#106632=CARTESIAN_POINT('Ctrl Pts',(8.49231307405274,8.29999999977353,-10.8805001085834)) ;
#106633=CARTESIAN_POINT('Ctrl Pts',(8.49410676862313,8.29999999978935,-10.882469327125)) ;
#106634=CARTESIAN_POINT('Ctrl Pts',(8.49555027122445,8.29999999981726,-10.8846968070099)) ;
#106635=CARTESIAN_POINT('Ctrl Pts',(8.49675259850851,8.2999999998405,-10.8865521274215)) ;
#106636=CARTESIAN_POINT('Ctrl Pts',(8.49764594203226,8.29999999986456,-10.8886368157432)) ;
#106637=CARTESIAN_POINT('Ctrl Pts',(8.49795530287013,8.29999999987615,-10.8908110374494)) ;
#106638=CARTESIAN_POINT('Ctrl Pts',(8.49801735255452,8.29999999987847,-10.8912471293982)) ;
#106639=CARTESIAN_POINT('Ctrl Pts',(8.49805590844335,8.29999999988033,-10.891686822978)) ;
#106640=CARTESIAN_POINT('Ctrl Pts',(8.49806875158487,8.29999999988168,-10.8921289896614)) ;
#106641=CARTESIAN_POINT('Ctrl Pts',(8.49822249685463,8.2999999998978,-10.8974221678068)) ;
#106642=CARTESIAN_POINT('Ctrl Pts',(8.49538250015675,8.29999999989889,-10.9023553442684)) ;
#106643=CARTESIAN_POINT('Ctrl Pts',(8.49246863081132,8.29999999993393,-10.906722860551)) ;
#106644=CARTESIAN_POINT('Ctrl Pts',(8.48983292606215,8.29999999996562,-10.9106734437939)) ;
#106645=CARTESIAN_POINT('Ctrl Pts',(8.48683766317128,8.3,-10.9143922110698)) ;
#106646=CARTESIAN_POINT('Ctrl Pts',(8.48377316486176,8.3,-10.9180519562975)) ;
#106647=CARTESIAN_POINT('',(8.48377223398316,8.3,-12.7)) ;
#106648=CARTESIAN_POINT('',(7.1,8.3,-12.7)) ;
#106649=CARTESIAN_POINT('',(8.48377267093845,8.29999999999968,-9.40194745499578)) ;
#106650=CARTESIAN_POINT('',(8.48377223398316,8.3,-12.7)) ;
#106651=CARTESIAN_POINT('',(8.4,8.3,-9.61792711014902)) ;
#106652=CARTESIAN_POINT('Ctrl Pts',(8.48377316486176,8.3,-9.40194804370243)) ;
#106653=CARTESIAN_POINT('Ctrl Pts',(8.48683766317131,8.3,-9.4056077889302)) ;
#106654=CARTESIAN_POINT('Ctrl Pts',(8.48983292606215,8.29999999996562,-9.40932655620614)) ;
#106655=CARTESIAN_POINT('Ctrl Pts',(8.49246863081132,8.29999999993393,-9.41327713944902)) ;
#106656=CARTESIAN_POINT('Ctrl Pts',(8.49538250015675,8.29999999989889,-9.41764465573158)) ;
#106657=CARTESIAN_POINT('Ctrl Pts',(8.49822249685462,8.2999999998978,-9.42257783219323)) ;
#106658=CARTESIAN_POINT('Ctrl Pts',(8.49806875158486,8.29999999988168,-9.42787101033858)) ;
#106659=CARTESIAN_POINT('Ctrl Pts',(8.49805590844334,8.29999999988033,-9.42831317702195)) ;
#106660=CARTESIAN_POINT('Ctrl Pts',(8.49801735255452,8.29999999987847,-9.42875287060182)) ;
#106661=CARTESIAN_POINT('Ctrl Pts',(8.49795530287013,8.29999999987615,-9.42918896255059)) ;
#106662=CARTESIAN_POINT('Ctrl Pts',(8.49764594190815,8.29999999986456,-9.43136318512906)) ;
#106663=CARTESIAN_POINT('Ctrl Pts',(8.49675259754385,8.2999999998405,-9.43344787406726)) ;
#106664=CARTESIAN_POINT('Ctrl Pts',(8.49555027122433,8.29999999981726,-9.43530319298998)) ;
#106665=CARTESIAN_POINT('Ctrl Pts',(8.49410676570212,8.29999999978935,-9.43753067738161)) ;
#106666=CARTESIAN_POINT('Ctrl Pts',(8.4923130692812,8.29999999977353,-9.439499896352)) ;
#106667=CARTESIAN_POINT('Ctrl Pts',(8.49047938958768,8.29999999977837,-9.44139729397482)) ;
#106668=CARTESIAN_POINT('Ctrl Pts',(8.48681202348067,8.29999999978804,-9.44519209617395)) ;
#106669=CARTESIAN_POINT('Ctrl Pts',(8.48287934332709,8.29999999986032,-9.4487346907302)) ;
#106670=CARTESIAN_POINT('Ctrl Pts',(8.47901674443308,8.29999999990152,-9.45234331475996)) ;
#106671=CARTESIAN_POINT('Ctrl Pts',(8.47874052296043,8.29999999990447,-9.45260137402811)) ;
#106672=CARTESIAN_POINT('Ctrl Pts',(8.4784645028431,8.2999999999073,-9.45285966135653)) ;
#106673=CARTESIAN_POINT('Ctrl Pts',(8.47818870097127,8.29999999991001,-9.4531181900299)) ;
#106674=CARTESIAN_POINT('Ctrl Pts',(8.47075185325581,8.29999999998296,-9.46008927532798)) ;
#106675=CARTESIAN_POINT('Ctrl Pts',(8.46347271757077,8.29999999998104,-9.467236821007)) ;
#106676=CARTESIAN_POINT('Ctrl Pts',(8.45667934899943,8.29999999998018,-9.4748126083154)) ;
#106677=CARTESIAN_POINT('Ctrl Pts',(8.44963335392747,8.29999999997929,-9.48267011810317)) ;
#106678=CARTESIAN_POINT('Ctrl Pts',(8.44304226791565,8.29999999996634,-9.49100025634497)) ;
#106679=CARTESIAN_POINT('Ctrl Pts',(8.43712466127421,8.29999999997622,-9.499666888942)) ;
#106680=CARTESIAN_POINT('Ctrl Pts',(8.43698358608697,8.29999999997646,-9.49987350065014)) ;
#106681=CARTESIAN_POINT('Ctrl Pts',(8.43684287437575,8.2999999999767,-9.50008035127934)) ;
#106682=CARTESIAN_POINT('Ctrl Pts',(8.43670252680327,8.29999999997696,-9.50028743949552)) ;
#106683=CARTESIAN_POINT('Ctrl Pts',(8.42665365624217,8.29999999999548,-9.51511493271403)) ;
#106684=CARTESIAN_POINT('Ctrl Pts',(8.41848789916333,8.29999999999779,-9.53113486319164)) ;
#106685=CARTESIAN_POINT('Ctrl Pts',(8.41242260582416,8.29999999999911,-9.54791805139679)) ;
#106686=CARTESIAN_POINT('Ctrl Pts',(8.40662497274209,8.30000000000037,-9.56396060065526)) ;
#106687=CARTESIAN_POINT('Ctrl Pts',(8.40274598945956,8.3,-9.58070219391593)) ;
#106688=CARTESIAN_POINT('Ctrl Pts',(8.40101973895731,8.3,-9.5977797883369)) ;
#106689=CARTESIAN_POINT('Ctrl Pts',(8.4003453349782,8.3,-9.60445158806471)) ;
#106690=CARTESIAN_POINT('Ctrl Pts',(8.40000003014814,8.3,-9.61117467303844)) ;
#106691=CARTESIAN_POINT('Ctrl Pts',(8.4,8.3,-9.61792711014901)) ;
#106692=CARTESIAN_POINT('',(8.4,8.3,-10.7436545563009)) ;
#106693=CARTESIAN_POINT('Origin',(10.,7.8,-12.7)) ;
#106694=CARTESIAN_POINT('',(8.56837722373804,8.27720759208727,-9.4274948832495)) ;
#106695=CARTESIAN_POINT('',(8.54843785958924,8.2838540468036,-9.4039803122607)) ;
#106696=CARTESIAN_POINT('Ctrl Pts',(8.56837722339832,8.27720759220056,-9.42749488336226)) ;
#106697=CARTESIAN_POINT('Ctrl Pts',(8.56792584473107,8.27735805175631,-9.42700469022775)) ;
#106698=CARTESIAN_POINT('Ctrl Pts',(8.56747319573485,8.27750893475505,-9.42651579326377)) ;
#106699=CARTESIAN_POINT('Ctrl Pts',(8.56702308739659,8.2776589708678,-9.42602430395872)) ;
#106700=CARTESIAN_POINT('Ctrl Pts',(8.56055949575605,8.27981350141465,-9.41896647833432)) ;
#106701=CARTESIAN_POINT('Ctrl Pts',(8.5543545977397,8.28188180075344,-9.41162839546916)) ;
#106702=CARTESIAN_POINT('Ctrl Pts',(8.54852002808959,8.28382665730347,-9.40398586635143)) ;
#106703=CARTESIAN_POINT('',(8.51539953939799,8.29486682020068,-9.39094033012292)) ;
#106704=CARTESIAN_POINT('Origin',(8.52916905055959,8.29027698314681,-9.41073447047856)) ;
#106705=CARTESIAN_POINT('',(8.51539501058484,8.29486832980505,-12.7)) ;
#106706=CARTESIAN_POINT('',(9.93162277660169,7.82279240779944,-9.2002872911617)) ;
#106707=CARTESIAN_POINT('',(9.93162277660169,7.82279240779944,-12.7)) ;
#106708=CARTESIAN_POINT('',(8.48593528106273,8.30468823964576,-9.44123520708485)) ;
#106709=CARTESIAN_POINT('Origin',(10.,6.8,-12.7)) ;
#106710=CARTESIAN_POINT('',(10.,6.8847127088383,-9.2002872911617)) ;
#106711=CARTESIAN_POINT('',(10.,7.72792407799439,-9.2002872911617)) ;
#106712=CARTESIAN_POINT('',(10.,7.8,-9.2002872911617)) ;
#106713=CARTESIAN_POINT('',(10.,7.72792407799439,-12.7)) ;
#106714=CARTESIAN_POINT('',(10.,6.8847127088383,-12.7)) ;
#106715=CARTESIAN_POINT('Origin',(8.5,6.55,-12.7)) ;
#106716=CARTESIAN_POINT('',(8.50816305748852,6.55136011924294,-9.38262737789189)) ;
#106717=CARTESIAN_POINT('Ctrl Pts',(8.5081612092262,6.5513602015377,-9.382623588472)) ;
#106718=CARTESIAN_POINT('Ctrl Pts',(8.50982330775211,6.55163721795868,-9.38181892781788)) ;
#106719=CARTESIAN_POINT('Ctrl Pts',(8.51162127657737,6.55193687942956,-9.38127902844107)) ;
#106720=CARTESIAN_POINT('Ctrl Pts',(8.51523682141479,6.5525394702358,-9.38057109233512)) ;
#106721=CARTESIAN_POINT('Ctrl Pts',(8.51710259142427,6.55285043190405,-9.38039346793926)) ;
#106722=CARTESIAN_POINT('Ctrl Pts',(8.52217030373287,6.55369505062214,-9.38023569112659)) ;
#106723=CARTESIAN_POINT('Ctrl Pts',(8.52587381749955,6.55431230291659,-9.38048388339446)) ;
#106724=CARTESIAN_POINT('Ctrl Pts',(8.53482421527996,6.55580403587999,-9.38172985018422)) ;
#106725=CARTESIAN_POINT('Ctrl Pts',(8.53952102462675,6.55658683673483,-9.38322044742373)) ;
#106726=CARTESIAN_POINT('Ctrl Pts',(8.54640674065816,6.5577344560734,-9.38636821224601)) ;
#106727=CARTESIAN_POINT('Ctrl Pts',(8.55013419152241,6.55835569858707,-9.38823673023074)) ;
#106728=CARTESIAN_POINT('Ctrl Pts',(8.55581906875222,6.55930317812537,-9.39204337543013)) ;
#106729=CARTESIAN_POINT('Ctrl Pts',(8.55861150732171,6.55976858455362,-9.39427755556342)) ;
#106730=CARTESIAN_POINT('Ctrl Pts',(8.56125821409731,6.56020970234955,-9.39744945665611)) ;
#106731=CARTESIAN_POINT('',(9.91643989873054,6.78607331645509,-9.2002872911617)) ;
#106732=CARTESIAN_POINT('',(9.98442535909739,6.79740422651623,-9.18895638110055)) ;
#106733=CARTESIAN_POINT('',(9.91643989873054,6.78607331645509,-12.7)) ;
#106734=CARTESIAN_POINT('',(8.50816364570071,6.55136060761679,-12.7)) ;
#106735=CARTESIAN_POINT('Origin',(1.25,6.55,-12.7)) ;
#106736=CARTESIAN_POINT('',(8.49172372711481,6.55000000000007,-10.9294558427306)) ;
#106737=CARTESIAN_POINT('',(8.49172374697018,6.55,-12.7)) ;
#106738=CARTESIAN_POINT('',(8.4,6.55,-10.7006780018997)) ;
#106739=CARTESIAN_POINT('Ctrl Pts',(8.49172374697018,6.55000000000105,-10.9294557456557)) ;
#106740=CARTESIAN_POINT('Ctrl Pts',(8.49606803673627,6.55000000001052,-10.9259505863269)) ;
#106741=CARTESIAN_POINT('Ctrl Pts',(8.50046735944503,6.54999999990302,-10.9225119042493)) ;
#106742=CARTESIAN_POINT('Ctrl Pts',(8.50920280475179,6.55000000136501,-10.9155160267021)) ;
#106743=CARTESIAN_POINT('Ctrl Pts',(8.51365366733341,6.55000000372466,-10.9120189182925)) ;
#106744=CARTESIAN_POINT('Ctrl Pts',(8.51786969589086,6.55000000840872,-10.907574051492)) ;
#106745=CARTESIAN_POINT('Ctrl Pts',(8.51824835575326,6.5500000088438,-10.9071628343558)) ;
#106746=CARTESIAN_POINT('Ctrl Pts',(8.51893753951067,6.55000000964298,-10.9063894122641)) ;
#106747=CARTESIAN_POINT('Ctrl Pts',(8.51925555226623,6.55000001000021,-10.9060246830609)) ;
#106748=CARTESIAN_POINT('Ctrl Pts',(8.52125362518914,6.55000001218547,-10.9036369664008)) ;
#106749=CARTESIAN_POINT('Ctrl Pts',(8.52280131776511,6.55000000862055,-10.9013625215737)) ;
#106750=CARTESIAN_POINT('Ctrl Pts',(8.52354796988914,6.55000000490364,-10.8962172682011)) ;
#106751=CARTESIAN_POINT('Ctrl Pts',(8.52233587755844,6.5500000056078,-10.8935629178231)) ;
#106752=CARTESIAN_POINT('Ctrl Pts',(8.52032554216538,6.55000000470579,-10.8911610105703)) ;
#106753=CARTESIAN_POINT('Ctrl Pts',(8.5200461874495,6.55000000456892,-10.8908554672244)) ;
#106754=CARTESIAN_POINT('Ctrl Pts',(8.51943244221702,6.55000000425258,-10.8902375575506)) ;
#106755=CARTESIAN_POINT('Ctrl Pts',(8.51910103101852,6.55000000405877,-10.8899172773213)) ;
#106756=CARTESIAN_POINT('Ctrl Pts',(8.51460799223802,6.5500000014124,-10.8857349310042)) ;
#106757=CARTESIAN_POINT('Ctrl Pts',(8.50969722522556,6.55000000036127,-10.8829602411529)) ;
#106758=CARTESIAN_POINT('Ctrl Pts',(8.50463600502755,6.55000000021577,-10.8796634748388)) ;
#106759=CARTESIAN_POINT('Ctrl Pts',(8.50427412871942,6.55000000020764,-10.8794272801265)) ;
#106760=CARTESIAN_POINT('Ctrl Pts',(8.49410349041847,6.55000000002642,-10.8727743312815)) ;
#106761=CARTESIAN_POINT('Ctrl Pts',(8.48448997361521,6.54999999999179,-10.8660809389623)) ;
#106762=CARTESIAN_POINT('Ctrl Pts',(8.46629237463078,6.55000000001684,-10.8509770243887)) ;
#106763=CARTESIAN_POINT('Ctrl Pts',(8.45766562693773,6.55000000000151,-10.8425939316618)) ;
#106764=CARTESIAN_POINT('Ctrl Pts',(8.44955830666693,6.54999999999999,-10.8332123342681)) ;
#106765=CARTESIAN_POINT('Ctrl Pts',(8.4493708101522,6.54999999999999,-10.8329944283116)) ;
#106766=CARTESIAN_POINT('Ctrl Pts',(8.43720071044502,6.5500000000026,-10.8187892740227)) ;
#106767=CARTESIAN_POINT('Ctrl Pts',(8.427213843659,6.55000000009149,-10.8032566681918)) ;
#106768=CARTESIAN_POINT('Ctrl Pts',(8.41184903642503,6.55000000007035,-10.7705950553225)) ;
#106769=CARTESIAN_POINT('Ctrl Pts',(8.40635547808451,6.5500000000232,-10.7535173325337)) ;
#106770=CARTESIAN_POINT('Ctrl Pts',(8.40108598764611,6.5499999999995,-10.7243588087582)) ;
#106771=CARTESIAN_POINT('Ctrl Pts',(8.4,6.55,-10.7125595279398)) ;
#106772=CARTESIAN_POINT('Ctrl Pts',(8.4,6.55,-10.7006780018997)) ;
#106773=CARTESIAN_POINT('',(8.4,6.55,-9.6193219981003)) ;
#106774=CARTESIAN_POINT('',(8.4,6.55,-9.43636060761679)) ;
#106775=CARTESIAN_POINT('',(8.4917237271148,6.5500000000004,-9.39054415726839)) ;
#106776=CARTESIAN_POINT('Ctrl Pts',(8.4,6.55,-9.6193219981003)) ;
#106777=CARTESIAN_POINT('Ctrl Pts',(8.4,6.55,-9.60146035159508)) ;
#106778=CARTESIAN_POINT('Ctrl Pts',(8.40245177849645,6.55000000000111,-9.58378505809112)) ;
#106779=CARTESIAN_POINT('Ctrl Pts',(8.40709634751483,6.55000000003438,-9.56675184875779)) ;
#106780=CARTESIAN_POINT('Ctrl Pts',(8.41193897064549,6.55000000006908,-9.54899230784436)) ;
#106781=CARTESIAN_POINT('Ctrl Pts',(8.41916594308043,6.55000000013771,-9.53192888814512)) ;
#106782=CARTESIAN_POINT('Ctrl Pts',(8.42853896333499,6.55000000013582,-9.51608126731972)) ;
#106783=CARTESIAN_POINT('Ctrl Pts',(8.434550587058,6.55000000013461,-9.50591699468187)) ;
#106784=CARTESIAN_POINT('Ctrl Pts',(8.44144611055218,6.55000000009671,-9.49625300072306)) ;
#106785=CARTESIAN_POINT('Ctrl Pts',(8.44917210140205,6.55000000005186,-9.48723268310166)) ;
#106786=CARTESIAN_POINT('Ctrl Pts',(8.44936219523638,6.55000000005075,-9.4870107430558)) ;
#106787=CARTESIAN_POINT('Ctrl Pts',(8.44955278293316,6.55000000004968,-9.48678920228628)) ;
#106788=CARTESIAN_POINT('Ctrl Pts',(8.44974386351697,6.55000000004864,-9.48656806301675)) ;
#106789=CARTESIAN_POINT('Ctrl Pts',(8.45766118910685,6.55000000000559,-9.47740527126339)) ;
#106790=CARTESIAN_POINT('Ctrl Pts',(8.46628870646479,6.54999999999864,-9.46902155150326)) ;
#106791=CARTESIAN_POINT('Ctrl Pts',(8.47555348469885,6.55000000000007,-9.46133527594906)) ;
#106792=CARTESIAN_POINT('Ctrl Pts',(8.48448851770303,6.55000000000144,-9.45392256470859)) ;
#106793=CARTESIAN_POINT('Ctrl Pts',(8.49410273695376,6.5500000000304,-9.44723469297056)) ;
#106794=CARTESIAN_POINT('Ctrl Pts',(8.50391213313781,6.55000000016212,-9.4408238957712)) ;
#106795=CARTESIAN_POINT('Ctrl Pts',(8.50409415224108,6.55000000016456,-9.44070493966671)) ;
#106796=CARTESIAN_POINT('Ctrl Pts',(8.50427622716233,6.55000000016576,-9.44058605979316)) ;
#106797=CARTESIAN_POINT('Ctrl Pts',(8.50445835579895,6.55000000016577,-9.44046725463207)) ;
#106798=CARTESIAN_POINT('Ctrl Pts',(8.50464048443556,6.55000000016577,-9.44034844947097)) ;
#106799=CARTESIAN_POINT('Ctrl Pts',(8.50482266678753,6.55000000016459,-9.44022971902234)) ;
#106800=CARTESIAN_POINT('Ctrl Pts',(8.50500490075221,6.55000000016234,-9.44011106176768)) ;
#106801=CARTESIAN_POINT('Ctrl Pts',(8.50970297364421,6.55000000010443,-9.43705202481732)) ;
#106802=CARTESIAN_POINT('Ctrl Pts',(8.51460443926437,6.55000000028677,-9.43427565407059)) ;
#106803=CARTESIAN_POINT('Ctrl Pts',(8.5187483092633,6.55000000038295,-9.43043698472844)) ;
#106804=CARTESIAN_POINT('Ctrl Pts',(8.51909542442958,6.55000000039101,-9.43011543498211)) ;
#106805=CARTESIAN_POINT('Ctrl Pts',(8.51943721516333,6.55000000039358,-9.42978641450153)) ;
#106806=CARTESIAN_POINT('Ctrl Pts',(8.51977310187182,6.55000000039099,-9.4294491161473)) ;
#106807=CARTESIAN_POINT('Ctrl Pts',(8.52085916897636,6.55000000038261,-9.42835848458113)) ;
#106808=CARTESIAN_POINT('Ctrl Pts',(8.5218239980174,6.55000000033869,-9.42704462088201)) ;
#106809=CARTESIAN_POINT('Ctrl Pts',(8.52246334063461,6.55000000029842,-9.42562676665968)) ;
#106810=CARTESIAN_POINT('Ctrl Pts',(8.52278301194322,6.55000000027829,-9.42491783954851)) ;
#106811=CARTESIAN_POINT('Ctrl Pts',(8.52302131164588,6.55000000025926,-9.42418291480655)) ;
#106812=CARTESIAN_POINT('Ctrl Pts',(8.52315270869754,6.55000000024662,-9.42343689763501)) ;
#106813=CARTESIAN_POINT('Ctrl Pts',(8.5232841057492,6.55000000023398,-9.42269088046346)) ;
#106814=CARTESIAN_POINT('Ctrl Pts',(8.52330860014988,6.55000000022778,-9.42193377086234)) ;
#106815=CARTESIAN_POINT('Ctrl Pts',(8.52320066085452,6.55000000023233,-9.42118047403286)) ;
#106816=CARTESIAN_POINT('Ctrl Pts',(8.5228403133075,6.55000000024754,-9.41866564693692)) ;
#106817=CARTESIAN_POINT('Ctrl Pts',(8.52133564423351,6.55000000029586,-9.41640673801312)) ;
#106818=CARTESIAN_POINT('Ctrl Pts',(8.5196587899188,6.55000000031744,-9.41439865149544)) ;
#106819=CARTESIAN_POINT('Ctrl Pts',(8.51932554032813,6.55000000032173,-9.41399957448309)) ;
#106820=CARTESIAN_POINT('Ctrl Pts',(8.51898545723479,6.55000000032523,-9.41361037576486)) ;
#106821=CARTESIAN_POINT('Ctrl Pts',(8.51864615038491,6.5500000003277,-9.41323101231938)) ;
#106822=CARTESIAN_POINT('Ctrl Pts',(8.5145508165866,6.55000000035749,-9.40865220720328)) ;
#106823=CARTESIAN_POINT('Ctrl Pts',(8.50963987409778,6.55000000028078,-9.40482020861866)) ;
#106824=CARTESIAN_POINT('Ctrl Pts',(8.5048217738226,6.55000000018958,-9.4009688701254)) ;
#106825=CARTESIAN_POINT('Ctrl Pts',(8.50046402923751,6.5500000001071,-9.3974855160012)) ;
#106826=CARTESIAN_POINT('Ctrl Pts',(8.49606692679175,6.55000000001227,-9.39404901054622)) ;
#106827=CARTESIAN_POINT('Ctrl Pts',(8.49172374697017,6.55000000000105,-9.39054425434379)) ;
#106828=CARTESIAN_POINT('',(8.49172374697018,6.55,-12.7)) ;
#106829=CARTESIAN_POINT('',(-0.9,6.55,-9.31)) ;
#106830=CARTESIAN_POINT('',(-0.900000000000001,6.55,-12.7)) ;
#106831=CARTESIAN_POINT('',(1.15,6.55,-9.31)) ;
#106832=CARTESIAN_POINT('',(1.25,6.55,-9.31)) ;
#106833=CARTESIAN_POINT('',(1.35,6.55,-9.51)) ;
#106834=CARTESIAN_POINT('Origin',(1.15,6.55,-9.51)) ;
#106835=CARTESIAN_POINT('',(1.35,6.55,-10.81)) ;
#106836=CARTESIAN_POINT('',(1.35,6.55,-10.91)) ;
#106837=CARTESIAN_POINT('',(1.15,6.55,-11.01)) ;
#106838=CARTESIAN_POINT('Origin',(1.15,6.55,-10.81)) ;
#106839=CARTESIAN_POINT('',(-0.9,6.55,-11.01)) ;
#106840=CARTESIAN_POINT('',(1.25,6.55,-11.01)) ;
#106841=CARTESIAN_POINT('',(-0.9,6.55,-12.7)) ;
#106842=CARTESIAN_POINT('Origin',(1.25,5.3,-12.7)) ;
#106843=CARTESIAN_POINT('',(1.25,3.15,-11.8031676725155)) ;
#106844=CARTESIAN_POINT('',(1.25,3.04189189189189,-11.6255279241354)) ;
#106845=CARTESIAN_POINT('Origin',(1.25,2.95,-11.8031676725155)) ;
#106846=CARTESIAN_POINT('',(1.25,3.15,-12.7)) ;
#106847=CARTESIAN_POINT('',(1.25,4.45,-11.8031676725155)) ;
#106848=CARTESIAN_POINT('',(1.25,4.45,-11.7411388300842)) ;
#106849=CARTESIAN_POINT('',(1.25,4.55810810810811,-11.6255279241354)) ;
#106850=CARTESIAN_POINT('Origin',(1.25,4.65,-11.8031676725155)) ;
#106851=CARTESIAN_POINT('',(1.25,5.26552792413544,-10.9181081081081)) ;
#106852=CARTESIAN_POINT('Origin',(1.25,3.8,-10.16)) ;
#106853=CARTESIAN_POINT('',(1.25,5.4431676725155,-10.81)) ;
#106854=CARTESIAN_POINT('Origin',(1.25,5.4431676725155,-11.01)) ;
#106855=CARTESIAN_POINT('',(1.25,6.45,-10.81)) ;
#106856=CARTESIAN_POINT('',(1.25,6.55,-10.81)) ;
#106857=CARTESIAN_POINT('',(1.25,6.45,-9.51)) ;
#106858=CARTESIAN_POINT('',(1.25,6.45,-9.41)) ;
#106859=CARTESIAN_POINT('',(1.25,5.4431676725155,-9.51)) ;
#106860=CARTESIAN_POINT('',(1.25,5.38113883008419,-9.51)) ;
#106861=CARTESIAN_POINT('',(1.25,5.26552792413544,-9.40189189189189)) ;
#106862=CARTESIAN_POINT('Origin',(1.25,5.4431676725155,-9.31)) ;
#106863=CARTESIAN_POINT('',(1.25,4.55810810810811,-8.69447207586456)) ;
#106864=CARTESIAN_POINT('Origin',(1.25,3.8,-10.16)) ;
#106865=CARTESIAN_POINT('',(1.25,4.45,-8.5168323274845)) ;
#106866=CARTESIAN_POINT('Origin',(1.25,4.65,-8.5168323274845)) ;
#106867=CARTESIAN_POINT('',(1.25,4.45,-7.62)) ;
#106868=CARTESIAN_POINT('',(1.25,3.15,-8.5168323274845)) ;
#106869=CARTESIAN_POINT('',(1.25,3.15,-8.57886116991581)) ;
#106870=CARTESIAN_POINT('',(1.25,3.04189189189189,-8.69447207586456)) ;
#106871=CARTESIAN_POINT('Origin',(1.25,2.95,-8.5168323274845)) ;
#106872=CARTESIAN_POINT('',(1.25,2.33447207586456,-9.40189189189189)) ;
#106873=CARTESIAN_POINT('Origin',(1.25,3.8,-10.16)) ;
#106874=CARTESIAN_POINT('',(1.25,2.1568323274845,-9.51)) ;
#106875=CARTESIAN_POINT('Origin',(1.25,2.1568323274845,-9.31)) ;
#106876=CARTESIAN_POINT('',(1.25,0.973783447787483,-9.51)) ;
#106877=CARTESIAN_POINT('',(1.25,0.895262490344437,-9.51)) ;
#106878=CARTESIAN_POINT('',(1.25,0.973783447787483,-10.81)) ;
#106879=CARTESIAN_POINT('Origin',(1.25,3.8,-10.16)) ;
#106880=CARTESIAN_POINT('',(1.25,2.1568323274845,-10.81)) ;
#106881=CARTESIAN_POINT('',(1.25,2.21886116991581,-10.81)) ;
#106882=CARTESIAN_POINT('',(1.25,2.33447207586456,-10.9181081081081)) ;
#106883=CARTESIAN_POINT('Origin',(1.25,2.1568323274845,-11.01)) ;
#106884=CARTESIAN_POINT('Origin',(1.25,3.8,-10.16)) ;
#106885=CARTESIAN_POINT('Origin',(-2.,0.,-12.7)) ;
#106886=CARTESIAN_POINT('',(0.899999999999999,0.,-11.76)) ;
#106887=CARTESIAN_POINT('',(1.1,0.,-11.56)) ;
#106888=CARTESIAN_POINT('Origin',(0.899999999999999,0.,-11.56)) ;
#106889=CARTESIAN_POINT('',(-2.,0.,-11.76)) ;
#106890=CARTESIAN_POINT('',(-2.,0.,-11.76)) ;
#106891=CARTESIAN_POINT('',(-2.,0.,-12.7)) ;
#106892=CARTESIAN_POINT('',(9.9,0.,-12.7)) ;
#106893=CARTESIAN_POINT('',(-2.,0.,-8.56)) ;
#106894=CARTESIAN_POINT('',(-2.,0.,-12.7)) ;
#106895=CARTESIAN_POINT('',(0.899999999999999,0.,-8.56)) ;
#106896=CARTESIAN_POINT('',(0.999999999999999,0.,-8.56)) ;
#106897=CARTESIAN_POINT('',(1.1,0.,-8.76)) ;
#106898=CARTESIAN_POINT('Origin',(0.899999999999999,0.,-8.76)) ;
#106899=CARTESIAN_POINT('',(1.1,0.,-11.66)) ;
#106900=CARTESIAN_POINT('Origin',(-2.,7.65,-12.7)) ;
#106901=CARTESIAN_POINT('',(-2.,6.9,-8.56)) ;
#106902=CARTESIAN_POINT('',(-2.,7.1,-8.76)) ;
#106903=CARTESIAN_POINT('Origin',(-2.,6.9,-8.76)) ;
#106904=CARTESIAN_POINT('',(-2.,-1.13380619344889E-17,-8.56)) ;
#106905=CARTESIAN_POINT('',(-2.,7.55,-12.7)) ;
#106906=CARTESIAN_POINT('',(-2.,6.9,-11.76)) ;
#106907=CARTESIAN_POINT('',(-2.,7.,-11.76)) ;
#106908=CARTESIAN_POINT('',(-2.,7.1,-11.56)) ;
#106909=CARTESIAN_POINT('Origin',(-2.,6.9,-11.56)) ;
#106910=CARTESIAN_POINT('',(-2.,7.1,-8.66)) ;
#106911=CARTESIAN_POINT('Origin',(-1.8,7.,-8.66)) ;
#106912=CARTESIAN_POINT('',(-1.7,0.1,-8.66)) ;
#106913=CARTESIAN_POINT('',(-1.9,0.1,-8.66)) ;
#106914=CARTESIAN_POINT('',(-2.,0.1,-8.66)) ;
#106915=CARTESIAN_POINT('',(-1.9,0.3,-8.66)) ;
#106916=CARTESIAN_POINT('',(-1.9,7.,-8.66)) ;
#106917=CARTESIAN_POINT('Origin',(-1.7,0.3,-8.66)) ;
#106918=CARTESIAN_POINT('Origin',(-1.8,7.,-11.66)) ;
#106919=CARTESIAN_POINT('',(-1.9,0.3,-11.66)) ;
#106920=CARTESIAN_POINT('',(-1.7,0.1,-11.66)) ;
#106921=CARTESIAN_POINT('Origin',(-1.7,0.3,-11.66)) ;
#106922=CARTESIAN_POINT('',(-1.9,0.1,-11.66)) ;
#106923=CARTESIAN_POINT('',(-1.9,1.23908819712629E-17,-11.66)) ;
#106924=CARTESIAN_POINT('',(0.999999999999999,0.1,-11.66)) ;
#106925=CARTESIAN_POINT('Origin',(-1.8,-2.2514151555628E-16,-10.16)) ;
#106926=CARTESIAN_POINT('',(-1.8,4.6,-10.81)) ;
#106927=CARTESIAN_POINT('',(-1.8,4.6,-9.51)) ;
#106928=CARTESIAN_POINT('',(-1.8,4.6,-9.61)) ;
#106929=CARTESIAN_POINT('',(-1.8,0.3,-9.51)) ;
#106930=CARTESIAN_POINT('',(-1.8,0.2,-9.51)) ;
#106931=CARTESIAN_POINT('',(-1.8,0.3,-8.76)) ;
#106932=CARTESIAN_POINT('',(-1.8,0.3,-8.66)) ;
#106933=CARTESIAN_POINT('',(-1.8,6.9,-8.76)) ;
#106934=CARTESIAN_POINT('',(-1.8,-5.16691679585995E-17,-8.76)) ;
#106935=CARTESIAN_POINT('',(-1.8,6.9,-11.56)) ;
#106936=CARTESIAN_POINT('',(-1.8,6.9,-10.16)) ;
#106937=CARTESIAN_POINT('',(-1.8,0.3,-11.56)) ;
#106938=CARTESIAN_POINT('',(-1.8,-3.98613863153961E-16,-11.56)) ;
#106939=CARTESIAN_POINT('',(-1.8,0.3,-10.81)) ;
#106940=CARTESIAN_POINT('',(-1.8,0.3,-10.71)) ;
#106941=CARTESIAN_POINT('',(-1.8,4.5,-10.81)) ;
#106942=CARTESIAN_POINT('Origin',(0.549999999999999,4.5,-9.61)) ;
#106943=CARTESIAN_POINT('',(-1.7,0.3,-9.61)) ;
#106944=CARTESIAN_POINT('',(-1.7,4.4,-9.61)) ;
#106945=CARTESIAN_POINT('',(-1.7,4.5,-9.61)) ;
#106946=CARTESIAN_POINT('',(0.45,4.4,-9.61)) ;
#106947=CARTESIAN_POINT('',(0.45,4.4,-9.61)) ;
#106948=CARTESIAN_POINT('',(0.45,0.3,-9.61)) ;
#106949=CARTESIAN_POINT('',(0.45,4.5,-9.61)) ;
#106950=CARTESIAN_POINT('',(0.549999999999999,0.3,-9.61)) ;
#106951=CARTESIAN_POINT('Origin',(0.549999999999999,4.5,-10.71)) ;
#106952=CARTESIAN_POINT('',(0.45,0.3,-10.71)) ;
#106953=CARTESIAN_POINT('',(0.45,4.4,-10.71)) ;
#106954=CARTESIAN_POINT('',(0.45,4.5,-10.71)) ;
#106955=CARTESIAN_POINT('',(-1.7,4.4,-10.71)) ;
#106956=CARTESIAN_POINT('',(-1.7,4.4,-10.71)) ;
#106957=CARTESIAN_POINT('',(-1.7,0.3,-10.71)) ;
#106958=CARTESIAN_POINT('',(-1.7,0.2,-10.71)) ;
#106959=CARTESIAN_POINT('',(0.549999999999999,0.3,-10.71)) ;
#106960=CARTESIAN_POINT('Origin',(0.549999999999999,4.5,-10.71)) ;
#106961=CARTESIAN_POINT('',(-1.7,4.5,-9.71)) ;
#106962=CARTESIAN_POINT('',(-1.7,4.5,-10.61)) ;
#106963=CARTESIAN_POINT('',(-1.7,4.5,-10.71)) ;
#106964=CARTESIAN_POINT('',(0.45,4.5,-10.61)) ;
#106965=CARTESIAN_POINT('',(0.45,4.5,-10.61)) ;
#106966=CARTESIAN_POINT('',(0.45,4.5,-9.71)) ;
#106967=CARTESIAN_POINT('',(0.45,4.5,-10.71)) ;
#106968=CARTESIAN_POINT('',(-1.7,4.5,-9.71)) ;
#106969=CARTESIAN_POINT('Origin',(0.55,3.09772049281573E-17,-10.16)) ;
#106970=CARTESIAN_POINT('',(0.55,2.61224989991992,-10.56)) ;
#106971=CARTESIAN_POINT('',(0.55,2.65280931275608,-10.61)) ;
#106972=CARTESIAN_POINT('Ctrl Pts',(0.55,2.61224989991992,-10.56)) ;
#106973=CARTESIAN_POINT('Ctrl Pts',(0.55,2.61224989991992,-10.563869744162)) ;
#106974=CARTESIAN_POINT('Ctrl Pts',(0.55,2.61317624258758,-10.5684201039157)) ;
#106975=CARTESIAN_POINT('Ctrl Pts',(0.55,2.61634258087509,-10.5766330008589)) ;
#106976=CARTESIAN_POINT('Ctrl Pts',(0.55,2.61951410407877,-10.5816304286453)) ;
#106977=CARTESIAN_POINT('Ctrl Pts',(0.55,2.63040394024853,-10.5949387190701)) ;
#106978=CARTESIAN_POINT('Ctrl Pts',(0.55,2.6414836688106,-10.6031705809674)) ;
#106979=CARTESIAN_POINT('Ctrl Pts',(0.55,2.65280931275608,-10.61)) ;
#106980=CARTESIAN_POINT('',(0.55,0.3,-10.61)) ;
#106981=CARTESIAN_POINT('',(0.55,1.39397422176708E-16,-10.61)) ;
#106982=CARTESIAN_POINT('',(0.55,0.3,-9.71)) ;
#106983=CARTESIAN_POINT('',(0.55,0.3,-9.61)) ;
#106984=CARTESIAN_POINT('',(0.55,2.65280931275594,-9.71000000000009)) ;
#106985=CARTESIAN_POINT('',(0.55,6.35032701027224E-17,-9.71)) ;
#106986=CARTESIAN_POINT('',(0.55,2.61224989991992,-9.76)) ;
#106987=CARTESIAN_POINT('Ctrl Pts',(0.55,2.65280931275594,-9.71000000000009)) ;
#106988=CARTESIAN_POINT('Ctrl Pts',(0.55,2.64148366881051,-9.71682941903265)) ;
#106989=CARTESIAN_POINT('Ctrl Pts',(0.55,2.6304039402485,-9.72506128092989)) ;
#106990=CARTESIAN_POINT('Ctrl Pts',(0.55,2.61951410407877,-9.73836957135471)) ;
#106991=CARTESIAN_POINT('Ctrl Pts',(0.55,2.61634258087509,-9.74336699914113)) ;
#106992=CARTESIAN_POINT('Ctrl Pts',(0.55,2.61317624258758,-9.75157989608431)) ;
#106993=CARTESIAN_POINT('Ctrl Pts',(0.55,2.61224989991992,-9.75613025583802)) ;
#106994=CARTESIAN_POINT('Ctrl Pts',(0.55,2.61224989991992,-9.76)) ;
#106995=CARTESIAN_POINT('',(0.55,2.61224989991992,-9.66)) ;
#106996=CARTESIAN_POINT('Origin',(0.,0.2,-10.16)) ;
#106997=CARTESIAN_POINT('',(-1.7,0.2,-10.81)) ;
#106998=CARTESIAN_POINT('',(-1.7,0.2,-11.56)) ;
#106999=CARTESIAN_POINT('',(-1.7,0.2,-11.66)) ;
#107000=CARTESIAN_POINT('',(0.899999999999999,0.2,-11.56)) ;
#107001=CARTESIAN_POINT('',(0.999999999999999,0.2,-11.56)) ;
#107002=CARTESIAN_POINT('',(0.899999999999999,0.2,-8.76)) ;
#107003=CARTESIAN_POINT('',(0.899999999999999,0.2,-8.66)) ;
#107004=CARTESIAN_POINT('',(-1.7,0.2,-8.76)) ;
#107005=CARTESIAN_POINT('',(-1.8,0.2,-8.76)) ;
#107006=CARTESIAN_POINT('',(-1.7,0.2,-9.51)) ;
#107007=CARTESIAN_POINT('',(-1.7,0.2,-9.61)) ;
#107008=CARTESIAN_POINT('',(0.65,0.2,-9.51)) ;
#107009=CARTESIAN_POINT('',(-1.16429916652874E-32,0.2,-9.51)) ;
#107010=CARTESIAN_POINT('',(0.65,0.2,-10.81)) ;
#107011=CARTESIAN_POINT('',(0.65,0.2,-10.71)) ;
#107012=CARTESIAN_POINT('',(-1.35834902761687E-32,0.2,-10.81)) ;
#107013=CARTESIAN_POINT('Origin',(3.,2.3,-12.7)) ;
#107014=CARTESIAN_POINT('',(3.,4.2,-9.66)) ;
#107015=CARTESIAN_POINT('',(3.,3.4,-9.66)) ;
#107016=CARTESIAN_POINT('',(3.,2.3,-9.66)) ;
#107017=CARTESIAN_POINT('',(3.,4.3,-9.76)) ;
#107018=CARTESIAN_POINT('Origin',(3.,4.2,-9.76)) ;
#107019=CARTESIAN_POINT('',(3.,4.3,-10.56)) ;
#107020=CARTESIAN_POINT('',(3.,4.3,-12.7)) ;
#107021=CARTESIAN_POINT('',(3.,4.2,-10.66)) ;
#107022=CARTESIAN_POINT('Origin',(3.,4.2,-10.56)) ;
#107023=CARTESIAN_POINT('',(3.,3.4,-10.66)) ;
#107024=CARTESIAN_POINT('',(3.,2.3,-10.66)) ;
#107025=CARTESIAN_POINT('',(3.,3.3,-10.56)) ;
#107026=CARTESIAN_POINT('Origin',(3.,3.4,-10.56)) ;
#107027=CARTESIAN_POINT('',(3.,3.3,-9.76)) ;
#107028=CARTESIAN_POINT('',(3.,3.3,-12.7)) ;
#107029=CARTESIAN_POINT('Origin',(3.,3.4,-9.76)) ;
#107030=CARTESIAN_POINT('Origin',(-1.,3.8,-10.16)) ;
#107031=CARTESIAN_POINT('',(-1.,1.6,-12.1221416870349)) ;
#107032=CARTESIAN_POINT('',(-1.,1.55483870967742,-11.9955519007746)) ;
#107033=CARTESIAN_POINT('Origin',(-1.,1.40000000000001,-12.1221416870349)) ;
#107034=CARTESIAN_POINT('',(-1.,1.6,-12.7)) ;
#107035=CARTESIAN_POINT('',(-1.,2.95,-11.8031676725155)) ;
#107036=CARTESIAN_POINT('',(-1.,2.95,-10.16)) ;
#107037=CARTESIAN_POINT('',(-1.,2.1568323274845,-11.01)) ;
#107038=CARTESIAN_POINT('Origin',(-1.,3.8,-10.16)) ;
#107039=CARTESIAN_POINT('',(-1.,1.02736587339765,-11.01)) ;
#107040=CARTESIAN_POINT('',(-1.,3.8,-11.01)) ;
#107041=CARTESIAN_POINT('Origin',(-1.,3.8,-10.16)) ;
#107042=CARTESIAN_POINT('Origin',(-1.,3.05,-12.71)) ;
#107043=CARTESIAN_POINT('',(1.15,3.05,-11.8031676725155)) ;
#107044=CARTESIAN_POINT('',(1.15,3.05,-11.7411388300842)) ;
#107045=CARTESIAN_POINT('',(-0.900000000000002,3.05,-11.8031676725155)) ;
#107046=CARTESIAN_POINT('',(-1.,3.05,-11.8031676725155)) ;
#107047=CARTESIAN_POINT('',(-0.900000000000002,3.05,-12.71)) ;
#107048=CARTESIAN_POINT('Origin',(-1.,2.21886116991581,-10.91)) ;
#107049=CARTESIAN_POINT('',(-0.900000000000002,2.1568323274845,-10.91)) ;
#107050=CARTESIAN_POINT('',(1.15,2.1568323274845,-10.91)) ;
#107051=CARTESIAN_POINT('',(1.25,2.1568323274845,-10.91)) ;
#107052=CARTESIAN_POINT('',(1.15,0.895262490344437,-10.91)) ;
#107053=CARTESIAN_POINT('',(-0.900000000000002,2.21886116991581,-10.91)) ;
#107054=CARTESIAN_POINT('Origin',(-1.,3.8,-10.16)) ;
#107055=CARTESIAN_POINT('',(-0.900000000000002,2.24565220167453,-10.9640540540541)) ;
#107056=CARTESIAN_POINT('',(-0.900000000000001,2.99594594594595,-11.7143477983255)) ;
#107057=CARTESIAN_POINT('Origin',(-0.900000000000001,3.8,-10.16)) ;
#107058=CARTESIAN_POINT('',(1.15,2.99594594594595,-11.7143477983255)) ;
#107059=CARTESIAN_POINT('',(-1.,2.99594594594595,-11.7143477983255)) ;
#107060=CARTESIAN_POINT('',(1.15,2.24565220167453,-10.9640540540541)) ;
#107061=CARTESIAN_POINT('Origin',(1.15,3.8,-10.16)) ;
#107062=CARTESIAN_POINT('',(-1.,2.24565220167453,-10.9640540540541)) ;
#107063=CARTESIAN_POINT('Origin',(-1.,3.8,-10.16)) ;
#107064=CARTESIAN_POINT('',(-0.900000000000002,2.99594594594594,-8.60565220167453)) ;
#107065=CARTESIAN_POINT('',(-0.900000000000002,2.24565220167453,-9.35594594594595)) ;
#107066=CARTESIAN_POINT('Origin',(-0.900000000000001,3.8,-10.16)) ;
#107067=CARTESIAN_POINT('',(1.15,2.24565220167453,-9.35594594594595)) ;
#107068=CARTESIAN_POINT('',(-1.,2.24565220167453,-9.35594594594595)) ;
#107069=CARTESIAN_POINT('',(1.15,2.99594594594594,-8.60565220167453)) ;
#107070=CARTESIAN_POINT('Origin',(1.15,3.8,-10.16)) ;
#107071=CARTESIAN_POINT('',(-1.,2.99594594594594,-8.60565220167453)) ;
#107072=CARTESIAN_POINT('Origin',(-1.,2.21886116991581,-9.41)) ;
#107073=CARTESIAN_POINT('',(1.15,2.1568323274845,-9.41)) ;
#107074=CARTESIAN_POINT('',(1.15,2.21886116991581,-9.41)) ;
#107075=CARTESIAN_POINT('',(-0.900000000000002,2.1568323274845,-9.41)) ;
#107076=CARTESIAN_POINT('',(-1.,2.1568323274845,-9.41)) ;
#107077=CARTESIAN_POINT('',(-0.900000000000002,0.895262490344437,-9.41)) ;
#107078=CARTESIAN_POINT('Origin',(-1.,3.05,-7.61)) ;
#107079=CARTESIAN_POINT('',(-0.900000000000002,3.05,-8.5168323274845)) ;
#107080=CARTESIAN_POINT('',(1.15,3.05,-8.5168323274845)) ;
#107081=CARTESIAN_POINT('',(1.25,3.05,-8.5168323274845)) ;
#107082=CARTESIAN_POINT('',(1.15,3.05,-7.62)) ;
#107083=CARTESIAN_POINT('',(-0.900000000000002,3.05,-8.57886116991581)) ;
#107084=CARTESIAN_POINT('Origin',(-1.,3.8,-10.16)) ;
#107085=CARTESIAN_POINT('',(-1.,2.1568323274845,-9.31)) ;
#107086=CARTESIAN_POINT('',(-1.,2.95,-8.5168323274845)) ;
#107087=CARTESIAN_POINT('Origin',(-1.,3.8,-10.16)) ;
#107088=CARTESIAN_POINT('',(-1.,2.95,-7.62)) ;
#107089=CARTESIAN_POINT('',(-1.,1.6,-8.19785831296513)) ;
#107090=CARTESIAN_POINT('',(-1.,1.6,-10.16)) ;
#107091=CARTESIAN_POINT('',(-1.,1.55483870967743,-8.32444809922545)) ;
#107092=CARTESIAN_POINT('Origin',(-1.,1.40000000000001,-8.19785831296513)) ;
#107093=CARTESIAN_POINT('',(-1.,1.02736587339765,-9.31)) ;
#107094=CARTESIAN_POINT('Origin',(-1.,3.8,-10.16)) ;
#107095=CARTESIAN_POINT('',(-1.,2.21886116991581,-9.31)) ;
#107096=CARTESIAN_POINT('Origin',(-1.,3.8,-10.16)) ;
#107097=CARTESIAN_POINT('',(-1.,5.4431676725155,-11.01)) ;
#107098=CARTESIAN_POINT('',(-1.,4.65,-11.8031676725155)) ;
#107099=CARTESIAN_POINT('Origin',(-1.,3.8,-10.16)) ;
#107100=CARTESIAN_POINT('',(-1.,4.65,-10.16)) ;
#107101=CARTESIAN_POINT('',(-1.,6.45,-11.01)) ;
#107102=CARTESIAN_POINT('',(-1.,6.45,-10.91)) ;
#107103=CARTESIAN_POINT('',(-1.,3.8,-11.01)) ;
#107104=CARTESIAN_POINT('Origin',(-1.,4.55,-11.7411388300842)) ;
#107105=CARTESIAN_POINT('',(-0.900000000000001,4.55,-11.8031676725155)) ;
#107106=CARTESIAN_POINT('',(1.15,4.55,-11.8031676725155)) ;
#107107=CARTESIAN_POINT('',(1.25,4.55,-11.8031676725155)) ;
#107108=CARTESIAN_POINT('',(1.15,4.55,-12.7)) ;
#107109=CARTESIAN_POINT('',(-0.900000000000001,4.55,-11.7411388300842)) ;
#107110=CARTESIAN_POINT('Origin',(-1.,3.8,-10.16)) ;
#107111=CARTESIAN_POINT('',(-0.900000000000001,4.60405405405406,-11.7143477983255)) ;
#107112=CARTESIAN_POINT('',(-0.900000000000001,5.35434779832547,-10.9640540540541)) ;
#107113=CARTESIAN_POINT('Origin',(-0.900000000000001,3.8,-10.16)) ;
#107114=CARTESIAN_POINT('',(1.15,5.35434779832547,-10.9640540540541)) ;
#107115=CARTESIAN_POINT('',(-1.,5.35434779832547,-10.9640540540541)) ;
#107116=CARTESIAN_POINT('',(1.15,4.60405405405405,-11.7143477983255)) ;
#107117=CARTESIAN_POINT('Origin',(1.15,3.8,-10.16)) ;
#107118=CARTESIAN_POINT('',(-1.,4.60405405405406,-11.7143477983255)) ;
#107119=CARTESIAN_POINT('Origin',(-1.,6.55,-10.91)) ;
#107120=CARTESIAN_POINT('',(-0.900000000000001,5.4431676725155,-10.91)) ;
#107121=CARTESIAN_POINT('',(-0.9,6.45,-10.91)) ;
#107122=CARTESIAN_POINT('',(-0.9,6.55,-10.91)) ;
#107123=CARTESIAN_POINT('',(1.15,6.45,-10.91)) ;
#107124=CARTESIAN_POINT('',(-1.,6.45,-10.91)) ;
#107125=CARTESIAN_POINT('',(1.15,5.4431676725155,-10.91)) ;
#107126=CARTESIAN_POINT('',(1.15,5.38113883008419,-10.91)) ;
#107127=CARTESIAN_POINT('',(-1.,5.4431676725155,-10.91)) ;
#107128=CARTESIAN_POINT('Origin',(-1.,3.8,-10.16)) ;
#107129=CARTESIAN_POINT('',(-0.900000000000001,5.35434779832547,-9.35594594594594)) ;
#107130=CARTESIAN_POINT('',(-0.900000000000001,4.60405405405405,-8.60565220167453)) ;
#107131=CARTESIAN_POINT('Origin',(-0.900000000000001,3.8,-10.16)) ;
#107132=CARTESIAN_POINT('',(1.15,4.60405405405405,-8.60565220167453)) ;
#107133=CARTESIAN_POINT('',(-1.,4.60405405405405,-8.60565220167453)) ;
#107134=CARTESIAN_POINT('',(1.15,5.35434779832547,-9.35594594594594)) ;
#107135=CARTESIAN_POINT('Origin',(1.15,3.8,-10.16)) ;
#107136=CARTESIAN_POINT('',(-1.,5.35434779832547,-9.35594594594594)) ;
#107137=CARTESIAN_POINT('Origin',(-1.,4.55,-8.57886116991581)) ;
#107138=CARTESIAN_POINT('',(1.15,4.55,-8.5168323274845)) ;
#107139=CARTESIAN_POINT('',(1.15,4.55,-8.57886116991581)) ;
#107140=CARTESIAN_POINT('',(-0.900000000000001,4.55,-8.5168323274845)) ;
#107141=CARTESIAN_POINT('',(-1.,4.55,-8.5168323274845)) ;
#107142=CARTESIAN_POINT('',(-0.900000000000001,4.55,-7.62)) ;
#107143=CARTESIAN_POINT('Origin',(-1.,6.55,-9.41)) ;
#107144=CARTESIAN_POINT('',(1.15,5.4431676725155,-9.41)) ;
#107145=CARTESIAN_POINT('',(1.15,6.45,-9.41)) ;
#107146=CARTESIAN_POINT('',(1.15,6.55,-9.41)) ;
#107147=CARTESIAN_POINT('',(-0.9,6.45,-9.41)) ;
#107148=CARTESIAN_POINT('',(-1.,6.45,-9.41)) ;
#107149=CARTESIAN_POINT('',(-0.900000000000001,5.4431676725155,-9.41)) ;
#107150=CARTESIAN_POINT('',(-0.900000000000001,5.38113883008419,-9.41)) ;
#107151=CARTESIAN_POINT('',(1.25,5.4431676725155,-9.41)) ;
#107152=CARTESIAN_POINT('Origin',(-1.,3.8,-10.16)) ;
#107153=CARTESIAN_POINT('',(-1.,5.4431676725155,-9.31)) ;
#107154=CARTESIAN_POINT('',(-1.,6.45,-9.31)) ;
#107155=CARTESIAN_POINT('',(-1.,6.55,-9.31)) ;
#107156=CARTESIAN_POINT('',(-1.,6.45,-10.16)) ;
#107157=CARTESIAN_POINT('',(-1.,4.65,-8.5168323274845)) ;
#107158=CARTESIAN_POINT('',(-1.,4.65,-8.57886116991581)) ;
#107159=CARTESIAN_POINT('Origin',(-1.,3.8,-10.16)) ;
#107160=CARTESIAN_POINT('Origin',(10.,4.35421736843756,-11.035)) ;
#107161=CARTESIAN_POINT('',(9.91643989873054,7.72792407799439,-11.0210733164551)) ;
#107162=CARTESIAN_POINT('',(8.58356010126947,8.17221734381475,-10.7989266835449)) ;
#107163=CARTESIAN_POINT('',(8.47075240319158,8.20981990984071,-10.7801254005319)) ;
#107164=CARTESIAN_POINT('',(8.58356010126947,6.66256607592813,-10.7989266835449)) ;
#107165=CARTESIAN_POINT('',(8.58356010126947,6.64863939238321,-10.7989266835449)) ;
#107166=CARTESIAN_POINT('',(9.91643989873054,6.8847127088383,-11.0210733164551)) ;
#107167=CARTESIAN_POINT('',(9.98442535909739,6.89604361889945,-11.0324042265162)) ;
#107168=CARTESIAN_POINT('',(9.91643989873054,7.8,-11.0210733164551)) ;
#107169=CARTESIAN_POINT('Origin',(8.5,4.35421736843756,-10.785)) ;
#107170=CARTESIAN_POINT('',(8.5,8.17221734381475,-10.7002872911617)) ;
#107171=CARTESIAN_POINT('',(8.50000000129681,8.20000000266559,-10.702105625353)) ;
#107172=CARTESIAN_POINT('Origin',(8.5,8.17870774546496,-10.8890376382098)) ;
#107173=CARTESIAN_POINT('',(8.5,8.2,-9.57634544369909)) ;
#107174=CARTESIAN_POINT('',(8.5,6.66256607592813,-9.61971270883831)) ;
#107175=CARTESIAN_POINT('',(8.5,6.64863939238321,-9.61971270883831)) ;
#107176=CARTESIAN_POINT('',(8.50000000002143,6.64999999935441,-9.61931784432624)) ;
#107177=CARTESIAN_POINT('Origin',(8.5,6.65811550105781,-9.42318847658934)) ;
#107178=CARTESIAN_POINT('',(8.49999999999933,6.65000073218972,-10.7006896909637)) ;
#107179=CARTESIAN_POINT('',(8.5,6.65,-10.8836393923832)) ;
#107180=CARTESIAN_POINT('',(8.5,6.66256607592813,-10.7002872911617)) ;
#107181=CARTESIAN_POINT('Origin',(8.5,6.65133313785406,-10.8970100509337)) ;
#107182=CARTESIAN_POINT('',(8.5,8.20007071090457,-10.7002872911617)) ;
#107183=CARTESIAN_POINT('Origin',(8.5,4.35421736843756,-9.535)) ;
#107184=CARTESIAN_POINT('',(9.91643989873054,6.8847127088383,-9.29892668354491)) ;
#107185=CARTESIAN_POINT('',(8.58356010126947,6.66256607592813,-9.52107331645509)) ;
#107186=CARTESIAN_POINT('',(8.48442535909739,6.64604361889945,-9.53759577348377)) ;
#107187=CARTESIAN_POINT('',(8.58356010126947,8.20007071090456,-9.52107331645509)) ;
#107188=CARTESIAN_POINT('',(9.91643989873054,7.72792407799439,-9.29892668354491)) ;
#107189=CARTESIAN_POINT('',(9.97075240319158,7.70981990984071,-9.28987459946807)) ;
#107190=CARTESIAN_POINT('',(9.91643989873054,6.8,-9.29892668354491)) ;
#107191=CARTESIAN_POINT('Origin',(8.5,3.65,-9.66)) ;
#107192=CARTESIAN_POINT('',(8.45734623443633,3.62014236410543,-10.0620655561573)) ;
#107193=CARTESIAN_POINT('',(8.02582401135442,3.3180768079481,-9.76)) ;
#107194=CARTESIAN_POINT('',(8.34729988159781,3.54310991711847,-9.98503310917037)) ;
#107195=CARTESIAN_POINT('',(8.02582401135442,3.31807680794809,-10.56)) ;
#107196=CARTESIAN_POINT('',(8.02582401135442,3.3180768079481,-9.66)) ;
#107197=CARTESIAN_POINT('',(8.45734623443633,3.62014236410543,-10.2579344438427)) ;
#107198=CARTESIAN_POINT('',(8.70083523513316,3.79058466459322,-10.0874921433549)) ;
#107199=CARTESIAN_POINT('',(8.45734623443633,3.62014236410543,-9.66)) ;
#107200=CARTESIAN_POINT('Origin',(8.5,3.95,-9.66)) ;
#107201=CARTESIAN_POINT('',(8.5,3.89793444384266,-10.2579344438427)) ;
#107202=CARTESIAN_POINT('',(8.5,3.89793444384266,-10.0620655561573)) ;
#107203=CARTESIAN_POINT('',(8.5,3.89793444384266,-9.66)) ;
#107204=CARTESIAN_POINT('',(8.5,3.70206555615734,-10.0620655561573)) ;
#107205=CARTESIAN_POINT('',(8.5,3.95,-10.0620655561573)) ;
#107206=CARTESIAN_POINT('',(8.5,3.70206555615734,-10.2579344438427)) ;
#107207=CARTESIAN_POINT('',(8.5,3.70206555615734,-9.66)) ;
#107208=CARTESIAN_POINT('',(8.5,3.95,-10.2579344438427)) ;
#107209=CARTESIAN_POINT('Origin',(8.,4.3,-9.66)) ;
#107210=CARTESIAN_POINT('',(8.45734623443633,3.97985763589457,-10.2579344438427)) ;
#107211=CARTESIAN_POINT('',(8.02582401135442,4.2819231920519,-10.56)) ;
#107212=CARTESIAN_POINT('',(8.32457260887054,4.07279917379062,-10.3508759817387)) ;
#107213=CARTESIAN_POINT('',(8.02582401135442,4.2819231920519,-9.76)) ;
#107214=CARTESIAN_POINT('',(8.02582401135442,4.2819231920519,-9.66)) ;
#107215=CARTESIAN_POINT('',(8.45734623443633,3.97985763589457,-10.0620655561573)) ;
#107216=CARTESIAN_POINT('',(7.97103725533518,4.32027392126537,-9.72164927078653)) ;
#107217=CARTESIAN_POINT('',(8.45734623443633,3.97985763589457,-9.66)) ;
#107218=CARTESIAN_POINT('Origin',(1.5,2.3,-9.66)) ;
#107219=CARTESIAN_POINT('',(7.96847777691809,3.4,-9.66)) ;
#107220=CARTESIAN_POINT('',(8.,3.4,-9.66)) ;
#107221=CARTESIAN_POINT('',(7.96847777691809,4.2,-9.66)) ;
#107222=CARTESIAN_POINT('',(7.96847777691809,4.2,-9.66)) ;
#107223=CARTESIAN_POINT('',(3.,4.2,-9.66)) ;
#107224=CARTESIAN_POINT('Origin',(1.5,2.3,-10.66)) ;
#107225=CARTESIAN_POINT('',(7.96847777691809,4.2,-10.66)) ;
#107226=CARTESIAN_POINT('',(1.5,4.2,-10.66)) ;
#107227=CARTESIAN_POINT('',(7.96847777691809,3.4,-10.66)) ;
#107228=CARTESIAN_POINT('',(7.96847777691809,2.3,-10.66)) ;
#107229=CARTESIAN_POINT('',(1.5,3.4,-10.66)) ;
#107230=CARTESIAN_POINT('Origin',(8.,3.3,-9.66)) ;
#107231=CARTESIAN_POINT('',(7.96847777691809,3.3,-10.56)) ;
#107232=CARTESIAN_POINT('',(8.,3.3,-10.56)) ;
#107233=CARTESIAN_POINT('',(7.96847777691809,3.3,-9.76)) ;
#107234=CARTESIAN_POINT('',(7.96847777691809,3.3,-9.66)) ;
#107235=CARTESIAN_POINT('',(3.,3.3,-9.76)) ;
#107236=CARTESIAN_POINT('Origin',(1.5,4.3,-9.66)) ;
#107237=CARTESIAN_POINT('',(7.96847777691809,4.3,-9.76)) ;
#107238=CARTESIAN_POINT('',(8.,4.3,-9.76)) ;
#107239=CARTESIAN_POINT('',(7.96847777691809,4.3,-10.56)) ;
#107240=CARTESIAN_POINT('',(7.96847777691809,4.3,-9.66)) ;
#107241=CARTESIAN_POINT('',(1.5,4.3,-10.56)) ;
#107242=CARTESIAN_POINT('Origin',(1.5,2.3,-9.66)) ;
#107243=CARTESIAN_POINT('',(-0.4,2.3,-9.66)) ;
#107244=CARTESIAN_POINT('',(-0.4,-3.36847777691809,-9.66)) ;
#107245=CARTESIAN_POINT('',(-0.4,-3.4,-9.66)) ;
#107246=CARTESIAN_POINT('',(0.4,-3.36847777691809,-9.66)) ;
#107247=CARTESIAN_POINT('',(0.4,-3.36847777691809,-9.66)) ;
#107248=CARTESIAN_POINT('',(0.4,2.29999999999999,-9.66)) ;
#107249=CARTESIAN_POINT('',(0.4,2.29999999999999,-9.66)) ;
#107250=CARTESIAN_POINT('',(0.536602540378444,2.83090991212703,-9.66)) ;
#107251=CARTESIAN_POINT('Origin',(1.5,2.3,-9.66)) ;
#107252=CARTESIAN_POINT('',(0.536602540378444,3.93764017256378,-9.66)) ;
#107253=CARTESIAN_POINT('',(0.536602540378444,2.83090991212703,-9.66)) ;
#107254=CARTESIAN_POINT('Origin',(1.5,2.3,-9.66)) ;
#107255=CARTESIAN_POINT('Origin',(1.5,2.3,-10.66)) ;
#107256=CARTESIAN_POINT('',(0.4,2.29999999999999,-10.66)) ;
#107257=CARTESIAN_POINT('',(0.4,-3.36847777691809,-10.66)) ;
#107258=CARTESIAN_POINT('',(0.4,2.3,-10.66)) ;
#107259=CARTESIAN_POINT('',(-0.4,-3.36847777691809,-10.66)) ;
#107260=CARTESIAN_POINT('',(1.5,-3.36847777691809,-10.66)) ;
#107261=CARTESIAN_POINT('',(-0.4,2.3,-10.66)) ;
#107262=CARTESIAN_POINT('',(-0.4,2.3,-10.66)) ;
#107263=CARTESIAN_POINT('',(0.536602540378444,3.93764017256378,-10.66)) ;
#107264=CARTESIAN_POINT('Origin',(1.5,2.3,-10.66)) ;
#107265=CARTESIAN_POINT('',(0.536602540378444,2.83090991212703,-10.66)) ;
#107266=CARTESIAN_POINT('',(0.536602540378444,3.93764017256378,-10.66)) ;
#107267=CARTESIAN_POINT('Origin',(1.5,2.3,-10.66)) ;
#107268=CARTESIAN_POINT('Origin',(1.5,2.3,-9.66)) ;
#107269=CARTESIAN_POINT('',(-0.5,2.3,-9.76)) ;
#107270=CARTESIAN_POINT('',(-0.5,2.3,-10.56)) ;
#107271=CARTESIAN_POINT('',(-0.5,2.3,-9.66)) ;
#107272=CARTESIAN_POINT('Origin',(1.5,2.3,-9.76)) ;
#107273=CARTESIAN_POINT('Origin',(1.5,2.3,-10.56)) ;
#107274=CARTESIAN_POINT('Origin',(-0.5,-3.4,-9.66)) ;
#107275=CARTESIAN_POINT('',(-0.5,-3.36847777691809,-10.56)) ;
#107276=CARTESIAN_POINT('',(-0.5,-3.4,-10.56)) ;
#107277=CARTESIAN_POINT('',(-0.5,-3.36847777691809,-9.76)) ;
#107278=CARTESIAN_POINT('',(-0.5,-3.36847777691809,-9.66)) ;
#107279=CARTESIAN_POINT('',(-0.5,2.3,-9.76)) ;
#107280=CARTESIAN_POINT('Origin',(-0.15,-3.9,-9.66)) ;
#107281=CARTESIAN_POINT('',(-0.179857635894567,-3.85734623443633,-10.0620655561573)) ;
#107282=CARTESIAN_POINT('',(-0.481923192051905,-3.42582401135442,-9.76)) ;
#107283=CARTESIAN_POINT('',(-0.256890082881532,-3.74729988159781,-9.98503310917037)) ;
#107284=CARTESIAN_POINT('',(-0.481923192051905,-3.42582401135442,-10.56)) ;
#107285=CARTESIAN_POINT('',(-0.481923192051905,-3.42582401135442,-9.66)) ;
#107286=CARTESIAN_POINT('',(-0.179857635894567,-3.85734623443633,-10.2579344438427)) ;
#107287=CARTESIAN_POINT('',(-0.00941533540678435,-4.10083523513317,-10.0874921433549)) ;
#107288=CARTESIAN_POINT('',(-0.179857635894567,-3.85734623443633,-9.66)) ;
#107289=CARTESIAN_POINT('Origin',(0.15,-3.9,-9.66)) ;
#107290=CARTESIAN_POINT('',(0.0979344438426627,-3.9,-10.2579344438427)) ;
#107291=CARTESIAN_POINT('',(0.0979344438426627,-3.9,-10.0620655561573)) ;
#107292=CARTESIAN_POINT('',(0.0979344438426627,-3.9,-9.66)) ;
#107293=CARTESIAN_POINT('',(-0.0979344438426628,-3.9,-10.0620655561573)) ;
#107294=CARTESIAN_POINT('',(0.15,-3.9,-10.0620655561573)) ;
#107295=CARTESIAN_POINT('',(-0.0979344438426628,-3.9,-10.2579344438427)) ;
#107296=CARTESIAN_POINT('',(-0.0979344438426628,-3.9,-9.66)) ;
#107297=CARTESIAN_POINT('',(0.15,-3.9,-10.2579344438427)) ;
#107298=CARTESIAN_POINT('Origin',(0.5,-3.4,-9.66)) ;
#107299=CARTESIAN_POINT('',(0.179857635894567,-3.85734623443633,-10.2579344438427)) ;
#107300=CARTESIAN_POINT('',(0.481923192051904,-3.42582401135442,-10.56)) ;
#107301=CARTESIAN_POINT('',(0.272799173790623,-3.72457260887054,-10.3508759817387)) ;
#107302=CARTESIAN_POINT('',(0.481923192051904,-3.42582401135442,-9.76)) ;
#107303=CARTESIAN_POINT('',(0.481923192051904,-3.42582401135442,-9.66)) ;
#107304=CARTESIAN_POINT('',(0.179857635894567,-3.85734623443633,-10.0620655561573)) ;
#107305=CARTESIAN_POINT('',(0.520273921265371,-3.37103725533519,-9.72164927078653)) ;
#107306=CARTESIAN_POINT('',(0.179857635894567,-3.85734623443633,-9.66)) ;
#107307=CARTESIAN_POINT('Origin',(0.5,2.29999999999999,-9.66)) ;
#107308=CARTESIAN_POINT('',(0.500000000000001,2.29999999999999,-9.76)) ;
#107309=CARTESIAN_POINT('',(0.5,-3.36847777691809,-9.76)) ;
#107310=CARTESIAN_POINT('',(0.5,-3.4,-9.76)) ;
#107311=CARTESIAN_POINT('',(0.5,-3.36847777691809,-10.56)) ;
#107312=CARTESIAN_POINT('',(0.5,-3.36847777691809,-9.66)) ;
#107313=CARTESIAN_POINT('',(0.500000000000001,2.29999999999999,-10.56)) ;
#107314=CARTESIAN_POINT('',(0.5,2.29999999999999,-10.56)) ;
#107315=CARTESIAN_POINT('',(0.500000000000001,2.29999999999999,-9.66)) ;
#107316=CARTESIAN_POINT('Origin',(1.5,2.3,-9.66)) ;
#107317=CARTESIAN_POINT('Origin',(1.5,2.3,-9.76)) ;
#107318=CARTESIAN_POINT('Origin',(1.5,2.3,-10.56)) ;
#107319=CARTESIAN_POINT('Origin',(8.,2.68967221921331,-10.66)) ;
#107320=CARTESIAN_POINT('',(8.45734623443633,3.70206555615734,-10.3398576358946)) ;
#107321=CARTESIAN_POINT('',(8.02582401135442,3.4,-10.6419231920519)) ;
#107322=CARTESIAN_POINT('',(7.75526480758232,3.21060855735952,-10.8313146346924)) ;
#107323=CARTESIAN_POINT('',(8.02582401135442,4.2,-10.6419231920519)) ;
#107324=CARTESIAN_POINT('',(8.02582401135442,2.68967221921331,-10.6419231920519)) ;
#107325=CARTESIAN_POINT('',(8.45734623443633,3.89793444384266,-10.3398576358946)) ;
#107326=CARTESIAN_POINT('',(8.54034505662341,3.83983526831171,-10.2817584603636)) ;
#107327=CARTESIAN_POINT('',(8.45734623443633,2.68967221921331,-10.3398576358946)) ;
#107328=CARTESIAN_POINT('Origin',(8.,2.68967221921331,-9.66)) ;
#107329=CARTESIAN_POINT('',(8.45734623443633,3.89793444384266,-9.98014236410544)) ;
#107330=CARTESIAN_POINT('',(8.02582401135442,4.2,-9.6780768079481)) ;
#107331=CARTESIAN_POINT('',(8.54034505662341,3.83983526831171,-10.0382415396364)) ;
#107332=CARTESIAN_POINT('',(8.02582401135442,3.4,-9.6780768079481)) ;
#107333=CARTESIAN_POINT('',(8.02582401135442,3.4,-9.6780768079481)) ;
#107334=CARTESIAN_POINT('',(8.45734623443633,3.70206555615734,-9.98014236410544)) ;
#107335=CARTESIAN_POINT('',(7.75526480758232,3.21060855735952,-9.48868536530762)) ;
#107336=CARTESIAN_POINT('',(8.45734623443633,2.68967221921331,-9.98014236410544)) ;
#107337=CARTESIAN_POINT('Origin',(-1.11032778078669,-3.9,-10.01)) ;
#107338=CARTESIAN_POINT('',(0.0979344438426626,-3.85734623443633,-9.98014236410544)) ;
#107339=CARTESIAN_POINT('',(0.4,-3.42582401135442,-9.6780768079481)) ;
#107340=CARTESIAN_POINT('',(-0.223548570072128,-4.31660768288603,-10.3016253780202)) ;
#107341=CARTESIAN_POINT('',(-0.400000000000001,-3.42582401135442,-9.6780768079481)) ;
#107342=CARTESIAN_POINT('',(-0.400000000000001,-3.42582401135442,-9.6780768079481)) ;
#107343=CARTESIAN_POINT('',(-0.0979344438426627,-3.85734623443633,-9.98014236410544)) ;
#107344=CARTESIAN_POINT('',(-0.326007604256636,-3.53152743384494,-9.75206920369146)) ;
#107345=CARTESIAN_POINT('',(-1.11032778078669,-3.85734623443633,-9.98014236410544)) ;
#107346=CARTESIAN_POINT('Origin',(-1.11032778078669,-3.4,-10.66)) ;
#107347=CARTESIAN_POINT('',(-0.0979344438426627,-3.85734623443633,-10.3398576358946)) ;
#107348=CARTESIAN_POINT('',(-0.4,-3.42582401135442,-10.6419231920519)) ;
#107349=CARTESIAN_POINT('',(-0.589391442640475,-3.15526480758232,-10.8313146346924)) ;
#107350=CARTESIAN_POINT('',(0.400000000000001,-3.42582401135442,-10.6419231920519)) ;
#107351=CARTESIAN_POINT('',(-1.11032778078669,-3.42582401135442,-10.6419231920519)) ;
#107352=CARTESIAN_POINT('',(0.0979344438426626,-3.85734623443633,-10.3398576358946)) ;
#107353=CARTESIAN_POINT('',(0.0398352683117103,-3.94034505662341,-10.2817584603636)) ;
#107354=CARTESIAN_POINT('',(-1.11032778078669,-3.85734623443633,-10.3398576358946)) ;
#107355=CARTESIAN_POINT('Origin',(10.,1.24999999999998,-12.7)) ;
#107356=CARTESIAN_POINT('',(9.91643989873054,1.26392668354489,-8.1158381198218)) ;
#107357=CARTESIAN_POINT('',(9.91643989873054,1.26392668354489,-12.7)) ;
#107358=CARTESIAN_POINT('',(8.50816364570057,1.49863939238321,-8.19785831296513)) ;
#107359=CARTESIAN_POINT('Origin',(43.705291680055,-4.36754861360758,-616.848202367929)) ;
#107360=CARTESIAN_POINT('',(8.50816364570057,1.49863939238321,-12.7)) ;
#107361=CARTESIAN_POINT('Origin',(8.49999999999985,3.8,-10.16)) ;
#107362=CARTESIAN_POINT('',(9.91643989873053,1.24322097942674,-8.17630356419405)) ;
#107363=CARTESIAN_POINT('',(9.91643989873053,1.24322097942648,-12.1436964358056)) ;
#107364=CARTESIAN_POINT('Origin',(9.91643989873053,3.8,-10.16)) ;
#107365=CARTESIAN_POINT('Origin',(36.548065263586,-40.3802619823314,562.117654689231)) ;
#107366=CARTESIAN_POINT('Origin',(36.5480653710647,-40.3802615702808,-582.437655339515)) ;
#107367=CARTESIAN_POINT('Origin',(10.,1.24999999999998,-12.7)) ;
#107368=CARTESIAN_POINT('',(8.50816364570059,1.49863939238321,-12.1221416870347)) ;
#107369=CARTESIAN_POINT('',(8.50816364570057,1.49863939238321,-12.7)) ;
#107370=CARTESIAN_POINT('',(9.91643989873054,1.26392668354489,-12.2041618801782)) ;
#107371=CARTESIAN_POINT('Origin',(43.7052916277413,-4.36754860543838,596.528201456572)) ;
#107372=CARTESIAN_POINT('',(9.91643989873054,1.26392668354489,-12.7)) ;
#107373=CARTESIAN_POINT('Origin',(-0.900000000000001,4.65,-10.16)) ;
#107374=CARTESIAN_POINT('Origin',(-0.900000000000001,4.65,-8.5168323274845)) ;
#107375=CARTESIAN_POINT('Origin',(-0.900000000000001,4.65,-8.5168323274845)) ;
#107376=CARTESIAN_POINT('Origin',(-0.900000000000001,4.65,-8.5168323274845)) ;
#107377=CARTESIAN_POINT('Origin',(-0.900000000000001,4.65,-8.5168323274845)) ;
#107378=CARTESIAN_POINT('Origin',(1.15,4.45,-8.57886116991581)) ;
#107379=CARTESIAN_POINT('Origin',(1.15,4.45,-8.5168323274845)) ;
#107380=CARTESIAN_POINT('Origin',(-1.,4.65,-8.5168323274845)) ;
#107381=CARTESIAN_POINT('Origin',(1.15,4.65,-8.5168323274845)) ;
#107382=CARTESIAN_POINT('Origin',(-0.900000000000001,3.8,-10.16)) ;
#107383=CARTESIAN_POINT('Origin',(-0.900000000000001,5.4431676725155,-9.31)) ;
#107384=CARTESIAN_POINT('Origin',(1.15,4.65,-8.5168323274845)) ;
#107385=CARTESIAN_POINT('Origin',(1.15,4.55810810810811,-8.69447207586456)) ;
#107386=CARTESIAN_POINT('Origin',(-0.900000000000001,5.4431676725155,-9.31)) ;
#107387=CARTESIAN_POINT('Origin',(-0.900000000000001,5.4431676725155,-9.31)) ;
#107388=CARTESIAN_POINT('Origin',(-0.900000000000001,5.4431676725155,-9.31)) ;
#107389=CARTESIAN_POINT('Origin',(-0.900000000000001,4.65,-10.16)) ;
#107390=CARTESIAN_POINT('Origin',(-0.900000000000001,4.65,-11.8031676725155)) ;
#107391=CARTESIAN_POINT('Origin',(-1.,4.65,-11.8031676725155)) ;
#107392=CARTESIAN_POINT('Origin',(1.15,4.65,-11.8031676725155)) ;
#107393=CARTESIAN_POINT('Origin',(-0.900000000000001,4.65,-11.8031676725155)) ;
#107394=CARTESIAN_POINT('Origin',(1.15,4.45,-11.7411388300842)) ;
#107395=CARTESIAN_POINT('Origin',(1.15,4.45,-11.8031676725155)) ;
#107396=CARTESIAN_POINT('Origin',(1.15,3.8,-10.16)) ;
#107397=CARTESIAN_POINT('Origin',(1.15,5.26552792413544,-9.40189189189189)) ;
#107398=CARTESIAN_POINT('Origin',(-1.,5.4431676725155,-9.31)) ;
#107399=CARTESIAN_POINT('Origin',(1.15,5.4431676725155,-9.31)) ;
#107400=CARTESIAN_POINT('Origin',(-0.900000000000001,3.8,-9.31)) ;
#107401=CARTESIAN_POINT('Origin',(-0.9,6.45,-9.31)) ;
#107402=CARTESIAN_POINT('Origin',(-0.9,6.45,-10.16)) ;
#107403=CARTESIAN_POINT('Origin',(-0.9,6.45,-9.31)) ;
#107404=CARTESIAN_POINT('Origin',(-0.900000000000001,4.65,-11.8031676725155)) ;
#107405=CARTESIAN_POINT('Origin',(-0.900000000000001,4.65,-11.8031676725155)) ;
#107406=CARTESIAN_POINT('Origin',(1.15,4.65,-11.8031676725155)) ;
#107407=CARTESIAN_POINT('Origin',(1.15,4.55810810810811,-11.6255279241354)) ;
#107408=CARTESIAN_POINT('Origin',(1.15,5.4431676725155,-9.31)) ;
#107409=CARTESIAN_POINT('Origin',(1.15,5.4431676725155,-9.51)) ;
#107410=CARTESIAN_POINT('Origin',(-0.9,6.45,-9.31)) ;
#107411=CARTESIAN_POINT('Origin',(-0.9,6.45,-9.31)) ;
#107412=CARTESIAN_POINT('Origin',(-0.900000000000001,3.8,-10.16)) ;
#107413=CARTESIAN_POINT('Origin',(-0.900000000000001,5.4431676725155,-11.01)) ;
#107414=CARTESIAN_POINT('Origin',(-1.,5.4431676725155,-11.01)) ;
#107415=CARTESIAN_POINT('Origin',(1.15,5.4431676725155,-11.01)) ;
#107416=CARTESIAN_POINT('Origin',(-0.900000000000001,5.4431676725155,-11.01)) ;
#107417=CARTESIAN_POINT('Origin',(1.15,3.8,-10.16)) ;
#107418=CARTESIAN_POINT('Origin',(1.15,5.26552792413544,-10.9181081081081)) ;
#107419=CARTESIAN_POINT('Origin',(1.15,6.55,-9.51)) ;
#107420=CARTESIAN_POINT('Origin',(1.15,6.45,-9.51)) ;
#107421=CARTESIAN_POINT('Origin',(1.25,6.45,-9.31)) ;
#107422=CARTESIAN_POINT('Origin',(1.15,6.45,-9.31)) ;
#107423=CARTESIAN_POINT('Origin',(-0.900000000000001,5.4431676725155,-11.01)) ;
#107424=CARTESIAN_POINT('Origin',(-0.900000000000001,5.4431676725155,-11.01)) ;
#107425=CARTESIAN_POINT('Origin',(1.15,5.4431676725155,-11.01)) ;
#107426=CARTESIAN_POINT('Origin',(1.15,5.4431676725155,-10.81)) ;
#107427=CARTESIAN_POINT('Origin',(1.15,6.45,-9.51)) ;
#107428=CARTESIAN_POINT('Origin',(1.35,6.45,-9.51)) ;
#107429=CARTESIAN_POINT('Origin',(-0.9,6.45,-10.16)) ;
#107430=CARTESIAN_POINT('Origin',(-0.9,6.45,-11.01)) ;
#107431=CARTESIAN_POINT('Origin',(-0.900000000000001,3.8,-11.01)) ;
#107432=CARTESIAN_POINT('Origin',(-0.9,6.45,-11.01)) ;
#107433=CARTESIAN_POINT('Origin',(1.15,6.55,-10.81)) ;
#107434=CARTESIAN_POINT('Origin',(1.15,6.45,-10.81)) ;
#107435=CARTESIAN_POINT('Origin',(1.35,6.45,-12.7)) ;
#107436=CARTESIAN_POINT('Origin',(1.35,6.45,-10.81)) ;
#107437=CARTESIAN_POINT('Origin',(-0.9,6.45,-11.01)) ;
#107438=CARTESIAN_POINT('Origin',(-0.9,6.45,-11.01)) ;
#107439=CARTESIAN_POINT('Origin',(1.15,6.45,-10.81)) ;
#107440=CARTESIAN_POINT('Origin',(1.15,6.45,-11.01)) ;
#107441=CARTESIAN_POINT('Origin',(-1.,6.45,-11.01)) ;
#107442=CARTESIAN_POINT('Origin',(-1.7,0.3,-10.81)) ;
#107443=CARTESIAN_POINT('Origin',(-1.7,0.3,-10.81)) ;
#107444=CARTESIAN_POINT('Origin',(-1.7,0.3,-10.81)) ;
#107445=CARTESIAN_POINT('Origin',(-1.7,0.3,-10.81)) ;
#107446=CARTESIAN_POINT('Origin',(0.549999999999999,0.3,-10.81)) ;
#107447=CARTESIAN_POINT('',(0.50857864376269,0.229289321881345,-10.7392893218813)) ;
#107448=CARTESIAN_POINT('Ctrl Pts',(0.65,0.200000000000001,-10.81)) ;
#107449=CARTESIAN_POINT('Ctrl Pts',(0.639834283464158,0.200000000000001,
-10.8049171417321)) ;
#107450=CARTESIAN_POINT('Ctrl Pts',(0.629316849080552,0.200389688120421,
-10.799657683858)) ;
#107451=CARTESIAN_POINT('Ctrl Pts',(0.606957334719714,0.202165884217636,
-10.7884679497194)) ;
#107452=CARTESIAN_POINT('Ctrl Pts',(0.595086727401161,0.203647820493433,
-10.782522761795)) ;
#107453=CARTESIAN_POINT('Ctrl Pts',(0.572283837383465,0.207685608830711,
-10.7711067603976)) ;
#107454=CARTESIAN_POINT('Ctrl Pts',(0.561337481656325,0.210178193246981,
-10.765629861311)) ;
#107455=CARTESIAN_POINT('Ctrl Pts',(0.549549942891011,0.213544620663898,
-10.7597406960422)) ;
#107456=CARTESIAN_POINT('Ctrl Pts',(0.548290718948482,0.213913346521136,
-10.7591116827675)) ;
#107457=CARTESIAN_POINT('Ctrl Pts',(0.536119229732729,0.217566912232509,
-10.7530327513518)) ;
#107458=CARTESIAN_POINT('Ctrl Pts',(0.525706917362472,0.221400308602604,
-10.7478422384291)) ;
#107459=CARTESIAN_POINT('Ctrl Pts',(0.513545110027223,0.226871185484677,
-10.7417711869643)) ;
#107460=CARTESIAN_POINT('Ctrl Pts',(0.511029334128303,0.228063976698517,
-10.7405146670642)) ;
#107461=CARTESIAN_POINT('Ctrl Pts',(0.50857864376269,0.229289321881369,
-10.7392893218813)) ;
#107462=CARTESIAN_POINT('Origin',(0.664280054289791,0.302990743360187,-10.8171421042438)) ;
#107463=CARTESIAN_POINT('Origin',(-1.7,4.5,-10.81)) ;
#107464=CARTESIAN_POINT('',(-1.77071067811864,4.45857864376272,-10.7392893218813)) ;
#107465=CARTESIAN_POINT('Origin',(-1.69703459697676,4.61417009504429,-10.8170866853763)) ;
#107466=CARTESIAN_POINT('Ctrl Pts',(-1.77071067811862,4.45857864376272,
-10.7392893218813)) ;
#107467=CARTESIAN_POINT('Ctrl Pts',(-1.77521675558369,4.46759079869279,
-10.7437953993464)) ;
#107468=CARTESIAN_POINT('Ctrl Pts',(-1.77928079264421,4.47748625817292,
-10.7487264816716)) ;
#107469=CARTESIAN_POINT('Ctrl Pts',(-1.78624680748783,4.49811277057336,
-10.7590208825501)) ;
#107470=CARTESIAN_POINT('Ctrl Pts',(-1.78918030782056,4.50880509434443,
-10.7643639841539)) ;
#107471=CARTESIAN_POINT('Ctrl Pts',(-1.79185985500503,4.52101859323025,
-10.7704747545378)) ;
#107472=CARTESIAN_POINT('Ctrl Pts',(-1.7921304506133,4.52228751723201,-10.7711097099114)) ;
#107473=CARTESIAN_POINT('Ctrl Pts',(-1.7947746790983,4.53504937002863,-10.777496289134)) ;
#107474=CARTESIAN_POINT('Ctrl Pts',(-1.79657370273653,4.54677936428204,
-10.7833715724062)) ;
#107475=CARTESIAN_POINT('Ctrl Pts',(-1.79896007643136,4.56920025888396,
-10.7945957747612)) ;
#107476=CARTESIAN_POINT('Ctrl Pts',(-1.79963010255188,4.57990192168158,
-10.799950075945)) ;
#107477=CARTESIAN_POINT('Ctrl Pts',(-1.79996164986962,4.593571160343,-10.806785573817)) ;
#107478=CARTESIAN_POINT('Ctrl Pts',(-1.8,4.59680282631916,-10.8084014131596)) ;
#107479=CARTESIAN_POINT('Ctrl Pts',(-1.8,4.6,-10.81)) ;
#107480=CARTESIAN_POINT('Origin',(-1.7,0.3,-10.16)) ;
#107481=CARTESIAN_POINT('Origin',(-1.7,0.3,-11.56)) ;
#107482=CARTESIAN_POINT('Origin',(0.65,0.3,-10.16)) ;
#107483=CARTESIAN_POINT('',(0.579289321881328,0.229289321881363,-10.6685786437627)) ;
#107484=CARTESIAN_POINT('Origin',(0.657086685372617,0.30296540302162,-10.8241700950363)) ;
#107485=CARTESIAN_POINT('Ctrl Pts',(0.579289321881328,0.229289321881363,
-10.6685786437627)) ;
#107486=CARTESIAN_POINT('Ctrl Pts',(0.583795399346358,0.22478324441633,
-10.6775907986928)) ;
#107487=CARTESIAN_POINT('Ctrl Pts',(0.588726481671642,0.220719207355776,
-10.6874862581729)) ;
#107488=CARTESIAN_POINT('Ctrl Pts',(0.599020882547812,0.213753192513727,
-10.7081127705688)) ;
#107489=CARTESIAN_POINT('Ctrl Pts',(0.604363984149138,0.21081969218206,
-10.7188050943348)) ;
#107490=CARTESIAN_POINT('Ctrl Pts',(0.610474754532864,0.208140144997068,
-10.7310185932204)) ;
#107491=CARTESIAN_POINT('Ctrl Pts',(0.611109709908962,0.20786954938772,
-10.7322875172271)) ;
#107492=CARTESIAN_POINT('Ctrl Pts',(0.617496289133932,0.205225320901711,
-10.7450493700286)) ;
#107493=CARTESIAN_POINT('Ctrl Pts',(0.623371572406165,0.203426297263479,
-10.756779364282)) ;
#107494=CARTESIAN_POINT('Ctrl Pts',(0.634595774761169,0.201039923568646,
-10.7792002588839)) ;
#107495=CARTESIAN_POINT('Ctrl Pts',(0.639950075944996,0.200369897448124,
-10.7899019216815)) ;
#107496=CARTESIAN_POINT('Ctrl Pts',(0.646785573817028,0.200038350130376,
-10.803571160343)) ;
#107497=CARTESIAN_POINT('Ctrl Pts',(0.648401413159574,0.2,-10.8068028263192)) ;
#107498=CARTESIAN_POINT('Ctrl Pts',(0.65,0.2,-10.81)) ;
#107499=CARTESIAN_POINT('',(0.579289321881328,0.229289321881363,-9.65142135623727)) ;
#107500=CARTESIAN_POINT('Ctrl Pts',(0.65,0.2,-9.51)) ;
#107501=CARTESIAN_POINT('Ctrl Pts',(0.644917141732078,0.2,-9.52016571653583)) ;
#107502=CARTESIAN_POINT('Ctrl Pts',(0.639657683858005,0.200389688120423,
-9.53068315091943)) ;
#107503=CARTESIAN_POINT('Ctrl Pts',(0.628467949719355,0.202165884217645,
-9.55304266528024)) ;
#107504=CARTESIAN_POINT('Ctrl Pts',(0.622522761794952,0.203647820493437,
-9.56491327259877)) ;
#107505=CARTESIAN_POINT('Ctrl Pts',(0.611106760396028,0.207685608831252,
-9.58771616261943)) ;
#107506=CARTESIAN_POINT('Ctrl Pts',(0.605629861308049,0.210178193248326,
-9.59866251834949)) ;
#107507=CARTESIAN_POINT('Ctrl Pts',(0.599740696039329,0.213544620665554,
-9.61045005711456)) ;
#107508=CARTESIAN_POINT('Ctrl Pts',(0.599111682766057,0.213913346521985,
-9.61170928105426)) ;
#107509=CARTESIAN_POINT('Ctrl Pts',(0.593032751351777,0.217566912232531,
-9.62388077026723)) ;
#107510=CARTESIAN_POINT('Ctrl Pts',(0.58784223842912,0.221400308602597,
-9.6342930826375)) ;
#107511=CARTESIAN_POINT('Ctrl Pts',(0.581771186964294,0.226871185484689,
-9.64645488997275)) ;
#107512=CARTESIAN_POINT('Ctrl Pts',(0.580514667064131,0.228063976698559,
-9.64897066587166)) ;
#107513=CARTESIAN_POINT('Ctrl Pts',(0.579289321881328,0.229289321881363,
-9.65142135623727)) ;
#107514=CARTESIAN_POINT('Origin',(0.657142104258034,0.302990743365752,-9.49571994568188)) ;
#107515=CARTESIAN_POINT('Origin',(-1.7,4.6,-10.71)) ;
#107516=CARTESIAN_POINT('',(-1.77071067811866,4.52928932188135,-10.6685786437627)) ;
#107517=CARTESIAN_POINT('Ctrl Pts',(-1.8,4.6,-10.81)) ;
#107518=CARTESIAN_POINT('Ctrl Pts',(-1.8,4.59491714173208,-10.7998342834642)) ;
#107519=CARTESIAN_POINT('Ctrl Pts',(-1.79961031187958,4.58965768385801,
-10.7893168490806)) ;
#107520=CARTESIAN_POINT('Ctrl Pts',(-1.79783411578236,4.57846794971936,
-10.7669573347197)) ;
#107521=CARTESIAN_POINT('Ctrl Pts',(-1.79635217950656,4.57252276179495,
-10.7550867274012)) ;
#107522=CARTESIAN_POINT('Ctrl Pts',(-1.79231439116873,4.56110676039597,
-10.7322838373804)) ;
#107523=CARTESIAN_POINT('Ctrl Pts',(-1.78982180675163,4.55562986130795,
-10.7213374816503)) ;
#107524=CARTESIAN_POINT('Ctrl Pts',(-1.78645537933439,4.54974069603923,
-10.7095499428852)) ;
#107525=CARTESIAN_POINT('Ctrl Pts',(-1.78608665347798,4.549111682766,-10.7082907189456)) ;
#107526=CARTESIAN_POINT('Ctrl Pts',(-1.78243308776746,4.54303275135177,
-10.6961192297327)) ;
#107527=CARTESIAN_POINT('Ctrl Pts',(-1.7785996913974,4.53784223842912,-10.6857069173624)) ;
#107528=CARTESIAN_POINT('Ctrl Pts',(-1.77312881451532,4.5317711869643,-10.6735451100272)) ;
#107529=CARTESIAN_POINT('Ctrl Pts',(-1.77193602330145,4.53051466706415,
-10.6710293341283)) ;
#107530=CARTESIAN_POINT('Ctrl Pts',(-1.77071067811866,4.52928932188135,
-10.6685786437627)) ;
#107531=CARTESIAN_POINT('Origin',(-1.69700925662349,4.60714210428443,-10.8242800543711)) ;
#107532=CARTESIAN_POINT('',(-1.77071067811866,4.52928932188135,-9.65142135623731)) ;
#107533=CARTESIAN_POINT('Origin',(-1.69703459696962,4.60708668539217,-9.49582990492436)) ;
#107534=CARTESIAN_POINT('Ctrl Pts',(-1.77071067811866,4.52928932188135,
-9.65142135623731)) ;
#107535=CARTESIAN_POINT('Ctrl Pts',(-1.77521675558367,4.53379539934636,
-9.64240920130727)) ;
#107536=CARTESIAN_POINT('Ctrl Pts',(-1.77928079264422,4.53872648167163,
-9.63251374182715)) ;
#107537=CARTESIAN_POINT('Ctrl Pts',(-1.7862468074862,4.5490208825477,-9.61188722943147)) ;
#107538=CARTESIAN_POINT('Ctrl Pts',(-1.78918030781783,4.55436398414893,
-9.60119490566563)) ;
#107539=CARTESIAN_POINT('Ctrl Pts',(-1.79185985500284,4.56047475453265,
-9.58898140678007)) ;
#107540=CARTESIAN_POINT('Ctrl Pts',(-1.79213045061223,4.56110970990885,
-9.58771248277321)) ;
#107541=CARTESIAN_POINT('Ctrl Pts',(-1.79477467909829,4.56749628913393,
-9.57495062997146)) ;
#107542=CARTESIAN_POINT('Ctrl Pts',(-1.79657370273652,4.57337157240617,
-9.56322063571803)) ;
#107543=CARTESIAN_POINT('Ctrl Pts',(-1.79896007643136,4.58459577476118,
-9.54079974111609)) ;
#107544=CARTESIAN_POINT('Ctrl Pts',(-1.79963010255188,4.58995007594501,
-9.53009807831846)) ;
#107545=CARTESIAN_POINT('Ctrl Pts',(-1.79996164986962,4.59678557381704,
-9.51642883965702)) ;
#107546=CARTESIAN_POINT('Ctrl Pts',(-1.8,4.59840141315958,-9.51319717368085)) ;
#107547=CARTESIAN_POINT('Ctrl Pts',(-1.8,4.6,-9.51)) ;
#107548=CARTESIAN_POINT('Origin',(-1.7,0.3,-11.56)) ;
#107549=CARTESIAN_POINT('Origin',(-1.7,0.1,-11.56)) ;
#107550=CARTESIAN_POINT('Origin',(-1.9,0.3,-11.56)) ;
#107551=CARTESIAN_POINT('Origin',(1.9668402209837E-32,0.1,-11.56)) ;
#107552=CARTESIAN_POINT('',(0.899999999999999,0.1,-11.66)) ;
#107553=CARTESIAN_POINT('',(-1.8,0.1,-11.66)) ;
#107554=CARTESIAN_POINT('Origin',(0.899999999999999,0.1,-11.56)) ;
#107555=CARTESIAN_POINT('Origin',(0.899999999999999,0.1,-11.56)) ;
#107556=CARTESIAN_POINT('',(0.999999999999999,0.1,-11.56)) ;
#107557=CARTESIAN_POINT('Origin',(0.899999999999999,0.1,-11.56)) ;
#107558=CARTESIAN_POINT('Origin',(0.899999999999999,0.1,-11.56)) ;
#107559=CARTESIAN_POINT('Origin',(0.549999999999999,0.3,-9.51)) ;
#107560=CARTESIAN_POINT('',(0.508578643762691,0.229289321881345,-9.58071067811866)) ;
#107561=CARTESIAN_POINT('Origin',(0.664170095055986,0.302965403025977,-9.50291331461772)) ;
#107562=CARTESIAN_POINT('Ctrl Pts',(0.50857864376269,0.229289321881343,
-9.58071067811865)) ;
#107563=CARTESIAN_POINT('Ctrl Pts',(0.517590798692746,0.224783244416322,
-9.57620460065363)) ;
#107564=CARTESIAN_POINT('Ctrl Pts',(0.527486258172873,0.220719207355776,
-9.57127351832836)) ;
#107565=CARTESIAN_POINT('Ctrl Pts',(0.548112770568385,0.213753192513845,
-9.56097911745236)) ;
#107566=CARTESIAN_POINT('Ctrl Pts',(0.558805094334016,0.210819692182259,
-9.55563601585123)) ;
#107567=CARTESIAN_POINT('Ctrl Pts',(0.571018593219555,0.208140144997224,
-9.5495252454675)) ;
#107568=CARTESIAN_POINT('Ctrl Pts',(0.572287517226615,0.207869549387789,
-9.54889029009121)) ;
#107569=CARTESIAN_POINT('Ctrl Pts',(0.585049370028563,0.205225320901693,
-9.54250371086602)) ;
#107570=CARTESIAN_POINT('Ctrl Pts',(0.596779364281993,0.203426297263461,
-9.53662842759377)) ;
#107571=CARTESIAN_POINT('Ctrl Pts',(0.619200258883917,0.201039923568636,
-9.52540422523876)) ;
#107572=CARTESIAN_POINT('Ctrl Pts',(0.629901921681539,0.20036989744812,
-9.52004992405495)) ;
#107573=CARTESIAN_POINT('Ctrl Pts',(0.643571160342975,0.200038350130376,
-9.51321442618296)) ;
#107574=CARTESIAN_POINT('Ctrl Pts',(0.646802826319151,0.200000000000001,
-9.51159858684042)) ;
#107575=CARTESIAN_POINT('Ctrl Pts',(0.65,0.200000000000001,-9.51)) ;
#107576=CARTESIAN_POINT('Origin',(-1.7,0.3,-9.51)) ;
#107577=CARTESIAN_POINT('Origin',(-1.7,4.5,-9.51)) ;
#107578=CARTESIAN_POINT('',(-1.77071067811864,4.45857864376272,-9.58071067811867)) ;
#107579=CARTESIAN_POINT('Ctrl Pts',(-1.8,4.6,-9.51)) ;
#107580=CARTESIAN_POINT('Ctrl Pts',(-1.8,4.58983428346417,-9.51508285826792)) ;
#107581=CARTESIAN_POINT('Ctrl Pts',(-1.79961031187958,4.57931684908058,
-9.52034231614199)) ;
#107582=CARTESIAN_POINT('Ctrl Pts',(-1.79783411578236,4.55695733471976,
-9.53153205028064)) ;
#107583=CARTESIAN_POINT('Ctrl Pts',(-1.79635217950656,4.54508672740121,
-9.53747723820505)) ;
#107584=CARTESIAN_POINT('Ctrl Pts',(-1.7923143911688,4.52228383738083,-9.54889323960384)) ;
#107585=CARTESIAN_POINT('Ctrl Pts',(-1.7898218067518,4.51133748165105,-9.55437013869168)) ;
#107586=CARTESIAN_POINT('Ctrl Pts',(-1.7864553793346,4.49954994288596,-9.56025930396041)) ;
#107587=CARTESIAN_POINT('Ctrl Pts',(-1.78608665347809,4.49829071894599,
-9.56088831723382)) ;
#107588=CARTESIAN_POINT('Ctrl Pts',(-1.78243308776746,4.48611922973275,
-9.56696724864823)) ;
#107589=CARTESIAN_POINT('Ctrl Pts',(-1.7785996913974,4.47570691736247,-9.57215776157089)) ;
#107590=CARTESIAN_POINT('Ctrl Pts',(-1.77312881451531,4.46354511002723,
-9.57822881303571)) ;
#107591=CARTESIAN_POINT('Ctrl Pts',(-1.77193602330144,4.46102933412832,
-9.57948533293587)) ;
#107592=CARTESIAN_POINT('Ctrl Pts',(-1.77071067811864,4.45857864376272,
-9.58071067811867)) ;
#107593=CARTESIAN_POINT('Origin',(-1.69700925663781,4.61428005430337,-9.50285789574935)) ;
#107594=CARTESIAN_POINT('Origin',(-1.7,0.3,-9.51)) ;
#107595=CARTESIAN_POINT('Origin',(-1.9,-4.11004745125224E-16,-11.56)) ;
#107596=CARTESIAN_POINT('',(-1.9,6.9,-11.66)) ;
#107597=CARTESIAN_POINT('Origin',(-1.9,6.9,-11.56)) ;
#107598=CARTESIAN_POINT('',(-1.9,7.,-11.66)) ;
#107599=CARTESIAN_POINT('Origin',(-2.,0.1,-11.76)) ;
#107600=CARTESIAN_POINT('Origin',(-1.89999999999984,0.100000000000157,-11.7600000000001)) ;
#107601=CARTESIAN_POINT('Origin',(0.899999999999999,0.1,-11.76)) ;
#107602=CARTESIAN_POINT('Origin',(0.899999999999999,0.1,-11.56)) ;
#107603=CARTESIAN_POINT('Origin',(1.1,0.1,-11.56)) ;
#107604=CARTESIAN_POINT('Origin',(0.899999999999999,0.1,-10.16)) ;
#107605=CARTESIAN_POINT('',(0.999999999999999,0.1,-8.76)) ;
#107606=CARTESIAN_POINT('',(0.999999999999999,0.1,-11.66)) ;
#107607=CARTESIAN_POINT('Origin',(0.899999999999999,0.1,-8.76)) ;
#107608=CARTESIAN_POINT('Origin',(-1.7,0.3,-9.51)) ;
#107609=CARTESIAN_POINT('Origin',(-1.7,0.3,-9.51)) ;
#107610=CARTESIAN_POINT('Origin',(-1.9,6.9,-11.56)) ;
#107611=CARTESIAN_POINT('',(-1.9,7.,-11.56)) ;
#107612=CARTESIAN_POINT('Origin',(-1.9,6.9,-11.56)) ;
#107613=CARTESIAN_POINT('Origin',(-1.9,6.9,-11.56)) ;
#107614=CARTESIAN_POINT('Origin',(-1.9,7.,-11.76)) ;
#107615=CARTESIAN_POINT('Origin',(-1.9,6.9,-11.76)) ;
#107616=CARTESIAN_POINT('Origin',(1.1,0.1,-8.66)) ;
#107617=CARTESIAN_POINT('Origin',(1.1,0.1,-8.76)) ;
#107618=CARTESIAN_POINT('Origin',(0.899999999999999,0.1,-8.76)) ;
#107619=CARTESIAN_POINT('',(0.899999999999999,0.1,-8.66)) ;
#107620=CARTESIAN_POINT('Origin',(0.899999999999999,0.1,-8.76)) ;
#107621=CARTESIAN_POINT('Origin',(0.899999999999999,0.1,-8.76)) ;
#107622=CARTESIAN_POINT('Origin',(-1.7,0.3,-10.16)) ;
#107623=CARTESIAN_POINT('Origin',(-1.7,0.3,-8.76)) ;
#107624=CARTESIAN_POINT('Origin',(-1.9,6.9,-10.16)) ;
#107625=CARTESIAN_POINT('',(-1.9,7.,-8.76)) ;
#107626=CARTESIAN_POINT('Origin',(-1.9,6.9,-8.76)) ;
#107627=CARTESIAN_POINT('',(-1.9,7.,-11.66)) ;
#107628=CARTESIAN_POINT('Origin',(-1.9,6.9,-11.56)) ;
#107629=CARTESIAN_POINT('Origin',(-1.9,7.1,-11.56)) ;
#107630=CARTESIAN_POINT('Origin',(0.899999999999999,0.1,-8.76)) ;
#107631=CARTESIAN_POINT('Origin',(0.899999999999999,0.1,-8.56)) ;
#107632=CARTESIAN_POINT('Origin',(-1.9668402209837E-32,0.1,-8.76)) ;
#107633=CARTESIAN_POINT('',(0.999999999999999,0.1,-8.66)) ;
#107634=CARTESIAN_POINT('Origin',(-1.7,0.1,-8.76)) ;
#107635=CARTESIAN_POINT('Origin',(-1.7,0.3,-8.76)) ;
#107636=CARTESIAN_POINT('Origin',(-1.9,0.3,-8.76)) ;
#107637=CARTESIAN_POINT('Origin',(-1.9,6.9,-8.76)) ;
#107638=CARTESIAN_POINT('',(-1.9,6.9,-8.66)) ;
#107639=CARTESIAN_POINT('Origin',(-1.9,6.9,-8.76)) ;
#107640=CARTESIAN_POINT('Origin',(-1.9,6.9,-8.76)) ;
#107641=CARTESIAN_POINT('Origin',(-1.9,7.1,-11.66)) ;
#107642=CARTESIAN_POINT('Origin',(-1.9,7.1,-8.76)) ;
#107643=CARTESIAN_POINT('Origin',(-1.8,0.1,-8.56)) ;
#107644=CARTESIAN_POINT('Origin',(-1.90000000000002,0.0999999999999822,
-8.56000000000002)) ;
#107645=CARTESIAN_POINT('Origin',(-1.9,-6.40600499298624E-17,-8.76)) ;
#107646=CARTESIAN_POINT('',(-1.9,7.,-8.66)) ;
#107647=CARTESIAN_POINT('Origin',(-1.9,6.9,-8.76)) ;
#107648=CARTESIAN_POINT('Origin',(-1.9,6.9,-8.56)) ;
#107649=CARTESIAN_POINT('Origin',(-1.9,7.,-8.56)) ;
#107650=CARTESIAN_POINT('Origin',(-0.900000000000002,2.95,-10.16)) ;
#107651=CARTESIAN_POINT('Origin',(-0.900000000000001,2.95,-11.8031676725155)) ;
#107652=CARTESIAN_POINT('Origin',(-0.900000000000002,2.95,-11.8031676725155)) ;
#107653=CARTESIAN_POINT('Origin',(-0.900000000000001,2.95,-11.8031676725155)) ;
#107654=CARTESIAN_POINT('Origin',(-0.900000000000002,2.95,-11.8031676725155)) ;
#107655=CARTESIAN_POINT('Origin',(1.15,3.15,-12.71)) ;
#107656=CARTESIAN_POINT('Origin',(1.15,3.15,-11.8031676725155)) ;
#107657=CARTESIAN_POINT('Origin',(-1.,2.95,-11.8031676725155)) ;
#107658=CARTESIAN_POINT('Origin',(1.15,2.95,-11.8031676725155)) ;
#107659=CARTESIAN_POINT('Origin',(-0.900000000000001,3.8,-10.16)) ;
#107660=CARTESIAN_POINT('Origin',(-0.900000000000002,2.1568323274845,-11.01)) ;
#107661=CARTESIAN_POINT('Origin',(-0.900000000000002,1.6,-10.16)) ;
#107662=CARTESIAN_POINT('Origin',(-0.900000000000002,1.6,-12.1221416870349)) ;
#107663=CARTESIAN_POINT('Origin',(13.9153543900904,1.4,-12.1221416870349)) ;
#107664=CARTESIAN_POINT('Origin',(8.49172374697002,1.4,-12.1221416870349)) ;
#107665=CARTESIAN_POINT('Origin',(-0.900000000000001,1.40000000000001,-12.1221416870349)) ;
#107666=CARTESIAN_POINT('Origin',(1.15,2.95,-11.8031676725155)) ;
#107667=CARTESIAN_POINT('Origin',(1.15,3.04189189189189,-11.6255279241354)) ;
#107668=CARTESIAN_POINT('Origin',(-0.900000000000002,2.1568323274845,-11.01)) ;
#107669=CARTESIAN_POINT('Origin',(-0.900000000000002,2.1568323274845,-11.01)) ;
#107670=CARTESIAN_POINT('Origin',(-0.900000000000002,2.1568323274845,-11.01)) ;
#107671=CARTESIAN_POINT('Origin',(-0.900000000000001,1.40000000000001,-12.1221416870349)) ;
#107672=CARTESIAN_POINT('Origin',(-0.900000000000002,1.55483870967742,-11.9955519007746)) ;
#107673=CARTESIAN_POINT('Origin',(1.15,3.8,-10.16)) ;
#107674=CARTESIAN_POINT('Origin',(1.15,2.33447207586456,-10.9181081081081)) ;
#107675=CARTESIAN_POINT('Origin',(-1.,2.1568323274845,-11.01)) ;
#107676=CARTESIAN_POINT('Origin',(1.15,2.1568323274845,-11.01)) ;
#107677=CARTESIAN_POINT('Origin',(-0.900000000000001,3.8,-11.01)) ;
#107678=CARTESIAN_POINT('Origin',(-0.900000000000002,1.02736587339765,-11.01)) ;
#107679=CARTESIAN_POINT('Origin',(-0.900000000000001,3.8,-10.16)) ;
#107680=CARTESIAN_POINT('Origin',(-0.900000000000002,1.02736587339765,-11.01)) ;
#107681=CARTESIAN_POINT('Origin',(13.9153543900904,1.4,-8.19785831296513)) ;
#107682=CARTESIAN_POINT('Origin',(8.49172374697002,1.4,-8.19785831296513)) ;
#107683=CARTESIAN_POINT('Origin',(-0.900000000000001,1.40000000000001,-8.19785831296513)) ;
#107684=CARTESIAN_POINT('Origin',(-0.900000000000002,1.6,-10.16)) ;
#107685=CARTESIAN_POINT('Origin',(-0.900000000000002,1.6,-8.19785831296513)) ;
#107686=CARTESIAN_POINT('Origin',(-0.900000000000002,2.95,-10.16)) ;
#107687=CARTESIAN_POINT('Origin',(-0.900000000000002,2.95,-8.5168323274845)) ;
#107688=CARTESIAN_POINT('Origin',(1.15,2.1568323274845,-11.01)) ;
#107689=CARTESIAN_POINT('Origin',(1.15,2.1568323274845,-10.81)) ;
#107690=CARTESIAN_POINT('Origin',(-0.900000000000002,1.02736587339765,-11.01)) ;
#107691=CARTESIAN_POINT('Origin',(-0.900000000000001,1.40000000000001,-8.19785831296513)) ;
#107692=CARTESIAN_POINT('Origin',(-0.900000000000002,1.55483870967743,-8.32444809922545)) ;
#107693=CARTESIAN_POINT('Origin',(-0.900000000000002,2.95,-8.5168323274845)) ;
#107694=CARTESIAN_POINT('Origin',(-0.900000000000002,2.95,-8.5168323274845)) ;
#107695=CARTESIAN_POINT('Origin',(-0.900000000000001,2.95,-8.5168323274845)) ;
#107696=CARTESIAN_POINT('Origin',(1.15,2.21886116991581,-10.81)) ;
#107697=CARTESIAN_POINT('Ctrl Pts',(1.15,1.02736587339765,-10.91)) ;
#107698=CARTESIAN_POINT('Ctrl Pts',(1.1608920328805,1.02736587339765,-10.91)) ;
#107699=CARTESIAN_POINT('Ctrl Pts',(1.17195716626105,1.02622125393927,-10.908143843926)) ;
#107700=CARTESIAN_POINT('Ctrl Pts',(1.1820844490224,1.02414637334385,-10.9047131887908)) ;
#107701=CARTESIAN_POINT('Ctrl Pts',(1.19245005921088,1.02202266415684,-10.9012017993431)) ;
#107702=CARTESIAN_POINT('Ctrl Pts',(1.20216743701154,1.01888103823701,-10.8959601980703)) ;
#107703=CARTESIAN_POINT('Ctrl Pts',(1.21053792402812,1.01518120925307,-10.8895937168021)) ;
#107704=CARTESIAN_POINT('Ctrl Pts',(1.219343173684,1.01128921135341,-10.8828965608439)) ;
#107705=CARTESIAN_POINT('Ctrl Pts',(1.22692289939014,1.00668521903338,-10.8747851615315)) ;
#107706=CARTESIAN_POINT('Ctrl Pts',(1.23290049538659,1.00186003905466,-10.8659241259624)) ;
#107707=CARTESIAN_POINT('Ctrl Pts',(1.23922345568944,0.9967560772818,-10.85655113117)) ;
#107708=CARTESIAN_POINT('Ctrl Pts',(1.24392209779927,0.991279542094837,
-10.8461045599897)) ;
#107709=CARTESIAN_POINT('Ctrl Pts',(1.24674870216524,0.985895902333124,
-10.8352920665297)) ;
#107710=CARTESIAN_POINT('Ctrl Pts',(1.24889292215336,0.981811953364218,
-10.8270898699727)) ;
#107711=CARTESIAN_POINT('Ctrl Pts',(1.25,0.977715885027402,-10.8185491686292)) ;
#107712=CARTESIAN_POINT('Ctrl Pts',(1.25,0.973783447787483,-10.81)) ;
#107713=CARTESIAN_POINT('Origin',(-0.900000000000001,3.8,-10.16)) ;
#107714=CARTESIAN_POINT('Origin',(-0.900000000000002,1.02736587339765,-9.31)) ;
#107715=CARTESIAN_POINT('Origin',(-0.900000000000001,3.8,-9.31)) ;
#107716=CARTESIAN_POINT('Origin',(-0.900000000000002,2.1568323274845,-9.31)) ;
#107717=CARTESIAN_POINT('Origin',(-0.900000000000002,1.02736587339765,-9.31)) ;
#107718=CARTESIAN_POINT('Origin',(-0.900000000000001,3.8,-10.16)) ;
#107719=CARTESIAN_POINT('Origin',(-0.900000000000002,2.1568323274845,-9.31)) ;
#107720=CARTESIAN_POINT('Origin',(-1.,2.95,-8.5168323274845)) ;
#107721=CARTESIAN_POINT('Origin',(1.15,2.95,-8.5168323274845)) ;
#107722=CARTESIAN_POINT('Origin',(1.15,3.15,-7.61)) ;
#107723=CARTESIAN_POINT('Origin',(1.15,3.15,-8.5168323274845)) ;
#107724=CARTESIAN_POINT('Ctrl Pts',(1.11028558574894,0.930383836951429,
-11.034994283658)) ;
#107725=CARTESIAN_POINT('Ctrl Pts',(1.14039000477529,0.892136466137752,
-10.909969718594)) ;
#107726=CARTESIAN_POINT('Ctrl Pts',(1.13015013463564,1.02610337426265,-10.9078511248828)) ;
#107727=CARTESIAN_POINT('Ctrl Pts',(1.1763969065272,0.935225109827845,-11.0501257399473)) ;
#107728=CARTESIAN_POINT('Ctrl Pts',(1.15491086542921,0.891146666106505,
-10.9092760504016)) ;
#107729=CARTESIAN_POINT('Ctrl Pts',(1.16319405445819,1.03078047702075,-10.9151648742452)) ;
#107730=CARTESIAN_POINT('Ctrl Pts',(1.24701363206619,0.927145283841869,
-11.0255522038252)) ;
#107731=CARTESIAN_POINT('Ctrl Pts',(1.1775998083145,0.893467326853714,-10.9126373120313)) ;
#107732=CARTESIAN_POINT('Ctrl Pts',(1.19848758201044,1.022974674531,-10.903287122555)) ;
#107733=CARTESIAN_POINT('Ctrl Pts',(1.33816236560078,0.900022463714239,
-10.929808850615)) ;
#107734=CARTESIAN_POINT('Ctrl Pts',(1.22862786282603,0.888037626603791,
-10.8831539643241)) ;
#107735=CARTESIAN_POINT('Ctrl Pts',(1.244032885045,0.996768276947704,-10.8570266594133)) ;
#107736=CARTESIAN_POINT('Ctrl Pts',(1.35959492575617,0.881455895025387,
-10.8585323412291)) ;
#107737=CARTESIAN_POINT('Ctrl Pts',(1.2532051975069,0.880428099081518,-10.8510649378273)) ;
#107738=CARTESIAN_POINT('Ctrl Pts',(1.25473603279823,0.978811277328879,
-10.8225574871508)) ;
#107739=CARTESIAN_POINT('Ctrl Pts',(1.34615355831638,0.867571605181199,
-10.7927925825334)) ;
#107740=CARTESIAN_POINT('Ctrl Pts',(1.25176090202798,0.87095013062452,-10.8094490170578)) ;
#107741=CARTESIAN_POINT('Ctrl Pts',(1.24801589497572,0.965423101361769,
-10.7908695481641)) ;
#107742=CARTESIAN_POINT('Origin',(1.35,0.973783447787483,-10.81)) ;
#107743=CARTESIAN_POINT('Origin',(-0.900000000000002,1.02736587339765,-9.31)) ;
#107744=CARTESIAN_POINT('',(-0.957735026918965,0.969630846478687,-9.36773502691896)) ;
#107745=CARTESIAN_POINT('Origin',(-0.900000000000002,1.02736587339765,-9.31)) ;
#107746=CARTESIAN_POINT('Origin',(-0.900000000000002,2.1568323274845,-9.31)) ;
#107747=CARTESIAN_POINT('Origin',(-0.900000000000002,2.1568323274845,-9.31)) ;
#107748=CARTESIAN_POINT('Origin',(1.15,2.95,-8.5168323274845)) ;
#107749=CARTESIAN_POINT('Origin',(1.15,3.04189189189189,-8.69447207586456)) ;
#107750=CARTESIAN_POINT('Origin',(1.35,3.8,-10.16)) ;
#107751=CARTESIAN_POINT('Origin',(1.35,0.973783447787484,-9.51)) ;
#107752=CARTESIAN_POINT('Origin',(-1.,2.1568323274845,-9.31)) ;
#107753=CARTESIAN_POINT('Origin',(1.15,2.1568323274845,-9.31)) ;
#107754=CARTESIAN_POINT('Origin',(1.15,3.8,-10.16)) ;
#107755=CARTESIAN_POINT('Origin',(1.15,2.33447207586456,-9.40189189189189)) ;
#107756=CARTESIAN_POINT('Ctrl Pts',(1.34754079198594,0.86915957129316,-9.51974853478551)) ;
#107757=CARTESIAN_POINT('Ctrl Pts',(1.25183398383324,0.871999770424347,
-9.5059986517603)) ;
#107758=CARTESIAN_POINT('Ctrl Pts',(1.24871534599026,0.966951450593918,
-9.52553571307356)) ;
#107759=CARTESIAN_POINT('Ctrl Pts',(1.3578897130187,0.882932151572339,-9.45577742826812)) ;
#107760=CARTESIAN_POINT('Ctrl Pts',(1.25138796519085,0.881019151005395,
-9.46648728142377)) ;
#107761=CARTESIAN_POINT('Ctrl Pts',(1.25389076424432,0.980237216252331,
-9.49468863425941)) ;
#107762=CARTESIAN_POINT('Ctrl Pts',(1.33642796493171,0.90055164307479,-9.3883167189688)) ;
#107763=CARTESIAN_POINT('Ctrl Pts',(1.22773025960893,0.888154519889375,
-9.43630235415234)) ;
#107764=CARTESIAN_POINT('Ctrl Pts',(1.24317203399028,0.99727835245108,-9.46206445828307)) ;
#107765=CARTESIAN_POINT('Ctrl Pts',(1.24851212064762,0.926675670999743,
-9.29611185418657)) ;
#107766=CARTESIAN_POINT('Ctrl Pts',(1.17855408504652,0.893378082604349,
-9.40793584540021)) ;
#107767=CARTESIAN_POINT('Ctrl Pts',(1.19923947710882,1.02252144543593,-9.41751118406066)) ;
#107768=CARTESIAN_POINT('Ctrl Pts',(1.18212686068543,0.93456788869825,-9.27189225990077)) ;
#107769=CARTESIAN_POINT('Ctrl Pts',(1.1569094747617,0.891342319659306,-9.41050130223919)) ;
#107770=CARTESIAN_POINT('Ctrl Pts',(1.1660589236879,1.03014681530415,-9.40580412352038)) ;
#107771=CARTESIAN_POINT('Ctrl Pts',(1.11776263740947,0.930888708579174,
-9.28342358191601)) ;
#107772=CARTESIAN_POINT('Ctrl Pts',(1.14197710563592,0.892059806626676,
-9.41008229965539)) ;
#107773=CARTESIAN_POINT('Ctrl Pts',(1.13388624958144,1.02659206201255,-9.41137785610126)) ;
#107774=CARTESIAN_POINT('Ctrl Pts',(1.15,1.02736587339764,-9.41)) ;
#107775=CARTESIAN_POINT('Ctrl Pts',(1.15623005440502,1.02736587339759,-9.40999999999987)) ;
#107776=CARTESIAN_POINT('Ctrl Pts',(1.16249579431471,1.02700282517053,-9.41059086606898)) ;
#107777=CARTESIAN_POINT('Ctrl Pts',(1.16857840195431,1.02630083270769,-9.41174093944667)) ;
#107778=CARTESIAN_POINT('Ctrl Pts',(1.1798885498395,1.02499553092934,-9.41387941372467)) ;
#107779=CARTESIAN_POINT('Ctrl Pts',(1.19084787809767,1.02245621903271,-9.41805069661522)) ;
#107780=CARTESIAN_POINT('Ctrl Pts',(1.20043335385463,1.01914369852331,-9.4236491064379)) ;
#107781=CARTESIAN_POINT('Ctrl Pts',(1.21063893018497,1.01561688548223,-9.42960968682249)) ;
#107782=CARTESIAN_POINT('Ctrl Pts',(1.21965078109605,1.01112191387731,-9.43735485110186)) ;
#107783=CARTESIAN_POINT('Ctrl Pts',(1.226898722009,1.00626683908294,-9.44607358485429)) ;
#107784=CARTESIAN_POINT('Ctrl Pts',(1.23435386869391,1.0012729663137,-9.45504157173658)) ;
#107785=CARTESIAN_POINT('Ctrl Pts',(1.24017476602864,0.995763540409855,
-9.46528702640693)) ;
#107786=CARTESIAN_POINT('Ctrl Pts',(1.24405759382605,0.990267693778535,
-9.47604165723046)) ;
#107787=CARTESIAN_POINT('Ctrl Pts',(1.24795610732226,0.9847496452368,-9.48683973419908)) ;
#107788=CARTESIAN_POINT('Ctrl Pts',(1.25,0.97910634898267,-9.49842794502798)) ;
#107789=CARTESIAN_POINT('Ctrl Pts',(1.25,0.973783447787483,-9.51)) ;
#107790=CARTESIAN_POINT('Origin',(1.15,2.1568323274845,-9.31)) ;
#107791=CARTESIAN_POINT('Origin',(1.15,2.1568323274845,-9.51)) ;
#107792=CARTESIAN_POINT('Origin',(1.15,2.21886116991581,-9.51)) ;
#107793=CARTESIAN_POINT('Origin',(1.5,2.3,-10.56)) ;
#107794=CARTESIAN_POINT('Ctrl Pts',(0.549999999999999,4.04473197180486,
-10.61)) ;
#107795=CARTESIAN_POINT('Ctrl Pts',(0.549999999999999,4.04340510574359,
-10.6120183916746)) ;
#107796=CARTESIAN_POINT('Ctrl Pts',(0.54993891248805,4.04197482121863,-10.6139799093559)) ;
#107797=CARTESIAN_POINT('Ctrl Pts',(0.549362579613717,4.03414945156058,
-10.623763201697)) ;
#107798=CARTESIAN_POINT('Ctrl Pts',(0.548040652125095,4.02633974827553,
-10.6305458262272)) ;
#107799=CARTESIAN_POINT('Ctrl Pts',(0.544205267183616,4.00519499286844,
-10.6446839427889)) ;
#107800=CARTESIAN_POINT('Ctrl Pts',(0.541221332378489,3.99011995637975,
-10.6512251154482)) ;
#107801=CARTESIAN_POINT('Ctrl Pts',(0.537814556431586,3.96385893187673,
-10.65793059224)) ;
#107802=CARTESIAN_POINT('Ctrl Pts',(0.536602540378443,3.9513239070287,-10.66)) ;
#107803=CARTESIAN_POINT('Ctrl Pts',(0.536602540378443,3.93764017256378,
-10.66)) ;
#107804=CARTESIAN_POINT('Origin',(-0.4,2.3,-10.56)) ;
#107805=CARTESIAN_POINT('Origin',(-0.4,-3.4,-10.56)) ;
#107806=CARTESIAN_POINT('Origin',(-0.4,-3.36847777691809,-10.56)) ;
#107807=CARTESIAN_POINT('Origin',(1.5,2.3,-10.56)) ;
#107808=CARTESIAN_POINT('Ctrl Pts',(0.536602540378442,2.83090991212703,
-10.66)) ;
#107809=CARTESIAN_POINT('Ctrl Pts',(0.536602540378442,2.80627146475495,
-10.66)) ;
#107810=CARTESIAN_POINT('Ctrl Pts',(0.538106903229178,2.77742679387655,
-10.6579527908126)) ;
#107811=CARTESIAN_POINT('Ctrl Pts',(0.545186976568879,2.71156844363324,
-10.64208398098)) ;
#107812=CARTESIAN_POINT('Ctrl Pts',(0.549999999999999,2.68282906082667,
-10.6281020558136)) ;
#107813=CARTESIAN_POINT('Ctrl Pts',(0.549999999999999,2.65280931275608,
-10.61)) ;
#107814=CARTESIAN_POINT('Origin',(0.400000000000001,2.29999999999999,-10.56)) ;
#107815=CARTESIAN_POINT('Origin',(0.0725078566451197,-4.04348900069683,
-10.0874921433549)) ;
#107816=CARTESIAN_POINT('Origin',(-0.4,-3.36847777691809,-10.56)) ;
#107817=CARTESIAN_POINT('Origin',(-0.0979344438426628,-3.8,-10.2579344438427)) ;
#107818=CARTESIAN_POINT('Origin',(1.5,2.3,-9.76)) ;
#107819=CARTESIAN_POINT('Ctrl Pts',(0.536602540378443,3.93764017256378,
-9.66)) ;
#107820=CARTESIAN_POINT('Ctrl Pts',(0.536602540378443,3.93925361219649,
-9.66)) ;
#107821=CARTESIAN_POINT('Ctrl Pts',(0.536619300889432,3.94087098263986,
-9.66002899725778)) ;
#107822=CARTESIAN_POINT('Ctrl Pts',(0.536997639747691,3.95938954612056,
-9.66068581289572)) ;
#107823=CARTESIAN_POINT('Ctrl Pts',(0.53914231517103,3.97567120869872,-9.66431206156154)) ;
#107824=CARTESIAN_POINT('Ctrl Pts',(0.544035197036615,4.00535605098064,
-9.67539939166588)) ;
#107825=CARTESIAN_POINT('Ctrl Pts',(0.546989816174385,4.01946236900589,
-9.68356994463487)) ;
#107826=CARTESIAN_POINT('Ctrl Pts',(0.549463062495682,4.03595536007394,
-9.69854738169706)) ;
#107827=CARTESIAN_POINT('Ctrl Pts',(0.550000000000879,4.04078397701433,
-9.70399442034631)) ;
#107828=CARTESIAN_POINT('Ctrl Pts',(0.549999999999999,4.04473197181449,
-9.71000000001465)) ;
#107829=CARTESIAN_POINT('Origin',(-0.4,2.3,-9.76)) ;
#107830=CARTESIAN_POINT('Origin',(0.4,2.29999999999999,-10.56)) ;
#107831=CARTESIAN_POINT('Origin',(0.4,-3.36847777691809,-10.56)) ;
#107832=CARTESIAN_POINT('Origin',(-0.0979344438426628,-3.8,-10.2579344438427)) ;
#107833=CARTESIAN_POINT('Origin',(-0.0979344438426628,-3.8,-10.2579344438427)) ;
#107834=CARTESIAN_POINT('Origin',(-0.0979344438426627,-3.8,-10.2579344438427)) ;
#107835=CARTESIAN_POINT('Origin',(-0.4,2.3,-9.76)) ;
#107836=CARTESIAN_POINT('Origin',(-0.4,-3.36847777691809,-9.76)) ;
#107837=CARTESIAN_POINT('Origin',(0.190875981738719,-3.6672263744342,-10.3508759817387)) ;
#107838=CARTESIAN_POINT('Origin',(0.400000000000001,-3.36847777691809,-10.56)) ;
#107839=CARTESIAN_POINT('Origin',(0.0979344438426626,-3.8,-10.2579344438427)) ;
#107840=CARTESIAN_POINT('Origin',(0.15,-3.8,-10.2579344438427)) ;
#107841=CARTESIAN_POINT('Origin',(0.0979344438426627,-3.8,-10.2579344438427)) ;
#107842=CARTESIAN_POINT('Origin',(-0.0979344438426628,-3.8,-9.66)) ;
#107843=CARTESIAN_POINT('Origin',(-0.0979344438426628,-3.8,-10.0620655561573)) ;
#107844=CARTESIAN_POINT('Origin',(-0.174966890829628,-3.68995364716148,
-9.98503310917037)) ;
#107845=CARTESIAN_POINT('Origin',(-0.400000000000001,-3.36847777691809,
-9.76)) ;
#107846=CARTESIAN_POINT('Origin',(-0.0979344438426627,-3.8,-10.0620655561573)) ;
#107847=CARTESIAN_POINT('Origin',(0.0979344438426627,-3.8,-10.2579344438427)) ;
#107848=CARTESIAN_POINT('Origin',(0.0979344438426628,-3.8,-10.2579344438427)) ;
#107849=CARTESIAN_POINT('Origin',(-0.0979344438426628,-3.8,-10.0620655561573)) ;
#107850=CARTESIAN_POINT('Origin',(-0.0979344438426628,-3.8,-10.0620655561573)) ;
#107851=CARTESIAN_POINT('Origin',(0.0979344438426627,-3.8,-9.66)) ;
#107852=CARTESIAN_POINT('Origin',(0.0979344438426627,-3.8,-10.0620655561573)) ;
#107853=CARTESIAN_POINT('Origin',(-1.11032778078669,-3.8,-10.0620655561573)) ;
#107854=CARTESIAN_POINT('Origin',(0.0979344438426626,-3.8,-10.0620655561573)) ;
#107855=CARTESIAN_POINT('Origin',(0.0979344438426627,-3.8,-10.0620655561573)) ;
#107856=CARTESIAN_POINT('Origin',(0.0979344438426627,-3.8,-10.0620655561573)) ;
#107857=CARTESIAN_POINT('Origin',(0.438350729213467,-3.31369102089885,-9.72164927078653)) ;
#107858=CARTESIAN_POINT('Origin',(0.399999999999999,-3.36847777691809,-9.76)) ;
#107859=CARTESIAN_POINT('Origin',(0.4,2.3,-9.76)) ;
#107860=CARTESIAN_POINT('Origin',(0.4,-3.36847777691809,-9.76)) ;
#107861=CARTESIAN_POINT('Origin',(0.4,2.29999999999999,-9.76)) ;
#107862=CARTESIAN_POINT('Origin',(1.5,2.3,-9.76)) ;
#107863=CARTESIAN_POINT('Ctrl Pts',(0.55,2.65280931275594,-9.71000000000009)) ;
#107864=CARTESIAN_POINT('Ctrl Pts',(0.550000000000012,2.67648433237897,
-9.69572384666271)) ;
#107865=CARTESIAN_POINT('Ctrl Pts',(0.54690886425279,2.69988533923261,-9.68352570084763)) ;
#107866=CARTESIAN_POINT('Ctrl Pts',(0.539540151921448,2.76165254733705,
-9.66409159819012)) ;
#107867=CARTESIAN_POINT('Ctrl Pts',(0.536602540378443,2.79600904778111,
-9.66)) ;
#107868=CARTESIAN_POINT('Ctrl Pts',(0.536602540378443,2.83090991212703,
-9.66)) ;
#107869=CARTESIAN_POINT('Origin',(8.,3.4,-10.56)) ;
#107870=CARTESIAN_POINT('Origin',(7.96847777691809,3.4,-10.56)) ;
#107871=CARTESIAN_POINT('Origin',(1.5,4.2,-10.56)) ;
#107872=CARTESIAN_POINT('Origin',(7.96847777691809,4.2,-10.56)) ;
#107873=CARTESIAN_POINT('Origin',(8.64348900069683,3.87250785664512,-10.0874921433549)) ;
#107874=CARTESIAN_POINT('Origin',(7.96847777691809,3.4,-10.56)) ;
#107875=CARTESIAN_POINT('Origin',(8.4,3.70206555615734,-10.2579344438427)) ;
#107876=CARTESIAN_POINT('Origin',(8.26722637443421,3.99087598173872,-10.3508759817387)) ;
#107877=CARTESIAN_POINT('Origin',(7.96847777691809,4.2,-10.56)) ;
#107878=CARTESIAN_POINT('Origin',(8.4,3.89793444384266,-10.2579344438427)) ;
#107879=CARTESIAN_POINT('Origin',(8.4,3.95,-10.2579344438427)) ;
#107880=CARTESIAN_POINT('Origin',(8.4,3.70206555615734,-10.2579344438427)) ;
#107881=CARTESIAN_POINT('Origin',(8.4,3.89793444384266,-10.2579344438427)) ;
#107882=CARTESIAN_POINT('Origin',(8.4,3.70206555615734,-10.2579344438427)) ;
#107883=CARTESIAN_POINT('Origin',(8.4,3.70206555615734,-10.2579344438427)) ;
#107884=CARTESIAN_POINT('Origin',(1.5,3.4,-9.76)) ;
#107885=CARTESIAN_POINT('Origin',(7.96847777691809,3.4,-9.76)) ;
#107886=CARTESIAN_POINT('Origin',(1.5,4.2,-9.76)) ;
#107887=CARTESIAN_POINT('Origin',(7.96847777691809,4.2,-9.76)) ;
#107888=CARTESIAN_POINT('Origin',(8.4,3.89793444384266,-10.2579344438427)) ;
#107889=CARTESIAN_POINT('Origin',(8.4,3.89793444384266,-10.2579344438427)) ;
#107890=CARTESIAN_POINT('Origin',(8.4,3.70206555615734,-9.66)) ;
#107891=CARTESIAN_POINT('Origin',(8.4,3.70206555615734,-10.0620655561573)) ;
#107892=CARTESIAN_POINT('Origin',(8.28995364716148,3.62503310917037,-9.98503310917037)) ;
#107893=CARTESIAN_POINT('Origin',(7.96847777691809,3.4,-9.76)) ;
#107894=CARTESIAN_POINT('Origin',(8.4,3.70206555615734,-10.0620655561573)) ;
#107895=CARTESIAN_POINT('Origin',(7.91369102089885,4.23835072921347,-9.72164927078653)) ;
#107896=CARTESIAN_POINT('Origin',(7.96847777691809,4.2,-9.76)) ;
#107897=CARTESIAN_POINT('Origin',(8.4,3.89793444384266,-10.0620655561573)) ;
#107898=CARTESIAN_POINT('Origin',(8.4,3.89793444384266,-9.66)) ;
#107899=CARTESIAN_POINT('Origin',(8.4,3.89793444384266,-10.0620655561573)) ;
#107900=CARTESIAN_POINT('Origin',(8.4,3.70206555615734,-10.0620655561573)) ;
#107901=CARTESIAN_POINT('Origin',(8.4,3.70206555615734,-10.0620655561573)) ;
#107902=CARTESIAN_POINT('Origin',(8.4,3.89793444384266,-10.0620655561573)) ;
#107903=CARTESIAN_POINT('Origin',(8.4,3.89793444384266,-10.0620655561573)) ;
#107904=CARTESIAN_POINT('Origin',(8.4,2.68967221921331,-10.0620655561573)) ;
#107905=CARTESIAN_POINT('Origin',(9.9,6.8847127088383,-12.7)) ;
#107906=CARTESIAN_POINT('Origin',(9.9,6.8847127088383,-11.1197127088383)) ;
#107907=CARTESIAN_POINT('Origin',(8.77035388141948,6.69643835574155,-10.9314383557415)) ;
#107908=CARTESIAN_POINT('Ctrl Pts',(8.58356010126947,6.66256607592813,-10.7989266835449)) ;
#107909=CARTESIAN_POINT('Ctrl Pts',(8.58266714977879,6.65676189123867,-10.7987778582964)) ;
#107910=CARTESIAN_POINT('Ctrl Pts',(8.58182526931896,6.6507714222091,-10.799114171474)) ;
#107911=CARTESIAN_POINT('Ctrl Pts',(8.58032528754337,6.63886560514819,-10.8009127350996)) ;
#107912=CARTESIAN_POINT('Ctrl Pts',(8.57966270906111,6.6329537021218,-10.8023448243328)) ;
#107913=CARTESIAN_POINT('Ctrl Pts',(8.57906641006222,6.62681909302514,-10.8044771744937)) ;
#107914=CARTESIAN_POINT('Ctrl Pts',(8.5790337515733,6.62647998752502,-10.8045971697284)) ;
#107915=CARTESIAN_POINT('Ctrl Pts',(8.57846569624187,6.62052582174809,-10.8067417316811)) ;
#107916=CARTESIAN_POINT('Ctrl Pts',(8.57802501793955,6.61503168015118,-10.8093142858563)) ;
#107917=CARTESIAN_POINT('Ctrl Pts',(8.57766199200563,6.60925146760179,-10.8127462133241)) ;
#107918=CARTESIAN_POINT('Ctrl Pts',(8.57762821177171,6.60869602779036,-10.813083835165)) ;
#107919=CARTESIAN_POINT('Ctrl Pts',(8.57728522755447,6.60286036001416,-10.8167147989574)) ;
#107920=CARTESIAN_POINT('Ctrl Pts',(8.57709550103272,6.59788070192258,-10.8205482210568)) ;
#107921=CARTESIAN_POINT('Ctrl Pts',(8.57703980289281,6.59299711069327,-10.8251723373554)) ;
#107922=CARTESIAN_POINT('Ctrl Pts',(8.57703670271024,6.59265952430004,-10.8254968925423)) ;
#107923=CARTESIAN_POINT('Ctrl Pts',(8.57701334129172,6.58927432516123,-10.8288013815953)) ;
#107924=CARTESIAN_POINT('Ctrl Pts',(8.57705699426438,6.58642971201546,-10.8319917444087)) ;
#107925=CARTESIAN_POINT('Ctrl Pts',(8.57735031225524,6.57961409340218,-10.8407954417554)) ;
#107926=CARTESIAN_POINT('Ctrl Pts',(8.5777085651344,6.5760438318291,-10.8466682455398)) ;
#107927=CARTESIAN_POINT('Ctrl Pts',(8.57865704971093,6.57055741297637,-10.8583322193387)) ;
#107928=CARTESIAN_POINT('Ctrl Pts',(8.57922107378969,6.56851476050451,-10.8640736349075)) ;
#107929=CARTESIAN_POINT('Ctrl Pts',(8.57993695782543,6.56687610193756,-10.8704559348161)) ;
#107930=CARTESIAN_POINT('Ctrl Pts',(8.58000419042984,6.56673001682056,-10.8710478351838)) ;
#107931=CARTESIAN_POINT('Ctrl Pts',(8.58074399738019,6.56520526212525,-10.8774812517351)) ;
#107932=CARTESIAN_POINT('Ctrl Pts',(8.58149993293344,6.5643813478578,-10.8833541800931)) ;
#107933=CARTESIAN_POINT('Ctrl Pts',(8.58236768178473,6.56403389662203,-10.8894987578229)) ;
#107934=CARTESIAN_POINT('Ctrl Pts',(8.58242358604546,6.56401394107886,-10.8898921736314)) ;
#107935=CARTESIAN_POINT('Ctrl Pts',(8.58283067264383,6.56388592662945,-10.8927394234264)) ;
#107936=CARTESIAN_POINT('Ctrl Pts',(8.58319156240649,6.56386525642004,-10.8951699505828)) ;
#107937=CARTESIAN_POINT('Ctrl Pts',(8.58356019967707,6.56392669994633,-10.8975662650647)) ;
#107938=CARTESIAN_POINT('Origin',(9.9,6.8847127088383,-11.1197127088383)) ;
#107939=CARTESIAN_POINT('Origin',(9.9,6.8847127088383,-11.1197127088383)) ;
#107940=CARTESIAN_POINT('Origin',(9.9,6.8847127088383,-11.1197127088383)) ;
#107941=CARTESIAN_POINT('Origin',(9.9,7.72792407799439,-12.7)) ;
#107942=CARTESIAN_POINT('Origin',(9.9,7.72792407799439,-11.1197127088383)) ;
#107943=CARTESIAN_POINT('Origin',(9.90000000000001,4.35421736843756,-11.1197127088383)) ;
#107944=CARTESIAN_POINT('Origin',(9.9,7.72792407799439,-11.1197127088383)) ;
#107945=CARTESIAN_POINT('Origin',(9.9,7.72792407799439,-11.1197127088383)) ;
#107946=CARTESIAN_POINT('Origin',(9.9,7.72792407799439,-11.1197127088383)) ;
#107947=CARTESIAN_POINT('Origin',(10.9628342502842,7.37364599456632,-11.2968517505523)) ;
#107948=CARTESIAN_POINT('Ctrl Pts',(8.56837732530586,8.2772075582313,-10.8925052537977)) ;
#107949=CARTESIAN_POINT('Ctrl Pts',(8.56753565030797,8.2774881236726,-10.8866129921974)) ;
#107950=CARTESIAN_POINT('Ctrl Pts',(8.56682045541689,8.2772118066791,-10.8805412944396)) ;
#107951=CARTESIAN_POINT('Ctrl Pts',(8.56575413148015,8.27538624160206,-10.8687284721175)) ;
#107952=CARTESIAN_POINT('Ctrl Pts',(8.56538426077853,8.27391165896469,-10.8629905624275)) ;
#107953=CARTESIAN_POINT('Ctrl Pts',(8.56517777855933,8.27166501362502,-10.857014775447)) ;
#107954=CARTESIAN_POINT('Ctrl Pts',(8.56516523451684,8.27151619608592,-10.8566276382837)) ;
#107955=CARTESIAN_POINT('Ctrl Pts',(8.56497390811217,8.26902793125449,-10.8502953359912)) ;
#107956=CARTESIAN_POINT('Ctrl Pts',(8.56499903025538,8.26597630129449,-10.8445357784659)) ;
#107957=CARTESIAN_POINT('Ctrl Pts',(8.56538588200261,8.26046191593053,-10.8365906723681)) ;
#107958=CARTESIAN_POINT('Ctrl Pts',(8.56556309332511,8.25853771611456,-10.8341212364558)) ;
#107959=CARTESIAN_POINT('Ctrl Pts',(8.56628156514553,8.25214511987157,-10.8268017566891)) ;
#107960=CARTESIAN_POINT('Ctrl Pts',(8.56700742874797,8.24720216256268,-10.822305445231)) ;
#107961=CARTESIAN_POINT('Ctrl Pts',(8.56880713798128,8.23661566152168,-10.81462449488)) ;
#107962=CARTESIAN_POINT('Ctrl Pts',(8.5698603939132,8.23102391526974,-10.8113848807256)) ;
#107963=CARTESIAN_POINT('Ctrl Pts',(8.57116255171754,8.22459552194135,-10.808446774527)) ;
#107964=CARTESIAN_POINT('Ctrl Pts',(8.5712749581022,8.22404408343789,-10.8082006607902)) ;
#107965=CARTESIAN_POINT('Ctrl Pts',(8.57260511146314,8.2175590131258,-10.8053749153055)) ;
#107966=CARTESIAN_POINT('Ctrl Pts',(8.57395629672842,8.2113575973091,-10.8033463864276)) ;
#107967=CARTESIAN_POINT('Ctrl Pts',(8.57552311082418,8.20452945286286,-10.8017495443173)) ;
#107968=CARTESIAN_POINT('Ctrl Pts',(8.57564505123014,8.20400026307087,-10.801629826956)) ;
#107969=CARTESIAN_POINT('Ctrl Pts',(8.57731301559526,8.19679193622634,-10.800053462537)) ;
#107970=CARTESIAN_POINT('Ctrl Pts',(8.57896065127871,8.19002168485358,-10.799210969344)) ;
#107971=CARTESIAN_POINT('Ctrl Pts',(8.58161366784368,8.17959769015476,-10.7987553172771)) ;
#107972=CARTESIAN_POINT('Ctrl Pts',(8.5825836286427,8.17587911616512,-10.7987639381071)) ;
#107973=CARTESIAN_POINT('Ctrl Pts',(8.58356010126947,8.17221734381475,-10.7989266835449)) ;
#107974=CARTESIAN_POINT('Origin',(7.96824861826159,6.56275414521524,-9.52224585478477)) ;
#107975=CARTESIAN_POINT('Origin',(8.59688370202626,6.66156024040307,-9.43124347526404)) ;
#107976=CARTESIAN_POINT('Origin',(9.9,6.8847127088383,-9.2002872911617)) ;
#107977=CARTESIAN_POINT('Origin',(9.9,6.8847127088383,-12.7)) ;
#107978=CARTESIAN_POINT('Origin',(9.9,6.8847127088383,-9.2002872911617)) ;
#107979=CARTESIAN_POINT('Origin',(9.9,6.8847127088383,-9.2002872911617)) ;
#107980=CARTESIAN_POINT('Origin',(9.9,6.8847127088383,-9.2002872911617)) ;
#107981=CARTESIAN_POINT('Origin',(9.9,6.8,-9.2002872911617)) ;
#107982=CARTESIAN_POINT('Origin',(9.9,7.72792407799439,-9.2002872911617)) ;
#107983=CARTESIAN_POINT('Origin',(9.9,7.72792407799439,-12.7)) ;
#107984=CARTESIAN_POINT('Origin',(9.9,7.72792407799439,-9.2002872911617)) ;
#107985=CARTESIAN_POINT('Origin',(9.9,7.72792407799439,-9.2002872911617)) ;
#107986=CARTESIAN_POINT('Origin',(9.9,7.72792407799439,-9.2002872911617)) ;
#107987=CARTESIAN_POINT('Origin',(9.60917571369883,7.82486550676144,-9.24875800554523)) ;
#107988=CARTESIAN_POINT('Origin',(8.59099001846081,8.18966234086565,-9.42516097389812)) ;
#107989=CARTESIAN_POINT('Origin',(0.45,4.4,-10.16)) ;
#107990=CARTESIAN_POINT('Origin',(0.45,4.4,-10.61)) ;
#107991=CARTESIAN_POINT('Origin',(0.45,4.4,-9.71)) ;
#107992=CARTESIAN_POINT('Origin',(-1.9,7.55,-12.7)) ;
#107993=CARTESIAN_POINT('Origin',(6.9,7.75,-12.7)) ;
#107994=CARTESIAN_POINT('Origin',(7.1,8.2,-12.7)) ;
#107995=CARTESIAN_POINT('Origin',(9.9,0.1,-12.7)) ;
#107996=CARTESIAN_POINT('Origin',(9.9,1.16528729116168,-12.7)) ;
#107997=CARTESIAN_POINT('Origin',(9.9,1.16528729116168,-12.2041618801782)) ;
#107998=CARTESIAN_POINT('Origin',(9.9,3.8,-10.16)) ;
#107999=CARTESIAN_POINT('Origin',(9.9,1.16528729116168,-8.1158381198218)) ;
#108000=CARTESIAN_POINT('Origin',(9.9,1.16528729116168,-12.2041618801782)) ;
#108001=CARTESIAN_POINT('Origin',(9.9,1.16528729116168,-12.7)) ;
#108002=CARTESIAN_POINT('Origin',(9.9,1.16528729116168,-8.1158381198218)) ;
#108003=CARTESIAN_POINT('Ctrl Pts',(0.55,0.3,-10.61)) ;
#108004=CARTESIAN_POINT('Ctrl Pts',(0.55,0.3,-10.71)) ;
#108005=CARTESIAN_POINT('Ctrl Pts',(0.45,0.3,-10.71)) ;
#108006=CARTESIAN_POINT('Ctrl Pts',(0.55,0.28690770353672,-10.6100000008183)) ;
#108007=CARTESIAN_POINT('Ctrl Pts',(0.549992696056779,0.300543498480462,
-10.7099926960868)) ;
#108008=CARTESIAN_POINT('Ctrl Pts',(0.450000000818259,0.286907703536723,
-10.71)) ;
#108009=CARTESIAN_POINT('Ctrl Pts',(0.552602750539093,0.273825167611082,
-10.6152055010782)) ;
#108010=CARTESIAN_POINT('Ctrl Pts',(0.546703256435901,0.299059401315789,
-10.7067032564359)) ;
#108011=CARTESIAN_POINT('Ctrl Pts',(0.455205501078185,0.273825167611078,
-10.7126027505391)) ;
#108012=CARTESIAN_POINT('Ctrl Pts',(0.56262134295865,0.249638145915901,
-10.6352426859173)) ;
#108013=CARTESIAN_POINT('Ctrl Pts',(0.544986924117067,0.282072776439536,
-10.7049869241171)) ;
#108014=CARTESIAN_POINT('Ctrl Pts',(0.4752426859173,0.249638145915905,-10.7226213429587)) ;
#108015=CARTESIAN_POINT('Ctrl Pts',(0.570033341471288,0.238545302291403,
-10.6500666829426)) ;
#108016=CARTESIAN_POINT('Ctrl Pts',(0.547116196858403,0.267914459835259,
-10.7071161968584)) ;
#108017=CARTESIAN_POINT('Ctrl Pts',(0.490066682942577,0.238545302291388,
-10.7300333414713)) ;
#108018=CARTESIAN_POINT('Ctrl Pts',(0.597801282701459,0.210777361061231,
-10.7056025654029)) ;
#108019=CARTESIAN_POINT('Ctrl Pts',(0.570853448890168,0.22637471385926,
-10.7308534488902)) ;
#108020=CARTESIAN_POINT('Ctrl Pts',(0.545602565402917,0.210777361061261,
-10.7578012827014)) ;
#108021=CARTESIAN_POINT('Ctrl Pts',(0.62374656717361,0.2,-10.7574931343473)) ;
#108022=CARTESIAN_POINT('Ctrl Pts',(0.610458667315072,0.2,-10.7704586673159)) ;
#108023=CARTESIAN_POINT('Ctrl Pts',(0.59749313434724,0.2,-10.7837465671738)) ;
#108024=CARTESIAN_POINT('Ctrl Pts',(0.65,0.2,-10.81)) ;
#108025=CARTESIAN_POINT('Ctrl Pts',(0.65,0.2,-10.81)) ;
#108026=CARTESIAN_POINT('Ctrl Pts',(0.65,0.2,-10.81)) ;
#108027=CARTESIAN_POINT('Origin',(0.45,0.3,-10.61)) ;
#108028=CARTESIAN_POINT('Origin',(0.45,1.24941393210234E-16,-10.61)) ;
#108029=CARTESIAN_POINT('Origin',(0.45,4.4,-10.61)) ;
#108030=CARTESIAN_POINT('Origin',(0.45,4.4,-10.61)) ;
#108031=CARTESIAN_POINT('Origin',(0.45,4.4,-10.61)) ;
#108032=CARTESIAN_POINT('Origin',(0.549999999999999,4.4,-10.61)) ;
#108033=CARTESIAN_POINT('Origin',(-1.7,4.4,-10.61)) ;
#108034=CARTESIAN_POINT('Ctrl Pts',(-1.8,4.6,-10.81)) ;
#108035=CARTESIAN_POINT('Ctrl Pts',(-1.8,4.6,-10.81)) ;
#108036=CARTESIAN_POINT('Ctrl Pts',(-1.8,4.6,-10.81)) ;
#108037=CARTESIAN_POINT('Ctrl Pts',(-1.8,4.57374656717364,-10.7574931343473)) ;
#108038=CARTESIAN_POINT('Ctrl Pts',(-1.8,4.56045866731614,-10.7704586673162)) ;
#108039=CARTESIAN_POINT('Ctrl Pts',(-1.8,4.5474931343473,-10.7837465671736)) ;
#108040=CARTESIAN_POINT('Ctrl Pts',(-1.78922263893876,4.54780128270145,
-10.7056025654029)) ;
#108041=CARTESIAN_POINT('Ctrl Pts',(-1.77362528614074,4.52085344889012,
-10.7308534488902)) ;
#108042=CARTESIAN_POINT('Ctrl Pts',(-1.78922263893877,4.49560256540291,
-10.7578012827015)) ;
#108043=CARTESIAN_POINT('Ctrl Pts',(-1.7614546977086,4.5200333414713,-10.6500666829426)) ;
#108044=CARTESIAN_POINT('Ctrl Pts',(-1.73208554016475,4.49711619685843,
-10.7071161968584)) ;
#108045=CARTESIAN_POINT('Ctrl Pts',(-1.7614546977086,4.44006668294258,-10.7300333414713)) ;
#108046=CARTESIAN_POINT('Ctrl Pts',(-1.7503618540841,4.51262134295865,-10.6352426859173)) ;
#108047=CARTESIAN_POINT('Ctrl Pts',(-1.71792722356046,4.49498692411707,
-10.704986924117)) ;
#108048=CARTESIAN_POINT('Ctrl Pts',(-1.75036185408409,4.42524268591729,
-10.7226213429587)) ;
#108049=CARTESIAN_POINT('Ctrl Pts',(-1.72617483238892,4.50260275053909,
-10.6152055010782)) ;
#108050=CARTESIAN_POINT('Ctrl Pts',(-1.70094059868421,4.4967032564359,-10.7067032564359)) ;
#108051=CARTESIAN_POINT('Ctrl Pts',(-1.72617483238892,4.4052055010782,-10.7126027505391)) ;
#108052=CARTESIAN_POINT('Ctrl Pts',(-1.71309229646328,4.5,-10.6100000008183)) ;
#108053=CARTESIAN_POINT('Ctrl Pts',(-1.69945650151111,4.49999269607724,
-10.7099926960867)) ;
#108054=CARTESIAN_POINT('Ctrl Pts',(-1.71309229646328,4.40000000081823,
-10.71)) ;
#108055=CARTESIAN_POINT('Ctrl Pts',(-1.7,4.5,-10.61)) ;
#108056=CARTESIAN_POINT('Ctrl Pts',(-1.7,4.5,-10.71)) ;
#108057=CARTESIAN_POINT('Ctrl Pts',(-1.7,4.4,-10.71)) ;
#108058=CARTESIAN_POINT('Ctrl Pts',(-1.8,4.6,-9.51)) ;
#108059=CARTESIAN_POINT('Ctrl Pts',(-1.8,4.6,-9.51)) ;
#108060=CARTESIAN_POINT('Ctrl Pts',(-1.8,4.6,-9.51)) ;
#108061=CARTESIAN_POINT('Ctrl Pts',(-1.8,4.5474931343473,-9.53625343282638)) ;
#108062=CARTESIAN_POINT('Ctrl Pts',(-1.8,4.56045866731616,-9.54954133268381)) ;
#108063=CARTESIAN_POINT('Ctrl Pts',(-1.8,4.57374656717364,-9.56250686565271)) ;
#108064=CARTESIAN_POINT('Ctrl Pts',(-1.78922263893877,4.49560256540291,
-9.56219871729854)) ;
#108065=CARTESIAN_POINT('Ctrl Pts',(-1.77362528614073,4.52085344889015,
-9.58914655110983)) ;
#108066=CARTESIAN_POINT('Ctrl Pts',(-1.78922263893876,4.54780128270145,
-9.61439743459709)) ;
#108067=CARTESIAN_POINT('Ctrl Pts',(-1.7614546977086,4.44006668294258,-9.58996665852871)) ;
#108068=CARTESIAN_POINT('Ctrl Pts',(-1.73208554016475,4.49711619685842,
-9.6128838031416)) ;
#108069=CARTESIAN_POINT('Ctrl Pts',(-1.7614546977086,4.5200333414713,-9.66993331705742)) ;
#108070=CARTESIAN_POINT('Ctrl Pts',(-1.75036185408409,4.42524268591729,
-9.59737865704135)) ;
#108071=CARTESIAN_POINT('Ctrl Pts',(-1.71792722356046,4.49498692411707,
-9.61501307588296)) ;
#108072=CARTESIAN_POINT('Ctrl Pts',(-1.7503618540841,4.51262134295865,-9.68475731408271)) ;
#108073=CARTESIAN_POINT('Ctrl Pts',(-1.72617483238892,4.4052055010782,-9.60739724946091)) ;
#108074=CARTESIAN_POINT('Ctrl Pts',(-1.70094059868421,4.4967032564359,-9.61329674356408)) ;
#108075=CARTESIAN_POINT('Ctrl Pts',(-1.72617483238892,4.50260275053909,
-9.70479449892181)) ;
#108076=CARTESIAN_POINT('Ctrl Pts',(-1.71309229646328,4.40000000081823,
-9.61)) ;
#108077=CARTESIAN_POINT('Ctrl Pts',(-1.69945650152659,4.49999269603973,
-9.61000730391312)) ;
#108078=CARTESIAN_POINT('Ctrl Pts',(-1.71309229646328,4.5,-9.70999999918169)) ;
#108079=CARTESIAN_POINT('Ctrl Pts',(-1.7,4.4,-9.61)) ;
#108080=CARTESIAN_POINT('Ctrl Pts',(-1.7,4.5,-9.61)) ;
#108081=CARTESIAN_POINT('Ctrl Pts',(-1.7,4.5,-9.71)) ;
#108082=CARTESIAN_POINT('Origin',(-1.7,4.4,-9.71)) ;
#108083=CARTESIAN_POINT('Origin',(0.549999999999999,4.4,-9.71)) ;
#108084=CARTESIAN_POINT('Origin',(0.45,4.4,-9.71)) ;
#108085=CARTESIAN_POINT('Origin',(0.45,4.4,-9.71)) ;
#108086=CARTESIAN_POINT('Origin',(0.45,4.4,-9.71)) ;
#108087=CARTESIAN_POINT('Origin',(0.45,4.9047241136249E-17,-9.71)) ;
#108088=CARTESIAN_POINT('Origin',(0.45,0.3,-9.71)) ;
#108089=CARTESIAN_POINT('Ctrl Pts',(0.45,0.3,-9.61)) ;
#108090=CARTESIAN_POINT('Ctrl Pts',(0.55,0.3,-9.61)) ;
#108091=CARTESIAN_POINT('Ctrl Pts',(0.55,0.3,-9.71)) ;
#108092=CARTESIAN_POINT('Ctrl Pts',(0.450000000818259,0.286907703536723,
-9.61)) ;
#108093=CARTESIAN_POINT('Ctrl Pts',(0.549992696056779,0.300543498480462,
-9.61000730391316)) ;
#108094=CARTESIAN_POINT('Ctrl Pts',(0.55,0.28690770353672,-9.70999999918169)) ;
#108095=CARTESIAN_POINT('Ctrl Pts',(0.455205501078185,0.273825167611078,
-9.60739724946091)) ;
#108096=CARTESIAN_POINT('Ctrl Pts',(0.5467032564359,0.299059401315789,-9.6132967435641)) ;
#108097=CARTESIAN_POINT('Ctrl Pts',(0.552602750539093,0.273825167611082,
-9.7047944989218)) ;
#108098=CARTESIAN_POINT('Ctrl Pts',(0.4752426859173,0.249638145915905,-9.59737865704135)) ;
#108099=CARTESIAN_POINT('Ctrl Pts',(0.544986924117068,0.282072776439536,
-9.61501307588293)) ;
#108100=CARTESIAN_POINT('Ctrl Pts',(0.56262134295865,0.249638145915901,
-9.68475731408271)) ;
#108101=CARTESIAN_POINT('Ctrl Pts',(0.490066682942577,0.238545302291388,
-9.5899666585287)) ;
#108102=CARTESIAN_POINT('Ctrl Pts',(0.547116196858391,0.26791445983525,
-9.61288380314157)) ;
#108103=CARTESIAN_POINT('Ctrl Pts',(0.570033341471288,0.238545302291403,
-9.66993331705742)) ;
#108104=CARTESIAN_POINT('Ctrl Pts',(0.545602565402917,0.210777361061261,
-9.56219871729857)) ;
#108105=CARTESIAN_POINT('Ctrl Pts',(0.570853448890192,0.226374713859273,
-9.58914655110988)) ;
#108106=CARTESIAN_POINT('Ctrl Pts',(0.597801282701459,0.210777361061231,
-9.61439743459709)) ;
#108107=CARTESIAN_POINT('Ctrl Pts',(0.59749313434724,0.2,-9.53625343282625)) ;
#108108=CARTESIAN_POINT('Ctrl Pts',(0.61045866731604,0.2,-9.54954133268394)) ;
#108109=CARTESIAN_POINT('Ctrl Pts',(0.623746567173607,0.2,-9.56250686565271)) ;
#108110=CARTESIAN_POINT('Ctrl Pts',(0.65,0.2,-9.51)) ;
#108111=CARTESIAN_POINT('Ctrl Pts',(0.65,0.2,-9.51)) ;
#108112=CARTESIAN_POINT('Ctrl Pts',(0.65,0.2,-9.51)) ;
#108113=CARTESIAN_POINT('Ctrl Pts',(8.5,8.17221734381475,-10.7002872911617)) ;
#108114=CARTESIAN_POINT('Ctrl Pts',(8.5,8.17221734381475,-10.785)) ;
#108115=CARTESIAN_POINT('Ctrl Pts',(8.58356010126947,8.17221734381475,-10.7989266835449)) ;
#108116=CARTESIAN_POINT('Ctrl Pts',(8.5,8.23335379241386,-10.700287292739)) ;
#108117=CARTESIAN_POINT('Ctrl Pts',(8.5,8.2084742596065,-10.7774575674216)) ;
#108118=CARTESIAN_POINT('Ctrl Pts',(8.57460439031228,8.20580126077887,-10.797434065052)) ;
#108119=CARTESIAN_POINT('Ctrl Pts',(8.5,8.29192178062155,-10.7271741150785)) ;
#108120=CARTESIAN_POINT('Ctrl Pts',(8.5,8.25010493984403,-10.7892546083117)) ;
#108121=CARTESIAN_POINT('Ctrl Pts',(8.56800970738924,8.23725302684489,-10.8097783631899)) ;
#108122=CARTESIAN_POINT('Ctrl Pts',(8.5,8.36583651094027,-10.8165506232914)) ;
#108123=CARTESIAN_POINT('Ctrl Pts',(8.5,8.29925403146167,-10.8433614370366)) ;
#108124=CARTESIAN_POINT('Ctrl Pts',(8.56373266208983,8.27563607377072,-10.8537537764131)) ;
#108125=CARTESIAN_POINT('Ctrl Pts',(8.5,8.38029241321775,-10.8779552056997)) ;
#108126=CARTESIAN_POINT('Ctrl Pts',(8.5,8.30669116589131,-10.8848088499411)) ;
#108127=CARTESIAN_POINT('Ctrl Pts',(8.5661012385937,8.28208399509957,-10.884808702407)) ;
#108128=CARTESIAN_POINT('Ctrl Pts',(8.5,8.36719795478507,-10.9360547234799)) ;
#108129=CARTESIAN_POINT('Ctrl Pts',(8.5,8.29381262650623,-10.9195151496718)) ;
#108130=CARTESIAN_POINT('Ctrl Pts',(8.57227762885807,8.27346847343705,-10.9149299876354)) ;
#108131=CARTESIAN_POINT('Ctrl Pts',(8.5485213309235,8.28383177029354,-10.9159865327337)) ;
#108132=CARTESIAN_POINT('Ctrl Pts',(8.54913757890789,8.28625057716298,-10.902921659184)) ;
#108133=CARTESIAN_POINT('Ctrl Pts',(8.549146361399,8.28675781111762,-10.8892647894026)) ;
#108134=CARTESIAN_POINT('Ctrl Pts',(8.54883414737369,8.28489376483071,-10.876098869425)) ;
#108135=CARTESIAN_POINT('Ctrl Pts',(8.54852072231757,8.28302248819127,-10.8628818808428)) ;
#108136=CARTESIAN_POINT('Ctrl Pts',(8.54791723678494,8.27865742078997,-10.8498312958117)) ;
#108137=CARTESIAN_POINT('Ctrl Pts',(8.54677696932927,8.27237937104781,-10.8381020767297)) ;
#108138=CARTESIAN_POINT('Ctrl Pts',(8.5454465495755,8.26505438658866,-10.8244168797302)) ;
#108139=CARTESIAN_POINT('Ctrl Pts',(8.54324462275112,8.25487237915563,-10.8122537533388)) ;
#108140=CARTESIAN_POINT('Ctrl Pts',(8.53884071267076,8.24480815719263,-10.8012071681992)) ;
#108141=CARTESIAN_POINT('Ctrl Pts',(8.5342440055524,8.23430333763594,-10.7896769789768)) ;
#108142=CARTESIAN_POINT('Ctrl Pts',(8.52670159721618,8.22420330618022,-10.778704260243)) ;
#108143=CARTESIAN_POINT('Ctrl Pts',(8.51928858688475,8.21729138318396,-10.7659881754653)) ;
#108144=CARTESIAN_POINT('Ctrl Pts',(8.51327528614099,8.21168455548023,-10.755673116045)) ;
#108145=CARTESIAN_POINT('Ctrl Pts',(8.50759525524367,8.20778929846109,-10.7439849430828)) ;
#108146=CARTESIAN_POINT('Ctrl Pts',(8.50412058850191,8.20498026622232,-10.7315739486628)) ;
#108147=CARTESIAN_POINT('Ctrl Pts',(8.50147164778345,8.20283877743224,-10.7221123251694)) ;
#108148=CARTESIAN_POINT('Ctrl Pts',(8.50000317248551,8.2012555848359,-10.712083357655)) ;
#108149=CARTESIAN_POINT('Ctrl Pts',(8.50000000513446,8.20000405629318,-10.7021052387284)) ;
#108150=CARTESIAN_POINT('Origin',(8.6,8.17221734381475,-10.7002872911617)) ;
#108151=CARTESIAN_POINT('Origin',(8.6,4.35421736843756,-10.7002872911617)) ;
#108152=CARTESIAN_POINT('Origin',(8.6,6.66256607592813,-10.7002872911617)) ;
#108153=CARTESIAN_POINT('Ctrl Pts',(8.5,6.47083593368087,-10.9448081099244)) ;
#108154=CARTESIAN_POINT('Ctrl Pts',(8.5,6.55684090505321,-10.9243877386952)) ;
#108155=CARTESIAN_POINT('Ctrl Pts',(8.58772778625753,6.56739561896918,-10.921881707091)) ;
#108156=CARTESIAN_POINT('Ctrl Pts',(8.5,6.45680686388585,-10.8857215297177)) ;
#108157=CARTESIAN_POINT('Ctrl Pts',(8.49999999999995,6.54406229478603,-10.8925101654037)) ;
#108158=CARTESIAN_POINT('Ctrl Pts',(8.58195196310351,6.55941415012443,-10.8913576868779)) ;
#108159=CARTESIAN_POINT('Ctrl Pts',(8.5,6.47061556584389,-10.8219524568049)) ;
#108160=CARTESIAN_POINT('Ctrl Pts',(8.5,6.54836369988887,-10.8523987274071)) ;
#108161=CARTESIAN_POINT('Ctrl Pts',(8.57801125828726,6.56566601372231,-10.8588344592028)) ;
#108162=CARTESIAN_POINT('Ctrl Pts',(8.5,6.54379299301796,-10.7286264716581)) ;
#108163=CARTESIAN_POINT('Ctrl Pts',(8.5,6.59071789516225,-10.7962265152922)) ;
#108164=CARTESIAN_POINT('Ctrl Pts',(8.57642058265786,6.60198961470444,-10.8119063540245)) ;
#108165=CARTESIAN_POINT('Ctrl Pts',(8.5,6.60220518075381,-10.7002872929747)) ;
#108166=CARTESIAN_POINT('Ctrl Pts',(8.4999999999998,6.62800697860326,-10.7809176707627)) ;
#108167=CARTESIAN_POINT('Ctrl Pts',(8.57879135173927,6.63156920211804,-10.7981318919565)) ;
#108168=CARTESIAN_POINT('Ctrl Pts',(8.5,6.66256607592813,-10.7002872911617)) ;
#108169=CARTESIAN_POINT('Ctrl Pts',(8.5,6.66256607592813,-10.785)) ;
#108170=CARTESIAN_POINT('Ctrl Pts',(8.58356010126947,6.66256607592813,-10.7989266835449)) ;
#108171=CARTESIAN_POINT('',(8.54565366748546,6.6165071194701,-10.7939653182916)) ;
#108172=CARTESIAN_POINT('Ctrl Pts',(8.54565366716096,6.61650712004144,-10.7939653178134)) ;
#108173=CARTESIAN_POINT('Ctrl Pts',(8.54527684775561,6.61717057264373,-10.7934100008636)) ;
#108174=CARTESIAN_POINT('Ctrl Pts',(8.54488909343999,6.61782772231442,-10.7928554298996)) ;
#108175=CARTESIAN_POINT('Ctrl Pts',(8.54449064961557,6.61847724592624,-10.7923008713851)) ;
#108176=CARTESIAN_POINT('Ctrl Pts',(8.54445329550703,6.61853813876485,-10.7922488815243)) ;
#108177=CARTESIAN_POINT('Ctrl Pts',(8.5444158475797,6.61859896452238,-10.7921968917916)) ;
#108178=CARTESIAN_POINT('Ctrl Pts',(8.54437830610593,6.61865972207475,-10.7921449015858)) ;
#108179=CARTESIAN_POINT('Ctrl Pts',(8.54363538409139,6.61986207559674,-10.7911160483067)) ;
#108180=CARTESIAN_POINT('Ctrl Pts',(8.54285495000579,6.62104203503548,-10.7900848621745)) ;
#108181=CARTESIAN_POINT('Ctrl Pts',(8.54204093171137,6.62218056960146,-10.789051115167)) ;
#108182=CARTESIAN_POINT('Ctrl Pts',(8.54157979215428,6.62282554690612,-10.7884654997817)) ;
#108183=CARTESIAN_POINT('Ctrl Pts',(8.54110770812182,6.62345780120153,-10.7878786499066)) ;
#108184=CARTESIAN_POINT('Ctrl Pts',(8.54062344907117,6.62407892448169,-10.7872869541397)) ;
#108185=CARTESIAN_POINT('Ctrl Pts',(8.54011932596481,6.62472552591745,-10.7866709873185)) ;
#108186=CARTESIAN_POINT('Ctrl Pts',(8.53960207832255,6.62535666566134,-10.7860509905891)) ;
#108187=CARTESIAN_POINT('Ctrl Pts',(8.53907286520403,6.62597244099098,-10.785425228811)) ;
#108188=CARTESIAN_POINT('Ctrl Pts',(8.53887441028459,6.6262033567396,-10.7851905681443)) ;
#108189=CARTESIAN_POINT('Ctrl Pts',(8.53867427664141,6.6264321129994,-10.7849550998211)) ;
#108190=CARTESIAN_POINT('Ctrl Pts',(8.53847256319997,6.62665871795109,-10.7847187642184)) ;
#108191=CARTESIAN_POINT('Ctrl Pts',(8.53842843838465,6.62670828778427,-10.7846670658053)) ;
#108192=CARTESIAN_POINT('Ctrl Pts',(8.53838423811747,6.62675775467668,-10.7846153260175)) ;
#108193=CARTESIAN_POINT('Ctrl Pts',(8.53833996369343,6.62680711871688,-10.7845635444601)) ;
#108194=CARTESIAN_POINT('Ctrl Pts',(8.53829707284513,6.62685494013082,-10.7845133810765)) ;
#108195=CARTESIAN_POINT('Ctrl Pts',(8.53825411240223,6.62690266502019,-10.7844631784931)) ;
#108196=CARTESIAN_POINT('Ctrl Pts',(8.53821108363804,6.62695029346534,-10.7844129364377)) ;
#108197=CARTESIAN_POINT('Ctrl Pts',(8.53803571435326,6.62714440934378,-10.7842081684534)) ;
#108198=CARTESIAN_POINT('Ctrl Pts',(8.53785876035506,6.62733753498029,-10.7840021836648)) ;
#108199=CARTESIAN_POINT('Ctrl Pts',(8.53767995296703,6.62753033615257,-10.7837944665652)) ;
#108200=CARTESIAN_POINT('Ctrl Pts',(8.53649871780653,6.62880401687798,-10.7824222484251)) ;
#108201=CARTESIAN_POINT('Ctrl Pts',(8.53528300832264,6.62998038079528,-10.7810380760596)) ;
#108202=CARTESIAN_POINT('Ctrl Pts',(8.53403203676336,6.63110281535145,-10.7796044865649)) ;
#108203=CARTESIAN_POINT('Ctrl Pts',(8.5334687038968,6.63160826591215,-10.7789589178679)) ;
#108204=CARTESIAN_POINT('Ctrl Pts',(8.5328995953692,6.63209979040223,-10.7783054256595)) ;
#108205=CARTESIAN_POINT('Ctrl Pts',(8.53232661340319,6.63257735344031,-10.7776437014439)) ;
#108206=CARTESIAN_POINT('Ctrl Pts',(8.53206474273904,6.63279561467255,-10.7773412727985)) ;
#108207=CARTESIAN_POINT('Ctrl Pts',(8.53180206199565,6.63301096017663,-10.7770371260807)) ;
#108208=CARTESIAN_POINT('Ctrl Pts',(8.53153874718657,6.63322338883724,-10.7767312388807)) ;
#108209=CARTESIAN_POINT('Ctrl Pts',(8.53007363658218,6.63440536369244,-10.7750292511271)) ;
#108210=CARTESIAN_POINT('Ctrl Pts',(8.52858926277506,6.63549697414123,-10.7732730839131)) ;
#108211=CARTESIAN_POINT('Ctrl Pts',(8.52711342564664,6.6364985663511,-10.7714611393064)) ;
#108212=CARTESIAN_POINT('Ctrl Pts',(8.52634316954117,6.63702130866458,-10.7705154649028)) ;
#108213=CARTESIAN_POINT('Ctrl Pts',(8.52557615349969,6.63751985710295,-10.7695557193112)) ;
#108214=CARTESIAN_POINT('Ctrl Pts',(8.5248140182343,6.63799287689813,-10.7685803261613)) ;
#108215=CARTESIAN_POINT('Ctrl Pts',(8.52460710835822,6.63812129566006,-10.7683155195253)) ;
#108216=CARTESIAN_POINT('Ctrl Pts',(8.52440075574004,6.63824801482191,-10.7680497539023)) ;
#108217=CARTESIAN_POINT('Ctrl Pts',(8.52419502810871,6.63837284070829,-10.7677830860811)) ;
#108218=CARTESIAN_POINT('Ctrl Pts',(8.52404824365685,6.63846190263541,-10.7675928214593)) ;
#108219=CARTESIAN_POINT('Ctrl Pts',(8.52390173612803,6.63855002749203,-10.7674020437347)) ;
#108220=CARTESIAN_POINT('Ctrl Pts',(8.52375553261475,6.63863721305423,-10.7672107628049)) ;
#108221=CARTESIAN_POINT('Ctrl Pts',(8.52294204127159,6.63912232246441,-10.7661464560925)) ;
#108222=CARTESIAN_POINT('Ctrl Pts',(8.52213801365705,6.63957834748689,-10.7650665375564)) ;
#108223=CARTESIAN_POINT('Ctrl Pts',(8.5213477449051,6.64000494097979,-10.7639729614464)) ;
#108224=CARTESIAN_POINT('Ctrl Pts',(8.51876608595596,6.64139854145543,-10.7604004545695)) ;
#108225=CARTESIAN_POINT('Ctrl Pts',(8.51630176076717,6.64256282842069,-10.7566245667844)) ;
#108226=CARTESIAN_POINT('Ctrl Pts',(8.5140473780102,6.64354662431173,-10.7526687582287)) ;
#108227=CARTESIAN_POINT('Ctrl Pts',(8.51174271377016,6.64455236266853,-10.7486247197926)) ;
#108228=CARTESIAN_POINT('Ctrl Pts',(8.50965863261299,6.64536892721963,-10.7443937780696)) ;
#108229=CARTESIAN_POINT('Ctrl Pts',(8.50786496313904,6.64606338785377,-10.740044165486)) ;
#108230=CARTESIAN_POINT('Ctrl Pts',(8.50767015284865,6.64613881316471,-10.7395717544299)) ;
#108231=CARTESIAN_POINT('Ctrl Pts',(8.50747873128295,6.64621281334901,-10.7390979736876)) ;
#108232=CARTESIAN_POINT('Ctrl Pts',(8.50729076020858,6.64628549377757,-10.7386229301939)) ;
#108233=CARTESIAN_POINT('Ctrl Pts',(8.5072202710557,6.64631274893828,-10.7384447888838)) ;
#108234=CARTESIAN_POINT('Ctrl Pts',(8.50715026706479,6.64633981850992,-10.7382664700193)) ;
#108235=CARTESIAN_POINT('Ctrl Pts',(8.50708075128543,6.64636670806329,-10.7380879793595)) ;
#108236=CARTESIAN_POINT('Ctrl Pts',(8.50659414082986,6.6465549349369,-10.736838544741)) ;
#108237=CARTESIAN_POINT('Ctrl Pts',(8.5061314759289,6.64673434010344,-10.735580683755)) ;
#108238=CARTESIAN_POINT('Ctrl Pts',(8.50569363751093,6.64690683932496,-10.7343164275023)) ;
#108239=CARTESIAN_POINT('Ctrl Pts',(8.50395436040313,6.64759207829622,-10.7292942735102)) ;
#108240=CARTESIAN_POINT('Ctrl Pts',(8.50258205288462,6.64816393978853,-10.724091559621)) ;
#108241=CARTESIAN_POINT('Ctrl Pts',(8.50162662717307,6.64864720987411,-10.7188041247526)) ;
#108242=CARTESIAN_POINT('Ctrl Pts',(8.50156399248323,6.64867889153345,-10.7184574972346)) ;
#108243=CARTESIAN_POINT('Ctrl Pts',(8.50150313499629,6.6487101993589,-10.718110507519)) ;
#108244=CARTESIAN_POINT('Ctrl Pts',(8.50144406283923,6.64874114271681,-10.717763183502)) ;
#108245=CARTESIAN_POINT('Ctrl Pts',(8.50057491246565,6.64919642372272,-10.7126528774934)) ;
#108246=CARTESIAN_POINT('Ctrl Pts',(8.50009537300572,6.64957062705852,-10.7074713290505)) ;
#108247=CARTESIAN_POINT('Ctrl Pts',(8.50001293997569,6.64989933182553,-10.7023144435397)) ;
#108248=CARTESIAN_POINT('Ctrl Pts',(8.50000430878269,6.64993374902796,-10.7017744891782)) ;
#108249=CARTESIAN_POINT('Ctrl Pts',(8.5,6.64996765698298,-10.7012348144279)) ;
#108250=CARTESIAN_POINT('Ctrl Pts',(8.5,6.65000108682384,-10.7006955361059)) ;
#108251=CARTESIAN_POINT('',(8.55245136877624,6.6009799437261,-10.8067801193796)) ;
#108252=CARTESIAN_POINT('Ctrl Pts',(8.55238056475493,6.60105295171775,-10.8068886154986)) ;
#108253=CARTESIAN_POINT('Ctrl Pts',(8.55170523171899,6.60308542368598,-10.8051022656145)) ;
#108254=CARTESIAN_POINT('Ctrl Pts',(8.55095829520335,6.60513808680204,-10.8033627348215)) ;
#108255=CARTESIAN_POINT('Ctrl Pts',(8.55012599030478,6.6071915298049,-10.8016544441805)) ;
#108256=CARTESIAN_POINT('Ctrl Pts',(8.54968322947846,6.60828389886617,-10.8007456856509)) ;
#108257=CARTESIAN_POINT('Ctrl Pts',(8.54921644930851,6.60937569995309,-10.7998462491231)) ;
#108258=CARTESIAN_POINT('Ctrl Pts',(8.54872481267394,6.61045954913298,-10.7989557465495)) ;
#108259=CARTESIAN_POINT('Ctrl Pts',(8.54779539897816,6.61250851009549,-10.7972722973719)) ;
#108260=CARTESIAN_POINT('Ctrl Pts',(8.54677348694547,6.61453549290076,-10.7956155908862)) ;
#108261=CARTESIAN_POINT('Ctrl Pts',(8.54565366748546,6.6165071194701,-10.7939653182916)) ;
#108262=CARTESIAN_POINT('',(8.55735473176743,6.58264207262467,-10.8249557973614)) ;
#108263=CARTESIAN_POINT('Ctrl Pts',(8.55735473168698,6.58264207302803,-10.8249557968439)) ;
#108264=CARTESIAN_POINT('Ctrl Pts',(8.55706916598051,6.58397660851281,-10.8232296933712)) ;
#108265=CARTESIAN_POINT('Ctrl Pts',(8.55678088122702,6.58528501693267,-10.8216621009602)) ;
#108266=CARTESIAN_POINT('Ctrl Pts',(8.5564740809182,6.58661569125897,-10.8201718232514)) ;
#108267=CARTESIAN_POINT('Ctrl Pts',(8.55614409617578,6.5880469226241,-10.8185689275185)) ;
#108268=CARTESIAN_POINT('Ctrl Pts',(8.55579261555188,6.58950524590115,-10.8170567950172)) ;
#108269=CARTESIAN_POINT('Ctrl Pts',(8.55539993844504,6.59102291080536,-10.8155875677793)) ;
#108270=CARTESIAN_POINT('Ctrl Pts',(8.55517214917306,6.59190329771265,-10.8147352792269)) ;
#108271=CARTESIAN_POINT('Ctrl Pts',(8.5549304988196,6.59280308289164,-10.8138983977538)) ;
#108272=CARTESIAN_POINT('Ctrl Pts',(8.55467134659044,6.59372113732161,-10.8130707946418)) ;
#108273=CARTESIAN_POINT('Ctrl Pts',(8.55434805237167,6.59486641664526,-10.8120383539701)) ;
#108274=CARTESIAN_POINT('Ctrl Pts',(8.55400737519029,6.59602723165038,-10.8110361981957)) ;
#108275=CARTESIAN_POINT('Ctrl Pts',(8.55365328858767,6.59718920061513,-10.8100452155133)) ;
#108276=CARTESIAN_POINT('Ctrl Pts',(8.5532816788869,6.59840867329807,-10.809005190911)) ;
#108277=CARTESIAN_POINT('Ctrl Pts',(8.55289390107691,6.59963546460033,-10.8079736796762)) ;
#108278=CARTESIAN_POINT('Ctrl Pts',(8.55249886556663,6.60083562835463,-10.8069081494348)) ;
#108279=CARTESIAN_POINT('Ctrl Pts',(8.5524830476332,6.60088368507326,-10.8068654836845)) ;
#108280=CARTESIAN_POINT('Ctrl Pts',(8.55246721522814,6.6009317901722,-10.806822806733)) ;
#108281=CARTESIAN_POINT('Ctrl Pts',(8.55245136877624,6.6009799437261,-10.8067801193796)) ;
#108282=CARTESIAN_POINT('Ctrl Pts',(8.56107669735261,6.5600938800009,-10.9223838472224)) ;
#108283=CARTESIAN_POINT('Ctrl Pts',(8.56115635543005,6.55978170524809,-10.9208207343832)) ;
#108284=CARTESIAN_POINT('Ctrl Pts',(8.56122592915386,6.55950119162287,-10.9192507129806)) ;
#108285=CARTESIAN_POINT('Ctrl Pts',(8.56128584055879,6.55925348717443,-10.9176933919486)) ;
#108286=CARTESIAN_POINT('Ctrl Pts',(8.56142626445294,6.55867290283843,-10.9140432508109)) ;
#108287=CARTESIAN_POINT('Ctrl Pts',(8.56152217534693,6.55825854507367,-10.910375633877)) ;
#108288=CARTESIAN_POINT('Ctrl Pts',(8.5615808174699,6.55798577878935,-10.9066701354254)) ;
#108289=CARTESIAN_POINT('Ctrl Pts',(8.56158917845351,6.55794688875061,-10.9061418187433)) ;
#108290=CARTESIAN_POINT('Ctrl Pts',(8.56159677639836,6.55791088241229,-10.9056126452595)) ;
#108291=CARTESIAN_POINT('Ctrl Pts',(8.56160362608008,6.55787769947531,-10.9050824674717)) ;
#108292=CARTESIAN_POINT('Ctrl Pts',(8.56164117305277,6.55769580506315,-10.902176263686)) ;
#108293=CARTESIAN_POINT('Ctrl Pts',(8.56164095204358,6.55766773657216,-10.8992640119966)) ;
#108294=CARTESIAN_POINT('Ctrl Pts',(8.5616130623009,6.55774920537472,-10.8963655672583)) ;
#108295=CARTESIAN_POINT('Ctrl Pts',(8.56157759693123,6.55785280336171,-10.8926798246079)) ;
#108296=CARTESIAN_POINT('Ctrl Pts',(8.56150275624661,6.55813669070951,-10.889004928021)) ;
#108297=CARTESIAN_POINT('Ctrl Pts',(8.56141108129146,6.55856506509338,-10.8853632925482)) ;
#108298=CARTESIAN_POINT('Ctrl Pts',(8.56136615997221,6.55877497130414,-10.883578867681)) ;
#108299=CARTESIAN_POINT('Ctrl Pts',(8.56131707129298,6.55902016312284,-10.8818016709684)) ;
#108300=CARTESIAN_POINT('Ctrl Pts',(8.56126585691692,6.55929956116446,-10.8800315254682)) ;
#108301=CARTESIAN_POINT('Ctrl Pts',(8.56116752027493,6.55983603289967,-10.8766326719095)) ;
#108302=CARTESIAN_POINT('Ctrl Pts',(8.56104954130216,6.56049109659203,-10.8732540075756)) ;
#108303=CARTESIAN_POINT('Ctrl Pts',(8.56091150449775,6.56129147625802,-10.8698304710248)) ;
#108304=CARTESIAN_POINT('Ctrl Pts',(8.56080235670743,6.56192434857305,-10.8671234288616)) ;
#108305=CARTESIAN_POINT('Ctrl Pts',(8.56068045333715,6.56264902401855,-10.8643872666893)) ;
#108306=CARTESIAN_POINT('Ctrl Pts',(8.56054379825318,6.56349285586902,-10.8616234877211)) ;
#108307=CARTESIAN_POINT('Ctrl Pts',(8.56050762866484,6.56371619955871,-10.860891976352)) ;
#108308=CARTESIAN_POINT('Ctrl Pts',(8.56047042218818,6.56394794674724,-10.8601587916983)) ;
#108309=CARTESIAN_POINT('Ctrl Pts',(8.56043213901761,6.56418871538695,-10.8594246234709)) ;
#108310=CARTESIAN_POINT('Ctrl Pts',(8.56026887460239,6.56521550994376,-10.8562936511792)) ;
#108311=CARTESIAN_POINT('Ctrl Pts',(8.56008532870545,6.56636514336274,-10.8532612149347)) ;
#108312=CARTESIAN_POINT('Ctrl Pts',(8.5598891591871,6.56762686151827,-10.8504713276669)) ;
#108313=CARTESIAN_POINT('Ctrl Pts',(8.55964574654527,6.5691924368027,-10.8470095572757)) ;
#108314=CARTESIAN_POINT('Ctrl Pts',(8.55938661160132,6.57080906160866,-10.843732634051)) ;
#108315=CARTESIAN_POINT('Ctrl Pts',(8.55911582090257,6.57246439798289,-10.840667212428)) ;
#108316=CARTESIAN_POINT('Ctrl Pts',(8.55888928658551,6.5738491962672,-10.8381027846354)) ;
#108317=CARTESIAN_POINT('Ctrl Pts',(8.5586381350289,6.57544444689329,-10.8353653454312)) ;
#108318=CARTESIAN_POINT('Ctrl Pts',(8.55834707044208,6.57718152485395,-10.832668125823)) ;
#108319=CARTESIAN_POINT('Ctrl Pts',(8.55828762047112,6.57753632320108,-10.8321172184483)) ;
#108320=CARTESIAN_POINT('Ctrl Pts',(8.55822651695171,6.57789694345782,-10.8315678465791)) ;
#108321=CARTESIAN_POINT('Ctrl Pts',(8.55816364958868,6.57826264684155,-10.8310215710793)) ;
#108322=CARTESIAN_POINT('Ctrl Pts',(8.55792499569721,6.57965091145842,-10.828947827764)) ;
#108323=CARTESIAN_POINT('Ctrl Pts',(8.5576603261423,6.58110993502793,-10.8269213132876)) ;
#108324=CARTESIAN_POINT('Ctrl Pts',(8.55735473176743,6.58264207262467,-10.8249557973614)) ;
#108325=CARTESIAN_POINT('Origin',(8.49172374697018,6.65,-12.7)) ;
#108326=CARTESIAN_POINT('Origin',(8.49226931255791,6.63793757615624,-10.9329882716319)) ;
#108327=CARTESIAN_POINT('Ctrl Pts',(8.40188506081778,6.5500005341705,-10.6715458308154)) ;
#108328=CARTESIAN_POINT('Ctrl Pts',(8.50280744587441,6.54966497091139,-10.6851950407542)) ;
#108329=CARTESIAN_POINT('Ctrl Pts',(8.50109204799973,6.65199687180763,-10.6856804549399)) ;
#108330=CARTESIAN_POINT('Ctrl Pts',(8.39296932930807,6.55000052027914,-10.7296758024219)) ;
#108331=CARTESIAN_POINT('Ctrl Pts',(8.49725036372766,6.54968051003383,-10.7169136026831)) ;
#108332=CARTESIAN_POINT('Ctrl Pts',(8.4966529651636,6.649356723178,-10.7160247114635)) ;
#108333=CARTESIAN_POINT('Ctrl Pts',(8.4114607955856,6.55000052635931,-10.7896088846459)) ;
#108334=CARTESIAN_POINT('Ctrl Pts',(8.50278789772746,6.54967384197898,-10.7410143519806)) ;
#108335=CARTESIAN_POINT('Ctrl Pts',(8.50590954255551,6.65051247736746,-10.7444272120936)) ;
#108336=CARTESIAN_POINT('Ctrl Pts',(8.45744515914182,6.55000045243508,-10.8428021918821)) ;
#108337=CARTESIAN_POINT('Ctrl Pts',(8.52023811680809,6.54973725194868,-10.781633015821)) ;
#108338=CARTESIAN_POINT('Ctrl Pts',(8.5289172307313,6.63643009777376,-10.7734751630783)) ;
#108339=CARTESIAN_POINT('Ctrl Pts',(8.46608867121689,6.55000043643008,-10.8511950991747)) ;
#108340=CARTESIAN_POINT('Ctrl Pts',(8.52334270167617,6.54974993059837,-10.7884702400789)) ;
#108341=CARTESIAN_POINT('Ctrl Pts',(8.53324349789231,6.63337968978886,-10.7782208913001)) ;
#108342=CARTESIAN_POINT('Ctrl Pts',(8.48465388181691,6.55000038323734,-10.8665763138744)) ;
#108343=CARTESIAN_POINT('Ctrl Pts',(8.53001210036428,6.5497893864682,-10.8051245951232)) ;
#108344=CARTESIAN_POINT('Ctrl Pts',(8.54253954944034,6.6232371034799,-10.788863146269)) ;
#108345=CARTESIAN_POINT('Ctrl Pts',(8.49467048074917,6.55000035131511,-10.8734884944613)) ;
#108346=CARTESIAN_POINT('Ctrl Pts',(8.53347884787438,6.54981166882502,-10.8130590311501)) ;
#108347=CARTESIAN_POINT('Ctrl Pts',(8.54755337534731,6.61714793548855,-10.7928676881263)) ;
#108348=CARTESIAN_POINT('Ctrl Pts',(8.50997930894009,6.55000022766094,-10.8833889027857)) ;
#108349=CARTESIAN_POINT('Ctrl Pts',(8.5386903515922,6.54988741100168,-10.8387742327548)) ;
#108350=CARTESIAN_POINT('Ctrl Pts',(8.55523846583761,6.59353839814627,-10.8135278831083)) ;
#108351=CARTESIAN_POINT('Ctrl Pts',(8.51532901080107,6.55000016113069,-10.8863389673192)) ;
#108352=CARTESIAN_POINT('Ctrl Pts',(8.54023459682689,6.54992340374046,-10.848489748387)) ;
#108353=CARTESIAN_POINT('Ctrl Pts',(8.55790835982308,6.58082417519551,-10.8215823085726)) ;
#108354=CARTESIAN_POINT('Ctrl Pts',(8.52186010906347,6.55000005932357,-10.8927927598772)) ;
#108355=CARTESIAN_POINT('Ctrl Pts',(8.54265823247977,6.5499732773141,-10.8779316441153)) ;
#108356=CARTESIAN_POINT('Ctrl Pts',(8.56121746518601,6.56135337205744,-10.8645883700756)) ;
#108357=CARTESIAN_POINT('Ctrl Pts',(8.52354993939972,6.55000003603139,-10.8958242622279)) ;
#108358=CARTESIAN_POINT('Ctrl Pts',(8.54350769968241,6.54998394755847,-10.8914238732007)) ;
#108359=CARTESIAN_POINT('Ctrl Pts',(8.5621431061544,6.55689632415131,-10.8874501335625)) ;
#108360=CARTESIAN_POINT('Ctrl Pts',(8.52268461318112,6.55000004733863,-10.9017875304158)) ;
#108361=CARTESIAN_POINT('Ctrl Pts',(8.54305517585924,6.54997881410037,-10.91281341214)) ;
#108362=CARTESIAN_POINT('Ctrl Pts',(8.5615325917139,6.55906016573919,-10.9227901815805)) ;
#108363=CARTESIAN_POINT('Ctrl Pts',(8.52060566253928,6.55000006807331,-10.9044138065497)) ;
#108364=CARTESIAN_POINT('Ctrl Pts',(8.54195943530538,6.54996919659463,-10.9204945748859)) ;
#108365=CARTESIAN_POINT('Ctrl Pts',(8.56058441628599,6.56302742363386,-10.9345079215137)) ;
#108366=CARTESIAN_POINT('Ctrl Pts',(8.51445291480387,6.55000012130567,-10.9112328149553)) ;
#108367=CARTESIAN_POINT('Ctrl Pts',(8.53868948987838,6.54994355920611,-10.9394191817675)) ;
#108368=CARTESIAN_POINT('Ctrl Pts',(8.55750149922673,6.57320954252653,-10.9611844353068)) ;
#108369=CARTESIAN_POINT('Ctrl Pts',(8.50953280296017,6.55000015625148,-10.9150479464373)) ;
#108370=CARTESIAN_POINT('Ctrl Pts',(8.53616288920968,6.54992588038507,-10.9477647485266)) ;
#108371=CARTESIAN_POINT('Ctrl Pts',(8.55504783006515,6.57989127253964,-10.9706993167928)) ;
#108372=CARTESIAN_POINT('Ctrl Pts',(8.49261655785715,6.55000026291039,-10.928492606569)) ;
#108373=CARTESIAN_POINT('Ctrl Pts',(8.52778251455091,6.5498671840875,-10.9757691608948)) ;
#108374=CARTESIAN_POINT('Ctrl Pts',(8.54658667616929,6.60027178071329,-10.9993533757438)) ;
#108375=CARTESIAN_POINT('Ctrl Pts',(8.48022165824505,6.55000031608562,-10.9377685341603)) ;
#108376=CARTESIAN_POINT('Ctrl Pts',(8.52288681814155,6.54983437262023,-10.987455948929)) ;
#108377=CARTESIAN_POINT('Ctrl Pts',(8.5404533945046,6.61042388759274,-11.0063019909605)) ;
#108378=CARTESIAN_POINT('Ctrl Pts',(8.46952991654832,6.55000035836672,-10.9490954462194)) ;
#108379=CARTESIAN_POINT('Ctrl Pts',(8.51900842894258,6.54980714069637,-11.0033676846771)) ;
#108380=CARTESIAN_POINT('Ctrl Pts',(8.53471369258706,6.61849392543723,-11.021383368443)) ;
#108381=CARTESIAN_POINT('Origin',(8.4,6.65,-10.7006780018997)) ;
#108382=CARTESIAN_POINT('Ctrl Pts',(8.54848814460234,8.28374914930622,-9.40353717477989)) ;
#108383=CARTESIAN_POINT('Ctrl Pts',(8.55964225199693,8.27720012980426,-9.40496794832229)) ;
#108384=CARTESIAN_POINT('Ctrl Pts',(8.572140519951,8.27365818248462,-9.40574176255693)) ;
#108385=CARTESIAN_POINT('Ctrl Pts',(8.54519582228985,8.29111303851996,-9.4279603788076)) ;
#108386=CARTESIAN_POINT('Ctrl Pts',(8.55569959891137,8.28406912459881,-9.42803761744086)) ;
#108387=CARTESIAN_POINT('Ctrl Pts',(8.56757951573628,8.27991709749371,-9.42819163391183)) ;
#108388=CARTESIAN_POINT('Ctrl Pts',(8.54340782920288,8.28927570119136,-9.45382299312326)) ;
#108389=CARTESIAN_POINT('Ctrl Pts',(8.55355053837511,8.282326185643,-9.45215464428979)) ;
#108390=CARTESIAN_POINT('Ctrl Pts',(8.56507848568421,8.27803412520746,-9.45113214305331)) ;
#108391=CARTESIAN_POINT('Ctrl Pts',(8.54340835145922,8.27841951799441,-9.47553501116171)) ;
#108392=CARTESIAN_POINT('Ctrl Pts',(8.55355093564017,8.27219257320284,-9.47242153876592)) ;
#108393=CARTESIAN_POINT('Ctrl Pts',(8.56507848521152,8.26835005667905,-9.47050028050403)) ;
#108394=CARTESIAN_POINT('Ctrl Pts',(8.54742026180265,8.27608084857565,-9.4743656412486)) ;
#108395=CARTESIAN_POINT('Ctrl Pts',(8.54754672558908,8.27683897030433,-9.47267457303652)) ;
#108396=CARTESIAN_POINT('Ctrl Pts',(8.54766225486891,8.27755642830997,-9.47096549730836)) ;
#108397=CARTESIAN_POINT('Ctrl Pts',(8.54776713596766,8.27823455672264,-9.46923501677752)) ;
#108398=CARTESIAN_POINT('Ctrl Pts',(8.54791712013336,8.27920430747293,-9.46676036041189)) ;
#108399=CARTESIAN_POINT('Ctrl Pts',(8.54806168001142,8.28008011045348,-9.46424633726765)) ;
#108400=CARTESIAN_POINT('Ctrl Pts',(8.54818998754192,8.28086237513953,-9.461718683859)) ;
#108401=CARTESIAN_POINT('Ctrl Pts',(8.5482419492675,8.28117917511833,-9.46069503986669)) ;
#108402=CARTESIAN_POINT('Ctrl Pts',(8.54829140719363,8.28148078264968,-9.45966867429037)) ;
#108403=CARTESIAN_POINT('Ctrl Pts',(8.54833813644415,8.28176759858573,-9.45863962997721)) ;
#108404=CARTESIAN_POINT('Ctrl Pts',(8.54850061324771,8.28276485268195,-9.4550616605289)) ;
#108405=CARTESIAN_POINT('Ctrl Pts',(8.54863339756397,8.28360845633787,-9.45135012352872)) ;
#108406=CARTESIAN_POINT('Ctrl Pts',(8.54873421749658,8.28426438239348,-9.44761308675746)) ;
#108407=CARTESIAN_POINT('Ctrl Pts',(8.54878752953697,8.28461122607277,-9.445636998794)) ;
#108408=CARTESIAN_POINT('Ctrl Pts',(8.54883168679926,8.2849064071404,-9.44365408207379)) ;
#108409=CARTESIAN_POINT('Ctrl Pts',(8.54886500248132,8.28515040605084,-9.44168185902952)) ;
#108410=CARTESIAN_POINT('Ctrl Pts',(8.5488738542235,8.28521523484357,-9.44115785325128)) ;
#108411=CARTESIAN_POINT('Ctrl Pts',(8.54888411330031,8.285275121517,-9.44063500919221)) ;
#108412=CARTESIAN_POINT('Ctrl Pts',(8.54889386083023,8.2853314308609,-9.44011208678616)) ;
#108413=CARTESIAN_POINT('Ctrl Pts',(8.54894969070931,8.28565394783543,-9.43711700034693)) ;
#108414=CARTESIAN_POINT('Ctrl Pts',(8.5489793513821,8.28586680424119,-9.43409863638302)) ;
#108415=CARTESIAN_POINT('Ctrl Pts',(8.54899968230028,8.28595875954336,-9.43106757780142)) ;
#108416=CARTESIAN_POINT('Ctrl Pts',(8.54900356561227,8.28597632348829,-9.43048862971749)) ;
#108417=CARTESIAN_POINT('Ctrl Pts',(8.54900713937599,8.28598945835116,-9.42990930880417)) ;
#108418=CARTESIAN_POINT('Ctrl Pts',(8.54901057288909,8.28599806377619,-9.42932984021849)) ;
#108419=CARTESIAN_POINT('Ctrl Pts',(8.54902784271198,8.28604134718934,-9.42641523947596)) ;
#108420=CARTESIAN_POINT('Ctrl Pts',(8.54901619593281,8.28598556136223,-9.4235157757218)) ;
#108421=CARTESIAN_POINT('Ctrl Pts',(8.5489843126011,8.28582669412323,-9.42060642867561)) ;
#108422=CARTESIAN_POINT('Ctrl Pts',(8.54893914418925,8.28560163041442,-9.41648482096991)) ;
#108423=CARTESIAN_POINT('Ctrl Pts',(8.54884805310403,8.28517290646448,-9.41237709996714)) ;
#108424=CARTESIAN_POINT('Ctrl Pts',(8.54869940582915,8.28455561418431,-9.40830707741439)) ;
#108425=CARTESIAN_POINT('Ctrl Pts',(8.54864697316337,8.28433787538059,-9.40687144980293)) ;
#108426=CARTESIAN_POINT('Ctrl Pts',(8.54858736435355,8.2840967659742,-9.40544083959257)) ;
#108427=CARTESIAN_POINT('Ctrl Pts',(8.54851996240544,8.28383343043592,-9.40401720308528)) ;
#108428=CARTESIAN_POINT('Origin',(8.4,6.65,-12.7)) ;
#108429=CARTESIAN_POINT('Origin',(8.4,6.65,-9.6193219981003)) ;
#108430=CARTESIAN_POINT('Origin',(8.49172374697018,6.65,-12.7)) ;
#108431=CARTESIAN_POINT('Origin',(8.4922548564967,6.63809817877304,-9.38700862834994)) ;
#108432=CARTESIAN_POINT('Origin',(8.6,4.35421736843756,-9.61971270883831)) ;
#108433=CARTESIAN_POINT('Origin',(8.6,6.66256607592813,-9.61971270883831)) ;
#108434=CARTESIAN_POINT('Ctrl Pts',(8.50134874936241,6.65217253603383,-9.63598525608075)) ;
#108435=CARTESIAN_POINT('Ctrl Pts',(8.50315244876583,6.5499712757702,-9.63658636925848)) ;
#108436=CARTESIAN_POINT('Ctrl Pts',(8.40269444133659,6.55000000392137,-9.6515964965758)) ;
#108437=CARTESIAN_POINT('Ctrl Pts',(8.4963175378395,6.6493370187709,-9.60501565239566)) ;
#108438=CARTESIAN_POINT('Ctrl Pts',(8.49707874924871,6.54997270174421,-9.60396122349838)) ;
#108439=CARTESIAN_POINT('Ctrl Pts',(8.39261127161985,6.55000000381175,-9.59255502081079)) ;
#108440=CARTESIAN_POINT('Ctrl Pts',(8.50556246021205,6.65075235208957,-9.57601104550147)) ;
#108441=CARTESIAN_POINT('Ctrl Pts',(8.50253957946704,6.54997202229482,-9.57964413045453)) ;
#108442=CARTESIAN_POINT('Ctrl Pts',(8.41103525938988,6.55000000386643,-9.53133834963448)) ;
#108443=CARTESIAN_POINT('Ctrl Pts',(8.52891970071471,6.63645479210457,-9.54652715848278)) ;
#108444=CARTESIAN_POINT('Ctrl Pts',(8.52027792490147,6.54997752826668,-9.53840493996115)) ;
#108445=CARTESIAN_POINT('Ctrl Pts',(8.4576425585103,6.5500000033157,-9.47739010158303)) ;
#108446=CARTESIAN_POINT('Ctrl Pts',(8.53324635448929,6.63340383613804,-9.54178206573817)) ;
#108447=CARTESIAN_POINT('Ctrl Pts',(8.52338394863782,6.54997861189313,-9.53157331389089)) ;
#108448=CARTESIAN_POINT('Ctrl Pts',(8.46627109069292,6.55000000319827,-9.4690047485327)) ;
#108449=CARTESIAN_POINT('Ctrl Pts',(8.54254332011239,6.62325922024831,-9.53114174821779)) ;
#108450=CARTESIAN_POINT('Ctrl Pts',(8.53005572430512,6.54998198465676,-9.51493264246807)) ;
#108451=CARTESIAN_POINT('Ctrl Pts',(8.48480454940901,6.55000000280808,-9.45362780882311)) ;
#108452=CARTESIAN_POINT('Ctrl Pts',(8.54755771953123,6.61716872587379,-9.52713854387739)) ;
#108453=CARTESIAN_POINT('Ctrl Pts',(8.53352383957155,6.54998388968238,-9.5070066149148)) ;
#108454=CARTESIAN_POINT('Ctrl Pts',(8.49480263348501,6.55000000257396,-9.44671727629916)) ;
#108455=CARTESIAN_POINT('Ctrl Pts',(8.55524400651032,6.59355301617583,-9.50648056989544)) ;
#108456=CARTESIAN_POINT('Ctrl Pts',(8.53873552501328,6.54999036710749,-9.48129485880943)) ;
#108457=CARTESIAN_POINT('Ctrl Pts',(8.51008526949052,6.55000000166752,-9.43677574941853)) ;
#108458=CARTESIAN_POINT('Ctrl Pts',(8.55791451833573,6.58083494429021,-9.49842706746385)) ;
#108459=CARTESIAN_POINT('Ctrl Pts',(8.54027978136636,6.54999344602542,-9.47157902883428)) ;
#108460=CARTESIAN_POINT('Ctrl Pts',(8.51542462880457,6.55000000118004,-9.43380634433862)) ;
#108461=CARTESIAN_POINT('Ctrl Pts',(8.56122429319342,6.56135755929237,-9.45541653896343)) ;
#108462=CARTESIAN_POINT('Ctrl Pts',(8.54270214007071,6.54999771321876,-9.44209990564423)) ;
#108463=CARTESIAN_POINT('Ctrl Pts',(8.52194436340203,6.55000000043437,-9.42726744367389)) ;
#108464=CARTESIAN_POINT('Ctrl Pts',(8.56215003896757,6.55689889598544,-9.43255134475621)) ;
#108465=CARTESIAN_POINT('Ctrl Pts',(8.54355112280984,6.54999862629018,-9.42858541402148)) ;
#108466=CARTESIAN_POINT('Ctrl Pts',(8.52363168464777,6.55000000026381,-9.42419376079454)) ;
#108467=CARTESIAN_POINT('Ctrl Pts',(8.56153943432817,6.55906352913392,-9.39720612379093)) ;
#108468=CARTESIAN_POINT('Ctrl Pts',(8.54309854033144,6.5499981870035,-9.40716316826849)) ;
#108469=CARTESIAN_POINT('Ctrl Pts',(8.52276767133746,6.5500000003466,-9.41816751318002)) ;
#108470=CARTESIAN_POINT('Ctrl Pts',(8.56059123720042,6.56303220640812,-9.38548694646253)) ;
#108471=CARTESIAN_POINT('Ctrl Pts',(8.54200379397878,6.54999736403672,-9.39947204706566)) ;
#108472=CARTESIAN_POINT('Ctrl Pts',(8.52069177703237,6.55000000049844,-9.41552134373608)) ;
#108473=CARTESIAN_POINT('Ctrl Pts',(8.55750819780173,6.57321782814891,-9.35880781453251)) ;
#108474=CARTESIAN_POINT('Ctrl Pts',(8.53873610184734,6.54999517041881,-9.38052685964291)) ;
#108475=CARTESIAN_POINT('Ctrl Pts',(8.51454797734041,6.55000000088831,-9.40865663082411)) ;
#108476=CARTESIAN_POINT('Ctrl Pts',(8.55505442469282,6.57990173798309,-9.34929267446123)) ;
#108477=CARTESIAN_POINT('Ctrl Pts',(8.53621107118182,6.54999365791211,-9.37217666040664)) ;
#108478=CARTESIAN_POINT('Ctrl Pts',(8.50963525726155,6.55000000114429,-9.40482618291573)) ;
#108479=CARTESIAN_POINT('Ctrl Pts',(8.55022399280474,6.59153973477787,-9.33293520591855)) ;
#108480=CARTESIAN_POINT('Ctrl Pts',(8.53156015545169,6.54999086985382,-9.35662116717933)) ;
#108481=CARTESIAN_POINT('Ctrl Pts',(8.49999539447558,6.55000000159032,-9.3971278236794)) ;
#108482=CARTESIAN_POINT('Ctrl Pts',(8.54779538881609,6.59665349532941,-9.32691619169829)) ;
#108483=CARTESIAN_POINT('Ctrl Pts',(8.5293657515114,6.54998957391998,-9.34999554735591)) ;
#108484=CARTESIAN_POINT('Ctrl Pts',(8.49512741158075,6.55000000178643,-9.39333641589862)) ;
#108485=CARTESIAN_POINT('Ctrl Pts',(8.54538355337156,6.60121171185029,-9.32167517448425)) ;
#108486=CARTESIAN_POINT('Ctrl Pts',(8.52733415536172,6.54998837980797,-9.34389835720993)) ;
#108487=CARTESIAN_POINT('Ctrl Pts',(8.49033880598513,6.55000000196131,-9.38944859709871)) ;
#108488=CARTESIAN_POINT('',(8.54582344182381,6.61635369861669,-9.52606365157295)) ;
#108489=CARTESIAN_POINT('Ctrl Pts',(8.54582344182381,6.61635369861669,-9.52606365157295)) ;
#108490=CARTESIAN_POINT('Ctrl Pts',(8.54493595163519,6.61793460914654,-9.52739407620991)) ;
#108491=CARTESIAN_POINT('Ctrl Pts',(8.5439844817107,6.61948114927954,-9.52871739283071)) ;
#108492=CARTESIAN_POINT('Ctrl Pts',(8.54296332801272,6.6209780844369,-9.53004073677983)) ;
#108493=CARTESIAN_POINT('Ctrl Pts',(8.53827263106763,6.62785429629763,-9.53611955276191)) ;
#108494=CARTESIAN_POINT('Ctrl Pts',(8.53198779426187,6.63349037496299,-9.54261156852439)) ;
#108495=CARTESIAN_POINT('Ctrl Pts',(8.5259873730411,6.63731070037229,-9.5500705892422)) ;
#108496=CARTESIAN_POINT('Ctrl Pts',(8.52000560405467,6.64111915034781,-9.55750642368737)) ;
#108497=CARTESIAN_POINT('Ctrl Pts',(8.51430181273566,6.64349626850742,-9.56603764730141)) ;
#108498=CARTESIAN_POINT('Ctrl Pts',(8.50998586672548,6.64522349213896,-9.57520098697005)) ;
#108499=CARTESIAN_POINT('Ctrl Pts',(8.50534188065424,6.64708199603772,-9.58506080025014)) ;
#108500=CARTESIAN_POINT('Ctrl Pts',(8.50212992821339,6.64824261275105,-9.59588754367484)) ;
#108501=CARTESIAN_POINT('Ctrl Pts',(8.50077314609738,6.64911992656046,-9.60682491191675)) ;
#108502=CARTESIAN_POINT('Ctrl Pts',(8.50025986706873,6.64945181977648,-9.61096258566769)) ;
#108503=CARTESIAN_POINT('Ctrl Pts',(8.50000017127792,6.64974165917873,-9.61514325510124)) ;
#108504=CARTESIAN_POINT('Ctrl Pts',(8.5000000000847,6.64999974464544,-9.61931786749562)) ;
#108505=CARTESIAN_POINT('',(8.55242393572493,6.60106172182543,-9.51324209871612)) ;
#108506=CARTESIAN_POINT('Ctrl Pts',(8.55241775170034,6.60106807917178,-9.51323281615444)) ;
#108507=CARTESIAN_POINT('Ctrl Pts',(8.55072388788561,6.6061902674336,-9.51772147695244)) ;
#108508=CARTESIAN_POINT('Ctrl Pts',(8.5485829404857,6.61143812822774,-9.52192692414486)) ;
#108509=CARTESIAN_POINT('Ctrl Pts',(8.54582344182381,6.61635369861669,-9.52606365157295)) ;
#108510=CARTESIAN_POINT('Ctrl Pts',(8.55635360773813,6.58637108369506,-9.49863239073381)) ;
#108511=CARTESIAN_POINT('Ctrl Pts',(8.55606387390184,6.58765239867384,-9.50011238280753)) ;
#108512=CARTESIAN_POINT('Ctrl Pts',(8.55575324501783,6.5889682390236,-9.5015659413336)) ;
#108513=CARTESIAN_POINT('Ctrl Pts',(8.55541196992769,6.59037241127503,-9.50304320494036)) ;
#108514=CARTESIAN_POINT('Ctrl Pts',(8.5552429000838,6.59106804711314,-9.50377505069942)) ;
#108515=CARTESIAN_POINT('Ctrl Pts',(8.5550663125072,6.59178496983021,-9.50451195883767)) ;
#108516=CARTESIAN_POINT('Ctrl Pts',(8.55488049708425,6.59252693597571,-9.50525627761903)) ;
#108517=CARTESIAN_POINT('Ctrl Pts',(8.55445908016384,6.59420966544519,-9.50694434270892)) ;
#108518=CARTESIAN_POINT('Ctrl Pts',(8.55403589309456,6.59584037906531,-9.50848837772247)) ;
#108519=CARTESIAN_POINT('Ctrl Pts',(8.55359592981646,6.59737680581849,-9.50990315623324)) ;
#108520=CARTESIAN_POINT('Ctrl Pts',(8.55324292160433,6.59860957066092,-9.51103831559199)) ;
#108521=CARTESIAN_POINT('Ctrl Pts',(8.55287861047124,6.59978201473818,-9.51209104250713)) ;
#108522=CARTESIAN_POINT('Ctrl Pts',(8.55248933155914,6.60087815532545,-9.51307712698674)) ;
#108523=CARTESIAN_POINT('Ctrl Pts',(8.55246754857564,6.6009394923555,-9.51313230557793)) ;
#108524=CARTESIAN_POINT('Ctrl Pts',(8.55244574956029,6.60100068203153,-9.51318729627853)) ;
#108525=CARTESIAN_POINT('Ctrl Pts',(8.55242393572493,6.60106172182543,-9.51324209871612)) ;
#108526=CARTESIAN_POINT('Ctrl Pts',(8.5,6.66256607592813,-9.61971270883831)) ;
#108527=CARTESIAN_POINT('Ctrl Pts',(8.5,6.66256607592813,-9.535)) ;
#108528=CARTESIAN_POINT('Ctrl Pts',(8.58356010126947,6.66256607592813,-9.52107331645509)) ;
#108529=CARTESIAN_POINT('Ctrl Pts',(8.5,6.61011302719829,-9.61971270726284)) ;
#108530=CARTESIAN_POINT('Ctrl Pts',(8.5,6.63245216822978,-9.53855723659927)) ;
#108531=CARTESIAN_POINT('Ctrl Pts',(8.5794176004298,6.63563981885128,-9.5217637332617)) ;
#108532=CARTESIAN_POINT('Ctrl Pts',(8.5,6.55934573373317,-9.59884690994277)) ;
#108533=CARTESIAN_POINT('Ctrl Pts',(8.5,6.60054351783575,-9.5280813958278)) ;
#108534=CARTESIAN_POINT('Ctrl Pts',(8.57705842698407,6.60987578993432,-9.51172752804771)) ;
#108535=CARTESIAN_POINT('Ctrl Pts',(8.5,6.52274941072028,-9.56225058927972)) ;
#108536=CARTESIAN_POINT('Ctrl Pts',(8.5,6.57873105977929,-9.50626894022071)) ;
#108537=CARTESIAN_POINT('Ctrl Pts',(8.57705842661295,6.59157413088145,-9.49342586911855)) ;
#108538=CARTESIAN_POINT('Origin',(8.49172374697003,1.4,-12.7)) ;
#108539=CARTESIAN_POINT('Origin',(8.49172374697003,1.4,-8.19785831296513)) ;
#108540=CARTESIAN_POINT('Origin',(8.49172374697002,1.4,-8.19785831296513)) ;
#108541=CARTESIAN_POINT('Origin',(8.49172374697003,1.4,-8.19785831296514)) ;
#108542=CARTESIAN_POINT('Ctrl Pts',(8.50816364570057,1.49863939238321,-8.19785831296512)) ;
#108543=CARTESIAN_POINT('Ctrl Pts',(8.51019246767907,1.4983012553868,-8.23292758407099)) ;
#108544=CARTESIAN_POINT('Ctrl Pts',(8.50816364570057,1.47636598119991,-8.26029201095831)) ;
#108545=CARTESIAN_POINT('Ctrl Pts',(8.97755831131126,1.42040694811477,-8.16994865115435)) ;
#108546=CARTESIAN_POINT('Ctrl Pts',(8.9787999739868,1.42020000433582,-8.20456667318447)) ;
#108547=CARTESIAN_POINT('Ctrl Pts',(8.97755831689146,1.39869563385688,-8.23169481695199)) ;
#108548=CARTESIAN_POINT('Ctrl Pts',(9.44698496305968,1.34216917282337,-8.14263137063053)) ;
#108549=CARTESIAN_POINT('Ctrl Pts',(9.44827639615869,1.34195393397321,-8.17677752860714)) ;
#108550=CARTESIAN_POINT('Ctrl Pts',(9.4469849688788,1.32097764915795,-8.20372298471039)) ;
#108551=CARTESIAN_POINT('Ctrl Pts',(9.91643989873053,1.26392668354489,-8.11583811982177)) ;
#108552=CARTESIAN_POINT('Ctrl Pts',(9.91830968165731,1.26361505305709,-8.14950934419701)) ;
#108553=CARTESIAN_POINT('Ctrl Pts',(9.91643989873053,1.24322097942674,-8.17630356419402)) ;
#108554=CARTESIAN_POINT('Origin',(9.9,1.16528729116168,-8.1158381198218)) ;
#108555=CARTESIAN_POINT('Origin',(9.9,1.16528729116168,-8.1158381198218)) ;
#108556=CARTESIAN_POINT('Origin',(-0.4,-3.36847777691809,-10.56)) ;
#108557=CARTESIAN_POINT('Origin',(-0.400000000000001,-3.36847777691809,
-10.56)) ;
#108558=CARTESIAN_POINT('Origin',(-0.4,-3.36847777691809,-10.56)) ;
#108559=CARTESIAN_POINT('Origin',(-0.400000000000001,-3.36847777691809,
-9.66)) ;
#108560=CARTESIAN_POINT('Origin',(-0.4,-3.36847777691809,-9.76)) ;
#108561=CARTESIAN_POINT('Origin',(-1.11032778078669,-3.36847777691809,-10.56)) ;
#108562=CARTESIAN_POINT('Origin',(0.4,-3.36847777691809,-10.56)) ;
#108563=CARTESIAN_POINT('Origin',(-0.400000000000001,-3.36847777691809,
-9.76)) ;
#108564=CARTESIAN_POINT('Origin',(-0.4,-3.36847777691809,-9.76)) ;
#108565=CARTESIAN_POINT('Origin',(0.400000000000001,-3.36847777691809,-10.56)) ;
#108566=CARTESIAN_POINT('Origin',(0.400000000000001,-3.36847777691809,-10.56)) ;
#108567=CARTESIAN_POINT('Origin',(1.5,-3.36847777691809,-9.76)) ;
#108568=CARTESIAN_POINT('Origin',(0.4,-3.36847777691809,-9.76)) ;
#108569=CARTESIAN_POINT('Origin',(0.4,-3.36847777691809,-9.66)) ;
#108570=CARTESIAN_POINT('Origin',(0.4,-3.36847777691809,-9.76)) ;
#108571=CARTESIAN_POINT('Origin',(0.4,-3.36847777691809,-9.76)) ;
#108572=CARTESIAN_POINT('Origin',(7.96847777691809,3.4,-10.56)) ;
#108573=CARTESIAN_POINT('Origin',(7.96847777691809,3.4,-10.56)) ;
#108574=CARTESIAN_POINT('Origin',(7.96847777691809,3.4,-10.56)) ;
#108575=CARTESIAN_POINT('Origin',(7.96847777691809,3.4,-9.66)) ;
#108576=CARTESIAN_POINT('Origin',(7.96847777691809,3.4,-9.76)) ;
#108577=CARTESIAN_POINT('Origin',(7.96847777691809,2.68967221921331,-10.56)) ;
#108578=CARTESIAN_POINT('Origin',(7.96847777691809,4.2,-10.56)) ;
#108579=CARTESIAN_POINT('Origin',(7.96847777691809,3.4,-9.76)) ;
#108580=CARTESIAN_POINT('Origin',(7.96847777691809,3.4,-9.76)) ;
#108581=CARTESIAN_POINT('Origin',(7.96847777691809,4.2,-10.56)) ;
#108582=CARTESIAN_POINT('Origin',(7.96847777691809,4.2,-10.56)) ;
#108583=CARTESIAN_POINT('Origin',(7.96847777691809,2.3,-9.76)) ;
#108584=CARTESIAN_POINT('Origin',(7.96847777691809,4.2,-9.76)) ;
#108585=CARTESIAN_POINT('Origin',(7.96847777691809,4.2,-9.66)) ;
#108586=CARTESIAN_POINT('Origin',(7.96847777691809,4.2,-9.76)) ;
#108587=CARTESIAN_POINT('Origin',(7.96847777691809,4.2,-9.76)) ;
#108588=CARTESIAN_POINT('Origin',(8.49172374697003,1.4,-12.7)) ;
#108589=CARTESIAN_POINT('Origin',(8.49172374697003,1.4,-12.1221416870349)) ;
#108590=CARTESIAN_POINT('Origin',(8.49172374697002,1.4,-12.1221416870349)) ;
#108591=CARTESIAN_POINT('Origin',(8.49172374697003,1.39999999999989,-12.1221416870347)) ;
#108592=CARTESIAN_POINT('Ctrl Pts',(8.50816364570058,1.47636598119991,-12.0597079890417)) ;
#108593=CARTESIAN_POINT('Ctrl Pts',(8.51019246767908,1.4983012553868,-12.087072415929)) ;
#108594=CARTESIAN_POINT('Ctrl Pts',(8.50816364570058,1.49863939238321,-12.1221416870349)) ;
#108595=CARTESIAN_POINT('Ctrl Pts',(8.97755831689155,1.39869563385768,-12.088305183049)) ;
#108596=CARTESIAN_POINT('Ctrl Pts',(8.97879997398666,1.42020000433619,-12.1154333268189)) ;
#108597=CARTESIAN_POINT('Ctrl Pts',(8.97755831131117,1.42040694811478,-12.1500513488473)) ;
#108598=CARTESIAN_POINT('Ctrl Pts',(9.44698496887881,1.32097764915819,-12.1162770152899)) ;
#108599=CARTESIAN_POINT('Ctrl Pts',(9.44827639615871,1.34195393397346,-12.1432224713932)) ;
#108600=CARTESIAN_POINT('Ctrl Pts',(9.44698496305967,1.34216917282337,-12.1773686293698)) ;
#108601=CARTESIAN_POINT('Ctrl Pts',(9.91643989873053,1.24322097942674,-12.143696435806)) ;
#108602=CARTESIAN_POINT('Ctrl Pts',(9.91830968165732,1.26361505305709,-12.170490655803)) ;
#108603=CARTESIAN_POINT('Ctrl Pts',(9.91643989873053,1.26392668354489,-12.2041618801782)) ;
#108604=CARTESIAN_POINT('Origin',(9.9,1.16528729116168,-12.2041618801782)) ;
#108605=CARTESIAN_POINT('Origin',(9.9,1.16528729116168,-12.2041618801782)) ;
#108606=CARTESIAN_POINT('Origin',(8.48377223398316,8.2,-12.7)) ;
#108607=CARTESIAN_POINT('Origin',(8.48238054867516,8.20007133354354,-9.41317893123556)) ;
#108608=CARTESIAN_POINT('Ctrl Pts',(8.40201662970151,8.3,-9.64597597792138)) ;
#108609=CARTESIAN_POINT('Ctrl Pts',(8.50299337454951,8.3,-9.63267481126358)) ;
#108610=CARTESIAN_POINT('Ctrl Pts',(8.50100123624933,8.19773961376461,-9.63268884611774)) ;
#108611=CARTESIAN_POINT('Ctrl Pts',(8.39454129798956,8.3,-9.59449818135068)) ;
#108612=CARTESIAN_POINT('Ctrl Pts',(8.49697875237678,8.3,-9.60537411133466)) ;
#108613=CARTESIAN_POINT('Ctrl Pts',(8.49727262260755,8.20135231978528,-9.60506706396228)) ;
#108614=CARTESIAN_POINT('Ctrl Pts',(8.40820218948348,8.3,-9.54202536352426)) ;
#108615=CARTESIAN_POINT('Ctrl Pts',(8.49818669687004,8.3,-9.58247172780125)) ;
#108616=CARTESIAN_POINT('Ctrl Pts',(8.50412619268403,8.20300739730715,-9.58038841002482)) ;
#108617=CARTESIAN_POINT('Ctrl Pts',(8.4430413476632,8.3,-9.49099693308713)) ;
#108618=CARTESIAN_POINT('Ctrl Pts',(8.50894174387209,8.3,-9.54085505538057)) ;
#108619=CARTESIAN_POINT('Ctrl Pts',(8.52157716465942,8.21896555381603,-9.55016612665033)) ;
#108620=CARTESIAN_POINT('Ctrl Pts',(8.44963266995283,8.3,-9.48266783197822)) ;
#108621=CARTESIAN_POINT('Ctrl Pts',(8.51095981317518,8.3,-9.5337494404835)) ;
#108622=CARTESIAN_POINT('Ctrl Pts',(8.52487915500778,8.22226238914487,-9.54495161805188)) ;
#108623=CARTESIAN_POINT('Ctrl Pts',(8.46372306360152,8.3,-9.46695472631993)) ;
#108624=CARTESIAN_POINT('Ctrl Pts',(8.51547368264944,8.3,-9.51763279105592)) ;
#108625=CARTESIAN_POINT('Ctrl Pts',(8.53193863144478,8.23129792829965,-9.53331747838551)) ;
#108626=CARTESIAN_POINT('Ctrl Pts',(8.47128983770084,8.3,-9.45955862714639)) ;
#108627=CARTESIAN_POINT('Ctrl Pts',(8.51796237042372,8.3,-9.50924649491276)) ;
#108628=CARTESIAN_POINT('Ctrl Pts',(8.53572833262714,8.23677343862357,-9.52742958850775)) ;
#108629=CARTESIAN_POINT('Ctrl Pts',(8.48287565264707,8.3,-9.44873079483315)) ;
#108630=CARTESIAN_POINT('Ctrl Pts',(8.52168214469875,8.3,-9.49074351942998)) ;
#108631=CARTESIAN_POINT('Ctrl Pts',(8.54153766811346,8.25077321967988,-9.51204498710733)) ;
#108632=CARTESIAN_POINT('Ctrl Pts',(8.48680760428678,8.3,-9.445187297402)) ;
#108633=CARTESIAN_POINT('Ctrl Pts',(8.52287759291299,8.3,-9.48414350493172)) ;
#108634=CARTESIAN_POINT('Ctrl Pts',(8.54350322705385,8.25646917637536,-9.50626226660349)) ;
#108635=CARTESIAN_POINT('Ctrl Pts',(8.49230810302881,8.3,-9.4394953499955)) ;
#108636=CARTESIAN_POINT('Ctrl Pts',(8.52426411271138,8.3,-9.46856652463357)) ;
#108637=CARTESIAN_POINT('Ctrl Pts',(8.54627296401924,8.268663848689,-9.48855256936155)) ;
#108638=CARTESIAN_POINT('Ctrl Pts',(8.49410170711668,8.3,-9.437526518934)) ;
#108639=CARTESIAN_POINT('Ctrl Pts',(8.52463604790915,8.3,-9.46240552536514)) ;
#108640=CARTESIAN_POINT('Ctrl Pts',(8.54716490137965,8.27360757863442,-9.48079595948253)) ;
#108641=CARTESIAN_POINT('Ctrl Pts',(8.49698869685299,8.3,-9.43307327880953)) ;
#108642=CARTESIAN_POINT('Ctrl Pts',(8.52523118911551,8.3,-9.4465929344383)) ;
#108643=CARTESIAN_POINT('Ctrl Pts',(8.54862931231184,8.28262305001772,-9.45784134927038)) ;
#108644=CARTESIAN_POINT('Ctrl Pts',(8.4979868777125,8.3,-9.43051652115658)) ;
#108645=CARTESIAN_POINT('Ctrl Pts',(8.52551930315387,8.3,-9.43690627604376)) ;
#108646=CARTESIAN_POINT('Ctrl Pts',(8.54912969489065,8.28574379441723,-9.44238189749318)) ;
#108647=CARTESIAN_POINT('Ctrl Pts',(8.49821791151747,8.3,-9.42257957093737)) ;
#108648=CARTESIAN_POINT('Ctrl Pts',(8.52559423327562,8.3,-9.41218912470487)) ;
#108649=CARTESIAN_POINT('Ctrl Pts',(8.54922875625408,8.28635135062006,-9.40323867004693)) ;
#108650=CARTESIAN_POINT('Ctrl Pts',(8.49537847603513,8.3,-9.41764691084576)) ;
#108651=CARTESIAN_POINT('Ctrl Pts',(8.52439331053439,8.3,-9.40147327498213)) ;
#108652=CARTESIAN_POINT('Ctrl Pts',(8.54781890418529,8.28040548672881,-9.38847179337203)) ;
#108653=CARTESIAN_POINT('Ctrl Pts',(8.48955273785443,8.3,-9.40891140345694)) ;
#108654=CARTESIAN_POINT('Ctrl Pts',(8.52168703568127,8.3,-9.38405258512814)) ;
#108655=CARTESIAN_POINT('Ctrl Pts',(8.54489815533717,8.2719421259912,-9.36616700770703)) ;
#108656=CARTESIAN_POINT('Ctrl Pts',(8.48620077197359,8.3,-9.40482630750476)) ;
#108657=CARTESIAN_POINT('Ctrl Pts',(8.52012703453235,8.3,-9.37710733289327)) ;
#108658=CARTESIAN_POINT('Ctrl Pts',(8.54324008387895,8.26788967346964,-9.35831423563837)) ;
#108659=CARTESIAN_POINT('Ctrl Pts',(8.48280151347419,8.3,-9.40079110964071)) ;
#108660=CARTESIAN_POINT('Ctrl Pts',(8.51858761497412,8.3,-9.3706520257852)) ;
#108661=CARTESIAN_POINT('Ctrl Pts',(8.54152015125555,8.26408224232382,-9.35133822503473)) ;
#108662=CARTESIAN_POINT('Origin',(8.4,8.2,-9.61792711014902)) ;
#108663=CARTESIAN_POINT('Origin',(8.4,8.2,-10.785)) ;
#108664=CARTESIAN_POINT('Origin',(8.4,8.2,-10.702072889851)) ;
#108665=CARTESIAN_POINT('Ctrl Pts',(8.50101530037394,8.19768718256761,-10.6872017745814)) ;
#108666=CARTESIAN_POINT('Ctrl Pts',(8.50305639000874,8.3,-10.6872198113573)) ;
#108667=CARTESIAN_POINT('Ctrl Pts',(8.40204633857704,8.3,-10.6738202021253)) ;
#108668=CARTESIAN_POINT('Ctrl Pts',(8.4972546444163,8.20131038948433,-10.7148679119095)) ;
#108669=CARTESIAN_POINT('Ctrl Pts',(8.49701391805271,8.3,-10.7145609423403)) ;
#108670=CARTESIAN_POINT('Ctrl Pts',(8.39450526457597,8.3,-10.725363291071)) ;
#108671=CARTESIAN_POINT('Ctrl Pts',(8.50410935041312,8.20295267265886,-10.7395792968115)) ;
#108672=CARTESIAN_POINT('Ctrl Pts',(8.49820749521502,8.3,-10.7374643378907)) ;
#108673=CARTESIAN_POINT('Ctrl Pts',(8.40816401923485,8.3,-10.7779187290435)) ;
#108674=CARTESIAN_POINT('Ctrl Pts',(8.52158236570989,8.21893216789647,-10.7698300407758)) ;
#108675=CARTESIAN_POINT('Ctrl Pts',(8.50896456566522,8.3,-10.779127678384)) ;
#108676=CARTESIAN_POINT('Ctrl Pts',(8.4430413476632,8.3,-10.8290030669129)) ;
#108677=CARTESIAN_POINT('Ctrl Pts',(8.5248849650705,8.222229916312,-10.7750437061782)) ;
#108678=CARTESIAN_POINT('Ctrl Pts',(8.51098076140208,8.3,-10.7862331109763)) ;
#108679=CARTESIAN_POINT('Ctrl Pts',(8.44963266995284,8.3,-10.8373321680218)) ;
#108680=CARTESIAN_POINT('Ctrl Pts',(8.53194575580938,8.23126818558571,-10.7866757349666)) ;
#108681=CARTESIAN_POINT('Ctrl Pts',(8.51549074202138,8.3,-10.8023505031351)) ;
#108682=CARTESIAN_POINT('Ctrl Pts',(8.4637230636015,8.3,-10.8530452736801)) ;
#108683=CARTESIAN_POINT('Ctrl Pts',(8.53573618291037,8.23674548871787,-10.7925623770273)) ;
#108684=CARTESIAN_POINT('Ctrl Pts',(8.51797743940284,8.3,-10.8107374625586)) ;
#108685=CARTESIAN_POINT('Ctrl Pts',(8.47128983770083,8.3,-10.8604413728536)) ;
#108686=CARTESIAN_POINT('Ctrl Pts',(8.54154687836689,8.25075037830458,-10.8079451319455)) ;
#108687=CARTESIAN_POINT('Ctrl Pts',(8.52169408444524,8.3,-10.8292435543493)) ;
#108688=CARTESIAN_POINT('Ctrl Pts',(8.48287565264706,8.3,-10.8712692051668)) ;
#108689=CARTESIAN_POINT('Ctrl Pts',(8.54351297666181,8.2564485941942,-10.8137272780162)) ;
#108690=CARTESIAN_POINT('Ctrl Pts',(8.52288848488737,8.3,-10.8358447315488)) ;
#108691=CARTESIAN_POINT('Ctrl Pts',(8.48680760428676,8.3,-10.874812702598)) ;
#108692=CARTESIAN_POINT('Ctrl Pts',(8.54628376412585,8.26864846827403,-10.8314376231601)) ;
#108693=CARTESIAN_POINT('Ctrl Pts',(8.52427341038692,8.3,-10.8514250170404)) ;
#108694=CARTESIAN_POINT('Ctrl Pts',(8.49230810302881,8.3,-10.8805046500045)) ;
#108695=CARTESIAN_POINT('Ctrl Pts',(8.54717611873857,8.27359443500942,-10.8391948837188)) ;
#108696=CARTESIAN_POINT('Ctrl Pts',(8.5246448044482,8.3,-10.8575873399142)) ;
#108697=CARTESIAN_POINT('Ctrl Pts',(8.49410170711667,8.3,-10.882473481066)) ;
#108698=CARTESIAN_POINT('Ctrl Pts',(8.54864126180654,8.28261417405718,-10.8621529061247)) ;
#108699=CARTESIAN_POINT('Ctrl Pts',(8.52523908688554,8.3,-10.8734032849062)) ;
#108700=CARTESIAN_POINT('Ctrl Pts',(8.49698869685298,8.3,-10.8869267211905)) ;
#108701=CARTESIAN_POINT('Ctrl Pts',(8.5491418548716,8.28573645090424,-10.877615282416)) ;
#108702=CARTESIAN_POINT('Ctrl Pts',(8.52552693815803,8.3,-10.8830919520162)) ;
#108703=CARTESIAN_POINT('Ctrl Pts',(8.4979868777125,8.3,-10.8894834788434)) ;
#108704=CARTESIAN_POINT('Ctrl Pts',(8.54924094958848,8.28634430798886,-10.9167659475987)) ;
#108705=CARTESIAN_POINT('Ctrl Pts',(8.52560181204939,8.3,-10.9078137517533)) ;
#108706=CARTESIAN_POINT('Ctrl Pts',(8.49821791151748,8.3,-10.8974204290626)) ;
#108707=CARTESIAN_POINT('Ctrl Pts',(8.54783079466743,8.28039553911294,-10.9315348059812)) ;
#108708=CARTESIAN_POINT('Ctrl Pts',(8.52440147378976,8.3,-10.9185312754322)) ;
#108709=CARTESIAN_POINT('Ctrl Pts',(8.49537847603513,8.3,-10.9023530891542)) ;
#108710=CARTESIAN_POINT('Ctrl Pts',(8.54465883986931,8.27120119512637,-10.9557571947032)) ;
#108711=CARTESIAN_POINT('Ctrl Pts',(8.52145785975947,8.3,-10.93749027833)) ;
#108712=CARTESIAN_POINT('Ctrl Pts',(8.48905244827038,8.3,-10.9118387647145)) ;
#108713=CARTESIAN_POINT('Ctrl Pts',(8.54267599402784,8.26648669506703,-10.9642949904304)) ;
#108714=CARTESIAN_POINT('Ctrl Pts',(8.5195878469242,8.3,-10.9452641321446)) ;
#108715=CARTESIAN_POINT('Ctrl Pts',(8.48503640902804,8.3,-10.9165685970659)) ;
#108716=CARTESIAN_POINT('Ctrl Pts',(8.54064021294345,8.26212437554839,-10.9722000298238)) ;
#108717=CARTESIAN_POINT('Ctrl Pts',(8.51779796763703,8.3,-10.9526895170151)) ;
#108718=CARTESIAN_POINT('Ctrl Pts',(8.48104783026778,8.3,-10.9212848074951)) ;
#108719=CARTESIAN_POINT('Origin',(8.48238054716045,8.20007132581614,-10.9068210673796)) ;
#108720=CARTESIAN_POINT('Origin',(8.48377223398316,8.2,-12.7)) ;
#108721=CARTESIAN_POINT('Ctrl Pts',(8.55305389383868,6.58518362856711,-14.5798163714329)) ;
#108722=CARTESIAN_POINT('Ctrl Pts',(8.56447181517253,6.58947636230805,-14.575523637692)) ;
#108723=CARTESIAN_POINT('Ctrl Pts',(8.57705842661295,6.59157413088145,-14.5734258691185)) ;
#108724=CARTESIAN_POINT('Ctrl Pts',(8.553051025152,6.55898702014118,-14.5536204597775)) ;
#108725=CARTESIAN_POINT('Ctrl Pts',(8.56446969712854,6.56479854221785,-14.5508465230912)) ;
#108726=CARTESIAN_POINT('Ctrl Pts',(8.5770584270977,6.56766897765924,-14.5495207157348)) ;
#108727=CARTESIAN_POINT('Ctrl Pts',(8.55608440539073,6.54967077654144,-14.5134724260347)) ;
#108728=CARTESIAN_POINT('Ctrl Pts',(8.56803673427363,6.55578248257735,-14.5131311242349)) ;
#108729=CARTESIAN_POINT('Ctrl Pts',(8.58110225049763,6.55837193275,-14.5132648466504)) ;
#108730=CARTESIAN_POINT('Ctrl Pts',(8.56106007075016,6.56033186051354,-14.4769784615962)) ;
#108731=CARTESIAN_POINT('Ctrl Pts',(8.57385418571953,6.56560017282096,-14.4782038837617)) ;
#108732=CARTESIAN_POINT('Ctrl Pts',(8.58763814880121,6.56727264871055,-14.4785929056926)) ;
#108733=CARTESIAN_POINT('',(8.56104219912065,6.56017369985344,-14.4776338509444)) ;
#108734=CARTESIAN_POINT('',(8.55704445183395,6.58320973295709,-14.5748316411921)) ;
#108735=CARTESIAN_POINT('Ctrl Pts',(8.56104219912065,6.56017369985344,-14.4776338509444)) ;
#108736=CARTESIAN_POINT('Ctrl Pts',(8.56172006948825,6.55755272988493,-14.4905099834262)) ;
#108737=CARTESIAN_POINT('Ctrl Pts',(8.56178854742204,6.55691761311389,-14.5040188634591)) ;
#108738=CARTESIAN_POINT('Ctrl Pts',(8.56147572200372,6.55855061087387,-14.5170710371545)) ;
#108739=CARTESIAN_POINT('Ctrl Pts',(8.56116227470662,6.56018685493861,-14.5301491578135)) ;
#108740=CARTESIAN_POINT('Ctrl Pts',(8.5604843297899,6.56417103596015,-14.5431290791339)) ;
#108741=CARTESIAN_POINT('Ctrl Pts',(8.55945615587251,6.57017322470283,-14.5548222126965)) ;
#108742=CARTESIAN_POINT('Ctrl Pts',(8.55883284154061,6.5738119576086,-14.5619109917552)) ;
#108743=CARTESIAN_POINT('Ctrl Pts',(8.55807185541709,6.57823677723142,-14.5686350483953)) ;
#108744=CARTESIAN_POINT('Ctrl Pts',(8.55704487707427,6.58320791316496,-14.5748324621195)) ;
#108745=CARTESIAN_POINT('',(8.55635403291171,6.58636921675995,-14.5786302321744)) ;
#108746=CARTESIAN_POINT('Origin',(8.54420290656139,6.62817328946518,-14.541941136554)) ;
#108747=CARTESIAN_POINT('',(8.57705842661295,6.59157413088145,-14.5734258691185)) ;
#108748=CARTESIAN_POINT('Origin',(8.6,6.52274941072028,-14.6422505892797)) ;
#108749=CARTESIAN_POINT('',(8.58355189313842,6.56397635572685,-14.502433776426)) ;
#108750=CARTESIAN_POINT('Origin',(8.59777129281801,6.65641294722147,-14.5008822359315)) ;
#108751=CARTESIAN_POINT('Ctrl Pts',(8.56104311409705,6.56017375480329,-14.4776348093723)) ;
#108752=CARTESIAN_POINT('Ctrl Pts',(8.56569547918964,6.5609490208508,-14.4831223861694)) ;
#108753=CARTESIAN_POINT('Ctrl Pts',(8.57049938306329,6.56176641478978,-14.4885092513474)) ;
#108754=CARTESIAN_POINT('Ctrl Pts',(8.57538893105709,6.56259599225627,-14.4937862661384)) ;
#108755=CARTESIAN_POINT('Ctrl Pts',(8.57808773793831,6.5630538810791,-14.4966989369719)) ;
#108756=CARTESIAN_POINT('Ctrl Pts',(8.58081254036864,6.56351521010419,-14.4995793793676)) ;
#108757=CARTESIAN_POINT('Ctrl Pts',(8.58355195315297,6.56397636517831,-14.5024336197205)) ;
#108758=CARTESIAN_POINT('Ctrl Pts',(8.5,8.35216169217141,-14.5924060982502)) ;
#108759=CARTESIAN_POINT('Ctrl Pts',(8.5,8.2900428850829,-14.561346694706)) ;
#108760=CARTESIAN_POINT('Ctrl Pts',(8.56507848521152,8.26835005667906,-14.550500280504)) ;
#108761=CARTESIAN_POINT('Ctrl Pts',(8.5,8.31945293993511,-14.6578235972685)) ;
#108762=CARTESIAN_POINT('Ctrl Pts',(8.5,8.26922013491168,-14.6029921887963)) ;
#108763=CARTESIAN_POINT('Ctrl Pts',(8.56507848601002,8.25199117628906,-14.5832180406186)) ;
#108764=CARTESIAN_POINT('Ctrl Pts',(8.5,8.24922766844411,-14.6997127068514)) ;
#108765=CARTESIAN_POINT('Ctrl Pts',(8.50000000000007,8.21777561643102,-14.6244773698228)) ;
#108766=CARTESIAN_POINT('Ctrl Pts',(8.57228151929421,8.21451202732351,-14.6029530801176)) ;
#108767=CARTESIAN_POINT('Ctrl Pts',(8.5,8.17221734381475,-14.6997127088383)) ;
#108768=CARTESIAN_POINT('Ctrl Pts',(8.5,8.17221734381475,-14.615)) ;
#108769=CARTESIAN_POINT('Ctrl Pts',(8.58356010126947,8.17221734381475,-14.6010733164551)) ;
#108770=CARTESIAN_POINT('',(8.50000000249538,8.20000280433619,-14.6979047436384)) ;
#108771=CARTESIAN_POINT('',(8.54742025481395,8.27608084305204,-14.5543656619559)) ;
#108772=CARTESIAN_POINT('Ctrl Pts',(8.50000000249538,8.20000280433619,-14.6979047436384)) ;
#108773=CARTESIAN_POINT('Ctrl Pts',(8.50000274011724,8.20154143765779,-14.6856354484511)) ;
#108774=CARTESIAN_POINT('Ctrl Pts',(8.50225788919788,8.20358050335012,-14.6732664749796)) ;
#108775=CARTESIAN_POINT('Ctrl Pts',(8.50614710304112,8.20657022673326,-14.6619159810139)) ;
#108776=CARTESIAN_POINT('Ctrl Pts',(8.51002595055128,8.20955198129041,-14.6505957407205)) ;
#108777=CARTESIAN_POINT('Ctrl Pts',(8.51564213392183,8.21362262975068,-14.6400461335207)) ;
#108778=CARTESIAN_POINT('Ctrl Pts',(8.52129493663065,8.21921832196825,-14.630621792234)) ;
#108779=CARTESIAN_POINT('Ctrl Pts',(8.52933132065201,8.22717351408127,-14.6172235489855)) ;
#108780=CARTESIAN_POINT('Ctrl Pts',(8.53683691159804,8.23885362788864,-14.6056624434434)) ;
#108781=CARTESIAN_POINT('Ctrl Pts',(8.54097226482464,8.25011947738646,-14.5928811696171)) ;
#108782=CARTESIAN_POINT('Ctrl Pts',(8.54447125915462,8.25965170869904,-14.5820667114082)) ;
#108783=CARTESIAN_POINT('Ctrl Pts',(8.54617119150717,8.26873789958222,-14.5699396101896)) ;
#108784=CARTESIAN_POINT('Ctrl Pts',(8.54724932284106,8.27506683274844,-14.5565664602513)) ;
#108785=CARTESIAN_POINT('Ctrl Pts',(8.54730817192851,8.27541229338911,-14.5558364956863)) ;
#108786=CARTESIAN_POINT('Ctrl Pts',(8.5473651061662,8.27575037116516,-14.555102832606)) ;
#108787=CARTESIAN_POINT('Ctrl Pts',(8.54742024083733,8.27608084608571,-14.5543656752073)) ;
#108788=CARTESIAN_POINT('',(8.56507848521152,8.26835005667905,-14.550500280504)) ;
#108789=CARTESIAN_POINT('Origin',(8.6,8.3521616921714,-14.5924060982502)) ;
#108790=CARTESIAN_POINT('',(8.58356010126947,8.17221734381475,-14.6010733164551)) ;
#108791=CARTESIAN_POINT('Origin',(8.59670327708558,8.16883734299686,-14.5070689695193)) ;
#108792=CARTESIAN_POINT('',(8.5,8.17221734381475,-14.6997127088383)) ;
#108793=CARTESIAN_POINT('Origin',(8.6,8.17221734381475,-14.6997127088383)) ;
#108794=CARTESIAN_POINT('Origin',(8.5,8.1664264877529,-14.4771077523706)) ;
#108795=CARTESIAN_POINT('Origin',(2.9,3.8,-15.24)) ;
#108796=CARTESIAN_POINT('',(3.,2.4,-15.24)) ;
#108797=CARTESIAN_POINT('Origin',(3.,3.8,-15.24)) ;
#108798=CARTESIAN_POINT('',(2.9,2.3,-15.24)) ;
#108799=CARTESIAN_POINT('Origin',(2.9,2.4,-15.24)) ;
#108800=CARTESIAN_POINT('Origin',(2.9,3.8,-15.24)) ;
#108801=CARTESIAN_POINT('Origin',(1.35,3.8,-15.24)) ;
#108802=CARTESIAN_POINT('',(1.35,2.3,-15.24)) ;
#108803=CARTESIAN_POINT('Origin',(1.35,3.8,-15.24)) ;
#108804=CARTESIAN_POINT('',(1.25,2.2,-15.24)) ;
#108805=CARTESIAN_POINT('Origin',(1.35,2.2,-15.24)) ;
#108806=CARTESIAN_POINT('Origin',(1.25,3.8,-15.24)) ;
#108807=CARTESIAN_POINT('Origin',(13.9153543900904,1.02736587339764,-14.39)) ;
#108808=CARTESIAN_POINT('',(1.15,1.02736587339764,-14.49)) ;
#108809=CARTESIAN_POINT('',(1.15,0.931757800066529,-14.3606896551724)) ;
#108810=CARTESIAN_POINT('Origin',(1.15,1.02736587339764,-14.39)) ;
#108811=CARTESIAN_POINT('',(-0.900000000000002,1.02736587339765,-14.49)) ;
#108812=CARTESIAN_POINT('',(-1.,1.02736587339765,-14.49)) ;
#108813=CARTESIAN_POINT('',(-0.900000000000002,0.982644513847654,-14.4794427191)) ;
#108814=CARTESIAN_POINT('Origin',(-0.900000000000002,1.02736587339765,-14.39)) ;
#108815=CARTESIAN_POINT('',(-0.900000000000002,0.93175780006653,-14.3606896551724)) ;
#108816=CARTESIAN_POINT('Origin',(-0.900000000000002,1.02736587339765,-14.39)) ;
#108817=CARTESIAN_POINT('',(13.9153543900904,0.931757800066525,-14.3606896551724)) ;
#108818=CARTESIAN_POINT('Origin',(13.9153543900904,1.02736587339764,-16.09)) ;
#108819=CARTESIAN_POINT('',(1.15,0.93175780006653,-16.1193103448276)) ;
#108820=CARTESIAN_POINT('',(1.15,1.02736587339765,-15.99)) ;
#108821=CARTESIAN_POINT('Origin',(1.15,1.02736587339765,-16.09)) ;
#108822=CARTESIAN_POINT('',(-0.900000000000002,0.931757800066531,-16.1193103448276)) ;
#108823=CARTESIAN_POINT('',(13.9153543900904,0.931757800066525,-16.1193103448276)) ;
#108824=CARTESIAN_POINT('',(-0.900000000000002,1.02736587339765,-15.99)) ;
#108825=CARTESIAN_POINT('Origin',(-0.900000000000002,1.02736587339765,-16.09)) ;
#108826=CARTESIAN_POINT('',(-1.,1.02736587339765,-15.99)) ;
#108827=CARTESIAN_POINT('Origin',(8.49172374697003,3.8,-15.24)) ;
#108828=CARTESIAN_POINT('',(8.49172374697003,1.47741935483871,-13.3411532060953)) ;
#108829=CARTESIAN_POINT('',(8.49172374697003,1.47741935483871,-17.1388467939047)) ;
#108830=CARTESIAN_POINT('Origin',(8.49172374697003,3.8,-15.24)) ;
#108831=CARTESIAN_POINT('',(8.50816364570057,1.47636598119991,-13.3402920109583)) ;
#108832=CARTESIAN_POINT('Origin',(8.49172374697003,1.4,-13.2778583129651)) ;
#108833=CARTESIAN_POINT('',(8.50816364570057,1.47636598119991,-17.1397079890417)) ;
#108834=CARTESIAN_POINT('Origin',(8.50816364570057,3.8,-15.24)) ;
#108835=CARTESIAN_POINT('Origin',(8.49172374697003,1.4,-17.2021416870349)) ;
#108836=CARTESIAN_POINT('Origin',(1.25,3.8,-15.24)) ;
#108837=CARTESIAN_POINT('',(1.25,2.3,-15.24)) ;
#108838=CARTESIAN_POINT('Origin',(13.9153543900904,3.8,-15.24)) ;
#108839=CARTESIAN_POINT('',(-0.900000000000002,1.47741935483872,-17.1388467939047)) ;
#108840=CARTESIAN_POINT('',(13.9153543900904,1.47741935483871,-17.1388467939047)) ;
#108841=CARTESIAN_POINT('Origin',(-0.900000000000001,3.8,-15.24)) ;
#108842=CARTESIAN_POINT('',(1.35,0.876327704607742,-15.9124137931035)) ;
#108843=CARTESIAN_POINT('Ctrl Pts',(1.35,0.876327704607742,-15.9124137931035)) ;
#108844=CARTESIAN_POINT('Ctrl Pts',(1.35,0.888571289407569,-15.9656492115953)) ;
#108845=CARTESIAN_POINT('Ctrl Pts',(1.32969623836296,0.902340613578954,
-16.0179295970213)) ;
#108846=CARTESIAN_POINT('Ctrl Pts',(1.25741074236298,0.924142973728496,
-16.0950150537158)) ;
#108847=CARTESIAN_POINT('Ctrl Pts',(1.20472523187106,0.93175780006653,-16.1193103448276)) ;
#108848=CARTESIAN_POINT('Ctrl Pts',(1.15,0.93175780006653,-16.1193103448276)) ;
#108849=CARTESIAN_POINT('',(1.35,0.876327704607742,-14.5675862068966)) ;
#108850=CARTESIAN_POINT('Origin',(1.35,3.8,-15.24)) ;
#108851=CARTESIAN_POINT('Ctrl Pts',(1.15,0.931757800066529,-14.3606896551724)) ;
#108852=CARTESIAN_POINT('Ctrl Pts',(1.20475877631964,0.931757800066529,
-14.3606896551724)) ;
#108853=CARTESIAN_POINT('Ctrl Pts',(1.2574100247738,0.924155896380522,-14.3849343608884)) ;
#108854=CARTESIAN_POINT('Ctrl Pts',(1.32987646938161,0.9022735155524,-14.4623125455279)) ;
#108855=CARTESIAN_POINT('Ctrl Pts',(1.35,0.888577265820266,-14.5143248028101)) ;
#108856=CARTESIAN_POINT('Ctrl Pts',(1.35,0.876327704607742,-14.5675862068966)) ;
#108857=CARTESIAN_POINT('',(-0.900000000000002,1.47741935483872,-13.3411532060953)) ;
#108858=CARTESIAN_POINT('Origin',(-0.900000000000001,3.8,-15.24)) ;
#108859=CARTESIAN_POINT('',(13.9153543900904,1.47741935483871,-13.3411532060953)) ;
#108860=CARTESIAN_POINT('Origin',(0.55,3.09772049281573E-17,-15.24)) ;
#108861=CARTESIAN_POINT('',(0.549999999999999,4.4,-14.79)) ;
#108862=CARTESIAN_POINT('',(0.549999999999999,4.4,-15.69)) ;
#108863=CARTESIAN_POINT('',(0.549999999999999,4.4,-15.24)) ;
#108864=CARTESIAN_POINT('',(0.55,4.04473197180486,-15.69)) ;
#108865=CARTESIAN_POINT('',(0.55,1.39397422176708E-16,-15.69)) ;
#108866=CARTESIAN_POINT('',(0.55,4.05997159067981,-15.64)) ;
#108867=CARTESIAN_POINT('Ctrl Pts',(0.549999999999999,4.04473197180486,
-15.69)) ;
#108868=CARTESIAN_POINT('Ctrl Pts',(0.549999999999999,4.04764757798806,
-15.6855648611277)) ;
#108869=CARTESIAN_POINT('Ctrl Pts',(0.549999999999999,4.05014503921306,
-15.6809481448659)) ;
#108870=CARTESIAN_POINT('Ctrl Pts',(0.549999999999999,4.0569489863933,-15.6656814456903)) ;
#108871=CARTESIAN_POINT('Ctrl Pts',(0.549999999999999,4.0599715906798,-15.6518214564414)) ;
#108872=CARTESIAN_POINT('Ctrl Pts',(0.549999999999999,4.0599715906798,-15.64)) ;
#108873=CARTESIAN_POINT('',(0.55,4.05997159067981,-14.84)) ;
#108874=CARTESIAN_POINT('',(0.55,4.05997159067981,-14.74)) ;
#108875=CARTESIAN_POINT('',(0.55,4.04473197181449,-14.7900000000146)) ;
#108876=CARTESIAN_POINT('Origin',(0.55003450380264,3.938694577917,-14.8424160296945)) ;
#108877=CARTESIAN_POINT('',(0.55,6.35032701027224E-17,-14.79)) ;
#108878=CARTESIAN_POINT('Origin',(10.,7.8,-17.78)) ;
#108879=CARTESIAN_POINT('',(9.93162277660169,7.82279240779944,-17.78)) ;
#108880=CARTESIAN_POINT('',(8.51539501058484,8.29486832980505,-17.78)) ;
#108881=CARTESIAN_POINT('',(10.,7.8,-17.78)) ;
#108882=CARTESIAN_POINT('',(8.51540095511711,8.29487265903615,-16.0090607599342)) ;
#108883=CARTESIAN_POINT('',(8.51539501058484,8.29486832980505,-17.78)) ;
#108884=CARTESIAN_POINT('',(8.54856023413467,8.2839858620311,-15.9960080665656)) ;
#108885=CARTESIAN_POINT('Ctrl Pts',(8.51540095511711,8.29487265903615,-16.0090607599342)) ;
#108886=CARTESIAN_POINT('Ctrl Pts',(8.51716444659958,8.29428466923189,-16.0096424828188)) ;
#108887=CARTESIAN_POINT('Ctrl Pts',(8.51901954868166,8.29366521079575,-16.0099704508582)) ;
#108888=CARTESIAN_POINT('Ctrl Pts',(8.52087614409667,8.2930450194617,-16.0100725025784)) ;
#108889=CARTESIAN_POINT('Ctrl Pts',(8.52171779595218,8.29276386763785,-16.0101187657647)) ;
#108890=CARTESIAN_POINT('Ctrl Pts',(8.52256005861364,8.29248252453828,-16.010119087778)) ;
#108891=CARTESIAN_POINT('Ctrl Pts',(8.52339613191994,8.29220315552769,-16.0100794460141)) ;
#108892=CARTESIAN_POINT('Ctrl Pts',(8.52456316579569,8.29181319797645,-16.0100241120128)) ;
#108893=CARTESIAN_POINT('Ctrl Pts',(8.52573147766846,8.29142195356397,-16.0098930049957)) ;
#108894=CARTESIAN_POINT('Ctrl Pts',(8.52689074379087,8.29103442649366,-16.009691327086)) ;
#108895=CARTESIAN_POINT('Ctrl Pts',(8.52858695132689,8.2904674071317,-16.0093962373015)) ;
#108896=CARTESIAN_POINT('Ctrl Pts',(8.53026630212624,8.2899212363328,-16.0089439218143)) ;
#108897=CARTESIAN_POINT('Ctrl Pts',(8.53190117913116,8.28939883282069,-16.0083683729162)) ;
#108898=CARTESIAN_POINT('Ctrl Pts',(8.53241671440274,8.28923410028383,-16.0081868817357)) ;
#108899=CARTESIAN_POINT('Ctrl Pts',(8.53292790037786,8.28907155799428,-16.0079933975174)) ;
#108900=CARTESIAN_POINT('Ctrl Pts',(8.53343404910735,8.28891083250768,-16.0077898379553)) ;
#108901=CARTESIAN_POINT('Ctrl Pts',(8.53529681408172,8.28831931900685,-16.0070406834076)) ;
#108902=CARTESIAN_POINT('Ctrl Pts',(8.53711612169876,8.28774836357888,-16.0061310088335)) ;
#108903=CARTESIAN_POINT('Ctrl Pts',(8.53885192161986,8.28720494689874,-16.005061264748)) ;
#108904=CARTESIAN_POINT('Ctrl Pts',(8.54015925159111,8.28679566878771,-16.0042555794339)) ;
#108905=CARTESIAN_POINT('Ctrl Pts',(8.54141951580282,8.28640152775899,-16.0033597461918)) ;
#108906=CARTESIAN_POINT('Ctrl Pts',(8.54261761299016,8.2860217121528,-16.0023927107854)) ;
#108907=CARTESIAN_POINT('Ctrl Pts',(8.54427390694792,8.28549664098141,-16.0010558451977)) ;
#108908=CARTESIAN_POINT('Ctrl Pts',(8.54582756795265,8.2849959222079,-15.9995574336961)) ;
#108909=CARTESIAN_POINT('Ctrl Pts',(8.54719190273363,8.28456181678108,-15.9979139760521)) ;
#108910=CARTESIAN_POINT('Ctrl Pts',(8.547685057547,8.2844049042815,-15.9973199290052)) ;
#108911=CARTESIAN_POINT('Ctrl Pts',(8.54815358395157,8.28425671205375,-15.9967074323075)) ;
#108912=CARTESIAN_POINT('Ctrl Pts',(8.54859369700691,8.28411936587097,-15.9960788545618)) ;
#108913=CARTESIAN_POINT('',(8.56837597005345,8.27720399148459,-15.9725054212675)) ;
#108914=CARTESIAN_POINT('Ctrl Pts',(8.5485198670553,8.28382649282421,-15.9960140527758)) ;
#108915=CARTESIAN_POINT('Ctrl Pts',(8.55267891820632,8.28243778061538,-15.9905631273053)) ;
#108916=CARTESIAN_POINT('Ctrl Pts',(8.55701747195682,8.28096933708255,-15.9852590577816)) ;
#108917=CARTESIAN_POINT('Ctrl Pts',(8.56150853123443,8.27945301063656,-15.9801132102135)) ;
#108918=CARTESIAN_POINT('Ctrl Pts',(8.56331520072586,8.27884302075229,-15.9780431315898)) ;
#108919=CARTESIAN_POINT('Ctrl Pts',(8.5651466343553,8.27822544298233,-15.9759980022295)) ;
#108920=CARTESIAN_POINT('Ctrl Pts',(8.56700126712394,8.27760232477898,-15.9739757856585)) ;
#108921=CARTESIAN_POINT('Ctrl Pts',(8.56745273479656,8.27745064099026,-15.9734835235653)) ;
#108922=CARTESIAN_POINT('Ctrl Pts',(8.56790562999349,8.27729861980367,-15.9729951953627)) ;
#108923=CARTESIAN_POINT('Ctrl Pts',(8.56835731300612,8.27714712982918,-15.9725055965825)) ;
#108924=CARTESIAN_POINT('',(9.93162277660169,7.82279240779944,-16.1997127088383)) ;
#108925=CARTESIAN_POINT('',(9.98593528106273,7.80468823964576,-16.2087647929151)) ;
#108926=CARTESIAN_POINT('',(9.93162277660169,7.82279240779944,-17.78)) ;
#108927=CARTESIAN_POINT('Origin',(10.,6.8,-17.78)) ;
#108928=CARTESIAN_POINT('',(10.,6.8847127088383,-17.78)) ;
#108929=CARTESIAN_POINT('',(10.,7.72792407799439,-17.78)) ;
#108930=CARTESIAN_POINT('',(10.,6.8,-17.78)) ;
#108931=CARTESIAN_POINT('',(10.,7.72792407799439,-16.1997127088383)) ;
#108932=CARTESIAN_POINT('',(10.,7.72792407799439,-17.78)) ;
#108933=CARTESIAN_POINT('',(10.,6.8847127088383,-16.1997127088383)) ;
#108934=CARTESIAN_POINT('',(10.,6.8,-16.1997127088383)) ;
#108935=CARTESIAN_POINT('',(10.,6.8847127088383,-17.78)) ;
#108936=CARTESIAN_POINT('Origin',(8.5,6.55,-17.78)) ;
#108937=CARTESIAN_POINT('',(9.91643989873054,6.78607331645509,-16.1997127088383)) ;
#108938=CARTESIAN_POINT('',(8.58355805979355,6.56393854759965,-15.9775665415707)) ;
#108939=CARTESIAN_POINT('',(8.48442535909739,6.54740422651623,-15.9610436188994)) ;
#108940=CARTESIAN_POINT('',(8.56107669735261,6.5600938800009,-16.0023838472224)) ;
#108941=CARTESIAN_POINT('Ctrl Pts',(8.58354728038624,6.56400494118525,-15.9775667486351)) ;
#108942=CARTESIAN_POINT('Ctrl Pts',(8.57838853885689,6.56313097816976,-15.9829365696478)) ;
#108943=CARTESIAN_POINT('Ctrl Pts',(8.5733012794654,6.56225500583436,-15.9883881686568)) ;
#108944=CARTESIAN_POINT('Ctrl Pts',(8.56834297134786,6.5614089984296,-15.9939607837898)) ;
#108945=CARTESIAN_POINT('Ctrl Pts',(8.56587587079858,6.56098805134775,-15.9967335444835)) ;
#108946=CARTESIAN_POINT('Ctrl Pts',(8.56344049907307,6.56057499921402,-15.9995353033204)) ;
#108947=CARTESIAN_POINT('Ctrl Pts',(8.56104288133097,6.56017406260212,-16.0023650362459)) ;
#108948=CARTESIAN_POINT('',(8.50816305748499,6.55136011924236,-16.0173726221053)) ;
#108949=CARTESIAN_POINT('Ctrl Pts',(8.56125813732196,6.56020968955366,-16.0025506353537)) ;
#108950=CARTESIAN_POINT('Ctrl Pts',(8.55737139916531,6.55956189986088,-16.007208599473)) ;
#108951=CARTESIAN_POINT('Ctrl Pts',(8.5530633519033,6.55884389198388,-16.0099674660867)) ;
#108952=CARTESIAN_POINT('Ctrl Pts',(8.54121332232538,6.55686888705423,-16.0165237407849)) ;
#108953=CARTESIAN_POINT('Ctrl Pts',(8.53496267038054,6.55582711173009,-16.0179613606699)) ;
#108954=CARTESIAN_POINT('Ctrl Pts',(8.52888665185221,6.55481444197537,-16.0192795539313)) ;
#108955=CARTESIAN_POINT('Ctrl Pts',(8.52471102104758,6.55411850350793,-16.0195977494013)) ;
#108956=CARTESIAN_POINT('Ctrl Pts',(8.52011475164549,6.55335245860758,-16.0197029599352)) ;
#108957=CARTESIAN_POINT('Ctrl Pts',(8.51754797133905,6.55292466188984,-16.019718645943)) ;
#108958=CARTESIAN_POINT('Ctrl Pts',(8.51248317870103,6.55208052978351,-16.0189638228623)) ;
#108959=CARTESIAN_POINT('Ctrl Pts',(8.51021540604925,6.55170256767487,-16.0183708961116)) ;
#108960=CARTESIAN_POINT('Ctrl Pts',(8.50816120922221,6.55136020153704,-16.0173764115261)) ;
#108961=CARTESIAN_POINT('',(8.50816364570071,6.55136060761679,-17.78)) ;
#108962=CARTESIAN_POINT('',(8.50816364570071,6.55136060761679,-17.78)) ;
#108963=CARTESIAN_POINT('',(9.91643989873054,6.78607331645509,-17.78)) ;
#108964=CARTESIAN_POINT('',(8.5,6.55,-17.78)) ;
#108965=CARTESIAN_POINT('',(9.91643989873054,6.78607331645509,-17.78)) ;
#108966=CARTESIAN_POINT('Origin',(10.,1.5,-17.78)) ;
#108967=CARTESIAN_POINT('',(-0.900000000000002,1.5,-17.2021416870349)) ;
#108968=CARTESIAN_POINT('',(8.49172374697003,1.5,-17.2021416870349)) ;
#108969=CARTESIAN_POINT('',(10.,1.5,-17.2021416870349)) ;
#108970=CARTESIAN_POINT('',(8.49172374697003,1.5,-17.78)) ;
#108971=CARTESIAN_POINT('',(8.49172374697003,1.5,-17.78)) ;
#108972=CARTESIAN_POINT('',(-0.900000000000001,1.5,-17.78)) ;
#108973=CARTESIAN_POINT('',(10.,1.5,-17.78)) ;
#108974=CARTESIAN_POINT('',(-0.900000000000002,1.5,-17.1661360284258)) ;
#108975=CARTESIAN_POINT('Origin',(10.,1.5,-17.78)) ;
#108976=CARTESIAN_POINT('',(8.49172374697003,1.5,-12.7)) ;
#108977=CARTESIAN_POINT('',(-0.900000000000001,1.5,-12.7)) ;
#108978=CARTESIAN_POINT('',(10.,1.5,-12.7)) ;
#108979=CARTESIAN_POINT('',(8.49172374697003,1.5,-13.2778583129651)) ;
#108980=CARTESIAN_POINT('',(8.49172374697003,1.5,-17.78)) ;
#108981=CARTESIAN_POINT('',(-0.900000000000002,1.5,-13.2778583129651)) ;
#108982=CARTESIAN_POINT('',(10.,1.5,-13.2778583129651)) ;
#108983=CARTESIAN_POINT('',(-0.900000000000001,1.5,-17.78)) ;
#108984=CARTESIAN_POINT('Origin',(10.,0.,-17.78)) ;
#108985=CARTESIAN_POINT('',(10.,0.1,-12.7)) ;
#108986=CARTESIAN_POINT('',(10.,1.16528729116168,-12.7)) ;
#108987=CARTESIAN_POINT('',(10.,0.,-12.7)) ;
#108988=CARTESIAN_POINT('',(10.,0.1,-17.78)) ;
#108989=CARTESIAN_POINT('',(10.,0.1,-17.78)) ;
#108990=CARTESIAN_POINT('',(10.,1.16528729116168,-17.78)) ;
#108991=CARTESIAN_POINT('',(10.,0.,-17.78)) ;
#108992=CARTESIAN_POINT('',(10.,1.16528729116168,-17.2841618801782)) ;
#108993=CARTESIAN_POINT('',(10.,1.16528729116168,-17.78)) ;
#108994=CARTESIAN_POINT('',(10.,1.16528729116168,-13.1958381198218)) ;
#108995=CARTESIAN_POINT('Origin',(10.,3.8,-15.24)) ;
#108996=CARTESIAN_POINT('',(10.,1.16528729116168,-17.78)) ;
#108997=CARTESIAN_POINT('Origin',(0.,0.,-17.78)) ;
#108998=CARTESIAN_POINT('',(8.48377223398316,8.3,-17.78)) ;
#108999=CARTESIAN_POINT('',(7.1,8.3,-17.78)) ;
#109000=CARTESIAN_POINT('',(8.5,8.3,-17.78)) ;
#109001=CARTESIAN_POINT('Origin',(8.48377223398316,8.2,-17.78)) ;
#109002=CARTESIAN_POINT('Origin',(9.9,7.72792407799439,-17.78)) ;
#109003=CARTESIAN_POINT('Origin',(9.9,6.8847127088383,-17.78)) ;
#109004=CARTESIAN_POINT('',(8.49172374697018,6.55,-17.78)) ;
#109005=CARTESIAN_POINT('Origin',(8.49172374697018,6.65,-17.78)) ;
#109006=CARTESIAN_POINT('',(-0.900000000000001,6.55,-17.78)) ;
#109007=CARTESIAN_POINT('',(1.25,6.55,-17.78)) ;
#109008=CARTESIAN_POINT('',(-1.,6.45,-17.78)) ;
#109009=CARTESIAN_POINT('Origin',(-0.9,6.45,-17.78)) ;
#109010=CARTESIAN_POINT('',(-1.,4.65,-17.78)) ;
#109011=CARTESIAN_POINT('',(-1.,3.46944695195362E-16,-17.78)) ;
#109012=CARTESIAN_POINT('',(-0.900000000000001,4.55,-17.78)) ;
#109013=CARTESIAN_POINT('Origin',(-0.900000000000001,4.65,-17.78)) ;
#109014=CARTESIAN_POINT('',(1.15,4.55,-17.78)) ;
#109015=CARTESIAN_POINT('',(1.57859836313889E-15,4.55,-17.78)) ;
#109016=CARTESIAN_POINT('',(1.25,4.45,-17.78)) ;
#109017=CARTESIAN_POINT('Origin',(1.15,4.45,-17.78)) ;
#109018=CARTESIAN_POINT('',(1.25,3.15,-17.78)) ;
#109019=CARTESIAN_POINT('',(1.25,1.5,-17.78)) ;
#109020=CARTESIAN_POINT('',(1.15,3.05,-17.78)) ;
#109021=CARTESIAN_POINT('Origin',(1.15,3.15,-17.78)) ;
#109022=CARTESIAN_POINT('',(-0.900000000000002,3.05,-17.78)) ;
#109023=CARTESIAN_POINT('',(1.05818132034585E-15,3.05,-17.78)) ;
#109024=CARTESIAN_POINT('',(-1.,2.95,-17.78)) ;
#109025=CARTESIAN_POINT('Origin',(-0.900000000000002,2.95,-17.78)) ;
#109026=CARTESIAN_POINT('',(-1.,1.6,-17.78)) ;
#109027=CARTESIAN_POINT('',(-1.,3.46944695195362E-16,-17.78)) ;
#109028=CARTESIAN_POINT('Origin',(-0.900000000000002,1.6,-17.78)) ;
#109029=CARTESIAN_POINT('',(8.50816364570057,1.49863939238321,-17.78)) ;
#109030=CARTESIAN_POINT('Origin',(8.49172374697003,1.4,-17.78)) ;
#109031=CARTESIAN_POINT('',(9.91643989873054,1.26392668354489,-17.78)) ;
#109032=CARTESIAN_POINT('',(10.,1.24999999999998,-17.78)) ;
#109033=CARTESIAN_POINT('Origin',(9.9,1.16528729116168,-17.78)) ;
#109034=CARTESIAN_POINT('',(9.9,0.,-17.78)) ;
#109035=CARTESIAN_POINT('Origin',(9.9,0.1,-17.78)) ;
#109036=CARTESIAN_POINT('',(-2.,0.,-17.78)) ;
#109037=CARTESIAN_POINT('',(-2.,0.,-17.78)) ;
#109038=CARTESIAN_POINT('',(-2.,7.55,-17.78)) ;
#109039=CARTESIAN_POINT('',(-2.,7.65,-17.78)) ;
#109040=CARTESIAN_POINT('',(-1.9,7.65,-17.78)) ;
#109041=CARTESIAN_POINT('Origin',(-1.9,7.55,-17.78)) ;
#109042=CARTESIAN_POINT('',(6.9,7.65,-17.78)) ;
#109043=CARTESIAN_POINT('',(7.,7.65,-17.78)) ;
#109044=CARTESIAN_POINT('',(7.,7.75,-17.78)) ;
#109045=CARTESIAN_POINT('Origin',(6.9,7.75,-17.78)) ;
#109046=CARTESIAN_POINT('',(7.,8.2,-17.78)) ;
#109047=CARTESIAN_POINT('',(7.,8.3,-17.78)) ;
#109048=CARTESIAN_POINT('Origin',(7.1,8.2,-17.78)) ;
#109049=CARTESIAN_POINT('Origin',(0.,0.,-12.7)) ;
#109050=CARTESIAN_POINT('',(9.93162277660169,7.82279240779944,-12.7)) ;
#109051=CARTESIAN_POINT('',(8.51539501058484,8.29486832980505,-12.7)) ;
#109052=CARTESIAN_POINT('',(10.,7.8,-12.7)) ;
#109053=CARTESIAN_POINT('',(8.48377223398316,8.3,-12.7)) ;
#109054=CARTESIAN_POINT('Origin',(8.48377223398316,8.2,-12.7)) ;
#109055=CARTESIAN_POINT('',(7.1,8.3,-12.7)) ;
#109056=CARTESIAN_POINT('',(8.5,8.3,-12.7)) ;
#109057=CARTESIAN_POINT('',(7.,8.2,-12.7)) ;
#109058=CARTESIAN_POINT('Origin',(7.1,8.2,-12.7)) ;
#109059=CARTESIAN_POINT('',(7.,7.75,-12.7)) ;
#109060=CARTESIAN_POINT('',(7.,8.3,-12.7)) ;
#109061=CARTESIAN_POINT('',(6.9,7.65,-12.7)) ;
#109062=CARTESIAN_POINT('Origin',(6.9,7.75,-12.7)) ;
#109063=CARTESIAN_POINT('',(-1.9,7.65,-12.7)) ;
#109064=CARTESIAN_POINT('',(7.,7.65,-12.7)) ;
#109065=CARTESIAN_POINT('',(-2.,7.55,-12.7)) ;
#109066=CARTESIAN_POINT('Origin',(-1.9,7.55,-12.7)) ;
#109067=CARTESIAN_POINT('',(-2.,0.,-12.7)) ;
#109068=CARTESIAN_POINT('',(-2.,7.65,-12.7)) ;
#109069=CARTESIAN_POINT('',(9.9,0.,-12.7)) ;
#109070=CARTESIAN_POINT('',(-2.,0.,-12.7)) ;
#109071=CARTESIAN_POINT('Origin',(9.9,0.1,-12.7)) ;
#109072=CARTESIAN_POINT('',(9.91643989873054,1.26392668354489,-12.7)) ;
#109073=CARTESIAN_POINT('Origin',(9.9,1.16528729116168,-12.7)) ;
#109074=CARTESIAN_POINT('',(8.50816364570057,1.49863939238321,-12.7)) ;
#109075=CARTESIAN_POINT('',(0.472972972972955,2.83783783783779,-12.7)) ;
#109076=CARTESIAN_POINT('Origin',(8.49172374697003,1.4,-12.7)) ;
#109077=CARTESIAN_POINT('',(-1.,1.6,-12.7)) ;
#109078=CARTESIAN_POINT('Origin',(-0.900000000000002,1.6,-12.7)) ;
#109079=CARTESIAN_POINT('',(-1.,2.95,-12.7)) ;
#109080=CARTESIAN_POINT('',(-1.,3.46944695195362E-16,-12.7)) ;
#109081=CARTESIAN_POINT('',(-0.900000000000002,3.05,-12.7)) ;
#109082=CARTESIAN_POINT('Origin',(-0.900000000000002,2.95,-12.7)) ;
#109083=CARTESIAN_POINT('',(1.15,3.05,-12.7)) ;
#109084=CARTESIAN_POINT('',(1.05818132034585E-15,3.05,-12.7)) ;
#109085=CARTESIAN_POINT('',(1.25,3.15,-12.7)) ;
#109086=CARTESIAN_POINT('Origin',(1.15,3.15,-12.7)) ;
#109087=CARTESIAN_POINT('',(1.25,4.45,-12.7)) ;
#109088=CARTESIAN_POINT('',(1.25,5.3,-12.7)) ;
#109089=CARTESIAN_POINT('',(1.15,4.55,-12.7)) ;
#109090=CARTESIAN_POINT('Origin',(1.15,4.45,-12.7)) ;
#109091=CARTESIAN_POINT('',(-0.900000000000001,4.55,-12.7)) ;
#109092=CARTESIAN_POINT('',(1.57859836313889E-15,4.55,-12.7)) ;
#109093=CARTESIAN_POINT('',(-1.,4.65,-12.7)) ;
#109094=CARTESIAN_POINT('Origin',(-0.900000000000001,4.65,-12.7)) ;
#109095=CARTESIAN_POINT('',(-1.,6.45,-12.7)) ;
#109096=CARTESIAN_POINT('',(-1.,3.46944695195362E-16,-12.7)) ;
#109097=CARTESIAN_POINT('',(-0.900000000000001,6.55,-12.7)) ;
#109098=CARTESIAN_POINT('Origin',(-0.9,6.45,-12.7)) ;
#109099=CARTESIAN_POINT('',(8.49172374697018,6.55,-12.7)) ;
#109100=CARTESIAN_POINT('',(1.25,6.55,-12.7)) ;
#109101=CARTESIAN_POINT('',(8.50816364570071,6.55136060761679,-12.7)) ;
#109102=CARTESIAN_POINT('Origin',(8.49172374697018,6.65,-12.7)) ;
#109103=CARTESIAN_POINT('',(9.91643989873054,6.78607331645509,-12.7)) ;
#109104=CARTESIAN_POINT('',(8.5,6.55,-12.7)) ;
#109105=CARTESIAN_POINT('',(10.,6.8847127088383,-12.7)) ;
#109106=CARTESIAN_POINT('Origin',(9.9,6.8847127088383,-12.7)) ;
#109107=CARTESIAN_POINT('',(10.,7.72792407799439,-12.7)) ;
#109108=CARTESIAN_POINT('',(10.,6.8,-12.7)) ;
#109109=CARTESIAN_POINT('Origin',(9.9,7.72792407799439,-12.7)) ;
#109110=CARTESIAN_POINT('Origin',(7.,7.65,-17.78)) ;
#109111=CARTESIAN_POINT('',(-1.9,7.65,-17.78)) ;
#109112=CARTESIAN_POINT('',(6.9,7.65,-17.78)) ;
#109113=CARTESIAN_POINT('Origin',(7.,8.3,-17.78)) ;
#109114=CARTESIAN_POINT('',(7.,7.75,-12.7)) ;
#109115=CARTESIAN_POINT('',(7.,8.2,-17.78)) ;
#109116=CARTESIAN_POINT('Origin',(8.5,8.3,-17.78)) ;
#109117=CARTESIAN_POINT('',(8.4,8.3,-15.782072889851)) ;
#109118=CARTESIAN_POINT('',(8.48377267093845,8.29999999999968,-15.9980525450042)) ;
#109119=CARTESIAN_POINT('Ctrl Pts',(8.4,8.3,-15.782072889851)) ;
#109120=CARTESIAN_POINT('Ctrl Pts',(8.40000007660113,8.3,-15.7992296501961)) ;
#109121=CARTESIAN_POINT('Ctrl Pts',(8.40222537906653,8.3,-15.8161962391188)) ;
#109122=CARTESIAN_POINT('Ctrl Pts',(8.40642689896248,8.3,-15.8326162565066)) ;
#109123=CARTESIAN_POINT('Ctrl Pts',(8.41084238024591,8.3,-15.84987245932)) ;
#109124=CARTESIAN_POINT('Ctrl Pts',(8.41744096861416,8.3,-15.866526744374)) ;
#109125=CARTESIAN_POINT('Ctrl Pts',(8.42598957610855,8.3,-15.8821622007355)) ;
#109126=CARTESIAN_POINT('Ctrl Pts',(8.42927578126156,8.3,-15.8881726904321)) ;
#109127=CARTESIAN_POINT('Ctrl Pts',(8.43285067318742,8.3,-15.8940324469635)) ;
#109128=CARTESIAN_POINT('Ctrl Pts',(8.43670279785319,8.3,-15.8997167867855)) ;
#109129=CARTESIAN_POINT('Ctrl Pts',(8.43684245837179,8.3,-15.8999228750916)) ;
#109130=CARTESIAN_POINT('Ctrl Pts',(8.43698247939112,8.3,-15.9001287268225)) ;
#109131=CARTESIAN_POINT('Ctrl Pts',(8.43712286024714,8.3,-15.9003343406941)) ;
#109132=CARTESIAN_POINT('Ctrl Pts',(8.44304092798571,8.3,-15.9090024515356)) ;
#109133=CARTESIAN_POINT('Ctrl Pts',(8.44963232699549,8.300000000002,-15.9173317313645)) ;
#109134=CARTESIAN_POINT('Ctrl Pts',(8.45667836512367,8.29999999999776,-15.9251882739642)) ;
#109135=CARTESIAN_POINT('Ctrl Pts',(8.46347186896914,8.29999999999367,-15.9327632333091)) ;
#109136=CARTESIAN_POINT('Ctrl Pts',(8.47075094334181,8.29999999998296,-15.9399098655154)) ;
#109137=CARTESIAN_POINT('Ctrl Pts',(8.47818849074308,8.29999999991001,-15.9468816128285)) ;
#109138=CARTESIAN_POINT('Ctrl Pts',(8.47846436286148,8.2999999999073,-15.9471402075771)) ;
#109139=CARTESIAN_POINT('Ctrl Pts',(8.47874045306876,8.29999999990447,-15.9473985605991)) ;
#109140=CARTESIAN_POINT('Ctrl Pts',(8.47901674447045,8.29999999990152,-15.9476566852)) ;
#109141=CARTESIAN_POINT('Ctrl Pts',(8.48287938578322,8.29999999986032,-15.9512653488833)) ;
#109142=CARTESIAN_POINT('Ctrl Pts',(8.48681205529409,8.29999999978803,-15.9548079367278)) ;
#109143=CARTESIAN_POINT('Ctrl Pts',(8.49047938959116,8.29999999977836,-15.9586027060218)) ;
#109144=CARTESIAN_POINT('Ctrl Pts',(8.49231307405274,8.29999999977353,-15.9605001085834)) ;
#109145=CARTESIAN_POINT('Ctrl Pts',(8.49410676862313,8.29999999978935,-15.962469327125)) ;
#109146=CARTESIAN_POINT('Ctrl Pts',(8.49555027122445,8.29999999981726,-15.9646968070099)) ;
#109147=CARTESIAN_POINT('Ctrl Pts',(8.49675259850851,8.2999999998405,-15.9665521274215)) ;
#109148=CARTESIAN_POINT('Ctrl Pts',(8.49764594203227,8.29999999986456,-15.9686368157432)) ;
#109149=CARTESIAN_POINT('Ctrl Pts',(8.49795530287013,8.29999999987615,-15.9708110374494)) ;
#109150=CARTESIAN_POINT('Ctrl Pts',(8.49801735255452,8.29999999987847,-15.9712471293982)) ;
#109151=CARTESIAN_POINT('Ctrl Pts',(8.49805590844334,8.29999999988033,-15.971686822978)) ;
#109152=CARTESIAN_POINT('Ctrl Pts',(8.49806875158486,8.29999999988168,-15.9721289896614)) ;
#109153=CARTESIAN_POINT('Ctrl Pts',(8.49822249685462,8.2999999998978,-15.9774221678068)) ;
#109154=CARTESIAN_POINT('Ctrl Pts',(8.49538250015675,8.29999999989889,-15.9823553442684)) ;
#109155=CARTESIAN_POINT('Ctrl Pts',(8.49246863081132,8.29999999993393,-15.986722860551)) ;
#109156=CARTESIAN_POINT('Ctrl Pts',(8.48983292606215,8.29999999996562,-15.9906734437939)) ;
#109157=CARTESIAN_POINT('Ctrl Pts',(8.48683766317129,8.3,-15.9943922110698)) ;
#109158=CARTESIAN_POINT('Ctrl Pts',(8.48377316486175,8.3,-15.9980519562975)) ;
#109159=CARTESIAN_POINT('',(8.48377223398316,8.3,-17.78)) ;
#109160=CARTESIAN_POINT('',(7.1,8.3,-17.78)) ;
#109161=CARTESIAN_POINT('',(8.48377267093845,8.29999999999968,-14.4819474549958)) ;
#109162=CARTESIAN_POINT('',(8.48377223398316,8.3,-17.78)) ;
#109163=CARTESIAN_POINT('',(8.4,8.3,-14.697927110149)) ;
#109164=CARTESIAN_POINT('Ctrl Pts',(8.48377316486179,8.3,-14.4819480437025)) ;
#109165=CARTESIAN_POINT('Ctrl Pts',(8.48683766317135,8.3,-14.4856077889302)) ;
#109166=CARTESIAN_POINT('Ctrl Pts',(8.48983292606214,8.29999999996562,-14.4893265562061)) ;
#109167=CARTESIAN_POINT('Ctrl Pts',(8.49246863081131,8.29999999993393,-14.493277139449)) ;
#109168=CARTESIAN_POINT('Ctrl Pts',(8.49538250015675,8.29999999989889,-14.4976446557316)) ;
#109169=CARTESIAN_POINT('Ctrl Pts',(8.49822249685463,8.2999999998978,-14.5025778321932)) ;
#109170=CARTESIAN_POINT('Ctrl Pts',(8.49806875158486,8.29999999988168,-14.5078710103386)) ;
#109171=CARTESIAN_POINT('Ctrl Pts',(8.49805590844334,8.29999999988033,-14.508313177022)) ;
#109172=CARTESIAN_POINT('Ctrl Pts',(8.49801735255452,8.29999999987847,-14.5087528706018)) ;
#109173=CARTESIAN_POINT('Ctrl Pts',(8.49795530287013,8.29999999987615,-14.5091889625506)) ;
#109174=CARTESIAN_POINT('Ctrl Pts',(8.49764594190815,8.29999999986456,-14.5113631851291)) ;
#109175=CARTESIAN_POINT('Ctrl Pts',(8.49675259754384,8.2999999998405,-14.5134478740673)) ;
#109176=CARTESIAN_POINT('Ctrl Pts',(8.49555027122431,8.29999999981726,-14.51530319299)) ;
#109177=CARTESIAN_POINT('Ctrl Pts',(8.4941067657021,8.29999999978935,-14.5175306773816)) ;
#109178=CARTESIAN_POINT('Ctrl Pts',(8.49231306928119,8.29999999977353,-14.519499896352)) ;
#109179=CARTESIAN_POINT('Ctrl Pts',(8.49047938958767,8.29999999977836,-14.5213972939748)) ;
#109180=CARTESIAN_POINT('Ctrl Pts',(8.48681202348066,8.29999999978803,-14.5251920961739)) ;
#109181=CARTESIAN_POINT('Ctrl Pts',(8.48287934332708,8.29999999986032,-14.5287346907302)) ;
#109182=CARTESIAN_POINT('Ctrl Pts',(8.47901674443308,8.29999999990152,-14.53234331476)) ;
#109183=CARTESIAN_POINT('Ctrl Pts',(8.47874052296043,8.29999999990447,-14.5326013740281)) ;
#109184=CARTESIAN_POINT('Ctrl Pts',(8.47846450284309,8.2999999999073,-14.5328596613565)) ;
#109185=CARTESIAN_POINT('Ctrl Pts',(8.47818870097126,8.29999999991001,-14.5331181900299)) ;
#109186=CARTESIAN_POINT('Ctrl Pts',(8.47075185325581,8.29999999998296,-14.540089275328)) ;
#109187=CARTESIAN_POINT('Ctrl Pts',(8.46347271757076,8.29999999998104,-14.547236821007)) ;
#109188=CARTESIAN_POINT('Ctrl Pts',(8.45667934899942,8.29999999998018,-14.5548126083154)) ;
#109189=CARTESIAN_POINT('Ctrl Pts',(8.44963335392745,8.2999999999793,-14.5626701181032)) ;
#109190=CARTESIAN_POINT('Ctrl Pts',(8.44304226791565,8.29999999996634,-14.571000256345)) ;
#109191=CARTESIAN_POINT('Ctrl Pts',(8.43712466127421,8.29999999997622,-14.579666888942)) ;
#109192=CARTESIAN_POINT('Ctrl Pts',(8.43698358608697,8.29999999997646,-14.5798735006502)) ;
#109193=CARTESIAN_POINT('Ctrl Pts',(8.43684287437574,8.29999999997671,-14.5800803512793)) ;
#109194=CARTESIAN_POINT('Ctrl Pts',(8.43670252680326,8.29999999997696,-14.5802874394955)) ;
#109195=CARTESIAN_POINT('Ctrl Pts',(8.42665365624143,8.29999999999548,-14.5951149327151)) ;
#109196=CARTESIAN_POINT('Ctrl Pts',(8.41848789916211,8.29999999999779,-14.611134863194)) ;
#109197=CARTESIAN_POINT('Ctrl Pts',(8.4124226058228,8.29999999999911,-14.6279180514005)) ;
#109198=CARTESIAN_POINT('Ctrl Pts',(8.40662497274065,8.30000000000037,-14.6439606006601)) ;
#109199=CARTESIAN_POINT('Ctrl Pts',(8.4027459894583,8.3,-14.660702193922)) ;
#109200=CARTESIAN_POINT('Ctrl Pts',(8.40101973895655,8.3,-14.6777797883442)) ;
#109201=CARTESIAN_POINT('Ctrl Pts',(8.40034533497793,8.3,-14.6844515880696)) ;
#109202=CARTESIAN_POINT('Ctrl Pts',(8.40000003014814,8.3,-14.6911746730409)) ;
#109203=CARTESIAN_POINT('Ctrl Pts',(8.4,8.3,-14.697927110149)) ;
#109204=CARTESIAN_POINT('',(8.4,8.3,-15.8236545563009)) ;
#109205=CARTESIAN_POINT('Origin',(10.,7.8,-17.78)) ;
#109206=CARTESIAN_POINT('',(8.56837722373804,8.27720759208727,-14.5074948832495)) ;
#109207=CARTESIAN_POINT('',(8.54843785958925,8.28385404680358,-14.4839803122607)) ;
#109208=CARTESIAN_POINT('Ctrl Pts',(8.56837722339832,8.27720759220056,-14.5074948833623)) ;
#109209=CARTESIAN_POINT('Ctrl Pts',(8.56792584473107,8.27735805175631,-14.5070046902277)) ;
#109210=CARTESIAN_POINT('Ctrl Pts',(8.56747319573485,8.27750893475505,-14.5065157932638)) ;
#109211=CARTESIAN_POINT('Ctrl Pts',(8.56702308739659,8.2776589708678,-14.5060243039587)) ;
#109212=CARTESIAN_POINT('Ctrl Pts',(8.56055949575605,8.27981350141465,-14.4989664783343)) ;
#109213=CARTESIAN_POINT('Ctrl Pts',(8.5543545977397,8.28188180075344,-14.4916283954692)) ;
#109214=CARTESIAN_POINT('Ctrl Pts',(8.54852002808959,8.28382665730347,-14.4839858663514)) ;
#109215=CARTESIAN_POINT('',(8.51539953939799,8.29486682020067,-14.4709403301229)) ;
#109216=CARTESIAN_POINT('Origin',(8.52916905055884,8.29027698314705,-14.490734470481)) ;
#109217=CARTESIAN_POINT('',(8.51539501058484,8.29486832980505,-17.78)) ;
#109218=CARTESIAN_POINT('',(9.93162277660169,7.82279240779944,-14.2802872911617)) ;
#109219=CARTESIAN_POINT('',(9.93162277660169,7.82279240779944,-17.78)) ;
#109220=CARTESIAN_POINT('',(8.48593528106273,8.30468823964576,-14.5212352070849)) ;
#109221=CARTESIAN_POINT('Origin',(10.,6.8,-17.78)) ;
#109222=CARTESIAN_POINT('',(10.,6.8847127088383,-14.2802872911617)) ;
#109223=CARTESIAN_POINT('',(10.,7.72792407799439,-14.2802872911617)) ;
#109224=CARTESIAN_POINT('',(10.,7.8,-14.2802872911617)) ;
#109225=CARTESIAN_POINT('',(10.,7.72792407799439,-17.78)) ;
#109226=CARTESIAN_POINT('',(10.,6.8847127088383,-17.78)) ;
#109227=CARTESIAN_POINT('Origin',(8.5,6.55,-17.78)) ;
#109228=CARTESIAN_POINT('',(8.50816305748851,6.55136011924293,-14.4626273778919)) ;
#109229=CARTESIAN_POINT('Ctrl Pts',(8.50816120922618,6.5513602015377,-14.462623588472)) ;
#109230=CARTESIAN_POINT('Ctrl Pts',(8.50982330775197,6.55163721795866,-14.4618189278179)) ;
#109231=CARTESIAN_POINT('Ctrl Pts',(8.51162127657709,6.55193687942951,-14.4612790284411)) ;
#109232=CARTESIAN_POINT('Ctrl Pts',(8.51523682141417,6.5525394702357,-14.4605710923352)) ;
#109233=CARTESIAN_POINT('Ctrl Pts',(8.51710259142354,6.55285043190392,-14.4603934679393)) ;
#109234=CARTESIAN_POINT('Ctrl Pts',(8.52217030373185,6.55369505062198,-14.4602356911265)) ;
#109235=CARTESIAN_POINT('Ctrl Pts',(8.52587381749838,6.5543123029164,-14.4604838833944)) ;
#109236=CARTESIAN_POINT('Ctrl Pts',(8.5348242152787,6.55580403587979,-14.4617298501839)) ;
#109237=CARTESIAN_POINT('Ctrl Pts',(8.53952102462535,6.5565868367346,-14.4632204474233)) ;
#109238=CARTESIAN_POINT('Ctrl Pts',(8.54640674065696,6.5577344560732,-14.4663682122454)) ;
#109239=CARTESIAN_POINT('Ctrl Pts',(8.55013419152133,6.55835569858689,-14.4682367302301)) ;
#109240=CARTESIAN_POINT('Ctrl Pts',(8.55581906875145,6.55930317812524,-14.4720433754295)) ;
#109241=CARTESIAN_POINT('Ctrl Pts',(8.55861150732132,6.55976858455355,-14.4742775555629)) ;
#109242=CARTESIAN_POINT('Ctrl Pts',(8.56125821409731,6.56020970234955,-14.4774494566561)) ;
#109243=CARTESIAN_POINT('',(9.91643989873054,6.78607331645509,-14.2802872911617)) ;
#109244=CARTESIAN_POINT('',(9.98442535909739,6.79740422651623,-14.2689563811006)) ;
#109245=CARTESIAN_POINT('',(9.91643989873054,6.78607331645509,-17.78)) ;
#109246=CARTESIAN_POINT('',(8.50816364570071,6.55136060761679,-17.78)) ;
#109247=CARTESIAN_POINT('Origin',(1.25,6.55,-17.78)) ;
#109248=CARTESIAN_POINT('',(8.49172372711481,6.55000000000007,-16.0094558427306)) ;
#109249=CARTESIAN_POINT('',(8.49172374697018,6.55,-17.78)) ;
#109250=CARTESIAN_POINT('',(8.4,6.55,-15.7806780018997)) ;
#109251=CARTESIAN_POINT('Ctrl Pts',(8.49172374697018,6.55000000000104,-16.0094557456557)) ;
#109252=CARTESIAN_POINT('Ctrl Pts',(8.49606803673629,6.55000000001052,-16.0059505863269)) ;
#109253=CARTESIAN_POINT('Ctrl Pts',(8.50046735944504,6.54999999990301,-16.0025119042493)) ;
#109254=CARTESIAN_POINT('Ctrl Pts',(8.50920280475194,6.55000000136501,-15.995516026702)) ;
#109255=CARTESIAN_POINT('Ctrl Pts',(8.51365366733368,6.55000000372466,-15.9920189182923)) ;
#109256=CARTESIAN_POINT('Ctrl Pts',(8.51786969589109,6.55000000840872,-15.9875740514917)) ;
#109257=CARTESIAN_POINT('Ctrl Pts',(8.5182483557534,6.5500000088438,-15.9871628343557)) ;
#109258=CARTESIAN_POINT('Ctrl Pts',(8.51893753951069,6.55000000964298,-15.9863894122641)) ;
#109259=CARTESIAN_POINT('Ctrl Pts',(8.51925555226624,6.55000001000021,-15.9860246830609)) ;
#109260=CARTESIAN_POINT('Ctrl Pts',(8.52125362518915,6.55000001218547,-15.9836369664008)) ;
#109261=CARTESIAN_POINT('Ctrl Pts',(8.52280131776514,6.55000000862054,-15.9813625215737)) ;
#109262=CARTESIAN_POINT('Ctrl Pts',(8.52354796988915,6.55000000490364,-15.9762172682012)) ;
#109263=CARTESIAN_POINT('Ctrl Pts',(8.52233587755862,6.5500000056078,-15.9735629178234)) ;
#109264=CARTESIAN_POINT('Ctrl Pts',(8.52032554216563,6.55000000470579,-15.9711610105706)) ;
#109265=CARTESIAN_POINT('Ctrl Pts',(8.52004618744964,6.55000000456892,-15.9708554672246)) ;
#109266=CARTESIAN_POINT('Ctrl Pts',(8.51943244221705,6.55000000425259,-15.9702375575506)) ;
#109267=CARTESIAN_POINT('Ctrl Pts',(8.51910103101854,6.55000000405877,-15.9699172773213)) ;
#109268=CARTESIAN_POINT('Ctrl Pts',(8.51460799223803,6.55000000141241,-15.9657349310042)) ;
#109269=CARTESIAN_POINT('Ctrl Pts',(8.50969722522558,6.55000000036127,-15.962960241153)) ;
#109270=CARTESIAN_POINT('Ctrl Pts',(8.50463600502757,6.55000000021577,-15.9596634748388)) ;
#109271=CARTESIAN_POINT('Ctrl Pts',(8.50427412871943,6.55000000020764,-15.9594272801265)) ;
#109272=CARTESIAN_POINT('Ctrl Pts',(8.49410349041848,6.55000000002643,-15.9527743312814)) ;
#109273=CARTESIAN_POINT('Ctrl Pts',(8.48448997361521,6.54999999999179,-15.9460809389623)) ;
#109274=CARTESIAN_POINT('Ctrl Pts',(8.46629237463075,6.55000000001684,-15.9309770243887)) ;
#109275=CARTESIAN_POINT('Ctrl Pts',(8.45766562693769,6.55000000000151,-15.9225939316618)) ;
#109276=CARTESIAN_POINT('Ctrl Pts',(8.44955830666689,6.54999999999999,-15.9132123342681)) ;
#109277=CARTESIAN_POINT('Ctrl Pts',(8.44937081015215,6.54999999999999,-15.9129944283117)) ;
#109278=CARTESIAN_POINT('Ctrl Pts',(8.43720071044432,6.5500000000026,-15.8987892740219)) ;
#109279=CARTESIAN_POINT('Ctrl Pts',(8.42721384365784,6.55000000009148,-15.8832566681901)) ;
#109280=CARTESIAN_POINT('Ctrl Pts',(8.41184903642351,6.55000000007035,-15.8505950553188)) ;
#109281=CARTESIAN_POINT('Ctrl Pts',(8.40635547808308,6.5500000000232,-15.8335173325289)) ;
#109282=CARTESIAN_POINT('Ctrl Pts',(8.40108598764573,6.5499999999995,-15.8043588087541)) ;
#109283=CARTESIAN_POINT('Ctrl Pts',(8.4,6.55,-15.7925595279378)) ;
#109284=CARTESIAN_POINT('Ctrl Pts',(8.4,6.55,-15.7806780018997)) ;
#109285=CARTESIAN_POINT('',(8.4,6.55,-14.6993219981003)) ;
#109286=CARTESIAN_POINT('',(8.4,6.55,-14.5163606076168)) ;
#109287=CARTESIAN_POINT('',(8.4917237271148,6.5500000000004,-14.4705441572684)) ;
#109288=CARTESIAN_POINT('Ctrl Pts',(8.4,6.55,-14.6993219981003)) ;
#109289=CARTESIAN_POINT('Ctrl Pts',(8.4,6.55,-14.6814603515949)) ;
#109290=CARTESIAN_POINT('Ctrl Pts',(8.40245177849651,6.55000000000111,-14.6637850580908)) ;
#109291=CARTESIAN_POINT('Ctrl Pts',(8.40709634751497,6.55000000003438,-14.6467518487573)) ;
#109292=CARTESIAN_POINT('Ctrl Pts',(8.41193897064573,6.55000000006908,-14.6289923078436)) ;
#109293=CARTESIAN_POINT('Ctrl Pts',(8.41916594308082,6.55000000013771,-14.6119288881443)) ;
#109294=CARTESIAN_POINT('Ctrl Pts',(8.42853896333557,6.55000000013582,-14.5960812673187)) ;
#109295=CARTESIAN_POINT('Ctrl Pts',(8.43455058705845,6.55000000013461,-14.5859169946812)) ;
#109296=CARTESIAN_POINT('Ctrl Pts',(8.44144611055244,6.55000000009672,-14.5762530007228)) ;
#109297=CARTESIAN_POINT('Ctrl Pts',(8.44917210140206,6.55000000005186,-14.5672326831017)) ;
#109298=CARTESIAN_POINT('Ctrl Pts',(8.44936219523639,6.55000000005076,-14.5670107430558)) ;
#109299=CARTESIAN_POINT('Ctrl Pts',(8.44955278293315,6.55000000004969,-14.5667892022863)) ;
#109300=CARTESIAN_POINT('Ctrl Pts',(8.44974386351696,6.55000000004865,-14.5665680630168)) ;
#109301=CARTESIAN_POINT('Ctrl Pts',(8.45766118910685,6.55000000000559,-14.5574052712634)) ;
#109302=CARTESIAN_POINT('Ctrl Pts',(8.46628870646478,6.54999999999864,-14.5490215515033)) ;
#109303=CARTESIAN_POINT('Ctrl Pts',(8.47555348469884,6.55000000000007,-14.5413352759491)) ;
#109304=CARTESIAN_POINT('Ctrl Pts',(8.48448851770303,6.55000000000144,-14.5339225647086)) ;
#109305=CARTESIAN_POINT('Ctrl Pts',(8.49410273695376,6.5500000000304,-14.5272346929705)) ;
#109306=CARTESIAN_POINT('Ctrl Pts',(8.50391213313781,6.55000000016212,-14.5208238957712)) ;
#109307=CARTESIAN_POINT('Ctrl Pts',(8.50409415224108,6.55000000016456,-14.5207049396667)) ;
#109308=CARTESIAN_POINT('Ctrl Pts',(8.50427622716234,6.55000000016576,-14.5205860597931)) ;
#109309=CARTESIAN_POINT('Ctrl Pts',(8.50445835579895,6.55000000016577,-14.520467254632)) ;
#109310=CARTESIAN_POINT('Ctrl Pts',(8.50464048443556,6.55000000016577,-14.5203484494708)) ;
#109311=CARTESIAN_POINT('Ctrl Pts',(8.50482266678753,6.55000000016459,-14.5202297190221)) ;
#109312=CARTESIAN_POINT('Ctrl Pts',(8.50500490075221,6.55000000016234,-14.5201110617675)) ;
#109313=CARTESIAN_POINT('Ctrl Pts',(8.50970297364421,6.55000000010443,-14.5170520248173)) ;
#109314=CARTESIAN_POINT('Ctrl Pts',(8.51460443926437,6.55000000028677,-14.5142756540706)) ;
#109315=CARTESIAN_POINT('Ctrl Pts',(8.5187483092633,6.55000000038295,-14.5104369847284)) ;
#109316=CARTESIAN_POINT('Ctrl Pts',(8.51909542442957,6.55000000039101,-14.5101154349821)) ;
#109317=CARTESIAN_POINT('Ctrl Pts',(8.51943721516332,6.55000000039358,-14.5097864145015)) ;
#109318=CARTESIAN_POINT('Ctrl Pts',(8.51977310187181,6.55000000039099,-14.5094491161473)) ;
#109319=CARTESIAN_POINT('Ctrl Pts',(8.52085916897635,6.55000000038261,-14.5083584845811)) ;
#109320=CARTESIAN_POINT('Ctrl Pts',(8.52182399801738,6.55000000033868,-14.507044620882)) ;
#109321=CARTESIAN_POINT('Ctrl Pts',(8.5224633406346,6.55000000029842,-14.5056267666597)) ;
#109322=CARTESIAN_POINT('Ctrl Pts',(8.52278301194321,6.55000000027829,-14.5049178395485)) ;
#109323=CARTESIAN_POINT('Ctrl Pts',(8.52302131164586,6.55000000025926,-14.5041829148066)) ;
#109324=CARTESIAN_POINT('Ctrl Pts',(8.52315270869753,6.55000000024662,-14.503436897635)) ;
#109325=CARTESIAN_POINT('Ctrl Pts',(8.52328410574919,6.55000000023398,-14.5026908804635)) ;
#109326=CARTESIAN_POINT('Ctrl Pts',(8.52330860014986,6.55000000022778,-14.5019337708624)) ;
#109327=CARTESIAN_POINT('Ctrl Pts',(8.52320066085451,6.55000000023233,-14.5011804740329)) ;
#109328=CARTESIAN_POINT('Ctrl Pts',(8.52284031330749,6.55000000024754,-14.4986656469369)) ;
#109329=CARTESIAN_POINT('Ctrl Pts',(8.52133564423351,6.55000000029586,-14.4964067380131)) ;
#109330=CARTESIAN_POINT('Ctrl Pts',(8.5196587899188,6.55000000031744,-14.4943986514954)) ;
#109331=CARTESIAN_POINT('Ctrl Pts',(8.51932554032813,6.55000000032173,-14.4939995744831)) ;
#109332=CARTESIAN_POINT('Ctrl Pts',(8.51898545723479,6.55000000032523,-14.4936103757649)) ;
#109333=CARTESIAN_POINT('Ctrl Pts',(8.51864615038492,6.5500000003277,-14.4932310123194)) ;
#109334=CARTESIAN_POINT('Ctrl Pts',(8.51455081658662,6.55000000035749,-14.4886522072033)) ;
#109335=CARTESIAN_POINT('Ctrl Pts',(8.50963987409779,6.55000000028079,-14.4848202086187)) ;
#109336=CARTESIAN_POINT('Ctrl Pts',(8.5048217738226,6.55000000018959,-14.4809688701254)) ;
#109337=CARTESIAN_POINT('Ctrl Pts',(8.5004640292375,6.5500000001071,-14.4774855160012)) ;
#109338=CARTESIAN_POINT('Ctrl Pts',(8.49606692679175,6.55000000001227,-14.4740490105462)) ;
#109339=CARTESIAN_POINT('Ctrl Pts',(8.49172374697017,6.55000000000105,-14.4705442543438)) ;
#109340=CARTESIAN_POINT('',(8.49172374697018,6.55,-17.78)) ;
#109341=CARTESIAN_POINT('',(-0.9,6.55,-14.39)) ;
#109342=CARTESIAN_POINT('',(-0.900000000000001,6.55,-17.78)) ;
#109343=CARTESIAN_POINT('',(1.15,6.55,-14.39)) ;
#109344=CARTESIAN_POINT('',(1.25,6.55,-14.39)) ;
#109345=CARTESIAN_POINT('',(1.35,6.55,-14.59)) ;
#109346=CARTESIAN_POINT('Origin',(1.15,6.55,-14.59)) ;
#109347=CARTESIAN_POINT('',(1.35,6.55,-15.89)) ;
#109348=CARTESIAN_POINT('',(1.35,6.55,-15.99)) ;
#109349=CARTESIAN_POINT('',(1.15,6.55,-16.09)) ;
#109350=CARTESIAN_POINT('Origin',(1.15,6.55,-15.89)) ;
#109351=CARTESIAN_POINT('',(-0.9,6.55,-16.09)) ;
#109352=CARTESIAN_POINT('',(1.25,6.55,-16.09)) ;
#109353=CARTESIAN_POINT('',(-0.9,6.55,-17.78)) ;
#109354=CARTESIAN_POINT('Origin',(1.25,5.3,-17.78)) ;
#109355=CARTESIAN_POINT('',(1.25,3.15,-16.8831676725155)) ;
#109356=CARTESIAN_POINT('',(1.25,3.04189189189189,-16.7055279241354)) ;
#109357=CARTESIAN_POINT('Origin',(1.25,2.95,-16.8831676725155)) ;
#109358=CARTESIAN_POINT('',(1.25,3.15,-17.78)) ;
#109359=CARTESIAN_POINT('',(1.25,4.45,-16.8831676725155)) ;
#109360=CARTESIAN_POINT('',(1.25,4.45,-16.8211388300842)) ;
#109361=CARTESIAN_POINT('',(1.25,4.55810810810811,-16.7055279241354)) ;
#109362=CARTESIAN_POINT('Origin',(1.25,4.65,-16.8831676725155)) ;
#109363=CARTESIAN_POINT('',(1.25,5.26552792413544,-15.9981081081081)) ;
#109364=CARTESIAN_POINT('Origin',(1.25,3.8,-15.24)) ;
#109365=CARTESIAN_POINT('',(1.25,5.4431676725155,-15.89)) ;
#109366=CARTESIAN_POINT('Origin',(1.25,5.4431676725155,-16.09)) ;
#109367=CARTESIAN_POINT('',(1.25,6.45,-15.89)) ;
#109368=CARTESIAN_POINT('',(1.25,6.55,-15.89)) ;
#109369=CARTESIAN_POINT('',(1.25,6.45,-14.59)) ;
#109370=CARTESIAN_POINT('',(1.25,6.45,-14.49)) ;
#109371=CARTESIAN_POINT('',(1.25,5.4431676725155,-14.59)) ;
#109372=CARTESIAN_POINT('',(1.25,5.38113883008419,-14.59)) ;
#109373=CARTESIAN_POINT('',(1.25,5.26552792413544,-14.4818918918919)) ;
#109374=CARTESIAN_POINT('Origin',(1.25,5.4431676725155,-14.39)) ;
#109375=CARTESIAN_POINT('',(1.25,4.55810810810811,-13.7744720758646)) ;
#109376=CARTESIAN_POINT('Origin',(1.25,3.8,-15.24)) ;
#109377=CARTESIAN_POINT('',(1.25,4.45,-13.5968323274845)) ;
#109378=CARTESIAN_POINT('Origin',(1.25,4.65,-13.5968323274845)) ;
#109379=CARTESIAN_POINT('',(1.25,4.45,-12.7)) ;
#109380=CARTESIAN_POINT('',(1.25,3.15,-13.5968323274845)) ;
#109381=CARTESIAN_POINT('',(1.25,3.15,-13.6588611699158)) ;
#109382=CARTESIAN_POINT('',(1.25,3.04189189189189,-13.7744720758646)) ;
#109383=CARTESIAN_POINT('Origin',(1.25,2.95,-13.5968323274845)) ;
#109384=CARTESIAN_POINT('',(1.25,2.33447207586456,-14.4818918918919)) ;
#109385=CARTESIAN_POINT('Origin',(1.25,3.8,-15.24)) ;
#109386=CARTESIAN_POINT('',(1.25,2.1568323274845,-14.59)) ;
#109387=CARTESIAN_POINT('Origin',(1.25,2.1568323274845,-14.39)) ;
#109388=CARTESIAN_POINT('',(1.25,0.973783447787483,-14.59)) ;
#109389=CARTESIAN_POINT('',(1.25,0.895262490344437,-14.59)) ;
#109390=CARTESIAN_POINT('',(1.25,0.973783447787483,-15.89)) ;
#109391=CARTESIAN_POINT('Origin',(1.25,3.8,-15.24)) ;
#109392=CARTESIAN_POINT('',(1.25,2.1568323274845,-15.89)) ;
#109393=CARTESIAN_POINT('',(1.25,2.21886116991581,-15.89)) ;
#109394=CARTESIAN_POINT('',(1.25,2.33447207586456,-15.9981081081081)) ;
#109395=CARTESIAN_POINT('Origin',(1.25,2.1568323274845,-16.09)) ;
#109396=CARTESIAN_POINT('Origin',(1.25,3.8,-15.24)) ;
#109397=CARTESIAN_POINT('Origin',(-2.,0.,-17.78)) ;
#109398=CARTESIAN_POINT('',(0.899999999999999,0.,-16.84)) ;
#109399=CARTESIAN_POINT('',(1.1,0.,-16.64)) ;
#109400=CARTESIAN_POINT('Origin',(0.899999999999999,0.,-16.64)) ;
#109401=CARTESIAN_POINT('',(-2.,0.,-16.84)) ;
#109402=CARTESIAN_POINT('',(-2.,0.,-16.84)) ;
#109403=CARTESIAN_POINT('',(-2.,0.,-17.78)) ;
#109404=CARTESIAN_POINT('',(9.9,0.,-17.78)) ;
#109405=CARTESIAN_POINT('',(-2.,0.,-13.64)) ;
#109406=CARTESIAN_POINT('',(-2.,0.,-17.78)) ;
#109407=CARTESIAN_POINT('',(0.899999999999999,0.,-13.64)) ;
#109408=CARTESIAN_POINT('',(0.999999999999999,0.,-13.64)) ;
#109409=CARTESIAN_POINT('',(1.1,0.,-13.84)) ;
#109410=CARTESIAN_POINT('Origin',(0.899999999999999,0.,-13.84)) ;
#109411=CARTESIAN_POINT('',(1.1,0.,-16.74)) ;
#109412=CARTESIAN_POINT('Origin',(-2.,7.65,-17.78)) ;
#109413=CARTESIAN_POINT('',(-2.,6.9,-13.64)) ;
#109414=CARTESIAN_POINT('',(-2.,7.1,-13.84)) ;
#109415=CARTESIAN_POINT('Origin',(-2.,6.9,-13.84)) ;
#109416=CARTESIAN_POINT('',(-2.,-1.13380619344889E-17,-13.64)) ;
#109417=CARTESIAN_POINT('',(-2.,7.55,-17.78)) ;
#109418=CARTESIAN_POINT('',(-2.,6.9,-16.84)) ;
#109419=CARTESIAN_POINT('',(-2.,7.,-16.84)) ;
#109420=CARTESIAN_POINT('',(-2.,7.1,-16.64)) ;
#109421=CARTESIAN_POINT('Origin',(-2.,6.9,-16.64)) ;
#109422=CARTESIAN_POINT('',(-2.,7.1,-13.74)) ;
#109423=CARTESIAN_POINT('Origin',(-1.8,7.,-13.74)) ;
#109424=CARTESIAN_POINT('',(-1.7,0.1,-13.74)) ;
#109425=CARTESIAN_POINT('',(-1.9,0.1,-13.74)) ;
#109426=CARTESIAN_POINT('',(-2.,0.1,-13.74)) ;
#109427=CARTESIAN_POINT('',(-1.9,0.3,-13.74)) ;
#109428=CARTESIAN_POINT('',(-1.9,7.,-13.74)) ;
#109429=CARTESIAN_POINT('Origin',(-1.7,0.3,-13.74)) ;
#109430=CARTESIAN_POINT('Origin',(-1.8,7.,-16.74)) ;
#109431=CARTESIAN_POINT('',(-1.9,0.3,-16.74)) ;
#109432=CARTESIAN_POINT('',(-1.7,0.1,-16.74)) ;
#109433=CARTESIAN_POINT('Origin',(-1.7,0.3,-16.74)) ;
#109434=CARTESIAN_POINT('',(-1.9,0.1,-16.74)) ;
#109435=CARTESIAN_POINT('',(-1.9,1.23908819712629E-17,-16.74)) ;
#109436=CARTESIAN_POINT('',(0.999999999999999,0.1,-16.74)) ;
#109437=CARTESIAN_POINT('Origin',(-1.8,-2.2514151555628E-16,-15.24)) ;
#109438=CARTESIAN_POINT('',(-1.8,4.6,-15.89)) ;
#109439=CARTESIAN_POINT('',(-1.8,4.6,-14.59)) ;
#109440=CARTESIAN_POINT('',(-1.8,4.6,-14.69)) ;
#109441=CARTESIAN_POINT('',(-1.8,0.3,-14.59)) ;
#109442=CARTESIAN_POINT('',(-1.8,0.2,-14.59)) ;
#109443=CARTESIAN_POINT('',(-1.8,0.3,-13.84)) ;
#109444=CARTESIAN_POINT('',(-1.8,0.3,-13.74)) ;
#109445=CARTESIAN_POINT('',(-1.8,6.9,-13.84)) ;
#109446=CARTESIAN_POINT('',(-1.8,-5.16691679585995E-17,-13.84)) ;
#109447=CARTESIAN_POINT('',(-1.8,6.9,-16.64)) ;
#109448=CARTESIAN_POINT('',(-1.8,6.9,-15.24)) ;
#109449=CARTESIAN_POINT('',(-1.8,0.3,-16.64)) ;
#109450=CARTESIAN_POINT('',(-1.8,-3.98613863153961E-16,-16.64)) ;
#109451=CARTESIAN_POINT('',(-1.8,0.3,-15.89)) ;
#109452=CARTESIAN_POINT('',(-1.8,0.3,-15.79)) ;
#109453=CARTESIAN_POINT('',(-1.8,4.5,-15.89)) ;
#109454=CARTESIAN_POINT('Origin',(0.549999999999999,4.5,-14.69)) ;
#109455=CARTESIAN_POINT('',(-1.7,0.3,-14.69)) ;
#109456=CARTESIAN_POINT('',(-1.7,4.4,-14.69)) ;
#109457=CARTESIAN_POINT('',(-1.7,4.5,-14.69)) ;
#109458=CARTESIAN_POINT('',(0.45,4.4,-14.69)) ;
#109459=CARTESIAN_POINT('',(0.45,4.4,-14.69)) ;
#109460=CARTESIAN_POINT('',(0.45,0.3,-14.69)) ;
#109461=CARTESIAN_POINT('',(0.45,4.5,-14.69)) ;
#109462=CARTESIAN_POINT('',(0.549999999999999,0.3,-14.69)) ;
#109463=CARTESIAN_POINT('Origin',(0.549999999999999,4.5,-15.79)) ;
#109464=CARTESIAN_POINT('',(0.45,0.3,-15.79)) ;
#109465=CARTESIAN_POINT('',(0.45,4.4,-15.79)) ;
#109466=CARTESIAN_POINT('',(0.45,4.5,-15.79)) ;
#109467=CARTESIAN_POINT('',(-1.7,4.4,-15.79)) ;
#109468=CARTESIAN_POINT('',(-1.7,4.4,-15.79)) ;
#109469=CARTESIAN_POINT('',(-1.7,0.3,-15.79)) ;
#109470=CARTESIAN_POINT('',(-1.7,0.2,-15.79)) ;
#109471=CARTESIAN_POINT('',(0.549999999999999,0.3,-15.79)) ;
#109472=CARTESIAN_POINT('Origin',(0.549999999999999,4.5,-15.79)) ;
#109473=CARTESIAN_POINT('',(-1.7,4.5,-14.79)) ;
#109474=CARTESIAN_POINT('',(-1.7,4.5,-15.69)) ;
#109475=CARTESIAN_POINT('',(-1.7,4.5,-15.79)) ;
#109476=CARTESIAN_POINT('',(0.45,4.5,-15.69)) ;
#109477=CARTESIAN_POINT('',(0.45,4.5,-15.69)) ;
#109478=CARTESIAN_POINT('',(0.45,4.5,-14.79)) ;
#109479=CARTESIAN_POINT('',(0.45,4.5,-15.79)) ;
#109480=CARTESIAN_POINT('',(-1.7,4.5,-14.79)) ;
#109481=CARTESIAN_POINT('Origin',(0.55,3.09772049281573E-17,-15.24)) ;
#109482=CARTESIAN_POINT('',(0.55,2.61224989991992,-15.64)) ;
#109483=CARTESIAN_POINT('',(0.55,2.65280931275608,-15.69)) ;
#109484=CARTESIAN_POINT('Ctrl Pts',(0.55,2.61224989991992,-15.64)) ;
#109485=CARTESIAN_POINT('Ctrl Pts',(0.55,2.61224989991992,-15.643869744162)) ;
#109486=CARTESIAN_POINT('Ctrl Pts',(0.55,2.61317624258758,-15.6484201039157)) ;
#109487=CARTESIAN_POINT('Ctrl Pts',(0.55,2.61634258087509,-15.6566330008589)) ;
#109488=CARTESIAN_POINT('Ctrl Pts',(0.55,2.61951410407877,-15.6616304286453)) ;
#109489=CARTESIAN_POINT('Ctrl Pts',(0.55,2.63040394024853,-15.6749387190701)) ;
#109490=CARTESIAN_POINT('Ctrl Pts',(0.55,2.6414836688106,-15.6831705809674)) ;
#109491=CARTESIAN_POINT('Ctrl Pts',(0.55,2.65280931275608,-15.69)) ;
#109492=CARTESIAN_POINT('',(0.55,0.3,-15.69)) ;
#109493=CARTESIAN_POINT('',(0.55,1.39397422176708E-16,-15.69)) ;
#109494=CARTESIAN_POINT('',(0.55,0.3,-14.79)) ;
#109495=CARTESIAN_POINT('',(0.55,0.3,-14.69)) ;
#109496=CARTESIAN_POINT('',(0.55,2.65280931275594,-14.7900000000001)) ;
#109497=CARTESIAN_POINT('',(0.55,6.35032701027224E-17,-14.79)) ;
#109498=CARTESIAN_POINT('',(0.55,2.61224989991992,-14.84)) ;
#109499=CARTESIAN_POINT('Ctrl Pts',(0.55,2.65280931275593,-14.7900000000001)) ;
#109500=CARTESIAN_POINT('Ctrl Pts',(0.55,2.64148366881051,-14.7968294190327)) ;
#109501=CARTESIAN_POINT('Ctrl Pts',(0.55,2.6304039402485,-14.8050612809299)) ;
#109502=CARTESIAN_POINT('Ctrl Pts',(0.55,2.61951410407877,-14.8183695713547)) ;
#109503=CARTESIAN_POINT('Ctrl Pts',(0.55,2.61634258087509,-14.8233669991411)) ;
#109504=CARTESIAN_POINT('Ctrl Pts',(0.55,2.61317624258758,-14.8315798960843)) ;
#109505=CARTESIAN_POINT('Ctrl Pts',(0.55,2.61224989991992,-14.836130255838)) ;
#109506=CARTESIAN_POINT('Ctrl Pts',(0.55,2.61224989991992,-14.84)) ;
#109507=CARTESIAN_POINT('',(0.55,2.61224989991992,-14.74)) ;
#109508=CARTESIAN_POINT('Origin',(0.,0.2,-15.24)) ;
#109509=CARTESIAN_POINT('',(-1.7,0.2,-15.89)) ;
#109510=CARTESIAN_POINT('',(-1.7,0.2,-16.64)) ;
#109511=CARTESIAN_POINT('',(-1.7,0.2,-16.74)) ;
#109512=CARTESIAN_POINT('',(0.899999999999999,0.2,-16.64)) ;
#109513=CARTESIAN_POINT('',(0.999999999999999,0.2,-16.64)) ;
#109514=CARTESIAN_POINT('',(0.899999999999999,0.2,-13.84)) ;
#109515=CARTESIAN_POINT('',(0.899999999999999,0.2,-13.74)) ;
#109516=CARTESIAN_POINT('',(-1.7,0.2,-13.84)) ;
#109517=CARTESIAN_POINT('',(-1.8,0.2,-13.84)) ;
#109518=CARTESIAN_POINT('',(-1.7,0.2,-14.59)) ;
#109519=CARTESIAN_POINT('',(-1.7,0.2,-14.69)) ;
#109520=CARTESIAN_POINT('',(0.65,0.2,-14.59)) ;
#109521=CARTESIAN_POINT('',(-1.16429916652874E-32,0.2,-14.59)) ;
#109522=CARTESIAN_POINT('',(0.65,0.2,-15.89)) ;
#109523=CARTESIAN_POINT('',(0.65,0.2,-15.79)) ;
#109524=CARTESIAN_POINT('',(-1.35834902761687E-32,0.2,-15.89)) ;
#109525=CARTESIAN_POINT('Origin',(3.,2.3,-17.78)) ;
#109526=CARTESIAN_POINT('',(3.,4.2,-14.74)) ;
#109527=CARTESIAN_POINT('',(3.,3.4,-14.74)) ;
#109528=CARTESIAN_POINT('',(3.,2.3,-14.74)) ;
#109529=CARTESIAN_POINT('',(3.,4.3,-14.84)) ;
#109530=CARTESIAN_POINT('Origin',(3.,4.2,-14.84)) ;
#109531=CARTESIAN_POINT('',(3.,4.3,-15.64)) ;
#109532=CARTESIAN_POINT('',(3.,4.3,-17.78)) ;
#109533=CARTESIAN_POINT('',(3.,4.2,-15.74)) ;
#109534=CARTESIAN_POINT('Origin',(3.,4.2,-15.64)) ;
#109535=CARTESIAN_POINT('',(3.,3.4,-15.74)) ;
#109536=CARTESIAN_POINT('',(3.,2.3,-15.74)) ;
#109537=CARTESIAN_POINT('',(3.,3.3,-15.64)) ;
#109538=CARTESIAN_POINT('Origin',(3.,3.4,-15.64)) ;
#109539=CARTESIAN_POINT('',(3.,3.3,-14.84)) ;
#109540=CARTESIAN_POINT('',(3.,3.3,-17.78)) ;
#109541=CARTESIAN_POINT('Origin',(3.,3.4,-14.84)) ;
#109542=CARTESIAN_POINT('Origin',(-1.,3.8,-15.24)) ;
#109543=CARTESIAN_POINT('',(-1.,1.6,-17.2021416870349)) ;
#109544=CARTESIAN_POINT('',(-1.,1.55483870967742,-17.0755519007745)) ;
#109545=CARTESIAN_POINT('Origin',(-1.,1.40000000000001,-17.2021416870349)) ;
#109546=CARTESIAN_POINT('',(-1.,1.6,-17.78)) ;
#109547=CARTESIAN_POINT('',(-1.,2.95,-16.8831676725155)) ;
#109548=CARTESIAN_POINT('',(-1.,2.95,-15.24)) ;
#109549=CARTESIAN_POINT('',(-1.,2.1568323274845,-16.09)) ;
#109550=CARTESIAN_POINT('Origin',(-1.,3.8,-15.24)) ;
#109551=CARTESIAN_POINT('',(-1.,1.02736587339765,-16.09)) ;
#109552=CARTESIAN_POINT('',(-1.,3.8,-16.09)) ;
#109553=CARTESIAN_POINT('Origin',(-1.,3.8,-15.24)) ;
#109554=CARTESIAN_POINT('Origin',(-1.,3.05,-17.79)) ;
#109555=CARTESIAN_POINT('',(1.15,3.05,-16.8831676725155)) ;
#109556=CARTESIAN_POINT('',(1.15,3.05,-16.8211388300842)) ;
#109557=CARTESIAN_POINT('',(-0.900000000000002,3.05,-16.8831676725155)) ;
#109558=CARTESIAN_POINT('',(-1.,3.05,-16.8831676725155)) ;
#109559=CARTESIAN_POINT('',(-0.900000000000002,3.05,-17.79)) ;
#109560=CARTESIAN_POINT('Origin',(-1.,2.21886116991581,-15.99)) ;
#109561=CARTESIAN_POINT('',(-0.900000000000002,2.1568323274845,-15.99)) ;
#109562=CARTESIAN_POINT('',(1.15,2.1568323274845,-15.99)) ;
#109563=CARTESIAN_POINT('',(1.25,2.1568323274845,-15.99)) ;
#109564=CARTESIAN_POINT('',(1.15,0.895262490344437,-15.99)) ;
#109565=CARTESIAN_POINT('',(-0.900000000000002,2.21886116991581,-15.99)) ;
#109566=CARTESIAN_POINT('Origin',(-1.,3.8,-15.24)) ;
#109567=CARTESIAN_POINT('',(-0.900000000000002,2.24565220167453,-16.0440540540541)) ;
#109568=CARTESIAN_POINT('',(-0.900000000000001,2.99594594594595,-16.7943477983255)) ;
#109569=CARTESIAN_POINT('Origin',(-0.900000000000001,3.8,-15.24)) ;
#109570=CARTESIAN_POINT('',(1.15,2.99594594594595,-16.7943477983255)) ;
#109571=CARTESIAN_POINT('',(-1.,2.99594594594595,-16.7943477983255)) ;
#109572=CARTESIAN_POINT('',(1.15,2.24565220167453,-16.0440540540541)) ;
#109573=CARTESIAN_POINT('Origin',(1.15,3.8,-15.24)) ;
#109574=CARTESIAN_POINT('',(-1.,2.24565220167453,-16.0440540540541)) ;
#109575=CARTESIAN_POINT('Origin',(-1.,3.8,-15.24)) ;
#109576=CARTESIAN_POINT('',(-0.900000000000002,2.99594594594594,-13.6856522016745)) ;
#109577=CARTESIAN_POINT('',(-0.900000000000002,2.24565220167453,-14.4359459459459)) ;
#109578=CARTESIAN_POINT('Origin',(-0.900000000000001,3.8,-15.24)) ;
#109579=CARTESIAN_POINT('',(1.15,2.24565220167453,-14.4359459459459)) ;
#109580=CARTESIAN_POINT('',(-1.,2.24565220167453,-14.4359459459459)) ;
#109581=CARTESIAN_POINT('',(1.15,2.99594594594594,-13.6856522016745)) ;
#109582=CARTESIAN_POINT('Origin',(1.15,3.8,-15.24)) ;
#109583=CARTESIAN_POINT('',(-1.,2.99594594594594,-13.6856522016745)) ;
#109584=CARTESIAN_POINT('Origin',(-1.,2.21886116991581,-14.49)) ;
#109585=CARTESIAN_POINT('',(1.15,2.1568323274845,-14.49)) ;
#109586=CARTESIAN_POINT('',(1.15,2.21886116991581,-14.49)) ;
#109587=CARTESIAN_POINT('',(-0.900000000000002,2.1568323274845,-14.49)) ;
#109588=CARTESIAN_POINT('',(-1.,2.1568323274845,-14.49)) ;
#109589=CARTESIAN_POINT('',(-0.900000000000002,0.895262490344437,-14.49)) ;
#109590=CARTESIAN_POINT('Origin',(-1.,3.05,-12.69)) ;
#109591=CARTESIAN_POINT('',(-0.900000000000002,3.05,-13.5968323274845)) ;
#109592=CARTESIAN_POINT('',(1.15,3.05,-13.5968323274845)) ;
#109593=CARTESIAN_POINT('',(1.25,3.05,-13.5968323274845)) ;
#109594=CARTESIAN_POINT('',(1.15,3.05,-12.7)) ;
#109595=CARTESIAN_POINT('',(-0.900000000000002,3.05,-13.6588611699158)) ;
#109596=CARTESIAN_POINT('Origin',(-1.,3.8,-15.24)) ;
#109597=CARTESIAN_POINT('',(-1.,2.1568323274845,-14.39)) ;
#109598=CARTESIAN_POINT('',(-1.,2.95,-13.5968323274845)) ;
#109599=CARTESIAN_POINT('Origin',(-1.,3.8,-15.24)) ;
#109600=CARTESIAN_POINT('',(-1.,2.95,-12.7)) ;
#109601=CARTESIAN_POINT('',(-1.,1.6,-13.2778583129651)) ;
#109602=CARTESIAN_POINT('',(-1.,1.6,-15.24)) ;
#109603=CARTESIAN_POINT('',(-1.,1.55483870967743,-13.4044480992254)) ;
#109604=CARTESIAN_POINT('Origin',(-1.,1.40000000000001,-13.2778583129651)) ;
#109605=CARTESIAN_POINT('',(-1.,1.02736587339765,-14.39)) ;
#109606=CARTESIAN_POINT('Origin',(-1.,3.8,-15.24)) ;
#109607=CARTESIAN_POINT('',(-1.,2.21886116991581,-14.39)) ;
#109608=CARTESIAN_POINT('Origin',(-1.,3.8,-15.24)) ;
#109609=CARTESIAN_POINT('',(-1.,5.4431676725155,-16.09)) ;
#109610=CARTESIAN_POINT('',(-1.,4.65,-16.8831676725155)) ;
#109611=CARTESIAN_POINT('Origin',(-1.,3.8,-15.24)) ;
#109612=CARTESIAN_POINT('',(-1.,4.65,-15.24)) ;
#109613=CARTESIAN_POINT('',(-1.,6.45,-16.09)) ;
#109614=CARTESIAN_POINT('',(-1.,6.45,-15.99)) ;
#109615=CARTESIAN_POINT('',(-1.,3.8,-16.09)) ;
#109616=CARTESIAN_POINT('Origin',(-1.,4.55,-16.8211388300842)) ;
#109617=CARTESIAN_POINT('',(-0.900000000000001,4.55,-16.8831676725155)) ;
#109618=CARTESIAN_POINT('',(1.15,4.55,-16.8831676725155)) ;
#109619=CARTESIAN_POINT('',(1.25,4.55,-16.8831676725155)) ;
#109620=CARTESIAN_POINT('',(1.15,4.55,-17.78)) ;
#109621=CARTESIAN_POINT('',(-0.900000000000001,4.55,-16.8211388300842)) ;
#109622=CARTESIAN_POINT('Origin',(-1.,3.8,-15.24)) ;
#109623=CARTESIAN_POINT('',(-0.900000000000001,4.60405405405406,-16.7943477983255)) ;
#109624=CARTESIAN_POINT('',(-0.900000000000001,5.35434779832547,-16.0440540540541)) ;
#109625=CARTESIAN_POINT('Origin',(-0.900000000000001,3.8,-15.24)) ;
#109626=CARTESIAN_POINT('',(1.15,5.35434779832547,-16.0440540540541)) ;
#109627=CARTESIAN_POINT('',(-1.,5.35434779832547,-16.0440540540541)) ;
#109628=CARTESIAN_POINT('',(1.15,4.60405405405405,-16.7943477983255)) ;
#109629=CARTESIAN_POINT('Origin',(1.15,3.8,-15.24)) ;
#109630=CARTESIAN_POINT('',(-1.,4.60405405405406,-16.7943477983255)) ;
#109631=CARTESIAN_POINT('Origin',(-1.,6.55,-15.99)) ;
#109632=CARTESIAN_POINT('',(-0.900000000000001,5.4431676725155,-15.99)) ;
#109633=CARTESIAN_POINT('',(-0.9,6.45,-15.99)) ;
#109634=CARTESIAN_POINT('',(-0.9,6.55,-15.99)) ;
#109635=CARTESIAN_POINT('',(1.15,6.45,-15.99)) ;
#109636=CARTESIAN_POINT('',(-1.,6.45,-15.99)) ;
#109637=CARTESIAN_POINT('',(1.15,5.4431676725155,-15.99)) ;
#109638=CARTESIAN_POINT('',(1.15,5.38113883008419,-15.99)) ;
#109639=CARTESIAN_POINT('',(-1.,5.4431676725155,-15.99)) ;
#109640=CARTESIAN_POINT('Origin',(-1.,3.8,-15.24)) ;
#109641=CARTESIAN_POINT('',(-0.900000000000001,5.35434779832547,-14.4359459459459)) ;
#109642=CARTESIAN_POINT('',(-0.900000000000001,4.60405405405405,-13.6856522016745)) ;
#109643=CARTESIAN_POINT('Origin',(-0.900000000000001,3.8,-15.24)) ;
#109644=CARTESIAN_POINT('',(1.15,4.60405405405405,-13.6856522016745)) ;
#109645=CARTESIAN_POINT('',(-1.,4.60405405405405,-13.6856522016745)) ;
#109646=CARTESIAN_POINT('',(1.15,5.35434779832547,-14.4359459459459)) ;
#109647=CARTESIAN_POINT('Origin',(1.15,3.8,-15.24)) ;
#109648=CARTESIAN_POINT('',(-1.,5.35434779832547,-14.4359459459459)) ;
#109649=CARTESIAN_POINT('Origin',(-1.,4.55,-13.6588611699158)) ;
#109650=CARTESIAN_POINT('',(1.15,4.55,-13.5968323274845)) ;
#109651=CARTESIAN_POINT('',(1.15,4.55,-13.6588611699158)) ;
#109652=CARTESIAN_POINT('',(-0.900000000000001,4.55,-13.5968323274845)) ;
#109653=CARTESIAN_POINT('',(-1.,4.55,-13.5968323274845)) ;
#109654=CARTESIAN_POINT('',(-0.900000000000001,4.55,-12.7)) ;
#109655=CARTESIAN_POINT('Origin',(-1.,6.55,-14.49)) ;
#109656=CARTESIAN_POINT('',(1.15,5.4431676725155,-14.49)) ;
#109657=CARTESIAN_POINT('',(1.15,6.45,-14.49)) ;
#109658=CARTESIAN_POINT('',(1.15,6.55,-14.49)) ;
#109659=CARTESIAN_POINT('',(-0.9,6.45,-14.49)) ;
#109660=CARTESIAN_POINT('',(-1.,6.45,-14.49)) ;
#109661=CARTESIAN_POINT('',(-0.900000000000001,5.4431676725155,-14.49)) ;
#109662=CARTESIAN_POINT('',(-0.900000000000001,5.38113883008419,-14.49)) ;
#109663=CARTESIAN_POINT('',(1.25,5.4431676725155,-14.49)) ;
#109664=CARTESIAN_POINT('Origin',(-1.,3.8,-15.24)) ;
#109665=CARTESIAN_POINT('',(-1.,5.4431676725155,-14.39)) ;
#109666=CARTESIAN_POINT('',(-1.,6.45,-14.39)) ;
#109667=CARTESIAN_POINT('',(-1.,6.55,-14.39)) ;
#109668=CARTESIAN_POINT('',(-1.,6.45,-15.24)) ;
#109669=CARTESIAN_POINT('',(-1.,4.65,-13.5968323274845)) ;
#109670=CARTESIAN_POINT('',(-1.,4.65,-13.6588611699158)) ;
#109671=CARTESIAN_POINT('Origin',(-1.,3.8,-15.24)) ;
#109672=CARTESIAN_POINT('Origin',(10.,4.35421736843756,-16.115)) ;
#109673=CARTESIAN_POINT('',(9.91643989873054,7.72792407799439,-16.1010733164551)) ;
#109674=CARTESIAN_POINT('',(8.58356010126947,8.17221734381475,-15.8789266835449)) ;
#109675=CARTESIAN_POINT('',(8.47075240319158,8.20981990984071,-15.8601254005319)) ;
#109676=CARTESIAN_POINT('',(8.58356010126947,6.66256607592813,-15.8789266835449)) ;
#109677=CARTESIAN_POINT('',(8.58356010126947,6.64863939238321,-15.8789266835449)) ;
#109678=CARTESIAN_POINT('',(9.91643989873054,6.8847127088383,-16.1010733164551)) ;
#109679=CARTESIAN_POINT('',(9.98442535909739,6.89604361889945,-16.1124042265162)) ;
#109680=CARTESIAN_POINT('',(9.91643989873054,7.8,-16.1010733164551)) ;
#109681=CARTESIAN_POINT('Origin',(8.5,4.35421736843756,-15.865)) ;
#109682=CARTESIAN_POINT('',(8.5,8.17221734381475,-15.7802872911617)) ;
#109683=CARTESIAN_POINT('',(8.50000000129681,8.20000000266559,-15.782105625353)) ;
#109684=CARTESIAN_POINT('Origin',(8.5,8.17870774547598,-15.9690376376839)) ;
#109685=CARTESIAN_POINT('',(8.5,8.2,-14.6563454436991)) ;
#109686=CARTESIAN_POINT('',(8.5,6.66256607592813,-14.6997127088383)) ;
#109687=CARTESIAN_POINT('',(8.5,6.64863939238321,-14.6997127088383)) ;
#109688=CARTESIAN_POINT('',(8.50000000002143,6.64999999935441,-14.6993178443262)) ;
#109689=CARTESIAN_POINT('Origin',(8.5,6.65811550062454,-14.503188522499)) ;
#109690=CARTESIAN_POINT('',(8.49999999999933,6.65000073218972,-15.7806896909636)) ;
#109691=CARTESIAN_POINT('',(8.5,6.65,-15.9636393923832)) ;
#109692=CARTESIAN_POINT('',(8.5,6.66256607592813,-15.7802872911617)) ;
#109693=CARTESIAN_POINT('Origin',(8.5,6.65133313712442,-15.9770100835082)) ;
#109694=CARTESIAN_POINT('',(8.5,8.20007071090457,-15.7802872911617)) ;
#109695=CARTESIAN_POINT('Origin',(8.5,4.35421736843756,-14.615)) ;
#109696=CARTESIAN_POINT('',(9.91643989873054,6.8847127088383,-14.3789266835449)) ;
#109697=CARTESIAN_POINT('',(8.58356010126947,6.66256607592813,-14.6010733164551)) ;
#109698=CARTESIAN_POINT('',(8.48442535909739,6.64604361889945,-14.6175957734838)) ;
#109699=CARTESIAN_POINT('',(8.58356010126947,8.20007071090456,-14.6010733164551)) ;
#109700=CARTESIAN_POINT('',(9.91643989873054,7.72792407799439,-14.3789266835449)) ;
#109701=CARTESIAN_POINT('',(9.97075240319158,7.70981990984071,-14.3698745994681)) ;
#109702=CARTESIAN_POINT('',(9.91643989873054,6.8,-14.3789266835449)) ;
#109703=CARTESIAN_POINT('Origin',(8.5,3.65,-14.74)) ;
#109704=CARTESIAN_POINT('',(8.45734623443633,3.62014236410543,-15.1420655561573)) ;
#109705=CARTESIAN_POINT('',(8.02582401135442,3.3180768079481,-14.84)) ;
#109706=CARTESIAN_POINT('',(8.34729988159781,3.54310991711847,-15.0650331091704)) ;
#109707=CARTESIAN_POINT('',(8.02582401135442,3.31807680794809,-15.64)) ;
#109708=CARTESIAN_POINT('',(8.02582401135442,3.3180768079481,-14.74)) ;
#109709=CARTESIAN_POINT('',(8.45734623443633,3.62014236410543,-15.3379344438427)) ;
#109710=CARTESIAN_POINT('',(8.70083523513316,3.79058466459322,-15.1674921433549)) ;
#109711=CARTESIAN_POINT('',(8.45734623443633,3.62014236410543,-14.74)) ;
#109712=CARTESIAN_POINT('Origin',(8.5,3.95,-14.74)) ;
#109713=CARTESIAN_POINT('',(8.5,3.89793444384266,-15.3379344438427)) ;
#109714=CARTESIAN_POINT('',(8.5,3.89793444384266,-15.1420655561573)) ;
#109715=CARTESIAN_POINT('',(8.5,3.89793444384266,-14.74)) ;
#109716=CARTESIAN_POINT('',(8.5,3.70206555615734,-15.1420655561573)) ;
#109717=CARTESIAN_POINT('',(8.5,3.95,-15.1420655561573)) ;
#109718=CARTESIAN_POINT('',(8.5,3.70206555615734,-15.3379344438427)) ;
#109719=CARTESIAN_POINT('',(8.5,3.70206555615734,-14.74)) ;
#109720=CARTESIAN_POINT('',(8.5,3.95,-15.3379344438427)) ;
#109721=CARTESIAN_POINT('Origin',(8.,4.3,-14.74)) ;
#109722=CARTESIAN_POINT('',(8.45734623443633,3.97985763589457,-15.3379344438427)) ;
#109723=CARTESIAN_POINT('',(8.02582401135442,4.2819231920519,-15.64)) ;
#109724=CARTESIAN_POINT('',(8.32457260887054,4.07279917379062,-15.4308759817387)) ;
#109725=CARTESIAN_POINT('',(8.02582401135442,4.2819231920519,-14.84)) ;
#109726=CARTESIAN_POINT('',(8.02582401135442,4.2819231920519,-14.74)) ;
#109727=CARTESIAN_POINT('',(8.45734623443633,3.97985763589457,-15.1420655561573)) ;
#109728=CARTESIAN_POINT('',(7.97103725533518,4.32027392126537,-14.8016492707865)) ;
#109729=CARTESIAN_POINT('',(8.45734623443633,3.97985763589457,-14.74)) ;
#109730=CARTESIAN_POINT('Origin',(1.5,2.3,-14.74)) ;
#109731=CARTESIAN_POINT('',(7.96847777691809,3.4,-14.74)) ;
#109732=CARTESIAN_POINT('',(8.,3.4,-14.74)) ;
#109733=CARTESIAN_POINT('',(7.96847777691809,4.2,-14.74)) ;
#109734=CARTESIAN_POINT('',(7.96847777691809,4.2,-14.74)) ;
#109735=CARTESIAN_POINT('',(3.,4.2,-14.74)) ;
#109736=CARTESIAN_POINT('Origin',(1.5,2.3,-15.74)) ;
#109737=CARTESIAN_POINT('',(7.96847777691809,4.2,-15.74)) ;
#109738=CARTESIAN_POINT('',(1.5,4.2,-15.74)) ;
#109739=CARTESIAN_POINT('',(7.96847777691809,3.4,-15.74)) ;
#109740=CARTESIAN_POINT('',(7.96847777691809,2.3,-15.74)) ;
#109741=CARTESIAN_POINT('',(1.5,3.4,-15.74)) ;
#109742=CARTESIAN_POINT('Origin',(8.,3.3,-14.74)) ;
#109743=CARTESIAN_POINT('',(7.96847777691809,3.3,-15.64)) ;
#109744=CARTESIAN_POINT('',(8.,3.3,-15.64)) ;
#109745=CARTESIAN_POINT('',(7.96847777691809,3.3,-14.84)) ;
#109746=CARTESIAN_POINT('',(7.96847777691809,3.3,-14.74)) ;
#109747=CARTESIAN_POINT('',(3.,3.3,-14.84)) ;
#109748=CARTESIAN_POINT('Origin',(1.5,4.3,-14.74)) ;
#109749=CARTESIAN_POINT('',(7.96847777691809,4.3,-14.84)) ;
#109750=CARTESIAN_POINT('',(8.,4.3,-14.84)) ;
#109751=CARTESIAN_POINT('',(7.96847777691809,4.3,-15.64)) ;
#109752=CARTESIAN_POINT('',(7.96847777691809,4.3,-14.74)) ;
#109753=CARTESIAN_POINT('',(1.5,4.3,-15.64)) ;
#109754=CARTESIAN_POINT('Origin',(1.5,2.3,-14.74)) ;
#109755=CARTESIAN_POINT('',(-0.4,2.3,-14.74)) ;
#109756=CARTESIAN_POINT('',(-0.4,-3.36847777691809,-14.74)) ;
#109757=CARTESIAN_POINT('',(-0.4,-3.4,-14.74)) ;
#109758=CARTESIAN_POINT('',(0.4,-3.36847777691809,-14.74)) ;
#109759=CARTESIAN_POINT('',(0.4,-3.36847777691809,-14.74)) ;
#109760=CARTESIAN_POINT('',(0.4,2.29999999999999,-14.74)) ;
#109761=CARTESIAN_POINT('',(0.4,2.29999999999999,-14.74)) ;
#109762=CARTESIAN_POINT('',(0.536602540378444,2.83090991212703,-14.74)) ;
#109763=CARTESIAN_POINT('Origin',(1.5,2.3,-14.74)) ;
#109764=CARTESIAN_POINT('',(0.536602540378444,3.93764017256378,-14.74)) ;
#109765=CARTESIAN_POINT('',(0.536602540378444,2.83090991212703,-14.74)) ;
#109766=CARTESIAN_POINT('Origin',(1.5,2.3,-14.74)) ;
#109767=CARTESIAN_POINT('Origin',(1.5,2.3,-15.74)) ;
#109768=CARTESIAN_POINT('',(0.4,2.29999999999999,-15.74)) ;
#109769=CARTESIAN_POINT('',(0.4,-3.36847777691809,-15.74)) ;
#109770=CARTESIAN_POINT('',(0.4,2.3,-15.74)) ;
#109771=CARTESIAN_POINT('',(-0.4,-3.36847777691809,-15.74)) ;
#109772=CARTESIAN_POINT('',(1.5,-3.36847777691809,-15.74)) ;
#109773=CARTESIAN_POINT('',(-0.4,2.3,-15.74)) ;
#109774=CARTESIAN_POINT('',(-0.4,2.3,-15.74)) ;
#109775=CARTESIAN_POINT('',(0.536602540378444,3.93764017256378,-15.74)) ;
#109776=CARTESIAN_POINT('Origin',(1.5,2.3,-15.74)) ;
#109777=CARTESIAN_POINT('',(0.536602540378444,2.83090991212703,-15.74)) ;
#109778=CARTESIAN_POINT('',(0.536602540378444,3.93764017256378,-15.74)) ;
#109779=CARTESIAN_POINT('Origin',(1.5,2.3,-15.74)) ;
#109780=CARTESIAN_POINT('Origin',(1.5,2.3,-14.74)) ;
#109781=CARTESIAN_POINT('',(-0.5,2.3,-14.84)) ;
#109782=CARTESIAN_POINT('',(-0.5,2.3,-15.64)) ;
#109783=CARTESIAN_POINT('',(-0.5,2.3,-14.74)) ;
#109784=CARTESIAN_POINT('Origin',(1.5,2.3,-14.84)) ;
#109785=CARTESIAN_POINT('Origin',(1.5,2.3,-15.64)) ;
#109786=CARTESIAN_POINT('Origin',(-0.5,-3.4,-14.74)) ;
#109787=CARTESIAN_POINT('',(-0.5,-3.36847777691809,-15.64)) ;
#109788=CARTESIAN_POINT('',(-0.5,-3.4,-15.64)) ;
#109789=CARTESIAN_POINT('',(-0.5,-3.36847777691809,-14.84)) ;
#109790=CARTESIAN_POINT('',(-0.5,-3.36847777691809,-14.74)) ;
#109791=CARTESIAN_POINT('',(-0.5,2.3,-14.84)) ;
#109792=CARTESIAN_POINT('Origin',(-0.15,-3.9,-14.74)) ;
#109793=CARTESIAN_POINT('',(-0.179857635894567,-3.85734623443633,-15.1420655561573)) ;
#109794=CARTESIAN_POINT('',(-0.481923192051905,-3.42582401135442,-14.84)) ;
#109795=CARTESIAN_POINT('',(-0.256890082881532,-3.74729988159781,-15.0650331091704)) ;
#109796=CARTESIAN_POINT('',(-0.481923192051905,-3.42582401135442,-15.64)) ;
#109797=CARTESIAN_POINT('',(-0.481923192051905,-3.42582401135442,-14.74)) ;
#109798=CARTESIAN_POINT('',(-0.179857635894567,-3.85734623443633,-15.3379344438427)) ;
#109799=CARTESIAN_POINT('',(-0.00941533540678435,-4.10083523513317,-15.1674921433549)) ;
#109800=CARTESIAN_POINT('',(-0.179857635894567,-3.85734623443633,-14.74)) ;
#109801=CARTESIAN_POINT('Origin',(0.15,-3.9,-14.74)) ;
#109802=CARTESIAN_POINT('',(0.0979344438426627,-3.9,-15.3379344438427)) ;
#109803=CARTESIAN_POINT('',(0.0979344438426627,-3.9,-15.1420655561573)) ;
#109804=CARTESIAN_POINT('',(0.0979344438426627,-3.9,-14.74)) ;
#109805=CARTESIAN_POINT('',(-0.0979344438426628,-3.9,-15.1420655561573)) ;
#109806=CARTESIAN_POINT('',(0.15,-3.9,-15.1420655561573)) ;
#109807=CARTESIAN_POINT('',(-0.0979344438426628,-3.9,-15.3379344438427)) ;
#109808=CARTESIAN_POINT('',(-0.0979344438426628,-3.9,-14.74)) ;
#109809=CARTESIAN_POINT('',(0.15,-3.9,-15.3379344438427)) ;
#109810=CARTESIAN_POINT('Origin',(0.5,-3.4,-14.74)) ;
#109811=CARTESIAN_POINT('',(0.179857635894567,-3.85734623443633,-15.3379344438427)) ;
#109812=CARTESIAN_POINT('',(0.481923192051904,-3.42582401135442,-15.64)) ;
#109813=CARTESIAN_POINT('',(0.272799173790623,-3.72457260887054,-15.4308759817387)) ;
#109814=CARTESIAN_POINT('',(0.481923192051904,-3.42582401135442,-14.84)) ;
#109815=CARTESIAN_POINT('',(0.481923192051904,-3.42582401135442,-14.74)) ;
#109816=CARTESIAN_POINT('',(0.179857635894567,-3.85734623443633,-15.1420655561573)) ;
#109817=CARTESIAN_POINT('',(0.520273921265371,-3.37103725533519,-14.8016492707865)) ;
#109818=CARTESIAN_POINT('',(0.179857635894567,-3.85734623443633,-14.74)) ;
#109819=CARTESIAN_POINT('Origin',(0.5,2.29999999999999,-14.74)) ;
#109820=CARTESIAN_POINT('',(0.500000000000001,2.29999999999999,-14.84)) ;
#109821=CARTESIAN_POINT('',(0.5,-3.36847777691809,-14.84)) ;
#109822=CARTESIAN_POINT('',(0.5,-3.4,-14.84)) ;
#109823=CARTESIAN_POINT('',(0.5,-3.36847777691809,-15.64)) ;
#109824=CARTESIAN_POINT('',(0.5,-3.36847777691809,-14.74)) ;
#109825=CARTESIAN_POINT('',(0.500000000000001,2.29999999999999,-15.64)) ;
#109826=CARTESIAN_POINT('',(0.5,2.29999999999999,-15.64)) ;
#109827=CARTESIAN_POINT('',(0.500000000000001,2.29999999999999,-14.74)) ;
#109828=CARTESIAN_POINT('Origin',(1.5,2.3,-14.74)) ;
#109829=CARTESIAN_POINT('Origin',(1.5,2.3,-14.84)) ;
#109830=CARTESIAN_POINT('Origin',(1.5,2.3,-15.64)) ;
#109831=CARTESIAN_POINT('Origin',(8.,2.68967221921331,-15.74)) ;
#109832=CARTESIAN_POINT('',(8.45734623443633,3.70206555615734,-15.4198576358946)) ;
#109833=CARTESIAN_POINT('',(8.02582401135442,3.4,-15.7219231920519)) ;
#109834=CARTESIAN_POINT('',(7.75526480758232,3.21060855735952,-15.9113146346924)) ;
#109835=CARTESIAN_POINT('',(8.02582401135442,4.2,-15.7219231920519)) ;
#109836=CARTESIAN_POINT('',(8.02582401135442,2.68967221921331,-15.7219231920519)) ;
#109837=CARTESIAN_POINT('',(8.45734623443633,3.89793444384266,-15.4198576358946)) ;
#109838=CARTESIAN_POINT('',(8.54034505662341,3.83983526831171,-15.3617584603636)) ;
#109839=CARTESIAN_POINT('',(8.45734623443633,2.68967221921331,-15.4198576358946)) ;
#109840=CARTESIAN_POINT('Origin',(8.,2.68967221921331,-14.74)) ;
#109841=CARTESIAN_POINT('',(8.45734623443633,3.89793444384266,-15.0601423641054)) ;
#109842=CARTESIAN_POINT('',(8.02582401135442,4.2,-14.7580768079481)) ;
#109843=CARTESIAN_POINT('',(8.54034505662341,3.83983526831171,-15.1182415396364)) ;
#109844=CARTESIAN_POINT('',(8.02582401135442,3.4,-14.7580768079481)) ;
#109845=CARTESIAN_POINT('',(8.02582401135442,3.4,-14.7580768079481)) ;
#109846=CARTESIAN_POINT('',(8.45734623443633,3.70206555615734,-15.0601423641054)) ;
#109847=CARTESIAN_POINT('',(7.75526480758232,3.21060855735952,-14.5686853653076)) ;
#109848=CARTESIAN_POINT('',(8.45734623443633,2.68967221921331,-15.0601423641054)) ;
#109849=CARTESIAN_POINT('Origin',(-1.11032778078669,-3.9,-15.09)) ;
#109850=CARTESIAN_POINT('',(0.0979344438426626,-3.85734623443633,-15.0601423641054)) ;
#109851=CARTESIAN_POINT('',(0.4,-3.42582401135442,-14.7580768079481)) ;
#109852=CARTESIAN_POINT('',(-0.223548570072128,-4.31660768288603,-15.3816253780202)) ;
#109853=CARTESIAN_POINT('',(-0.400000000000001,-3.42582401135442,-14.7580768079481)) ;
#109854=CARTESIAN_POINT('',(-0.400000000000001,-3.42582401135442,-14.7580768079481)) ;
#109855=CARTESIAN_POINT('',(-0.0979344438426627,-3.85734623443633,-15.0601423641054)) ;
#109856=CARTESIAN_POINT('',(-0.326007604256636,-3.53152743384494,-14.8320692036915)) ;
#109857=CARTESIAN_POINT('',(-1.11032778078669,-3.85734623443633,-15.0601423641054)) ;
#109858=CARTESIAN_POINT('Origin',(-1.11032778078669,-3.4,-15.74)) ;
#109859=CARTESIAN_POINT('',(-0.0979344438426627,-3.85734623443633,-15.4198576358946)) ;
#109860=CARTESIAN_POINT('',(-0.4,-3.42582401135442,-15.7219231920519)) ;
#109861=CARTESIAN_POINT('',(-0.589391442640475,-3.15526480758232,-15.9113146346924)) ;
#109862=CARTESIAN_POINT('',(0.400000000000001,-3.42582401135442,-15.7219231920519)) ;
#109863=CARTESIAN_POINT('',(-1.11032778078669,-3.42582401135442,-15.7219231920519)) ;
#109864=CARTESIAN_POINT('',(0.0979344438426626,-3.85734623443633,-15.4198576358946)) ;
#109865=CARTESIAN_POINT('',(0.0398352683117103,-3.94034505662341,-15.3617584603636)) ;
#109866=CARTESIAN_POINT('',(-1.11032778078669,-3.85734623443633,-15.4198576358946)) ;
#109867=CARTESIAN_POINT('Origin',(10.,1.24999999999998,-17.78)) ;
#109868=CARTESIAN_POINT('',(9.91643989873054,1.26392668354489,-13.1958381198218)) ;
#109869=CARTESIAN_POINT('',(9.91643989873054,1.26392668354489,-17.78)) ;
#109870=CARTESIAN_POINT('',(8.50816364570057,1.49863939238321,-13.2778583129651)) ;
#109871=CARTESIAN_POINT('Origin',(43.7052916800694,-4.36754861267736,-621.928202370209)) ;
#109872=CARTESIAN_POINT('',(8.50816364570057,1.49863939238321,-17.78)) ;
#109873=CARTESIAN_POINT('Origin',(8.49999999999985,3.8,-15.24)) ;
#109874=CARTESIAN_POINT('',(9.91643989873053,1.24322097942674,-13.2563035641941)) ;
#109875=CARTESIAN_POINT('',(9.91643989873053,1.24322097942648,-17.2236964358056)) ;
#109876=CARTESIAN_POINT('Origin',(9.91643989873053,3.8,-15.24)) ;
#109877=CARTESIAN_POINT('Origin',(36.548065341889,-40.3802616891523,557.037655188902)) ;
#109878=CARTESIAN_POINT('Origin',(36.5480653700872,-40.3802615697373,-587.517655338219)) ;
#109879=CARTESIAN_POINT('Origin',(10.,1.24999999999998,-17.78)) ;
#109880=CARTESIAN_POINT('',(8.50816364570059,1.49863939238321,-17.2021416870347)) ;
#109881=CARTESIAN_POINT('',(8.50816364570057,1.49863939238321,-17.78)) ;
#109882=CARTESIAN_POINT('',(9.91643989873054,1.26392668354489,-17.2841618801782)) ;
#109883=CARTESIAN_POINT('Origin',(43.7052917204119,-4.36754862113872,591.448203083967)) ;
#109884=CARTESIAN_POINT('',(9.91643989873054,1.26392668354489,-17.78)) ;
#109885=CARTESIAN_POINT('Origin',(-0.900000000000001,4.65,-15.24)) ;
#109886=CARTESIAN_POINT('Origin',(-0.900000000000001,4.65,-13.5968323274845)) ;
#109887=CARTESIAN_POINT('Origin',(-0.900000000000001,4.65,-13.5968323274845)) ;
#109888=CARTESIAN_POINT('Origin',(-0.900000000000001,4.65,-13.5968323274845)) ;
#109889=CARTESIAN_POINT('Origin',(-0.900000000000001,4.65,-13.5968323274845)) ;
#109890=CARTESIAN_POINT('Origin',(1.15,4.45,-13.6588611699158)) ;
#109891=CARTESIAN_POINT('Origin',(1.15,4.45,-13.5968323274845)) ;
#109892=CARTESIAN_POINT('Origin',(-1.,4.65,-13.5968323274845)) ;
#109893=CARTESIAN_POINT('Origin',(1.15,4.65,-13.5968323274845)) ;
#109894=CARTESIAN_POINT('Origin',(-0.900000000000001,3.8,-15.24)) ;
#109895=CARTESIAN_POINT('Origin',(-0.900000000000001,5.4431676725155,-14.39)) ;
#109896=CARTESIAN_POINT('Origin',(1.15,4.65,-13.5968323274845)) ;
#109897=CARTESIAN_POINT('Origin',(1.15,4.55810810810811,-13.7744720758646)) ;
#109898=CARTESIAN_POINT('Origin',(-0.900000000000001,5.4431676725155,-14.39)) ;
#109899=CARTESIAN_POINT('Origin',(-0.900000000000001,5.4431676725155,-14.39)) ;
#109900=CARTESIAN_POINT('Origin',(-0.900000000000001,5.4431676725155,-14.39)) ;
#109901=CARTESIAN_POINT('Origin',(-0.900000000000001,4.65,-15.24)) ;
#109902=CARTESIAN_POINT('Origin',(-0.900000000000001,4.65,-16.8831676725155)) ;
#109903=CARTESIAN_POINT('Origin',(-1.,4.65,-16.8831676725155)) ;
#109904=CARTESIAN_POINT('Origin',(1.15,4.65,-16.8831676725155)) ;
#109905=CARTESIAN_POINT('Origin',(-0.900000000000001,4.65,-16.8831676725155)) ;
#109906=CARTESIAN_POINT('Origin',(1.15,4.45,-16.8211388300842)) ;
#109907=CARTESIAN_POINT('Origin',(1.15,4.45,-16.8831676725155)) ;
#109908=CARTESIAN_POINT('Origin',(1.15,3.8,-15.24)) ;
#109909=CARTESIAN_POINT('Origin',(1.15,5.26552792413544,-14.4818918918919)) ;
#109910=CARTESIAN_POINT('Origin',(-1.,5.4431676725155,-14.39)) ;
#109911=CARTESIAN_POINT('Origin',(1.15,5.4431676725155,-14.39)) ;
#109912=CARTESIAN_POINT('Origin',(-0.900000000000001,3.8,-14.39)) ;
#109913=CARTESIAN_POINT('Origin',(-0.9,6.45,-14.39)) ;
#109914=CARTESIAN_POINT('Origin',(-0.9,6.45,-15.24)) ;
#109915=CARTESIAN_POINT('Origin',(-0.9,6.45,-14.39)) ;
#109916=CARTESIAN_POINT('Origin',(-0.900000000000001,4.65,-16.8831676725155)) ;
#109917=CARTESIAN_POINT('Origin',(-0.900000000000001,4.65,-16.8831676725155)) ;
#109918=CARTESIAN_POINT('Origin',(1.15,4.65,-16.8831676725155)) ;
#109919=CARTESIAN_POINT('Origin',(1.15,4.55810810810811,-16.7055279241354)) ;
#109920=CARTESIAN_POINT('Origin',(1.15,5.4431676725155,-14.39)) ;
#109921=CARTESIAN_POINT('Origin',(1.15,5.4431676725155,-14.59)) ;
#109922=CARTESIAN_POINT('Origin',(-0.9,6.45,-14.39)) ;
#109923=CARTESIAN_POINT('Origin',(-0.9,6.45,-14.39)) ;
#109924=CARTESIAN_POINT('Origin',(-0.900000000000001,3.8,-15.24)) ;
#109925=CARTESIAN_POINT('Origin',(-0.900000000000001,5.4431676725155,-16.09)) ;
#109926=CARTESIAN_POINT('Origin',(-1.,5.4431676725155,-16.09)) ;
#109927=CARTESIAN_POINT('Origin',(1.15,5.4431676725155,-16.09)) ;
#109928=CARTESIAN_POINT('Origin',(-0.900000000000001,5.4431676725155,-16.09)) ;
#109929=CARTESIAN_POINT('Origin',(1.15,3.8,-15.24)) ;
#109930=CARTESIAN_POINT('Origin',(1.15,5.26552792413544,-15.9981081081081)) ;
#109931=CARTESIAN_POINT('Origin',(1.15,6.55,-14.59)) ;
#109932=CARTESIAN_POINT('Origin',(1.15,6.45,-14.59)) ;
#109933=CARTESIAN_POINT('Origin',(1.25,6.45,-14.39)) ;
#109934=CARTESIAN_POINT('Origin',(1.15,6.45,-14.39)) ;
#109935=CARTESIAN_POINT('Origin',(-0.900000000000001,5.4431676725155,-16.09)) ;
#109936=CARTESIAN_POINT('Origin',(-0.900000000000001,5.4431676725155,-16.09)) ;
#109937=CARTESIAN_POINT('Origin',(1.15,5.4431676725155,-16.09)) ;
#109938=CARTESIAN_POINT('Origin',(1.15,5.4431676725155,-15.89)) ;
#109939=CARTESIAN_POINT('Origin',(1.15,6.45,-14.59)) ;
#109940=CARTESIAN_POINT('Origin',(1.35,6.45,-14.59)) ;
#109941=CARTESIAN_POINT('Origin',(-0.9,6.45,-15.24)) ;
#109942=CARTESIAN_POINT('Origin',(-0.9,6.45,-16.09)) ;
#109943=CARTESIAN_POINT('Origin',(-0.900000000000001,3.8,-16.09)) ;
#109944=CARTESIAN_POINT('Origin',(-0.9,6.45,-16.09)) ;
#109945=CARTESIAN_POINT('Origin',(1.15,6.55,-15.89)) ;
#109946=CARTESIAN_POINT('Origin',(1.15,6.45,-15.89)) ;
#109947=CARTESIAN_POINT('Origin',(1.35,6.45,-17.78)) ;
#109948=CARTESIAN_POINT('Origin',(1.35,6.45,-15.89)) ;
#109949=CARTESIAN_POINT('Origin',(-0.9,6.45,-16.09)) ;
#109950=CARTESIAN_POINT('Origin',(-0.9,6.45,-16.09)) ;
#109951=CARTESIAN_POINT('Origin',(1.15,6.45,-15.89)) ;
#109952=CARTESIAN_POINT('Origin',(1.15,6.45,-16.09)) ;
#109953=CARTESIAN_POINT('Origin',(-1.,6.45,-16.09)) ;
#109954=CARTESIAN_POINT('Origin',(-1.7,0.3,-15.89)) ;
#109955=CARTESIAN_POINT('Origin',(-1.7,0.3,-15.89)) ;
#109956=CARTESIAN_POINT('Origin',(-1.7,0.3,-15.89)) ;
#109957=CARTESIAN_POINT('Origin',(-1.7,0.3,-15.89)) ;
#109958=CARTESIAN_POINT('Origin',(0.549999999999999,0.3,-15.89)) ;
#109959=CARTESIAN_POINT('',(0.508578643762786,0.229289321881393,-15.8192893218813)) ;
#109960=CARTESIAN_POINT('Ctrl Pts',(0.65,0.200000000000001,-15.89)) ;
#109961=CARTESIAN_POINT('Ctrl Pts',(0.639834283464216,0.200000000000001,
-15.8849171417321)) ;
#109962=CARTESIAN_POINT('Ctrl Pts',(0.629316849080668,0.200389688120421,
-15.879657683858)) ;
#109963=CARTESIAN_POINT('Ctrl Pts',(0.606957334719987,0.202165884217636,
-15.8684679497194)) ;
#109964=CARTESIAN_POINT('Ctrl Pts',(0.595086727401534,0.203647820493406,
-15.8625227617951)) ;
#109965=CARTESIAN_POINT('Ctrl Pts',(0.572283837383803,0.207685608830691,
-15.8511067603976)) ;
#109966=CARTESIAN_POINT('Ctrl Pts',(0.561337481656533,0.210178193246995,
-15.845629861311)) ;
#109967=CARTESIAN_POINT('Ctrl Pts',(0.549549942891241,0.21354462066391,
-15.8397406960421)) ;
#109968=CARTESIAN_POINT('Ctrl Pts',(0.548290718948854,0.213913346521105,
-15.8391116827675)) ;
#109969=CARTESIAN_POINT('Ctrl Pts',(0.536119229733182,0.217566912232434,
-15.8330327513519)) ;
#109970=CARTESIAN_POINT('Ctrl Pts',(0.525706917362863,0.221400308602525,
-15.8278422384292)) ;
#109971=CARTESIAN_POINT('Ctrl Pts',(0.513545110027474,0.226871185484662,
-15.8217711869643)) ;
#109972=CARTESIAN_POINT('Ctrl Pts',(0.511029334128474,0.228063976698571,
-15.8205146670641)) ;
#109973=CARTESIAN_POINT('Ctrl Pts',(0.508578643762786,0.229289321881393,
-15.8192893218813)) ;
#109974=CARTESIAN_POINT('Origin',(0.664280054284628,0.302990743358677,-15.8971421042412)) ;
#109975=CARTESIAN_POINT('Origin',(-1.7,4.5,-15.89)) ;
#109976=CARTESIAN_POINT('',(-1.77071067811866,4.45857864376269,-15.8192893218813)) ;
#109977=CARTESIAN_POINT('Origin',(-1.69703459697991,4.61417009502528,-15.8970866853669)) ;
#109978=CARTESIAN_POINT('Ctrl Pts',(-1.77071067811863,4.45857864376269,
-15.8192893218813)) ;
#109979=CARTESIAN_POINT('Ctrl Pts',(-1.77521675558369,4.46759079869274,
-15.8237953993464)) ;
#109980=CARTESIAN_POINT('Ctrl Pts',(-1.77928079264421,4.47748625817285,
-15.8287264816716)) ;
#109981=CARTESIAN_POINT('Ctrl Pts',(-1.78624680748596,4.49811277056786,
-15.8390208825473)) ;
#109982=CARTESIAN_POINT('Ctrl Pts',(-1.78918030781743,4.50880509433296,
-15.8443639841482)) ;
#109983=CARTESIAN_POINT('Ctrl Pts',(-1.79185985500253,4.52101859321847,
-15.8504747545319)) ;
#109984=CARTESIAN_POINT('Ctrl Pts',(-1.79213045061208,4.52228751722605,
-15.8511097099085)) ;
#109985=CARTESIAN_POINT('Ctrl Pts',(-1.7947746790983,4.53504937002851,-15.8574962891339)) ;
#109986=CARTESIAN_POINT('Ctrl Pts',(-1.79657370273652,4.54677936428193,
-15.8633715724062)) ;
#109987=CARTESIAN_POINT('Ctrl Pts',(-1.79896007643135,4.56920025888384,
-15.8745957747611)) ;
#109988=CARTESIAN_POINT('Ctrl Pts',(-1.79963010255187,4.57990192168146,
-15.8799500759449)) ;
#109989=CARTESIAN_POINT('Ctrl Pts',(-1.79996164986962,4.59357116034291,
-15.886785573817)) ;
#109990=CARTESIAN_POINT('Ctrl Pts',(-1.8,4.59680282631912,-15.8884014131596)) ;
#109991=CARTESIAN_POINT('Ctrl Pts',(-1.8,4.6,-15.89)) ;
#109992=CARTESIAN_POINT('Origin',(-1.7,0.3,-15.24)) ;
#109993=CARTESIAN_POINT('Origin',(-1.7,0.3,-16.64)) ;
#109994=CARTESIAN_POINT('Origin',(0.65,0.3,-15.24)) ;
#109995=CARTESIAN_POINT('',(0.579289321881345,0.229289321881345,-15.7485786437627)) ;
#109996=CARTESIAN_POINT('Origin',(0.65708668537483,0.30296540302241,-15.9041700950407)) ;
#109997=CARTESIAN_POINT('Ctrl Pts',(0.579289321881345,0.229289321881345,
-15.7485786437627)) ;
#109998=CARTESIAN_POINT('Ctrl Pts',(0.583795399346368,0.224783244416322,
-15.7575907986927)) ;
#109999=CARTESIAN_POINT('Ctrl Pts',(0.588726481671644,0.220719207355776,
-15.7674862581729)) ;
#110000=CARTESIAN_POINT('Ctrl Pts',(0.599020882547771,0.213753192513755,
-15.7881127705687)) ;
#110001=CARTESIAN_POINT('Ctrl Pts',(0.604363984149059,0.210819692182103,
-15.7988050943346)) ;
#110002=CARTESIAN_POINT('Ctrl Pts',(0.610474754532788,0.2081401449971,-15.8110185932201)) ;
#110003=CARTESIAN_POINT('Ctrl Pts',(0.611109709908931,0.207869549387732,
-15.8122875172269)) ;
#110004=CARTESIAN_POINT('Ctrl Pts',(0.617496289133965,0.205225320901699,
-15.8250493700286)) ;
#110005=CARTESIAN_POINT('Ctrl Pts',(0.623371572406214,0.203426297263465,
-15.836779364282)) ;
#110006=CARTESIAN_POINT('Ctrl Pts',(0.634595774761229,0.201039923568636,
-15.859200258884)) ;
#110007=CARTESIAN_POINT('Ctrl Pts',(0.639950075945052,0.200369897448118,
-15.8699019216816)) ;
#110008=CARTESIAN_POINT('Ctrl Pts',(0.646785573817061,0.200038350130375,
-15.883571160343)) ;
#110009=CARTESIAN_POINT('Ctrl Pts',(0.64840141315959,0.2,-15.8868028263192)) ;
#110010=CARTESIAN_POINT('Ctrl Pts',(0.65,0.2,-15.89)) ;
#110011=CARTESIAN_POINT('',(0.579289321881328,0.229289321881363,-14.7314213562373)) ;
#110012=CARTESIAN_POINT('Ctrl Pts',(0.65,0.2,-14.59)) ;
#110013=CARTESIAN_POINT('Ctrl Pts',(0.644917141732081,0.2,-14.6001657165358)) ;
#110014=CARTESIAN_POINT('Ctrl Pts',(0.639657683858012,0.200389688120423,
-14.6106831509194)) ;
#110015=CARTESIAN_POINT('Ctrl Pts',(0.628467949719366,0.202165884217642,
-14.6330426652802)) ;
#110016=CARTESIAN_POINT('Ctrl Pts',(0.622522761794963,0.203647820493433,
-14.6449132725987)) ;
#110017=CARTESIAN_POINT('Ctrl Pts',(0.611106760396033,0.207685608831249,
-14.6677161626194)) ;
#110018=CARTESIAN_POINT('Ctrl Pts',(0.605629861308049,0.210178193248326,
-14.6786625183495)) ;
#110019=CARTESIAN_POINT('Ctrl Pts',(0.599740696039329,0.213544620665554,
-14.6904500571145)) ;
#110020=CARTESIAN_POINT('Ctrl Pts',(0.599111682766062,0.213913346521981,
-14.6917092810542)) ;
#110021=CARTESIAN_POINT('Ctrl Pts',(0.593032751351783,0.217566912232526,
-14.7038807702672)) ;
#110022=CARTESIAN_POINT('Ctrl Pts',(0.587842238429121,0.221400308602596,
-14.7142930826375)) ;
#110023=CARTESIAN_POINT('Ctrl Pts',(0.581771186964291,0.226871185484691,
-14.7264548899728)) ;
#110024=CARTESIAN_POINT('Ctrl Pts',(0.58051466706413,0.22806397669856,-14.7289706658717)) ;
#110025=CARTESIAN_POINT('Ctrl Pts',(0.579289321881328,0.229289321881363,
-14.7314213562373)) ;
#110026=CARTESIAN_POINT('Origin',(0.657142104261918,0.302990743367277,-14.5757199456745)) ;
#110027=CARTESIAN_POINT('Origin',(-1.7,4.6,-15.79)) ;
#110028=CARTESIAN_POINT('',(-1.77071067811866,4.52928932188135,-15.7485786437627)) ;
#110029=CARTESIAN_POINT('Ctrl Pts',(-1.8,4.6,-15.89)) ;
#110030=CARTESIAN_POINT('Ctrl Pts',(-1.8,4.5949171417321,-15.8798342834642)) ;
#110031=CARTESIAN_POINT('Ctrl Pts',(-1.79961031187958,4.58965768385803,
-15.8693168490805)) ;
#110032=CARTESIAN_POINT('Ctrl Pts',(-1.79783411578236,4.57846794971939,
-15.8469573347197)) ;
#110033=CARTESIAN_POINT('Ctrl Pts',(-1.79635217950657,4.57252276179498,
-15.8350867274011)) ;
#110034=CARTESIAN_POINT('Ctrl Pts',(-1.79231439116877,4.5611067603961,-15.8122838373806)) ;
#110035=CARTESIAN_POINT('Ctrl Pts',(-1.78982180675173,4.55562986130817,
-15.8013374816506)) ;
#110036=CARTESIAN_POINT('Ctrl Pts',(-1.78645537933451,4.54974069603944,
-15.7895499428856)) ;
#110037=CARTESIAN_POINT('Ctrl Pts',(-1.78608665347804,4.5491116827661,-15.7882907189457)) ;
#110038=CARTESIAN_POINT('Ctrl Pts',(-1.78243308776746,4.54303275135176,
-15.7761192297327)) ;
#110039=CARTESIAN_POINT('Ctrl Pts',(-1.7785996913974,4.53784223842911,-15.7657069173624)) ;
#110040=CARTESIAN_POINT('Ctrl Pts',(-1.77312881451532,4.5317711869643,-15.7535451100272)) ;
#110041=CARTESIAN_POINT('Ctrl Pts',(-1.77193602330145,4.53051466706415,
-15.7510293341283)) ;
#110042=CARTESIAN_POINT('Ctrl Pts',(-1.77071067811866,4.52928932188135,
-15.7485786437627)) ;
#110043=CARTESIAN_POINT('Origin',(-1.69700925664399,4.60714210423621,-15.9042800542741)) ;
#110044=CARTESIAN_POINT('',(-1.77071067811866,4.52928932188135,-14.7314213562373)) ;
#110045=CARTESIAN_POINT('Origin',(-1.69703459697175,4.60708668538575,-14.5758299049368)) ;
#110046=CARTESIAN_POINT('Ctrl Pts',(-1.77071067811866,4.52928932188135,
-14.7314213562373)) ;
#110047=CARTESIAN_POINT('Ctrl Pts',(-1.77521675558368,4.53379539934637,
-14.7224092013072)) ;
#110048=CARTESIAN_POINT('Ctrl Pts',(-1.77928079264423,4.53872648167164,
-14.7125137418271)) ;
#110049=CARTESIAN_POINT('Ctrl Pts',(-1.78624680748634,4.54902088254791,
-14.6918872294311)) ;
#110050=CARTESIAN_POINT('Ctrl Pts',(-1.78918030781805,4.55436398414935,
-14.6811949056648)) ;
#110051=CARTESIAN_POINT('Ctrl Pts',(-1.79185985500302,4.56047475453307,
-14.6689814067792)) ;
#110052=CARTESIAN_POINT('Ctrl Pts',(-1.79213045061232,4.56110970990906,
-14.6677124827727)) ;
#110053=CARTESIAN_POINT('Ctrl Pts',(-1.7947746790983,4.56749628913395,-14.6549506299714)) ;
#110054=CARTESIAN_POINT('Ctrl Pts',(-1.79657370273653,4.5733715724062,-14.643220635718)) ;
#110055=CARTESIAN_POINT('Ctrl Pts',(-1.79896007643137,4.58459577476124,
-14.620799741116)) ;
#110056=CARTESIAN_POINT('Ctrl Pts',(-1.79963010255189,4.58995007594508,
-14.6100980783183)) ;
#110057=CARTESIAN_POINT('Ctrl Pts',(-1.79996164986963,4.59678557381709,
-14.5964288396569)) ;
#110058=CARTESIAN_POINT('Ctrl Pts',(-1.8,4.5984014131596,-14.5931971736808)) ;
#110059=CARTESIAN_POINT('Ctrl Pts',(-1.8,4.6,-14.59)) ;
#110060=CARTESIAN_POINT('Origin',(-1.7,0.3,-16.64)) ;
#110061=CARTESIAN_POINT('Origin',(-1.7,0.1,-16.64)) ;
#110062=CARTESIAN_POINT('Origin',(-1.9,0.3,-16.64)) ;
#110063=CARTESIAN_POINT('Origin',(1.9668402209837E-32,0.1,-16.64)) ;
#110064=CARTESIAN_POINT('',(0.899999999999999,0.1,-16.74)) ;
#110065=CARTESIAN_POINT('',(-1.8,0.1,-16.74)) ;
#110066=CARTESIAN_POINT('Origin',(0.899999999999999,0.1,-16.64)) ;
#110067=CARTESIAN_POINT('Origin',(0.899999999999999,0.1,-16.64)) ;
#110068=CARTESIAN_POINT('',(0.999999999999999,0.1,-16.64)) ;
#110069=CARTESIAN_POINT('Origin',(0.899999999999999,0.1,-16.64)) ;
#110070=CARTESIAN_POINT('Origin',(0.899999999999999,0.1,-16.64)) ;
#110071=CARTESIAN_POINT('Origin',(0.549999999999999,0.3,-14.59)) ;
#110072=CARTESIAN_POINT('',(0.50857864376269,0.229289321881346,-14.6607106781187)) ;
#110073=CARTESIAN_POINT('Origin',(0.664170095063304,0.30296540302746,-14.5829133146142)) ;
#110074=CARTESIAN_POINT('Ctrl Pts',(0.50857864376269,0.229289321881369,
-14.6607106781187)) ;
#110075=CARTESIAN_POINT('Ctrl Pts',(0.517590798692736,0.224783244416307,
-14.6562046006536)) ;
#110076=CARTESIAN_POINT('Ctrl Pts',(0.52748625817285,0.22071920735579,-14.6512735183284)) ;
#110077=CARTESIAN_POINT('Ctrl Pts',(0.548112770567762,0.21375319251403,
-14.6409791174526)) ;
#110078=CARTESIAN_POINT('Ctrl Pts',(0.558805094332743,0.210819692182585,
-14.6356360158518)) ;
#110079=CARTESIAN_POINT('Ctrl Pts',(0.571018593218257,0.208140144997491,
-14.6295252454681)) ;
#110080=CARTESIAN_POINT('Ctrl Pts',(0.572287517225956,0.207869549387918,
-14.6288902900915)) ;
#110081=CARTESIAN_POINT('Ctrl Pts',(0.585049370028551,0.205225320901704,
-14.622503710866)) ;
#110082=CARTESIAN_POINT('Ctrl Pts',(0.596779364281985,0.20342629726345,
-14.6166284275937)) ;
#110083=CARTESIAN_POINT('Ctrl Pts',(0.619200258883932,0.201039923568639,
-14.6054042252388)) ;
#110084=CARTESIAN_POINT('Ctrl Pts',(0.629901921681571,0.200369897448121,
-14.600049924055)) ;
#110085=CARTESIAN_POINT('Ctrl Pts',(0.643571160343008,0.200038350130376,
-14.593214426183)) ;
#110086=CARTESIAN_POINT('Ctrl Pts',(0.646802826319167,0.200000000000001,
-14.5915985868404)) ;
#110087=CARTESIAN_POINT('Ctrl Pts',(0.65,0.200000000000001,-14.59)) ;
#110088=CARTESIAN_POINT('Origin',(-1.7,0.3,-14.59)) ;
#110089=CARTESIAN_POINT('Origin',(-1.7,4.5,-14.59)) ;
#110090=CARTESIAN_POINT('',(-1.77071067811864,4.45857864376273,-14.6607106781187)) ;
#110091=CARTESIAN_POINT('Ctrl Pts',(-1.8,4.6,-14.59)) ;
#110092=CARTESIAN_POINT('Ctrl Pts',(-1.8,4.58983428346416,-14.5950828582679)) ;
#110093=CARTESIAN_POINT('Ctrl Pts',(-1.79961031187958,4.57931684908054,
-14.600342316142)) ;
#110094=CARTESIAN_POINT('Ctrl Pts',(-1.79783411578235,4.5569573347197,-14.6115320502807)) ;
#110095=CARTESIAN_POINT('Ctrl Pts',(-1.79635217950654,4.54508672740115,
-14.6174772382051)) ;
#110096=CARTESIAN_POINT('Ctrl Pts',(-1.79231439116922,4.52228383738327,
-14.6288932396026)) ;
#110097=CARTESIAN_POINT('Ctrl Pts',(-1.7898218067529,4.51133748165596,-14.6343701386892)) ;
#110098=CARTESIAN_POINT('Ctrl Pts',(-1.78645537933596,4.49954994289065,
-14.6402593039581)) ;
#110099=CARTESIAN_POINT('Ctrl Pts',(-1.78608665347877,4.49829071894828,
-14.6408883172327)) ;
#110100=CARTESIAN_POINT('Ctrl Pts',(-1.78243308776744,4.48611922973267,
-14.6469672486483)) ;
#110101=CARTESIAN_POINT('Ctrl Pts',(-1.77859969139738,4.4757069173624,-14.6521577615709)) ;
#110102=CARTESIAN_POINT('Ctrl Pts',(-1.7731288145153,4.46354511002718,-14.6582288130357)) ;
#110103=CARTESIAN_POINT('Ctrl Pts',(-1.77193602330142,4.4610293341283,-14.6594853329359)) ;
#110104=CARTESIAN_POINT('Ctrl Pts',(-1.77071067811862,4.45857864376273,
-14.6607106781187)) ;
#110105=CARTESIAN_POINT('Origin',(-1.69700925663777,4.6142800543045,-14.5828578957488)) ;
#110106=CARTESIAN_POINT('Origin',(-1.7,0.3,-14.59)) ;
#110107=CARTESIAN_POINT('Origin',(-1.9,-4.11004745125224E-16,-16.64)) ;
#110108=CARTESIAN_POINT('',(-1.9,6.9,-16.74)) ;
#110109=CARTESIAN_POINT('Origin',(-1.9,6.9,-16.64)) ;
#110110=CARTESIAN_POINT('',(-1.9,7.,-16.74)) ;
#110111=CARTESIAN_POINT('Origin',(-2.,0.1,-16.84)) ;
#110112=CARTESIAN_POINT('Origin',(-1.89999999999978,0.100000000000219,-16.8400000000002)) ;
#110113=CARTESIAN_POINT('Origin',(0.899999999999999,0.1,-16.84)) ;
#110114=CARTESIAN_POINT('Origin',(0.899999999999999,0.1,-16.64)) ;
#110115=CARTESIAN_POINT('Origin',(1.1,0.1,-16.64)) ;
#110116=CARTESIAN_POINT('Origin',(0.899999999999999,0.1,-15.24)) ;
#110117=CARTESIAN_POINT('',(0.999999999999999,0.1,-13.84)) ;
#110118=CARTESIAN_POINT('',(0.999999999999999,0.1,-16.74)) ;
#110119=CARTESIAN_POINT('Origin',(0.899999999999999,0.1,-13.84)) ;
#110120=CARTESIAN_POINT('Origin',(-1.7,0.3,-14.59)) ;
#110121=CARTESIAN_POINT('Origin',(-1.7,0.3,-14.59)) ;
#110122=CARTESIAN_POINT('Origin',(-1.9,6.9,-16.64)) ;
#110123=CARTESIAN_POINT('',(-1.9,7.,-16.64)) ;
#110124=CARTESIAN_POINT('Origin',(-1.9,6.9,-16.64)) ;
#110125=CARTESIAN_POINT('Origin',(-1.9,6.9,-16.64)) ;
#110126=CARTESIAN_POINT('Origin',(-1.9,7.,-16.84)) ;
#110127=CARTESIAN_POINT('Origin',(-1.9,6.9,-16.84)) ;
#110128=CARTESIAN_POINT('Origin',(1.1,0.1,-13.74)) ;
#110129=CARTESIAN_POINT('Origin',(1.1,0.1,-13.84)) ;
#110130=CARTESIAN_POINT('Origin',(0.899999999999999,0.1,-13.84)) ;
#110131=CARTESIAN_POINT('',(0.899999999999999,0.1,-13.74)) ;
#110132=CARTESIAN_POINT('Origin',(0.899999999999999,0.1,-13.84)) ;
#110133=CARTESIAN_POINT('Origin',(0.899999999999999,0.1,-13.84)) ;
#110134=CARTESIAN_POINT('Origin',(-1.7,0.3,-15.24)) ;
#110135=CARTESIAN_POINT('Origin',(-1.7,0.3,-13.84)) ;
#110136=CARTESIAN_POINT('Origin',(-1.9,6.9,-15.24)) ;
#110137=CARTESIAN_POINT('',(-1.9,7.,-13.84)) ;
#110138=CARTESIAN_POINT('Origin',(-1.9,6.9,-13.84)) ;
#110139=CARTESIAN_POINT('',(-1.9,7.,-16.74)) ;
#110140=CARTESIAN_POINT('Origin',(-1.9,6.9,-16.64)) ;
#110141=CARTESIAN_POINT('Origin',(-1.9,7.1,-16.64)) ;
#110142=CARTESIAN_POINT('Origin',(0.899999999999999,0.1,-13.84)) ;
#110143=CARTESIAN_POINT('Origin',(0.899999999999999,0.1,-13.64)) ;
#110144=CARTESIAN_POINT('Origin',(-1.9668402209837E-32,0.1,-13.84)) ;
#110145=CARTESIAN_POINT('',(0.999999999999999,0.1,-13.74)) ;
#110146=CARTESIAN_POINT('Origin',(-1.7,0.1,-13.84)) ;
#110147=CARTESIAN_POINT('Origin',(-1.7,0.3,-13.84)) ;
#110148=CARTESIAN_POINT('Origin',(-1.9,0.3,-13.84)) ;
#110149=CARTESIAN_POINT('Origin',(-1.9,6.9,-13.84)) ;
#110150=CARTESIAN_POINT('',(-1.9,6.9,-13.74)) ;
#110151=CARTESIAN_POINT('Origin',(-1.9,6.9,-13.84)) ;
#110152=CARTESIAN_POINT('Origin',(-1.9,6.9,-13.84)) ;
#110153=CARTESIAN_POINT('Origin',(-1.9,7.1,-16.74)) ;
#110154=CARTESIAN_POINT('Origin',(-1.9,7.1,-13.84)) ;
#110155=CARTESIAN_POINT('Origin',(-1.8,0.1,-13.64)) ;
#110156=CARTESIAN_POINT('Origin',(-1.90000000000006,0.0999999999999441,
-13.6400000000001)) ;
#110157=CARTESIAN_POINT('Origin',(-1.9,-6.40600499298624E-17,-13.84)) ;
#110158=CARTESIAN_POINT('',(-1.9,7.,-13.74)) ;
#110159=CARTESIAN_POINT('Origin',(-1.9,6.9,-13.84)) ;
#110160=CARTESIAN_POINT('Origin',(-1.9,6.9,-13.64)) ;
#110161=CARTESIAN_POINT('Origin',(-1.9,7.,-13.64)) ;
#110162=CARTESIAN_POINT('Origin',(-0.900000000000002,2.95,-15.24)) ;
#110163=CARTESIAN_POINT('Origin',(-0.900000000000001,2.95,-16.8831676725155)) ;
#110164=CARTESIAN_POINT('Origin',(-0.900000000000002,2.95,-16.8831676725155)) ;
#110165=CARTESIAN_POINT('Origin',(-0.900000000000001,2.95,-16.8831676725155)) ;
#110166=CARTESIAN_POINT('Origin',(-0.900000000000002,2.95,-16.8831676725155)) ;
#110167=CARTESIAN_POINT('Origin',(1.15,3.15,-17.79)) ;
#110168=CARTESIAN_POINT('Origin',(1.15,3.15,-16.8831676725155)) ;
#110169=CARTESIAN_POINT('Origin',(-1.,2.95,-16.8831676725155)) ;
#110170=CARTESIAN_POINT('Origin',(1.15,2.95,-16.8831676725155)) ;
#110171=CARTESIAN_POINT('Origin',(-0.900000000000001,3.8,-15.24)) ;
#110172=CARTESIAN_POINT('Origin',(-0.900000000000002,2.1568323274845,-16.09)) ;
#110173=CARTESIAN_POINT('Origin',(-0.900000000000002,1.6,-15.24)) ;
#110174=CARTESIAN_POINT('Origin',(-0.900000000000002,1.6,-17.2021416870349)) ;
#110175=CARTESIAN_POINT('Origin',(13.9153543900904,1.4,-17.2021416870349)) ;
#110176=CARTESIAN_POINT('Origin',(8.49172374697002,1.4,-17.2021416870349)) ;
#110177=CARTESIAN_POINT('Origin',(-0.900000000000001,1.40000000000001,-17.2021416870349)) ;
#110178=CARTESIAN_POINT('Origin',(1.15,2.95,-16.8831676725155)) ;
#110179=CARTESIAN_POINT('Origin',(1.15,3.04189189189189,-16.7055279241354)) ;
#110180=CARTESIAN_POINT('Origin',(-0.900000000000002,2.1568323274845,-16.09)) ;
#110181=CARTESIAN_POINT('Origin',(-0.900000000000002,2.1568323274845,-16.09)) ;
#110182=CARTESIAN_POINT('Origin',(-0.900000000000002,2.1568323274845,-16.09)) ;
#110183=CARTESIAN_POINT('Origin',(-0.900000000000001,1.40000000000001,-17.2021416870349)) ;
#110184=CARTESIAN_POINT('Origin',(-0.900000000000002,1.55483870967742,-17.0755519007745)) ;
#110185=CARTESIAN_POINT('Origin',(1.15,3.8,-15.24)) ;
#110186=CARTESIAN_POINT('Origin',(1.15,2.33447207586456,-15.9981081081081)) ;
#110187=CARTESIAN_POINT('Origin',(-1.,2.1568323274845,-16.09)) ;
#110188=CARTESIAN_POINT('Origin',(1.15,2.1568323274845,-16.09)) ;
#110189=CARTESIAN_POINT('Origin',(-0.900000000000001,3.8,-16.09)) ;
#110190=CARTESIAN_POINT('Origin',(-0.900000000000002,1.02736587339765,-16.09)) ;
#110191=CARTESIAN_POINT('Origin',(-0.900000000000001,3.8,-15.24)) ;
#110192=CARTESIAN_POINT('Origin',(-0.900000000000002,1.02736587339765,-16.09)) ;
#110193=CARTESIAN_POINT('Origin',(13.9153543900904,1.4,-13.2778583129651)) ;
#110194=CARTESIAN_POINT('Origin',(8.49172374697002,1.4,-13.2778583129651)) ;
#110195=CARTESIAN_POINT('Origin',(-0.900000000000001,1.40000000000001,-13.2778583129651)) ;
#110196=CARTESIAN_POINT('Origin',(-0.900000000000002,1.6,-15.24)) ;
#110197=CARTESIAN_POINT('Origin',(-0.900000000000002,1.6,-13.2778583129651)) ;
#110198=CARTESIAN_POINT('Origin',(-0.900000000000002,2.95,-15.24)) ;
#110199=CARTESIAN_POINT('Origin',(-0.900000000000002,2.95,-13.5968323274845)) ;
#110200=CARTESIAN_POINT('Origin',(1.15,2.1568323274845,-16.09)) ;
#110201=CARTESIAN_POINT('Origin',(1.15,2.1568323274845,-15.89)) ;
#110202=CARTESIAN_POINT('Origin',(-0.900000000000002,1.02736587339765,-16.09)) ;
#110203=CARTESIAN_POINT('Origin',(-0.900000000000001,1.40000000000001,-13.2778583129651)) ;
#110204=CARTESIAN_POINT('Origin',(-0.900000000000002,1.55483870967743,-13.4044480992254)) ;
#110205=CARTESIAN_POINT('Origin',(-0.900000000000002,2.95,-13.5968323274845)) ;
#110206=CARTESIAN_POINT('Origin',(-0.900000000000002,2.95,-13.5968323274845)) ;
#110207=CARTESIAN_POINT('Origin',(-0.900000000000001,2.95,-13.5968323274845)) ;
#110208=CARTESIAN_POINT('Origin',(1.15,2.21886116991581,-15.89)) ;
#110209=CARTESIAN_POINT('Ctrl Pts',(1.15,1.02736587339765,-15.99)) ;
#110210=CARTESIAN_POINT('Ctrl Pts',(1.1608920328805,1.02736587339765,-15.99)) ;
#110211=CARTESIAN_POINT('Ctrl Pts',(1.17195716626105,1.02622125393927,-15.988143843926)) ;
#110212=CARTESIAN_POINT('Ctrl Pts',(1.1820844490224,1.02414637334385,-15.9847131887908)) ;
#110213=CARTESIAN_POINT('Ctrl Pts',(1.19245005921088,1.02202266415684,-15.9812017993431)) ;
#110214=CARTESIAN_POINT('Ctrl Pts',(1.20216743701154,1.01888103823701,-15.9759601980703)) ;
#110215=CARTESIAN_POINT('Ctrl Pts',(1.21053792402812,1.01518120925307,-15.969593716802)) ;
#110216=CARTESIAN_POINT('Ctrl Pts',(1.219343173684,1.01128921135341,-15.9628965608439)) ;
#110217=CARTESIAN_POINT('Ctrl Pts',(1.22692289939014,1.00668521903338,-15.9547851615315)) ;
#110218=CARTESIAN_POINT('Ctrl Pts',(1.23290049538659,1.00186003905466,-15.9459241259624)) ;
#110219=CARTESIAN_POINT('Ctrl Pts',(1.23922345568944,0.9967560772818,-15.93655113117)) ;
#110220=CARTESIAN_POINT('Ctrl Pts',(1.24392209779927,0.991279542094837,
-15.9261045599897)) ;
#110221=CARTESIAN_POINT('Ctrl Pts',(1.24674870216524,0.985895902333124,
-15.9152920665297)) ;
#110222=CARTESIAN_POINT('Ctrl Pts',(1.24889292215336,0.981811953364218,
-15.9070898699727)) ;
#110223=CARTESIAN_POINT('Ctrl Pts',(1.25,0.977715885027402,-15.8985491686292)) ;
#110224=CARTESIAN_POINT('Ctrl Pts',(1.25,0.973783447787483,-15.89)) ;
#110225=CARTESIAN_POINT('Origin',(-0.900000000000001,3.8,-15.24)) ;
#110226=CARTESIAN_POINT('Origin',(-0.900000000000002,1.02736587339765,-14.39)) ;
#110227=CARTESIAN_POINT('Origin',(-0.900000000000001,3.8,-14.39)) ;
#110228=CARTESIAN_POINT('Origin',(-0.900000000000002,2.1568323274845,-14.39)) ;
#110229=CARTESIAN_POINT('Origin',(-0.900000000000002,1.02736587339765,-14.39)) ;
#110230=CARTESIAN_POINT('Origin',(-0.900000000000001,3.8,-15.24)) ;
#110231=CARTESIAN_POINT('Origin',(-0.900000000000002,2.1568323274845,-14.39)) ;
#110232=CARTESIAN_POINT('Origin',(-1.,2.95,-13.5968323274845)) ;
#110233=CARTESIAN_POINT('Origin',(1.15,2.95,-13.5968323274845)) ;
#110234=CARTESIAN_POINT('Origin',(1.15,3.15,-12.69)) ;
#110235=CARTESIAN_POINT('Origin',(1.15,3.15,-13.5968323274845)) ;
#110236=CARTESIAN_POINT('Ctrl Pts',(1.11028558574901,0.930383836951479,
-16.1149942836582)) ;
#110237=CARTESIAN_POINT('Ctrl Pts',(1.14039000477524,0.89213646613791,-15.989969718594)) ;
#110238=CARTESIAN_POINT('Ctrl Pts',(1.13015013463564,1.02610337426268,-15.9878511248827)) ;
#110239=CARTESIAN_POINT('Ctrl Pts',(1.17639690652713,0.93522510982765,-16.1301257399467)) ;
#110240=CARTESIAN_POINT('Ctrl Pts',(1.15491086542928,0.891146666106907,
-15.9892760504014)) ;
#110241=CARTESIAN_POINT('Ctrl Pts',(1.16319405445819,1.03078047702079,-15.9951648742452)) ;
#110242=CARTESIAN_POINT('Ctrl Pts',(1.24701363206612,0.927145283841805,
-16.1055522038251)) ;
#110243=CARTESIAN_POINT('Ctrl Pts',(1.17759980831447,0.893467326853923,
-15.9926373120314)) ;
#110244=CARTESIAN_POINT('Ctrl Pts',(1.19848758201044,1.02297467453101,-15.983287122555)) ;
#110245=CARTESIAN_POINT('Ctrl Pts',(1.33816236560056,0.900022463714239,
-16.0098088506149)) ;
#110246=CARTESIAN_POINT('Ctrl Pts',(1.22862786282606,0.888037626604014,
-15.963153964324)) ;
#110247=CARTESIAN_POINT('Ctrl Pts',(1.24403288504499,0.996768276947748,
-15.9370266594133)) ;
#110248=CARTESIAN_POINT('Ctrl Pts',(1.35959492575597,0.881455895025368,
-15.938532341229)) ;
#110249=CARTESIAN_POINT('Ctrl Pts',(1.25320519750665,0.88042809908173,-15.9310649378274)) ;
#110250=CARTESIAN_POINT('Ctrl Pts',(1.25473603279823,0.978811277328846,
-15.9025574871508)) ;
#110251=CARTESIAN_POINT('Ctrl Pts',(1.34615355831624,0.867571605181224,
-15.8727925825335)) ;
#110252=CARTESIAN_POINT('Ctrl Pts',(1.2517609020281,0.870950130624643,-15.8894490170578)) ;
#110253=CARTESIAN_POINT('Ctrl Pts',(1.24801589497573,0.965423101361847,
-15.8708695481641)) ;
#110254=CARTESIAN_POINT('Origin',(1.35,0.973783447787483,-15.89)) ;
#110255=CARTESIAN_POINT('Origin',(-0.900000000000002,1.02736587339765,-14.39)) ;
#110256=CARTESIAN_POINT('',(-0.957735026918965,0.969630846478687,-14.447735026919)) ;
#110257=CARTESIAN_POINT('Origin',(-0.900000000000002,1.02736587339765,-14.39)) ;
#110258=CARTESIAN_POINT('Origin',(-0.900000000000002,2.1568323274845,-14.39)) ;
#110259=CARTESIAN_POINT('Origin',(-0.900000000000002,2.1568323274845,-14.39)) ;
#110260=CARTESIAN_POINT('Origin',(1.15,2.95,-13.5968323274845)) ;
#110261=CARTESIAN_POINT('Origin',(1.15,3.04189189189189,-13.7744720758646)) ;
#110262=CARTESIAN_POINT('Origin',(1.35,3.8,-15.24)) ;
#110263=CARTESIAN_POINT('Origin',(1.35,0.973783447787484,-14.59)) ;
#110264=CARTESIAN_POINT('Origin',(-1.,2.1568323274845,-14.39)) ;
#110265=CARTESIAN_POINT('Origin',(1.15,2.1568323274845,-14.39)) ;
#110266=CARTESIAN_POINT('Origin',(1.15,3.8,-15.24)) ;
#110267=CARTESIAN_POINT('Origin',(1.15,2.33447207586456,-14.4818918918919)) ;
#110268=CARTESIAN_POINT('Ctrl Pts',(1.34754079198594,0.869159571293157,
-14.5997485347855)) ;
#110269=CARTESIAN_POINT('Ctrl Pts',(1.25183398383325,0.87199977042434,-14.5859986517604)) ;
#110270=CARTESIAN_POINT('Ctrl Pts',(1.24871534599026,0.966951450593922,
-14.6055357130736)) ;
#110271=CARTESIAN_POINT('Ctrl Pts',(1.3578897130187,0.882932151572343,-14.5357774282681)) ;
#110272=CARTESIAN_POINT('Ctrl Pts',(1.25138796519083,0.881019151005405,
-14.5464872814236)) ;
#110273=CARTESIAN_POINT('Ctrl Pts',(1.25389076424432,0.980237216252324,
-14.5746886342594)) ;
#110274=CARTESIAN_POINT('Ctrl Pts',(1.33642796493171,0.90055164307479,-14.4683167189688)) ;
#110275=CARTESIAN_POINT('Ctrl Pts',(1.22773025960896,0.888154519889406,
-14.5163023541524)) ;
#110276=CARTESIAN_POINT('Ctrl Pts',(1.24317203399028,0.99727835245108,-14.5420644582831)) ;
#110277=CARTESIAN_POINT('Ctrl Pts',(1.24851212064762,0.926675670999743,
-14.3761118541866)) ;
#110278=CARTESIAN_POINT('Ctrl Pts',(1.17855408504648,0.893378082604318,
-14.4879358454001)) ;
#110279=CARTESIAN_POINT('Ctrl Pts',(1.19923947710882,1.02252144543593,-14.4975111840607)) ;
#110280=CARTESIAN_POINT('Ctrl Pts',(1.18212686068543,0.934567888698249,
-14.3518922599008)) ;
#110281=CARTESIAN_POINT('Ctrl Pts',(1.15690947476175,0.891342319659322,
-14.4905013022392)) ;
#110282=CARTESIAN_POINT('Ctrl Pts',(1.1660589236879,1.03014681530415,-14.4858041235204)) ;
#110283=CARTESIAN_POINT('Ctrl Pts',(1.11776263740948,0.930888708579174,
-14.363423581916)) ;
#110284=CARTESIAN_POINT('Ctrl Pts',(1.1419771056359,0.892059806626674,-14.4900822996554)) ;
#110285=CARTESIAN_POINT('Ctrl Pts',(1.13388624958143,1.02659206201255,-14.4913778561013)) ;
#110286=CARTESIAN_POINT('Ctrl Pts',(1.15,1.02736587339764,-14.49)) ;
#110287=CARTESIAN_POINT('Ctrl Pts',(1.15623005440502,1.02736587339759,-14.4899999999999)) ;
#110288=CARTESIAN_POINT('Ctrl Pts',(1.16249579431471,1.02700282517053,-14.490590866069)) ;
#110289=CARTESIAN_POINT('Ctrl Pts',(1.16857840195431,1.02630083270769,-14.4917409394467)) ;
#110290=CARTESIAN_POINT('Ctrl Pts',(1.1798885498395,1.02499553092934,-14.4938794137247)) ;
#110291=CARTESIAN_POINT('Ctrl Pts',(1.19084787809767,1.02245621903271,-14.4980506966152)) ;
#110292=CARTESIAN_POINT('Ctrl Pts',(1.20043335385463,1.01914369852331,-14.5036491064379)) ;
#110293=CARTESIAN_POINT('Ctrl Pts',(1.21063893018497,1.01561688548223,-14.5096096868225)) ;
#110294=CARTESIAN_POINT('Ctrl Pts',(1.21965078109605,1.01112191387731,-14.5173548511019)) ;
#110295=CARTESIAN_POINT('Ctrl Pts',(1.226898722009,1.00626683908294,-14.5260735848543)) ;
#110296=CARTESIAN_POINT('Ctrl Pts',(1.23435386869391,1.0012729663137,-14.5350415717366)) ;
#110297=CARTESIAN_POINT('Ctrl Pts',(1.24017476602864,0.995763540409855,
-14.5452870264069)) ;
#110298=CARTESIAN_POINT('Ctrl Pts',(1.24405759382605,0.990267693778535,
-14.5560416572305)) ;
#110299=CARTESIAN_POINT('Ctrl Pts',(1.24795610732226,0.9847496452368,-14.5668397341991)) ;
#110300=CARTESIAN_POINT('Ctrl Pts',(1.25,0.97910634898267,-14.578427945028)) ;
#110301=CARTESIAN_POINT('Ctrl Pts',(1.25,0.973783447787483,-14.59)) ;
#110302=CARTESIAN_POINT('Origin',(1.15,2.1568323274845,-14.39)) ;
#110303=CARTESIAN_POINT('Origin',(1.15,2.1568323274845,-14.59)) ;
#110304=CARTESIAN_POINT('Origin',(1.15,2.21886116991581,-14.59)) ;
#110305=CARTESIAN_POINT('Origin',(1.5,2.3,-15.64)) ;
#110306=CARTESIAN_POINT('Ctrl Pts',(0.549999999999999,4.04473197180487,
-15.69)) ;
#110307=CARTESIAN_POINT('Ctrl Pts',(0.549999999999999,4.04340510574362,
-15.6920183916746)) ;
#110308=CARTESIAN_POINT('Ctrl Pts',(0.549938912488053,4.04197482121869,
-15.6939799093558)) ;
#110309=CARTESIAN_POINT('Ctrl Pts',(0.549362579613731,4.03414945156067,
-15.7037632016969)) ;
#110310=CARTESIAN_POINT('Ctrl Pts',(0.548040652125111,4.02633974827563,
-15.7105458262271)) ;
#110311=CARTESIAN_POINT('Ctrl Pts',(0.544205267183641,4.00519499286858,
-15.7246839427888)) ;
#110312=CARTESIAN_POINT('Ctrl Pts',(0.541221332378522,3.99011995637991,
-15.7312251154481)) ;
#110313=CARTESIAN_POINT('Ctrl Pts',(0.537814556431575,3.96385893187674,
-15.73793059224)) ;
#110314=CARTESIAN_POINT('Ctrl Pts',(0.536602540378442,3.95132390702861,
-15.74)) ;
#110315=CARTESIAN_POINT('Ctrl Pts',(0.536602540378442,3.93764017256378,
-15.74)) ;
#110316=CARTESIAN_POINT('Origin',(-0.4,2.3,-15.64)) ;
#110317=CARTESIAN_POINT('Origin',(-0.4,-3.4,-15.64)) ;
#110318=CARTESIAN_POINT('Origin',(-0.4,-3.36847777691809,-15.64)) ;
#110319=CARTESIAN_POINT('Origin',(1.5,2.3,-15.64)) ;
#110320=CARTESIAN_POINT('Ctrl Pts',(0.536602540378442,2.83090991212703,
-15.74)) ;
#110321=CARTESIAN_POINT('Ctrl Pts',(0.536602540378442,2.80627146475495,
-15.74)) ;
#110322=CARTESIAN_POINT('Ctrl Pts',(0.538106903229178,2.77742679387655,
-15.7379527908126)) ;
#110323=CARTESIAN_POINT('Ctrl Pts',(0.545186976568879,2.71156844363324,
-15.72208398098)) ;
#110324=CARTESIAN_POINT('Ctrl Pts',(0.549999999999999,2.68282906082667,
-15.7081020558136)) ;
#110325=CARTESIAN_POINT('Ctrl Pts',(0.549999999999999,2.65280931275608,
-15.69)) ;
#110326=CARTESIAN_POINT('Origin',(0.400000000000001,2.29999999999999,-15.64)) ;
#110327=CARTESIAN_POINT('Origin',(0.0725078566451197,-4.04348900069683,
-15.1674921433549)) ;
#110328=CARTESIAN_POINT('Origin',(-0.4,-3.36847777691809,-15.64)) ;
#110329=CARTESIAN_POINT('Origin',(-0.0979344438426628,-3.8,-15.3379344438427)) ;
#110330=CARTESIAN_POINT('Origin',(1.5,2.3,-14.84)) ;
#110331=CARTESIAN_POINT('Ctrl Pts',(0.536602540378443,3.93764017256378,
-14.74)) ;
#110332=CARTESIAN_POINT('Ctrl Pts',(0.536602540378443,3.93925361219667,
-14.74)) ;
#110333=CARTESIAN_POINT('Ctrl Pts',(0.536619300889436,3.94087098264022,
-14.7400289972578)) ;
#110334=CARTESIAN_POINT('Ctrl Pts',(0.536997639747737,3.95938954612103,
-14.7406858128958)) ;
#110335=CARTESIAN_POINT('Ctrl Pts',(0.539142315171097,3.97567120869923,
-14.7443120615617)) ;
#110336=CARTESIAN_POINT('Ctrl Pts',(0.544035197036717,4.00535605098116,
-14.7553993916662)) ;
#110337=CARTESIAN_POINT('Ctrl Pts',(0.546989816174457,4.01946236900627,
-14.7635699446351)) ;
#110338=CARTESIAN_POINT('Ctrl Pts',(0.549463062495699,4.0359553600741,-14.7785473816972)) ;
#110339=CARTESIAN_POINT('Ctrl Pts',(0.550000000000877,4.04078397701437,
-14.7839944203464)) ;
#110340=CARTESIAN_POINT('Ctrl Pts',(0.549999999999999,4.04473197181447,
-14.7900000000146)) ;
#110341=CARTESIAN_POINT('Origin',(-0.4,2.3,-14.84)) ;
#110342=CARTESIAN_POINT('Origin',(0.4,2.29999999999999,-15.64)) ;
#110343=CARTESIAN_POINT('Origin',(0.4,-3.36847777691809,-15.64)) ;
#110344=CARTESIAN_POINT('Origin',(-0.0979344438426628,-3.8,-15.3379344438427)) ;
#110345=CARTESIAN_POINT('Origin',(-0.0979344438426628,-3.8,-15.3379344438427)) ;
#110346=CARTESIAN_POINT('Origin',(-0.0979344438426627,-3.8,-15.3379344438427)) ;
#110347=CARTESIAN_POINT('Origin',(-0.4,2.3,-14.84)) ;
#110348=CARTESIAN_POINT('Origin',(-0.4,-3.36847777691809,-14.84)) ;
#110349=CARTESIAN_POINT('Origin',(0.190875981738719,-3.6672263744342,-15.4308759817387)) ;
#110350=CARTESIAN_POINT('Origin',(0.400000000000001,-3.36847777691809,-15.64)) ;
#110351=CARTESIAN_POINT('Origin',(0.0979344438426626,-3.8,-15.3379344438427)) ;
#110352=CARTESIAN_POINT('Origin',(0.15,-3.8,-15.3379344438427)) ;
#110353=CARTESIAN_POINT('Origin',(0.0979344438426627,-3.8,-15.3379344438427)) ;
#110354=CARTESIAN_POINT('Origin',(-0.0979344438426628,-3.8,-14.74)) ;
#110355=CARTESIAN_POINT('Origin',(-0.0979344438426628,-3.8,-15.1420655561573)) ;
#110356=CARTESIAN_POINT('Origin',(-0.174966890829628,-3.68995364716148,
-15.0650331091704)) ;
#110357=CARTESIAN_POINT('Origin',(-0.400000000000001,-3.36847777691809,
-14.84)) ;
#110358=CARTESIAN_POINT('Origin',(-0.0979344438426627,-3.8,-15.1420655561573)) ;
#110359=CARTESIAN_POINT('Origin',(0.0979344438426627,-3.8,-15.3379344438427)) ;
#110360=CARTESIAN_POINT('Origin',(0.0979344438426628,-3.8,-15.3379344438427)) ;
#110361=CARTESIAN_POINT('Origin',(-0.0979344438426628,-3.8,-15.1420655561573)) ;
#110362=CARTESIAN_POINT('Origin',(-0.0979344438426628,-3.8,-15.1420655561573)) ;
#110363=CARTESIAN_POINT('Origin',(0.0979344438426627,-3.8,-14.74)) ;
#110364=CARTESIAN_POINT('Origin',(0.0979344438426627,-3.8,-15.1420655561573)) ;
#110365=CARTESIAN_POINT('Origin',(-1.11032778078669,-3.8,-15.1420655561573)) ;
#110366=CARTESIAN_POINT('Origin',(0.0979344438426626,-3.8,-15.1420655561573)) ;
#110367=CARTESIAN_POINT('Origin',(0.0979344438426627,-3.8,-15.1420655561573)) ;
#110368=CARTESIAN_POINT('Origin',(0.0979344438426627,-3.8,-15.1420655561573)) ;
#110369=CARTESIAN_POINT('Origin',(0.438350729213467,-3.31369102089885,-14.8016492707865)) ;
#110370=CARTESIAN_POINT('Origin',(0.399999999999999,-3.36847777691809,-14.84)) ;
#110371=CARTESIAN_POINT('Origin',(0.4,2.3,-14.84)) ;
#110372=CARTESIAN_POINT('Origin',(0.4,-3.36847777691809,-14.84)) ;
#110373=CARTESIAN_POINT('Origin',(0.4,2.29999999999999,-14.84)) ;
#110374=CARTESIAN_POINT('Origin',(1.5,2.3,-14.84)) ;
#110375=CARTESIAN_POINT('Ctrl Pts',(0.55,2.65280931275593,-14.7900000000001)) ;
#110376=CARTESIAN_POINT('Ctrl Pts',(0.550000000000012,2.67648433237896,
-14.7757238466627)) ;
#110377=CARTESIAN_POINT('Ctrl Pts',(0.546908864252792,2.69988533923259,
-14.7635257008476)) ;
#110378=CARTESIAN_POINT('Ctrl Pts',(0.539540151921449,2.76165254733703,
-14.7440915981901)) ;
#110379=CARTESIAN_POINT('Ctrl Pts',(0.536602540378443,2.79600904778111,
-14.74)) ;
#110380=CARTESIAN_POINT('Ctrl Pts',(0.536602540378443,2.83090991212703,
-14.74)) ;
#110381=CARTESIAN_POINT('Origin',(8.,3.4,-15.64)) ;
#110382=CARTESIAN_POINT('Origin',(7.96847777691809,3.4,-15.64)) ;
#110383=CARTESIAN_POINT('Origin',(1.5,4.2,-15.64)) ;
#110384=CARTESIAN_POINT('Origin',(7.96847777691809,4.2,-15.64)) ;
#110385=CARTESIAN_POINT('Origin',(8.64348900069683,3.87250785664512,-15.1674921433549)) ;
#110386=CARTESIAN_POINT('Origin',(7.96847777691809,3.4,-15.64)) ;
#110387=CARTESIAN_POINT('Origin',(8.4,3.70206555615734,-15.3379344438427)) ;
#110388=CARTESIAN_POINT('Origin',(8.26722637443421,3.99087598173872,-15.4308759817387)) ;
#110389=CARTESIAN_POINT('Origin',(7.96847777691809,4.2,-15.64)) ;
#110390=CARTESIAN_POINT('Origin',(8.4,3.89793444384266,-15.3379344438427)) ;
#110391=CARTESIAN_POINT('Origin',(8.4,3.95,-15.3379344438427)) ;
#110392=CARTESIAN_POINT('Origin',(8.4,3.70206555615734,-15.3379344438427)) ;
#110393=CARTESIAN_POINT('Origin',(8.4,3.89793444384266,-15.3379344438427)) ;
#110394=CARTESIAN_POINT('Origin',(8.4,3.70206555615734,-15.3379344438427)) ;
#110395=CARTESIAN_POINT('Origin',(8.4,3.70206555615734,-15.3379344438427)) ;
#110396=CARTESIAN_POINT('Origin',(1.5,3.4,-14.84)) ;
#110397=CARTESIAN_POINT('Origin',(7.96847777691809,3.4,-14.84)) ;
#110398=CARTESIAN_POINT('Origin',(1.5,4.2,-14.84)) ;
#110399=CARTESIAN_POINT('Origin',(7.96847777691809,4.2,-14.84)) ;
#110400=CARTESIAN_POINT('Origin',(8.4,3.89793444384266,-15.3379344438427)) ;
#110401=CARTESIAN_POINT('Origin',(8.4,3.89793444384266,-15.3379344438427)) ;
#110402=CARTESIAN_POINT('Origin',(8.4,3.70206555615734,-14.74)) ;
#110403=CARTESIAN_POINT('Origin',(8.4,3.70206555615734,-15.1420655561573)) ;
#110404=CARTESIAN_POINT('Origin',(8.28995364716148,3.62503310917037,-15.0650331091704)) ;
#110405=CARTESIAN_POINT('Origin',(7.96847777691809,3.4,-14.84)) ;
#110406=CARTESIAN_POINT('Origin',(8.4,3.70206555615734,-15.1420655561573)) ;
#110407=CARTESIAN_POINT('Origin',(7.91369102089885,4.23835072921347,-14.8016492707865)) ;
#110408=CARTESIAN_POINT('Origin',(7.96847777691809,4.2,-14.84)) ;
#110409=CARTESIAN_POINT('Origin',(8.4,3.89793444384266,-15.1420655561573)) ;
#110410=CARTESIAN_POINT('Origin',(8.4,3.89793444384266,-14.74)) ;
#110411=CARTESIAN_POINT('Origin',(8.4,3.89793444384266,-15.1420655561573)) ;
#110412=CARTESIAN_POINT('Origin',(8.4,3.70206555615734,-15.1420655561573)) ;
#110413=CARTESIAN_POINT('Origin',(8.4,3.70206555615734,-15.1420655561573)) ;
#110414=CARTESIAN_POINT('Origin',(8.4,3.89793444384266,-15.1420655561573)) ;
#110415=CARTESIAN_POINT('Origin',(8.4,3.89793444384266,-15.1420655561573)) ;
#110416=CARTESIAN_POINT('Origin',(8.4,2.68967221921331,-15.1420655561573)) ;
#110417=CARTESIAN_POINT('Origin',(9.9,6.8847127088383,-17.78)) ;
#110418=CARTESIAN_POINT('Origin',(9.9,6.8847127088383,-16.1997127088383)) ;
#110419=CARTESIAN_POINT('Origin',(8.77035388141948,6.69643835574155,-16.0114383557416)) ;
#110420=CARTESIAN_POINT('Ctrl Pts',(8.58356010126946,6.66256607592812,-15.878926683545)) ;
#110421=CARTESIAN_POINT('Ctrl Pts',(8.58266714977878,6.65676189123867,-15.8787778582965)) ;
#110422=CARTESIAN_POINT('Ctrl Pts',(8.58182526931893,6.65077142220909,-15.8791141714741)) ;
#110423=CARTESIAN_POINT('Ctrl Pts',(8.58032528754329,6.63886560514777,-15.8809127350998)) ;
#110424=CARTESIAN_POINT('Ctrl Pts',(8.57966270906098,6.63295370212097,-15.8823448243331)) ;
#110425=CARTESIAN_POINT('Ctrl Pts',(8.57906641006212,6.62681909302431,-15.8844771744941)) ;
#110426=CARTESIAN_POINT('Ctrl Pts',(8.57903375157323,6.6264799875246,-15.8845971697286)) ;
#110427=CARTESIAN_POINT('Ctrl Pts',(8.57846569624192,6.6205258217488,-15.886741731681)) ;
#110428=CARTESIAN_POINT('Ctrl Pts',(8.57802501793965,6.61503168015257,-15.8893142858557)) ;
#110429=CARTESIAN_POINT('Ctrl Pts',(8.57766199200568,6.60925146760312,-15.8927462133234)) ;
#110430=CARTESIAN_POINT('Ctrl Pts',(8.57762821177172,6.60869602779103,-15.8930838351647)) ;
#110431=CARTESIAN_POINT('Ctrl Pts',(8.57728522755446,6.60286036001455,-15.8967147989572)) ;
#110432=CARTESIAN_POINT('Ctrl Pts',(8.57709550103271,6.59788070192331,-15.9005482210564)) ;
#110433=CARTESIAN_POINT('Ctrl Pts',(8.57703980289278,6.59299711069393,-15.9051723373549)) ;
#110434=CARTESIAN_POINT('Ctrl Pts',(8.57703670271021,6.59265952430039,-15.9054968925421)) ;
#110435=CARTESIAN_POINT('Ctrl Pts',(8.57701334129169,6.58927432516127,-15.9088013815953)) ;
#110436=CARTESIAN_POINT('Ctrl Pts',(8.57705699426434,6.5864297120155,-15.9119917444088)) ;
#110437=CARTESIAN_POINT('Ctrl Pts',(8.57735031225521,6.57961409340222,-15.9207954417554)) ;
#110438=CARTESIAN_POINT('Ctrl Pts',(8.57770856513437,6.57604383182914,-15.9266682455399)) ;
#110439=CARTESIAN_POINT('Ctrl Pts',(8.57865704971091,6.57055741297636,-15.9383322193388)) ;
#110440=CARTESIAN_POINT('Ctrl Pts',(8.57922107378969,6.56851476050447,-15.9440736349076)) ;
#110441=CARTESIAN_POINT('Ctrl Pts',(8.57993695782543,6.56687610193754,-15.9504559348163)) ;
#110442=CARTESIAN_POINT('Ctrl Pts',(8.58000419042984,6.56673001682056,-15.9510478351839)) ;
#110443=CARTESIAN_POINT('Ctrl Pts',(8.58074399738019,6.56520526212522,-15.9574812517353)) ;
#110444=CARTESIAN_POINT('Ctrl Pts',(8.58149993293348,6.56438134785777,-15.9633541800934)) ;
#110445=CARTESIAN_POINT('Ctrl Pts',(8.58236768178477,6.56403389662202,-15.9694987578232)) ;
#110446=CARTESIAN_POINT('Ctrl Pts',(8.58242358604549,6.56401394107886,-15.9698921736316)) ;
#110447=CARTESIAN_POINT('Ctrl Pts',(8.58283067264383,6.56388592662946,-15.9727394234264)) ;
#110448=CARTESIAN_POINT('Ctrl Pts',(8.58319156240649,6.56386525642005,-15.9751699505828)) ;
#110449=CARTESIAN_POINT('Ctrl Pts',(8.58356019967707,6.56392669994633,-15.9775662650647)) ;
#110450=CARTESIAN_POINT('Origin',(9.9,6.8847127088383,-16.1997127088383)) ;
#110451=CARTESIAN_POINT('Origin',(9.9,6.8847127088383,-16.1997127088383)) ;
#110452=CARTESIAN_POINT('Origin',(9.9,6.8847127088383,-16.1997127088383)) ;
#110453=CARTESIAN_POINT('Origin',(9.9,7.72792407799439,-17.78)) ;
#110454=CARTESIAN_POINT('Origin',(9.9,7.72792407799439,-16.1997127088383)) ;
#110455=CARTESIAN_POINT('Origin',(9.90000000000001,4.35421736843756,-16.1997127088383)) ;
#110456=CARTESIAN_POINT('Origin',(9.9,7.72792407799439,-16.1997127088383)) ;
#110457=CARTESIAN_POINT('Origin',(9.9,7.72792407799439,-16.1997127088383)) ;
#110458=CARTESIAN_POINT('Origin',(9.9,7.72792407799439,-16.1997127088383)) ;
#110459=CARTESIAN_POINT('Origin',(10.9628342502842,7.37364599456632,-16.3768517505523)) ;
#110460=CARTESIAN_POINT('Ctrl Pts',(8.56837732530591,8.27720755823129,-15.972505253798)) ;
#110461=CARTESIAN_POINT('Ctrl Pts',(8.56753565030799,8.27748812367261,-15.9666129921977)) ;
#110462=CARTESIAN_POINT('Ctrl Pts',(8.5668204554169,8.27721180667912,-15.9605412944397)) ;
#110463=CARTESIAN_POINT('Ctrl Pts',(8.56575413148011,8.27538624160202,-15.9487284721173)) ;
#110464=CARTESIAN_POINT('Ctrl Pts',(8.56538426077847,8.27391165896455,-15.9429905624269)) ;
#110465=CARTESIAN_POINT('Ctrl Pts',(8.56517777855929,8.27166501362482,-15.9370147754464)) ;
#110466=CARTESIAN_POINT('Ctrl Pts',(8.56516523451681,8.27151619608583,-15.9366276382834)) ;
#110467=CARTESIAN_POINT('Ctrl Pts',(8.56497390811214,8.26902793125451,-15.9302953359912)) ;
#110468=CARTESIAN_POINT('Ctrl Pts',(8.56499903025534,8.2659763012945,-15.9245357784659)) ;
#110469=CARTESIAN_POINT('Ctrl Pts',(8.56538588200257,8.26046191593055,-15.9165906723681)) ;
#110470=CARTESIAN_POINT('Ctrl Pts',(8.56556309332507,8.25853771611458,-15.9141212364558)) ;
#110471=CARTESIAN_POINT('Ctrl Pts',(8.56628156514548,8.25214511987158,-15.9068017566891)) ;
#110472=CARTESIAN_POINT('Ctrl Pts',(8.56700742874793,8.2472021625627,-15.902305445231)) ;
#110473=CARTESIAN_POINT('Ctrl Pts',(8.56880713798126,8.23661566152159,-15.8946244948799)) ;
#110474=CARTESIAN_POINT('Ctrl Pts',(8.56986039391321,8.23102391526953,-15.8913848807254)) ;
#110475=CARTESIAN_POINT('Ctrl Pts',(8.57116255171756,8.22459552194113,-15.8884467745269)) ;
#110476=CARTESIAN_POINT('Ctrl Pts',(8.57127495810218,8.22404408343781,-15.8882006607901)) ;
#110477=CARTESIAN_POINT('Ctrl Pts',(8.57260511146311,8.21755901312583,-15.8853749153055)) ;
#110478=CARTESIAN_POINT('Ctrl Pts',(8.57395629672839,8.2113575973091,-15.8833463864276)) ;
#110479=CARTESIAN_POINT('Ctrl Pts',(8.57552311082417,8.20452945286286,-15.8817495443173)) ;
#110480=CARTESIAN_POINT('Ctrl Pts',(8.57564505123012,8.2040002630709,-15.881629826956)) ;
#110481=CARTESIAN_POINT('Ctrl Pts',(8.57731301559523,8.1967919362264,-15.880053462537)) ;
#110482=CARTESIAN_POINT('Ctrl Pts',(8.57896065127869,8.19002168485366,-15.879210969344)) ;
#110483=CARTESIAN_POINT('Ctrl Pts',(8.58161366784366,8.17959769015482,-15.8787553172771)) ;
#110484=CARTESIAN_POINT('Ctrl Pts',(8.58258362864269,8.17587911616515,-15.8787639381071)) ;
#110485=CARTESIAN_POINT('Ctrl Pts',(8.58356010126947,8.17221734381475,-15.8789266835449)) ;
#110486=CARTESIAN_POINT('Origin',(7.96824861826159,6.56275414521524,-14.6022458547848)) ;
#110487=CARTESIAN_POINT('Origin',(8.59688370202597,6.66156024040237,-14.5112434752653)) ;
#110488=CARTESIAN_POINT('Origin',(9.9,6.8847127088383,-14.2802872911617)) ;
#110489=CARTESIAN_POINT('Origin',(9.9,6.8847127088383,-17.78)) ;
#110490=CARTESIAN_POINT('Origin',(9.9,6.8847127088383,-14.2802872911617)) ;
#110491=CARTESIAN_POINT('Origin',(9.9,6.8847127088383,-14.2802872911617)) ;
#110492=CARTESIAN_POINT('Origin',(9.9,6.8847127088383,-14.2802872911617)) ;
#110493=CARTESIAN_POINT('Origin',(9.9,6.8,-14.2802872911617)) ;
#110494=CARTESIAN_POINT('Origin',(9.9,7.72792407799439,-14.2802872911617)) ;
#110495=CARTESIAN_POINT('Origin',(9.9,7.72792407799439,-17.78)) ;
#110496=CARTESIAN_POINT('Origin',(9.9,7.72792407799439,-14.2802872911617)) ;
#110497=CARTESIAN_POINT('Origin',(9.9,7.72792407799439,-14.2802872911617)) ;
#110498=CARTESIAN_POINT('Origin',(9.9,7.72792407799439,-14.2802872911617)) ;
#110499=CARTESIAN_POINT('Origin',(9.60917571369883,7.82486550676144,-14.3287580055452)) ;
#110500=CARTESIAN_POINT('Origin',(8.59099001846147,8.18966234086349,-14.5051609738971)) ;
#110501=CARTESIAN_POINT('Origin',(0.45,4.4,-15.24)) ;
#110502=CARTESIAN_POINT('Origin',(0.45,4.4,-15.69)) ;
#110503=CARTESIAN_POINT('Origin',(0.45,4.4,-14.79)) ;
#110504=CARTESIAN_POINT('Origin',(-1.9,7.55,-17.78)) ;
#110505=CARTESIAN_POINT('Origin',(6.9,7.75,-17.78)) ;
#110506=CARTESIAN_POINT('Origin',(7.1,8.2,-17.78)) ;
#110507=CARTESIAN_POINT('Origin',(9.9,0.1,-17.78)) ;
#110508=CARTESIAN_POINT('Origin',(9.9,1.16528729116168,-17.78)) ;
#110509=CARTESIAN_POINT('Origin',(9.9,1.16528729116168,-17.2841618801782)) ;
#110510=CARTESIAN_POINT('Origin',(9.9,3.8,-15.24)) ;
#110511=CARTESIAN_POINT('Origin',(9.9,1.16528729116168,-13.1958381198218)) ;
#110512=CARTESIAN_POINT('Origin',(9.9,1.16528729116168,-17.2841618801782)) ;
#110513=CARTESIAN_POINT('Origin',(9.9,1.16528729116168,-17.78)) ;
#110514=CARTESIAN_POINT('Origin',(9.9,1.16528729116168,-13.1958381198218)) ;
#110515=CARTESIAN_POINT('Ctrl Pts',(0.55,0.3,-15.69)) ;
#110516=CARTESIAN_POINT('Ctrl Pts',(0.55,0.3,-15.79)) ;
#110517=CARTESIAN_POINT('Ctrl Pts',(0.45,0.3,-15.79)) ;
#110518=CARTESIAN_POINT('Ctrl Pts',(0.55,0.28690770353672,-15.6900000008182)) ;
#110519=CARTESIAN_POINT('Ctrl Pts',(0.549992696056738,0.300543498484345,
-15.7899926960962)) ;
#110520=CARTESIAN_POINT('Ctrl Pts',(0.450000000818259,0.286907703536713,
-15.79)) ;
#110521=CARTESIAN_POINT('Ctrl Pts',(0.552602750539093,0.273825167611082,
-15.6952055010782)) ;
#110522=CARTESIAN_POINT('Ctrl Pts',(0.546703256435903,0.299059401315785,
-15.7867032564359)) ;
#110523=CARTESIAN_POINT('Ctrl Pts',(0.455205501078185,0.273825167611091,
-15.7926027505391)) ;
#110524=CARTESIAN_POINT('Ctrl Pts',(0.56262134295865,0.249638145915901,
-15.7152426859173)) ;
#110525=CARTESIAN_POINT('Ctrl Pts',(0.544986924117065,0.28207277643954,
-15.7849869241171)) ;
#110526=CARTESIAN_POINT('Ctrl Pts',(0.4752426859173,0.249638145915891,-15.8026213429587)) ;
#110527=CARTESIAN_POINT('Ctrl Pts',(0.570033341471288,0.238545302291403,
-15.7300666829426)) ;
#110528=CARTESIAN_POINT('Ctrl Pts',(0.54711619685839,0.267914459835251,
-15.7871161968584)) ;
#110529=CARTESIAN_POINT('Ctrl Pts',(0.490066682942577,0.238545302291388,
-15.8100333414713)) ;
#110530=CARTESIAN_POINT('Ctrl Pts',(0.597801282701459,0.210777361061231,
-15.7856025654029)) ;
#110531=CARTESIAN_POINT('Ctrl Pts',(0.570853448890191,0.226374713859272,
-15.8108534488901)) ;
#110532=CARTESIAN_POINT('Ctrl Pts',(0.545602565402917,0.21077736106126,
-15.8378012827014)) ;
#110533=CARTESIAN_POINT('Ctrl Pts',(0.623746567173686,0.2,-15.8374931343473)) ;
#110534=CARTESIAN_POINT('Ctrl Pts',(0.610458667316253,0.2,-15.8504586673162)) ;
#110535=CARTESIAN_POINT('Ctrl Pts',(0.59749313434734,0.2,-15.8637465671735)) ;
#110536=CARTESIAN_POINT('Ctrl Pts',(0.65,0.2,-15.89)) ;
#110537=CARTESIAN_POINT('Ctrl Pts',(0.65,0.2,-15.89)) ;
#110538=CARTESIAN_POINT('Ctrl Pts',(0.65,0.2,-15.89)) ;
#110539=CARTESIAN_POINT('Origin',(0.45,0.3,-15.69)) ;
#110540=CARTESIAN_POINT('Origin',(0.45,1.24941393210234E-16,-15.69)) ;
#110541=CARTESIAN_POINT('Origin',(0.45,4.4,-15.69)) ;
#110542=CARTESIAN_POINT('Origin',(0.45,4.4,-15.69)) ;
#110543=CARTESIAN_POINT('Origin',(0.45,4.4,-15.69)) ;
#110544=CARTESIAN_POINT('Origin',(0.549999999999999,4.4,-15.69)) ;
#110545=CARTESIAN_POINT('Origin',(-1.7,4.4,-15.69)) ;
#110546=CARTESIAN_POINT('Ctrl Pts',(-1.8,4.6,-15.89)) ;
#110547=CARTESIAN_POINT('Ctrl Pts',(-1.8,4.6,-15.89)) ;
#110548=CARTESIAN_POINT('Ctrl Pts',(-1.8,4.6,-15.89)) ;
#110549=CARTESIAN_POINT('Ctrl Pts',(-1.8,4.57374656717372,-15.8374931343473)) ;
#110550=CARTESIAN_POINT('Ctrl Pts',(-1.8,4.56045866731429,-15.8504586673144)) ;
#110551=CARTESIAN_POINT('Ctrl Pts',(-1.8,4.54749313434728,-15.8637465671737)) ;
#110552=CARTESIAN_POINT('Ctrl Pts',(-1.78922263893876,4.54780128270145,
-15.7856025654029)) ;
#110553=CARTESIAN_POINT('Ctrl Pts',(-1.77362528614074,4.52085344889015,
-15.8108534488901)) ;
#110554=CARTESIAN_POINT('Ctrl Pts',(-1.78922263893874,4.49560256540291,
-15.8378012827014)) ;
#110555=CARTESIAN_POINT('Ctrl Pts',(-1.7614546977086,4.5200333414713,-15.7300666829426)) ;
#110556=CARTESIAN_POINT('Ctrl Pts',(-1.73208554016474,4.49711619685842,
-15.7871161968584)) ;
#110557=CARTESIAN_POINT('Ctrl Pts',(-1.76145469770861,4.44006668294258,
-15.8100333414713)) ;
#110558=CARTESIAN_POINT('Ctrl Pts',(-1.7503618540841,4.51262134295865,-15.7152426859173)) ;
#110559=CARTESIAN_POINT('Ctrl Pts',(-1.71792722356046,4.49498692411707,
-15.7849869241171)) ;
#110560=CARTESIAN_POINT('Ctrl Pts',(-1.75036185408411,4.42524268591729,
-15.8026213429587)) ;
#110561=CARTESIAN_POINT('Ctrl Pts',(-1.72617483238892,4.50260275053909,
-15.6952055010782)) ;
#110562=CARTESIAN_POINT('Ctrl Pts',(-1.70094059868422,4.4967032564359,-15.7867032564359)) ;
#110563=CARTESIAN_POINT('Ctrl Pts',(-1.72617483238891,4.4052055010782,-15.7926027505391)) ;
#110564=CARTESIAN_POINT('Ctrl Pts',(-1.71309229646328,4.5,-15.6900000008182)) ;
#110565=CARTESIAN_POINT('Ctrl Pts',(-1.69945650152272,4.49999269603968,
-15.7899926960963)) ;
#110566=CARTESIAN_POINT('Ctrl Pts',(-1.71309229646329,4.40000000081823,
-15.79)) ;
#110567=CARTESIAN_POINT('Ctrl Pts',(-1.7,4.5,-15.69)) ;
#110568=CARTESIAN_POINT('Ctrl Pts',(-1.7,4.5,-15.79)) ;
#110569=CARTESIAN_POINT('Ctrl Pts',(-1.7,4.4,-15.79)) ;
#110570=CARTESIAN_POINT('Ctrl Pts',(-1.8,4.6,-14.59)) ;
#110571=CARTESIAN_POINT('Ctrl Pts',(-1.8,4.6,-14.59)) ;
#110572=CARTESIAN_POINT('Ctrl Pts',(-1.8,4.6,-14.59)) ;
#110573=CARTESIAN_POINT('Ctrl Pts',(-1.8,4.54749313434729,-14.6162534328264)) ;
#110574=CARTESIAN_POINT('Ctrl Pts',(-1.8,4.56045866731616,-14.6295413326839)) ;
#110575=CARTESIAN_POINT('Ctrl Pts',(-1.8,4.57374656717362,-14.6425068656528)) ;
#110576=CARTESIAN_POINT('Ctrl Pts',(-1.78922263893879,4.49560256540291,
-14.6421987172985)) ;
#110577=CARTESIAN_POINT('Ctrl Pts',(-1.77362528614072,4.52085344889015,
-14.6691465511098)) ;
#110578=CARTESIAN_POINT('Ctrl Pts',(-1.78922263893876,4.54780128270145,
-14.694397434597)) ;
#110579=CARTESIAN_POINT('Ctrl Pts',(-1.76145469770859,4.44006668294258,
-14.6699666585287)) ;
#110580=CARTESIAN_POINT('Ctrl Pts',(-1.73208554016476,4.49711619685842,
-14.6928838031416)) ;
#110581=CARTESIAN_POINT('Ctrl Pts',(-1.7614546977086,4.5200333414713,-14.7499333170575)) ;
#110582=CARTESIAN_POINT('Ctrl Pts',(-1.75036185408409,4.42524268591729,
-14.6773786570414)) ;
#110583=CARTESIAN_POINT('Ctrl Pts',(-1.71792722356047,4.49498692411705,
-14.695013075883)) ;
#110584=CARTESIAN_POINT('Ctrl Pts',(-1.7503618540841,4.51262134295865,-14.7647573140827)) ;
#110585=CARTESIAN_POINT('Ctrl Pts',(-1.72617483238892,4.4052055010782,-14.6873972494609)) ;
#110586=CARTESIAN_POINT('Ctrl Pts',(-1.7009405986842,4.49670325643591,-14.6932967435641)) ;
#110587=CARTESIAN_POINT('Ctrl Pts',(-1.72617483238892,4.50260275053909,
-14.7847944989218)) ;
#110588=CARTESIAN_POINT('Ctrl Pts',(-1.71309229646328,4.40000000081823,
-14.69)) ;
#110589=CARTESIAN_POINT('Ctrl Pts',(-1.69945650151499,4.49999269606786,
-14.6900073039133)) ;
#110590=CARTESIAN_POINT('Ctrl Pts',(-1.71309229646328,4.5,-14.7899999991817)) ;
#110591=CARTESIAN_POINT('Ctrl Pts',(-1.7,4.4,-14.69)) ;
#110592=CARTESIAN_POINT('Ctrl Pts',(-1.7,4.5,-14.69)) ;
#110593=CARTESIAN_POINT('Ctrl Pts',(-1.7,4.5,-14.79)) ;
#110594=CARTESIAN_POINT('Origin',(-1.7,4.4,-14.79)) ;
#110595=CARTESIAN_POINT('Origin',(0.549999999999999,4.4,-14.79)) ;
#110596=CARTESIAN_POINT('Origin',(0.45,4.4,-14.79)) ;
#110597=CARTESIAN_POINT('Origin',(0.45,4.4,-14.79)) ;
#110598=CARTESIAN_POINT('Origin',(0.45,4.4,-14.79)) ;
#110599=CARTESIAN_POINT('Origin',(0.45,4.9047241136249E-17,-14.79)) ;
#110600=CARTESIAN_POINT('Origin',(0.45,0.3,-14.79)) ;
#110601=CARTESIAN_POINT('Ctrl Pts',(0.45,0.3,-14.69)) ;
#110602=CARTESIAN_POINT('Ctrl Pts',(0.55,0.3,-14.69)) ;
#110603=CARTESIAN_POINT('Ctrl Pts',(0.55,0.3,-14.79)) ;
#110604=CARTESIAN_POINT('Ctrl Pts',(0.450000000818259,0.286907703536723,
-14.69)) ;
#110605=CARTESIAN_POINT('Ctrl Pts',(0.549992696019264,0.300543498464983,
-14.690007303913)) ;
#110606=CARTESIAN_POINT('Ctrl Pts',(0.55,0.28690770353672,-14.7899999991817)) ;
#110607=CARTESIAN_POINT('Ctrl Pts',(0.455205501078185,0.273825167611078,
-14.6873972494609)) ;
#110608=CARTESIAN_POINT('Ctrl Pts',(0.546703256435899,0.299059401315789,
-14.6932967435641)) ;
#110609=CARTESIAN_POINT('Ctrl Pts',(0.552602750539093,0.273825167611082,
-14.7847944989218)) ;
#110610=CARTESIAN_POINT('Ctrl Pts',(0.4752426859173,0.249638145915905,-14.6773786570414)) ;
#110611=CARTESIAN_POINT('Ctrl Pts',(0.544986924117067,0.282072776439535,
-14.6950130758829)) ;
#110612=CARTESIAN_POINT('Ctrl Pts',(0.56262134295865,0.249638145915901,
-14.7647573140827)) ;
#110613=CARTESIAN_POINT('Ctrl Pts',(0.490066682942577,0.238545302291402,
-14.6699666585287)) ;
#110614=CARTESIAN_POINT('Ctrl Pts',(0.547116196858397,0.267914459835244,
-14.6928838031416)) ;
#110615=CARTESIAN_POINT('Ctrl Pts',(0.570033341471288,0.238545302291403,
-14.7499333170574)) ;
#110616=CARTESIAN_POINT('Ctrl Pts',(0.545602565402917,0.210777361061233,
-14.6421987172985)) ;
#110617=CARTESIAN_POINT('Ctrl Pts',(0.570853448890184,0.226374713859283,
-14.6691465511098)) ;
#110618=CARTESIAN_POINT('Ctrl Pts',(0.597801282701459,0.210777361061231,
-14.6943974345971)) ;
#110619=CARTESIAN_POINT('Ctrl Pts',(0.59749313434723,0.2,-14.6162534328263)) ;
#110620=CARTESIAN_POINT('Ctrl Pts',(0.610458667316026,0.2,-14.629541332684)) ;
#110621=CARTESIAN_POINT('Ctrl Pts',(0.623746567173609,0.2,-14.6425068656527)) ;
#110622=CARTESIAN_POINT('Ctrl Pts',(0.65,0.2,-14.59)) ;
#110623=CARTESIAN_POINT('Ctrl Pts',(0.65,0.2,-14.59)) ;
#110624=CARTESIAN_POINT('Ctrl Pts',(0.65,0.2,-14.59)) ;
#110625=CARTESIAN_POINT('Ctrl Pts',(8.5,8.17221734381475,-15.7802872911617)) ;
#110626=CARTESIAN_POINT('Ctrl Pts',(8.5,8.17221734381475,-15.865)) ;
#110627=CARTESIAN_POINT('Ctrl Pts',(8.58356010126947,8.17221734381475,-15.8789266835449)) ;
#110628=CARTESIAN_POINT('Ctrl Pts',(8.5,8.23335379241386,-15.7802872927391)) ;
#110629=CARTESIAN_POINT('Ctrl Pts',(8.5,8.20847425960662,-15.8574575674223)) ;
#110630=CARTESIAN_POINT('Ctrl Pts',(8.57460439031233,8.20580126077889,-15.8774340650521)) ;
#110631=CARTESIAN_POINT('Ctrl Pts',(8.5,8.29192178062155,-15.8071741150785)) ;
#110632=CARTESIAN_POINT('Ctrl Pts',(8.5,8.25010493984403,-15.8692546083117)) ;
#110633=CARTESIAN_POINT('Ctrl Pts',(8.56800970738924,8.23725302684489,-15.8897783631899)) ;
#110634=CARTESIAN_POINT('Ctrl Pts',(8.5,8.36583651094027,-15.8965506232914)) ;
#110635=CARTESIAN_POINT('Ctrl Pts',(8.5,8.29925403146167,-15.9233614370366)) ;
#110636=CARTESIAN_POINT('Ctrl Pts',(8.56373266208983,8.27563607377072,-15.9337537764131)) ;
#110637=CARTESIAN_POINT('Ctrl Pts',(8.5,8.38029241321759,-15.9579552056996)) ;
#110638=CARTESIAN_POINT('Ctrl Pts',(8.5,8.30669116589121,-15.9648088499411)) ;
#110639=CARTESIAN_POINT('Ctrl Pts',(8.56610123859376,8.28208399509955,-15.964808702407)) ;
#110640=CARTESIAN_POINT('Ctrl Pts',(8.5,8.36719795478508,-16.0160547234799)) ;
#110641=CARTESIAN_POINT('Ctrl Pts',(8.5,8.29381262650623,-15.9995151496718)) ;
#110642=CARTESIAN_POINT('Ctrl Pts',(8.57227762885807,8.27346847343705,-15.9949299876354)) ;
#110643=CARTESIAN_POINT('Ctrl Pts',(8.5485213309235,8.28383177029354,-15.9959865327337)) ;
#110644=CARTESIAN_POINT('Ctrl Pts',(8.54913757890789,8.28625057716298,-15.982921659184)) ;
#110645=CARTESIAN_POINT('Ctrl Pts',(8.549146361399,8.28675781111762,-15.9692647894026)) ;
#110646=CARTESIAN_POINT('Ctrl Pts',(8.54883414737369,8.28489376483071,-15.956098869425)) ;
#110647=CARTESIAN_POINT('Ctrl Pts',(8.54852072231757,8.28302248819127,-15.9428818808428)) ;
#110648=CARTESIAN_POINT('Ctrl Pts',(8.54791723678494,8.27865742078997,-15.9298312958117)) ;
#110649=CARTESIAN_POINT('Ctrl Pts',(8.54677696932927,8.27237937104781,-15.9181020767297)) ;
#110650=CARTESIAN_POINT('Ctrl Pts',(8.5454465495755,8.26505438658866,-15.9044168797302)) ;
#110651=CARTESIAN_POINT('Ctrl Pts',(8.54324462275112,8.25487237915563,-15.8922537533388)) ;
#110652=CARTESIAN_POINT('Ctrl Pts',(8.53884071267076,8.24480815719263,-15.8812071681992)) ;
#110653=CARTESIAN_POINT('Ctrl Pts',(8.5342440055524,8.23430333763594,-15.8696769789768)) ;
#110654=CARTESIAN_POINT('Ctrl Pts',(8.52670159721618,8.22420330618022,-15.858704260243)) ;
#110655=CARTESIAN_POINT('Ctrl Pts',(8.51928858688475,8.21729138318396,-15.8459881754653)) ;
#110656=CARTESIAN_POINT('Ctrl Pts',(8.51327528614099,8.21168455548023,-15.835673116045)) ;
#110657=CARTESIAN_POINT('Ctrl Pts',(8.50759525524367,8.20778929846109,-15.8239849430828)) ;
#110658=CARTESIAN_POINT('Ctrl Pts',(8.50412058850191,8.20498026622232,-15.8115739486628)) ;
#110659=CARTESIAN_POINT('Ctrl Pts',(8.50147164778345,8.20283877743224,-15.8021123251694)) ;
#110660=CARTESIAN_POINT('Ctrl Pts',(8.50000317248551,8.2012555848359,-15.792083357655)) ;
#110661=CARTESIAN_POINT('Ctrl Pts',(8.50000000513446,8.20000405629318,-15.7821052387284)) ;
#110662=CARTESIAN_POINT('Origin',(8.6,8.17221734381475,-15.7802872911617)) ;
#110663=CARTESIAN_POINT('Origin',(8.6,4.35421736843756,-15.7802872911617)) ;
#110664=CARTESIAN_POINT('Origin',(8.6,6.66256607592813,-15.7802872911617)) ;
#110665=CARTESIAN_POINT('Ctrl Pts',(8.5,6.47083593368087,-16.0248081099244)) ;
#110666=CARTESIAN_POINT('Ctrl Pts',(8.5,6.55684090505321,-16.0043877386952)) ;
#110667=CARTESIAN_POINT('Ctrl Pts',(8.58772778625753,6.56739561896918,-16.001881707091)) ;
#110668=CARTESIAN_POINT('Ctrl Pts',(8.5,6.45680686388577,-15.9657215297177)) ;
#110669=CARTESIAN_POINT('Ctrl Pts',(8.5,6.544062294786,-15.9725101654037)) ;
#110670=CARTESIAN_POINT('Ctrl Pts',(8.58195196310359,6.55941415012443,-15.9713576868778)) ;
#110671=CARTESIAN_POINT('Ctrl Pts',(8.5,6.47061556584392,-15.9019524568048)) ;
#110672=CARTESIAN_POINT('Ctrl Pts',(8.5,6.54836369988892,-15.9323987274072)) ;
#110673=CARTESIAN_POINT('Ctrl Pts',(8.57801125828727,6.5656660137223,-15.9388344592028)) ;
#110674=CARTESIAN_POINT('Ctrl Pts',(8.5,6.54379299301794,-15.8086264716581)) ;
#110675=CARTESIAN_POINT('Ctrl Pts',(8.5,6.5907178951622,-15.8762265152921)) ;
#110676=CARTESIAN_POINT('Ctrl Pts',(8.57642058265785,6.60198961470446,-15.8919063540245)) ;
#110677=CARTESIAN_POINT('Ctrl Pts',(8.5,6.60220518075383,-15.7802872929745)) ;
#110678=CARTESIAN_POINT('Ctrl Pts',(8.5,6.62800697860329,-15.8609176707628)) ;
#110679=CARTESIAN_POINT('Ctrl Pts',(8.57879135173924,6.63156920211803,-15.8781318919565)) ;
#110680=CARTESIAN_POINT('Ctrl Pts',(8.5,6.66256607592813,-15.7802872911617)) ;
#110681=CARTESIAN_POINT('Ctrl Pts',(8.5,6.66256607592813,-15.865)) ;
#110682=CARTESIAN_POINT('Ctrl Pts',(8.58356010126947,6.66256607592813,-15.8789266835449)) ;
#110683=CARTESIAN_POINT('',(8.54565366748552,6.61650711946997,-15.8739653182917)) ;
#110684=CARTESIAN_POINT('Ctrl Pts',(8.54565366716102,6.61650712004131,-15.8739653178135)) ;
#110685=CARTESIAN_POINT('Ctrl Pts',(8.54527684775567,6.61717057264361,-15.8734100008637)) ;
#110686=CARTESIAN_POINT('Ctrl Pts',(8.54488909344006,6.61782772231432,-15.8728554298997)) ;
#110687=CARTESIAN_POINT('Ctrl Pts',(8.54449064961563,6.61847724592616,-15.8723008713851)) ;
#110688=CARTESIAN_POINT('Ctrl Pts',(8.54445329550709,6.61853813876477,-15.8722488815244)) ;
#110689=CARTESIAN_POINT('Ctrl Pts',(8.54441584757976,6.6185989645223,-15.8721968917916)) ;
#110690=CARTESIAN_POINT('Ctrl Pts',(8.54437830610599,6.61865972207468,-15.8721449015859)) ;
#110691=CARTESIAN_POINT('Ctrl Pts',(8.54363538409151,6.61986207559658,-15.8711160483068)) ;
#110692=CARTESIAN_POINT('Ctrl Pts',(8.54285495000594,6.62104203503528,-15.8700848621747)) ;
#110693=CARTESIAN_POINT('Ctrl Pts',(8.54204093171157,6.6221805696012,-15.8690511151673)) ;
#110694=CARTESIAN_POINT('Ctrl Pts',(8.54157979215442,6.62282554690595,-15.8684654997818)) ;
#110695=CARTESIAN_POINT('Ctrl Pts',(8.5411077081219,6.62345780120144,-15.8678786499067)) ;
#110696=CARTESIAN_POINT('Ctrl Pts',(8.54062344907118,6.62407892448169,-15.8672869541396)) ;
#110697=CARTESIAN_POINT('Ctrl Pts',(8.54011932596482,6.62472552591744,-15.8666709873185)) ;
#110698=CARTESIAN_POINT('Ctrl Pts',(8.53960207832256,6.62535666566134,-15.866050990589)) ;
#110699=CARTESIAN_POINT('Ctrl Pts',(8.53907286520408,6.62597244099096,-15.8654252288111)) ;
#110700=CARTESIAN_POINT('Ctrl Pts',(8.53887441028465,6.62620335673957,-15.8651905681443)) ;
#110701=CARTESIAN_POINT('Ctrl Pts',(8.53867427664143,6.6264321129994,-15.8649550998211)) ;
#110702=CARTESIAN_POINT('Ctrl Pts',(8.53847256319998,6.62665871795108,-15.8647187642184)) ;
#110703=CARTESIAN_POINT('Ctrl Pts',(8.53842843838466,6.62670828778426,-15.8646670658053)) ;
#110704=CARTESIAN_POINT('Ctrl Pts',(8.53838423811749,6.62675775467668,-15.8646153260174)) ;
#110705=CARTESIAN_POINT('Ctrl Pts',(8.53833996369345,6.62680711871688,-15.8645635444601)) ;
#110706=CARTESIAN_POINT('Ctrl Pts',(8.53829707284515,6.62685494013081,-15.8645133810765)) ;
#110707=CARTESIAN_POINT('Ctrl Pts',(8.53825411240224,6.62690266502018,-15.8644631784931)) ;
#110708=CARTESIAN_POINT('Ctrl Pts',(8.53821108363806,6.62695029346532,-15.8644129364377)) ;
#110709=CARTESIAN_POINT('Ctrl Pts',(8.53803571435332,6.62714440934376,-15.8642081684534)) ;
#110710=CARTESIAN_POINT('Ctrl Pts',(8.53785876035507,6.62733753498028,-15.8640021836648)) ;
#110711=CARTESIAN_POINT('Ctrl Pts',(8.53767995296704,6.62753033615257,-15.8637944665652)) ;
#110712=CARTESIAN_POINT('Ctrl Pts',(8.53649871780655,6.62880401687797,-15.862422248425)) ;
#110713=CARTESIAN_POINT('Ctrl Pts',(8.53528300832266,6.62998038079526,-15.8610380760596)) ;
#110714=CARTESIAN_POINT('Ctrl Pts',(8.53403203676338,6.63110281535143,-15.8596044865649)) ;
#110715=CARTESIAN_POINT('Ctrl Pts',(8.53346870389682,6.63160826591213,-15.8589589178679)) ;
#110716=CARTESIAN_POINT('Ctrl Pts',(8.53289959536922,6.63209979040222,-15.8583054256595)) ;
#110717=CARTESIAN_POINT('Ctrl Pts',(8.53232661340321,6.63257735344029,-15.8576437014439)) ;
#110718=CARTESIAN_POINT('Ctrl Pts',(8.53206474273906,6.63279561467254,-15.8573412727985)) ;
#110719=CARTESIAN_POINT('Ctrl Pts',(8.53180206199568,6.63301096017662,-15.8570371260807)) ;
#110720=CARTESIAN_POINT('Ctrl Pts',(8.53153874718659,6.63322338883723,-15.8567312388807)) ;
#110721=CARTESIAN_POINT('Ctrl Pts',(8.5300736365822,6.63440536369243,-15.8550292511271)) ;
#110722=CARTESIAN_POINT('Ctrl Pts',(8.52858926277509,6.63549697414123,-15.8532730839131)) ;
#110723=CARTESIAN_POINT('Ctrl Pts',(8.52711342564667,6.63649856635108,-15.8514611393064)) ;
#110724=CARTESIAN_POINT('Ctrl Pts',(8.5263431695412,6.63702130866457,-15.8505154649028)) ;
#110725=CARTESIAN_POINT('Ctrl Pts',(8.52557615349971,6.63751985710294,-15.8495557193112)) ;
#110726=CARTESIAN_POINT('Ctrl Pts',(8.52481401823432,6.63799287689813,-15.8485803261613)) ;
#110727=CARTESIAN_POINT('Ctrl Pts',(8.52460710835824,6.63812129566006,-15.8483155195253)) ;
#110728=CARTESIAN_POINT('Ctrl Pts',(8.52440075574006,6.63824801482191,-15.8480497539023)) ;
#110729=CARTESIAN_POINT('Ctrl Pts',(8.52419502810873,6.63837284070828,-15.8477830860811)) ;
#110730=CARTESIAN_POINT('Ctrl Pts',(8.52404824365687,6.63846190263541,-15.8475928214593)) ;
#110731=CARTESIAN_POINT('Ctrl Pts',(8.52390173612806,6.63855002749202,-15.8474020437347)) ;
#110732=CARTESIAN_POINT('Ctrl Pts',(8.52375553261478,6.63863721305422,-15.8472107628049)) ;
#110733=CARTESIAN_POINT('Ctrl Pts',(8.52294204127162,6.63912232246439,-15.8461464560924)) ;
#110734=CARTESIAN_POINT('Ctrl Pts',(8.52213801365707,6.63957834748689,-15.8450665375564)) ;
#110735=CARTESIAN_POINT('Ctrl Pts',(8.52134774490512,6.64000494097979,-15.8439729614464)) ;
#110736=CARTESIAN_POINT('Ctrl Pts',(8.51876608595598,6.64139854145541,-15.8404004545695)) ;
#110737=CARTESIAN_POINT('Ctrl Pts',(8.51630176076719,6.64256282842068,-15.8366245667844)) ;
#110738=CARTESIAN_POINT('Ctrl Pts',(8.51404737801022,6.64354662431173,-15.8326687582286)) ;
#110739=CARTESIAN_POINT('Ctrl Pts',(8.51174271377018,6.64455236266853,-15.8286247197926)) ;
#110740=CARTESIAN_POINT('Ctrl Pts',(8.50965863261302,6.64536892721963,-15.8243937780696)) ;
#110741=CARTESIAN_POINT('Ctrl Pts',(8.50786496313903,6.64606338785378,-15.8200441654859)) ;
#110742=CARTESIAN_POINT('Ctrl Pts',(8.50767015284864,6.64613881316472,-15.8195717544298)) ;
#110743=CARTESIAN_POINT('Ctrl Pts',(8.50747873128293,6.64621281334902,-15.8190979736875)) ;
#110744=CARTESIAN_POINT('Ctrl Pts',(8.50729076020857,6.64628549377757,-15.8186229301938)) ;
#110745=CARTESIAN_POINT('Ctrl Pts',(8.50722027105568,6.64631274893828,-15.8184447888837)) ;
#110746=CARTESIAN_POINT('Ctrl Pts',(8.50715026706478,6.64633981850992,-15.8182664700192)) ;
#110747=CARTESIAN_POINT('Ctrl Pts',(8.50708075128542,6.6463667080633,-15.8180879793594)) ;
#110748=CARTESIAN_POINT('Ctrl Pts',(8.50659414082988,6.6465549349369,-15.816838544741)) ;
#110749=CARTESIAN_POINT('Ctrl Pts',(8.50613147592892,6.64673434010344,-15.815580683755)) ;
#110750=CARTESIAN_POINT('Ctrl Pts',(8.50569363751095,6.64690683932496,-15.8143164275023)) ;
#110751=CARTESIAN_POINT('Ctrl Pts',(8.50395436040201,6.64759207829665,-15.8092942735069)) ;
#110752=CARTESIAN_POINT('Ctrl Pts',(8.50258205288293,6.64816393978924,-15.8040915596145)) ;
#110753=CARTESIAN_POINT('Ctrl Pts',(8.50162662717129,6.64864720987501,-15.7988041247427)) ;
#110754=CARTESIAN_POINT('Ctrl Pts',(8.50156399248209,6.64867889153404,-15.798457497228)) ;
#110755=CARTESIAN_POINT('Ctrl Pts',(8.50150313499575,6.64871019935918,-15.7981105075157)) ;
#110756=CARTESIAN_POINT('Ctrl Pts',(8.50144406283925,6.6487411427168,-15.797763183502)) ;
#110757=CARTESIAN_POINT('Ctrl Pts',(8.50057491246561,6.64919642372274,-15.7926528774931)) ;
#110758=CARTESIAN_POINT('Ctrl Pts',(8.50009537300568,6.64957062705855,-15.78747132905)) ;
#110759=CARTESIAN_POINT('Ctrl Pts',(8.50001293997568,6.64989933182557,-15.782314443539)) ;
#110760=CARTESIAN_POINT('Ctrl Pts',(8.50000430878269,6.64993374902799,-15.7817744891777)) ;
#110761=CARTESIAN_POINT('Ctrl Pts',(8.5,6.649967656983,-15.7812348144276)) ;
#110762=CARTESIAN_POINT('Ctrl Pts',(8.5,6.65000108682384,-15.7806955361059)) ;
#110763=CARTESIAN_POINT('',(8.55245136877618,6.60097994372616,-15.8867801193795)) ;
#110764=CARTESIAN_POINT('Ctrl Pts',(8.5523805647549,6.60105295171781,-15.8868886154986)) ;
#110765=CARTESIAN_POINT('Ctrl Pts',(8.55170523171907,6.6030854236856,-15.8851022656148)) ;
#110766=CARTESIAN_POINT('Ctrl Pts',(8.55095829520368,6.60513808680113,-15.8833627348222)) ;
#110767=CARTESIAN_POINT('Ctrl Pts',(8.55012599030534,6.60719152980351,-15.8816544441816)) ;
#110768=CARTESIAN_POINT('Ctrl Pts',(8.54968322947886,6.60828389886524,-15.8807456856517)) ;
#110769=CARTESIAN_POINT('Ctrl Pts',(8.54921644930871,6.60937569995262,-15.8798462491235)) ;
#110770=CARTESIAN_POINT('Ctrl Pts',(8.54872481267394,6.61045954913298,-15.8789557465494)) ;
#110771=CARTESIAN_POINT('Ctrl Pts',(8.54779539897816,6.61250851009546,-15.8772722973719)) ;
#110772=CARTESIAN_POINT('Ctrl Pts',(8.54677348694555,6.61453549290065,-15.8756155908862)) ;
#110773=CARTESIAN_POINT('Ctrl Pts',(8.54565366748552,6.61650711946997,-15.8739653182917)) ;
#110774=CARTESIAN_POINT('',(8.55735473176745,6.58264207262453,-15.9049557973616)) ;
#110775=CARTESIAN_POINT('Ctrl Pts',(8.557354731687,6.58264207302789,-15.9049557968441)) ;
#110776=CARTESIAN_POINT('Ctrl Pts',(8.55706916598052,6.58397660851271,-15.9032296933714)) ;
#110777=CARTESIAN_POINT('Ctrl Pts',(8.55678088122702,6.58528501693262,-15.9016621009603)) ;
#110778=CARTESIAN_POINT('Ctrl Pts',(8.55647408091819,6.58661569125896,-15.9001718232515)) ;
#110779=CARTESIAN_POINT('Ctrl Pts',(8.55614409617577,6.58804692262413,-15.8985689275185)) ;
#110780=CARTESIAN_POINT('Ctrl Pts',(8.55579261555186,6.5895052459012,-15.8970567950172)) ;
#110781=CARTESIAN_POINT('Ctrl Pts',(8.55539993844502,6.59102291080544,-15.8955875677792)) ;
#110782=CARTESIAN_POINT('Ctrl Pts',(8.55517214917305,6.59190329771266,-15.894735279227)) ;
#110783=CARTESIAN_POINT('Ctrl Pts',(8.55493049881961,6.59280308289159,-15.8938983977538)) ;
#110784=CARTESIAN_POINT('Ctrl Pts',(8.55467134659048,6.59372113732149,-15.8930707946419)) ;
#110785=CARTESIAN_POINT('Ctrl Pts',(8.5543480523717,6.59486641664517,-15.8920383539702)) ;
#110786=CARTESIAN_POINT('Ctrl Pts',(8.55400737519029,6.59602723165037,-15.8910361981957)) ;
#110787=CARTESIAN_POINT('Ctrl Pts',(8.55365328858766,6.59718920061514,-15.8900452155133)) ;
#110788=CARTESIAN_POINT('Ctrl Pts',(8.55328167888691,6.59840867329803,-15.889005190911)) ;
#110789=CARTESIAN_POINT('Ctrl Pts',(8.55289390107693,6.59963546460028,-15.8879736796763)) ;
#110790=CARTESIAN_POINT('Ctrl Pts',(8.55249886556661,6.60083562835457,-15.8869081494348)) ;
#110791=CARTESIAN_POINT('Ctrl Pts',(8.55248304763317,6.60088368507324,-15.8868654836845)) ;
#110792=CARTESIAN_POINT('Ctrl Pts',(8.55246721522809,6.60093179017222,-15.886822806733)) ;
#110793=CARTESIAN_POINT('Ctrl Pts',(8.55245136877618,6.60097994372616,-15.8867801193795)) ;
#110794=CARTESIAN_POINT('Ctrl Pts',(8.56107669735261,6.5600938800009,-16.0023838472224)) ;
#110795=CARTESIAN_POINT('Ctrl Pts',(8.56115635543005,6.55978170524809,-16.0008207343832)) ;
#110796=CARTESIAN_POINT('Ctrl Pts',(8.56122592915387,6.55950119162288,-15.9992507129806)) ;
#110797=CARTESIAN_POINT('Ctrl Pts',(8.56128584055879,6.55925348717443,-15.9976933919487)) ;
#110798=CARTESIAN_POINT('Ctrl Pts',(8.56142626445294,6.55867290283842,-15.9940432508109)) ;
#110799=CARTESIAN_POINT('Ctrl Pts',(8.56152217534693,6.55825854507366,-15.9903756338769)) ;
#110800=CARTESIAN_POINT('Ctrl Pts',(8.5615808174699,6.55798577878933,-15.9866701354253)) ;
#110801=CARTESIAN_POINT('Ctrl Pts',(8.56158917845351,6.5579468887506,-15.9861418187432)) ;
#110802=CARTESIAN_POINT('Ctrl Pts',(8.56159677639836,6.55791088241228,-15.9856126452595)) ;
#110803=CARTESIAN_POINT('Ctrl Pts',(8.56160362608007,6.55787769947531,-15.9850824674717)) ;
#110804=CARTESIAN_POINT('Ctrl Pts',(8.56164117305277,6.55769580506315,-15.982176263686)) ;
#110805=CARTESIAN_POINT('Ctrl Pts',(8.56164095204357,6.55766773657216,-15.9792640119966)) ;
#110806=CARTESIAN_POINT('Ctrl Pts',(8.56161306230089,6.55774920537472,-15.9763655672583)) ;
#110807=CARTESIAN_POINT('Ctrl Pts',(8.56157759693122,6.55785280336172,-15.9726798246079)) ;
#110808=CARTESIAN_POINT('Ctrl Pts',(8.5615027562466,6.55813669070952,-15.969004928021)) ;
#110809=CARTESIAN_POINT('Ctrl Pts',(8.56141108129145,6.55856506509339,-15.9653632925482)) ;
#110810=CARTESIAN_POINT('Ctrl Pts',(8.5613661599722,6.55877497130414,-15.963578867681)) ;
#110811=CARTESIAN_POINT('Ctrl Pts',(8.56131707129297,6.55902016312284,-15.9618016709685)) ;
#110812=CARTESIAN_POINT('Ctrl Pts',(8.56126585691691,6.55929956116447,-15.9600315254682)) ;
#110813=CARTESIAN_POINT('Ctrl Pts',(8.56116752027492,6.55983603289968,-15.9566326719095)) ;
#110814=CARTESIAN_POINT('Ctrl Pts',(8.56104954130216,6.56049109659204,-15.9532540075756)) ;
#110815=CARTESIAN_POINT('Ctrl Pts',(8.56091150449775,6.56129147625803,-15.9498304710248)) ;
#110816=CARTESIAN_POINT('Ctrl Pts',(8.56080235670743,6.56192434857304,-15.9471234288616)) ;
#110817=CARTESIAN_POINT('Ctrl Pts',(8.56068045333715,6.56264902401852,-15.9443872666894)) ;
#110818=CARTESIAN_POINT('Ctrl Pts',(8.56054379825319,6.56349285586897,-15.9416234877212)) ;
#110819=CARTESIAN_POINT('Ctrl Pts',(8.56050762866484,6.56371619955867,-15.9408919763521)) ;
#110820=CARTESIAN_POINT('Ctrl Pts',(8.56047042218818,6.56394794674722,-15.9401587916983)) ;
#110821=CARTESIAN_POINT('Ctrl Pts',(8.5604321390176,6.56418871538696,-15.9394246234709)) ;
#110822=CARTESIAN_POINT('Ctrl Pts',(8.56026887460239,6.56521550994376,-15.9362936511792)) ;
#110823=CARTESIAN_POINT('Ctrl Pts',(8.56008532870545,6.56636514336275,-15.9332612149346)) ;
#110824=CARTESIAN_POINT('Ctrl Pts',(8.5598891591871,6.56762686151827,-15.9304713276669)) ;
#110825=CARTESIAN_POINT('Ctrl Pts',(8.55964574654527,6.56919243680269,-15.9270095572757)) ;
#110826=CARTESIAN_POINT('Ctrl Pts',(8.55938661160132,6.57080906160865,-15.923732634051)) ;
#110827=CARTESIAN_POINT('Ctrl Pts',(8.55911582090257,6.57246439798288,-15.920667212428)) ;
#110828=CARTESIAN_POINT('Ctrl Pts',(8.55888928658553,6.5738491962671,-15.9181027846356)) ;
#110829=CARTESIAN_POINT('Ctrl Pts',(8.55863813502893,6.57544444689309,-15.9153653454316)) ;
#110830=CARTESIAN_POINT('Ctrl Pts',(8.55834707044213,6.57718152485361,-15.9126681258235)) ;
#110831=CARTESIAN_POINT('Ctrl Pts',(8.55828762047115,6.57753632320085,-15.9121172184487)) ;
#110832=CARTESIAN_POINT('Ctrl Pts',(8.55822651695173,6.5778969434577,-15.9115678465793)) ;
#110833=CARTESIAN_POINT('Ctrl Pts',(8.55816364958867,6.57826264684155,-15.9110215710793)) ;
#110834=CARTESIAN_POINT('Ctrl Pts',(8.55792499569721,6.57965091145837,-15.9089478277641)) ;
#110835=CARTESIAN_POINT('Ctrl Pts',(8.5576603261423,6.58110993502786,-15.9069213132877)) ;
#110836=CARTESIAN_POINT('Ctrl Pts',(8.55735473176745,6.58264207262453,-15.9049557973616)) ;
#110837=CARTESIAN_POINT('Origin',(8.49172374697018,6.65,-17.78)) ;
#110838=CARTESIAN_POINT('Origin',(8.4922693126432,6.63793757512217,-16.0129882716364)) ;
#110839=CARTESIAN_POINT('Ctrl Pts',(8.40188506081761,6.5500005341705,-15.7515458308153)) ;
#110840=CARTESIAN_POINT('Ctrl Pts',(8.5028074458744,6.54966497091121,-15.7651950407541)) ;
#110841=CARTESIAN_POINT('Ctrl Pts',(8.50109204799972,6.65199687180764,-15.7656804549399)) ;
#110842=CARTESIAN_POINT('Ctrl Pts',(8.3929693293079,6.55000052027914,-15.809675802422)) ;
#110843=CARTESIAN_POINT('Ctrl Pts',(8.49725036372771,6.54968051003366,-15.7969136026831)) ;
#110844=CARTESIAN_POINT('Ctrl Pts',(8.49665296516362,6.64935672317804,-15.7960247114635)) ;
#110845=CARTESIAN_POINT('Ctrl Pts',(8.41146079558545,6.55000052635931,-15.869608884646)) ;
#110846=CARTESIAN_POINT('Ctrl Pts',(8.50278789772742,6.54967384197881,-15.8210143519806)) ;
#110847=CARTESIAN_POINT('Ctrl Pts',(8.50590954255545,6.65051247736746,-15.8244272120935)) ;
#110848=CARTESIAN_POINT('Ctrl Pts',(8.4574451591417,6.55000045243508,-15.9228021918822)) ;
#110849=CARTESIAN_POINT('Ctrl Pts',(8.5202381168081,6.54973725194854,-15.861633015821)) ;
#110850=CARTESIAN_POINT('Ctrl Pts',(8.52891723073131,6.63643009777378,-15.8534751630783)) ;
#110851=CARTESIAN_POINT('Ctrl Pts',(8.46608867121678,6.55000043643008,-15.9311950991748)) ;
#110852=CARTESIAN_POINT('Ctrl Pts',(8.52334270167613,6.54974993059824,-15.868470240079)) ;
#110853=CARTESIAN_POINT('Ctrl Pts',(8.53324349789231,6.63337968978884,-15.8582208913001)) ;
#110854=CARTESIAN_POINT('Ctrl Pts',(8.48465388181683,6.55000038323734,-15.9465763138745)) ;
#110855=CARTESIAN_POINT('Ctrl Pts',(8.53001210036429,6.54978938646809,-15.8851245951232)) ;
#110856=CARTESIAN_POINT('Ctrl Pts',(8.54253954944034,6.62323710347996,-15.868863146269)) ;
#110857=CARTESIAN_POINT('Ctrl Pts',(8.49467048074911,6.55000035131511,-15.9534884944614)) ;
#110858=CARTESIAN_POINT('Ctrl Pts',(8.53347884787437,6.54981166882492,-15.89305903115)) ;
#110859=CARTESIAN_POINT('Ctrl Pts',(8.5475533753473,6.6171479354886,-15.8728676881263)) ;
#110860=CARTESIAN_POINT('Ctrl Pts',(8.50997930894003,6.55000022766094,-15.9633889027859)) ;
#110861=CARTESIAN_POINT('Ctrl Pts',(8.53869035159217,6.54988741100163,-15.9187742327549)) ;
#110862=CARTESIAN_POINT('Ctrl Pts',(8.55523846583762,6.59353839814627,-15.8935278831083)) ;
#110863=CARTESIAN_POINT('Ctrl Pts',(8.51532901080101,6.5500001611307,-15.9663389673193)) ;
#110864=CARTESIAN_POINT('Ctrl Pts',(8.54023459682686,6.54992340374042,-15.9284897483873)) ;
#110865=CARTESIAN_POINT('Ctrl Pts',(8.55790835982308,6.58082417519535,-15.9015823085729)) ;
#110866=CARTESIAN_POINT('Ctrl Pts',(8.52186010906342,6.55000005932357,-15.9727927598773)) ;
#110867=CARTESIAN_POINT('Ctrl Pts',(8.54265823247975,6.54997327731409,-15.9579316441152)) ;
#110868=CARTESIAN_POINT('Ctrl Pts',(8.56121746518601,6.56135337205752,-15.9445883700754)) ;
#110869=CARTESIAN_POINT('Ctrl Pts',(8.52354993939967,6.55000003603139,-15.9758242622279)) ;
#110870=CARTESIAN_POINT('Ctrl Pts',(8.54350769968238,6.54998394755847,-15.9714238732007)) ;
#110871=CARTESIAN_POINT('Ctrl Pts',(8.5621431061544,6.55689632415131,-15.9674501335625)) ;
#110872=CARTESIAN_POINT('Ctrl Pts',(8.52268461318107,6.55000004733862,-15.9817875304157)) ;
#110873=CARTESIAN_POINT('Ctrl Pts',(8.54305517585921,6.54997881410036,-15.99281341214)) ;
#110874=CARTESIAN_POINT('Ctrl Pts',(8.5615325917139,6.55906016573919,-16.0027901815805)) ;
#110875=CARTESIAN_POINT('Ctrl Pts',(8.52060566253923,6.55000006807331,-15.9844138065496)) ;
#110876=CARTESIAN_POINT('Ctrl Pts',(8.54195943530535,6.54996919659462,-16.0004945748859)) ;
#110877=CARTESIAN_POINT('Ctrl Pts',(8.56058441628599,6.56302742363386,-16.0145079215137)) ;
#110878=CARTESIAN_POINT('Ctrl Pts',(8.51445291480382,6.55000012130567,-15.9912328149552)) ;
#110879=CARTESIAN_POINT('Ctrl Pts',(8.53868948987836,6.54994355920607,-16.0194191817675)) ;
#110880=CARTESIAN_POINT('Ctrl Pts',(8.55750149922673,6.57320954252654,-16.0411844353069)) ;
#110881=CARTESIAN_POINT('Ctrl Pts',(8.50953280296012,6.55000015625148,-15.9950479464372)) ;
#110882=CARTESIAN_POINT('Ctrl Pts',(8.53616288920967,6.54992588038503,-16.0277647485266)) ;
#110883=CARTESIAN_POINT('Ctrl Pts',(8.55504783006516,6.57989127253965,-16.0506993167928)) ;
#110884=CARTESIAN_POINT('Ctrl Pts',(8.49261655785707,6.55000026291038,-16.0084926065689)) ;
#110885=CARTESIAN_POINT('Ctrl Pts',(8.52778251455087,6.54986718408742,-16.0557691608947)) ;
#110886=CARTESIAN_POINT('Ctrl Pts',(8.54658667616929,6.60027178071326,-16.0793533757438)) ;
#110887=CARTESIAN_POINT('Ctrl Pts',(8.48022165824516,6.55000031608562,-16.0177685341604)) ;
#110888=CARTESIAN_POINT('Ctrl Pts',(8.52288681814154,6.54983437262021,-16.0674559489292)) ;
#110889=CARTESIAN_POINT('Ctrl Pts',(8.54045339450462,6.610423887593,-16.0863019909606)) ;
#110890=CARTESIAN_POINT('Ctrl Pts',(8.46952991654744,6.55000035836673,-16.0290954462183)) ;
#110891=CARTESIAN_POINT('Ctrl Pts',(8.51900842894269,6.54980714069599,-16.0833676846763)) ;
#110892=CARTESIAN_POINT('Ctrl Pts',(8.53471369258699,6.61849392543639,-16.1013833684425)) ;
#110893=CARTESIAN_POINT('Origin',(8.4,6.65,-15.7806780018997)) ;
#110894=CARTESIAN_POINT('Ctrl Pts',(8.54848814460235,8.28374914930622,-14.4835371747799)) ;
#110895=CARTESIAN_POINT('Ctrl Pts',(8.55964225199693,8.27720012980426,-14.4849679483223)) ;
#110896=CARTESIAN_POINT('Ctrl Pts',(8.572140519951,8.27365818248462,-14.4857417625569)) ;
#110897=CARTESIAN_POINT('Ctrl Pts',(8.54519582228985,8.29111303851996,-14.5079603788076)) ;
#110898=CARTESIAN_POINT('Ctrl Pts',(8.55569959891137,8.28406912459881,-14.5080376174409)) ;
#110899=CARTESIAN_POINT('Ctrl Pts',(8.56757951573628,8.27991709749371,-14.5081916339118)) ;
#110900=CARTESIAN_POINT('Ctrl Pts',(8.54340782920288,8.28927570119136,-14.5338229931233)) ;
#110901=CARTESIAN_POINT('Ctrl Pts',(8.55355053837511,8.28232618564301,-14.5321546442898)) ;
#110902=CARTESIAN_POINT('Ctrl Pts',(8.56507848568421,8.27803412520747,-14.5311321430533)) ;
#110903=CARTESIAN_POINT('Ctrl Pts',(8.54340835145922,8.27841951799441,-14.5555350111617)) ;
#110904=CARTESIAN_POINT('Ctrl Pts',(8.55355093564017,8.27219257320284,-14.5524215387659)) ;
#110905=CARTESIAN_POINT('Ctrl Pts',(8.56507848521152,8.26835005667905,-14.550500280504)) ;
#110906=CARTESIAN_POINT('Ctrl Pts',(8.54742026180266,8.27608084857564,-14.5543656412486)) ;
#110907=CARTESIAN_POINT('Ctrl Pts',(8.54754672558908,8.27683897030432,-14.5526745730365)) ;
#110908=CARTESIAN_POINT('Ctrl Pts',(8.54766225486891,8.27755642830995,-14.5509654973084)) ;
#110909=CARTESIAN_POINT('Ctrl Pts',(8.54776713596767,8.27823455672262,-14.5492350167776)) ;
#110910=CARTESIAN_POINT('Ctrl Pts',(8.54791712013338,8.27920430747298,-14.5467603604118)) ;
#110911=CARTESIAN_POINT('Ctrl Pts',(8.54806168001143,8.28008011045357,-14.5442463372674)) ;
#110912=CARTESIAN_POINT('Ctrl Pts',(8.54818998754194,8.28086237513967,-14.5417186838585)) ;
#110913=CARTESIAN_POINT('Ctrl Pts',(8.54824194926751,8.28117917511843,-14.5406950398664)) ;
#110914=CARTESIAN_POINT('Ctrl Pts',(8.54829140719363,8.28148078264973,-14.5396686742902)) ;
#110915=CARTESIAN_POINT('Ctrl Pts',(8.54833813644415,8.28176759858575,-14.5386396299772)) ;
#110916=CARTESIAN_POINT('Ctrl Pts',(8.5485006132477,8.28276485268188,-14.5350616605292)) ;
#110917=CARTESIAN_POINT('Ctrl Pts',(8.54863339756394,8.28360845633773,-14.5313501235293)) ;
#110918=CARTESIAN_POINT('Ctrl Pts',(8.54873421749655,8.28426438239332,-14.5276130867584)) ;
#110919=CARTESIAN_POINT('Ctrl Pts',(8.54878752953696,8.28461122607269,-14.5256369987946)) ;
#110920=CARTESIAN_POINT('Ctrl Pts',(8.54883168679926,8.28490640714037,-14.523654082074)) ;
#110921=CARTESIAN_POINT('Ctrl Pts',(8.54886500248133,8.28515040605085,-14.5216818590294)) ;
#110922=CARTESIAN_POINT('Ctrl Pts',(8.54887385422351,8.28521523484358,-14.5211578532513)) ;
#110923=CARTESIAN_POINT('Ctrl Pts',(8.54888411330031,8.285275121517,-14.5206350091922)) ;
#110924=CARTESIAN_POINT('Ctrl Pts',(8.54889386083023,8.2853314308609,-14.5201120867862)) ;
#110925=CARTESIAN_POINT('Ctrl Pts',(8.54894969070932,8.28565394783543,-14.5171170003469)) ;
#110926=CARTESIAN_POINT('Ctrl Pts',(8.5489793513821,8.28586680424119,-14.514098636383)) ;
#110927=CARTESIAN_POINT('Ctrl Pts',(8.54899968230029,8.28595875954336,-14.5110675778014)) ;
#110928=CARTESIAN_POINT('Ctrl Pts',(8.54900356561227,8.28597632348829,-14.5104886297175)) ;
#110929=CARTESIAN_POINT('Ctrl Pts',(8.54900713937599,8.28598945835116,-14.5099093088042)) ;
#110930=CARTESIAN_POINT('Ctrl Pts',(8.54901057288909,8.2859980637762,-14.5093298402185)) ;
#110931=CARTESIAN_POINT('Ctrl Pts',(8.54902784271198,8.28604134718934,-14.5064152394759)) ;
#110932=CARTESIAN_POINT('Ctrl Pts',(8.54901619593281,8.28598556136223,-14.5035157757219)) ;
#110933=CARTESIAN_POINT('Ctrl Pts',(8.54898431260111,8.28582669412323,-14.5006064286757)) ;
#110934=CARTESIAN_POINT('Ctrl Pts',(8.54893914418925,8.2856016304144,-14.4964848209696)) ;
#110935=CARTESIAN_POINT('Ctrl Pts',(8.54884805310402,8.28517290646441,-14.4923770999664)) ;
#110936=CARTESIAN_POINT('Ctrl Pts',(8.54869940582912,8.28455561418415,-14.4883070774133)) ;
#110937=CARTESIAN_POINT('Ctrl Pts',(8.54864697316335,8.28433787538047,-14.4868714498022)) ;
#110938=CARTESIAN_POINT('Ctrl Pts',(8.54858736435354,8.28409676597413,-14.4854408395922)) ;
#110939=CARTESIAN_POINT('Ctrl Pts',(8.54851996240545,8.28383343043592,-14.4840172030853)) ;
#110940=CARTESIAN_POINT('Origin',(8.4,6.65,-17.78)) ;
#110941=CARTESIAN_POINT('Origin',(8.4,6.65,-14.6993219981003)) ;
#110942=CARTESIAN_POINT('Origin',(8.49172374697018,6.65,-17.78)) ;
#110943=CARTESIAN_POINT('Origin',(8.49225485644025,6.63809817934705,-14.4670086283546)) ;
#110944=CARTESIAN_POINT('Origin',(8.6,4.35421736843756,-14.6997127088383)) ;
#110945=CARTESIAN_POINT('Origin',(8.6,6.66256607592813,-14.6997127088383)) ;
#110946=CARTESIAN_POINT('Ctrl Pts',(8.5013487493624,6.65217253603386,-14.7159852560807)) ;
#110947=CARTESIAN_POINT('Ctrl Pts',(8.50315244876585,6.54997127577019,-14.7165863692585)) ;
#110948=CARTESIAN_POINT('Ctrl Pts',(8.4026944413366,6.55000000392136,-14.7315964965758)) ;
#110949=CARTESIAN_POINT('Ctrl Pts',(8.49631753783951,6.64933701877093,-14.6850156523956)) ;
#110950=CARTESIAN_POINT('Ctrl Pts',(8.49707874924869,6.54997270174421,-14.6839612234984)) ;
#110951=CARTESIAN_POINT('Ctrl Pts',(8.39261127161985,6.55000000381175,-14.6725550208108)) ;
#110952=CARTESIAN_POINT('Ctrl Pts',(8.50556246021206,6.65075235208957,-14.6560110455015)) ;
#110953=CARTESIAN_POINT('Ctrl Pts',(8.50253957946711,6.54997202229479,-14.6596441304545)) ;
#110954=CARTESIAN_POINT('Ctrl Pts',(8.41103525938989,6.55000000386643,-14.6113383496345)) ;
#110955=CARTESIAN_POINT('Ctrl Pts',(8.52891970071471,6.63645479210458,-14.6265271584828)) ;
#110956=CARTESIAN_POINT('Ctrl Pts',(8.52027792490147,6.54997752826669,-14.6184049399612)) ;
#110957=CARTESIAN_POINT('Ctrl Pts',(8.4576425585103,6.5500000033157,-14.557390101583)) ;
#110958=CARTESIAN_POINT('Ctrl Pts',(8.53324635448929,6.63340383613806,-14.6217820657382)) ;
#110959=CARTESIAN_POINT('Ctrl Pts',(8.52338394863781,6.54997861189312,-14.6115733138909)) ;
#110960=CARTESIAN_POINT('Ctrl Pts',(8.46627109069291,6.55000000319827,-14.5490047485327)) ;
#110961=CARTESIAN_POINT('Ctrl Pts',(8.5425433201124,6.62325922024832,-14.6111417482178)) ;
#110962=CARTESIAN_POINT('Ctrl Pts',(8.53005572430513,6.54998198465677,-14.5949326424681)) ;
#110963=CARTESIAN_POINT('Ctrl Pts',(8.48480454940903,6.55000000280808,-14.5336278088231)) ;
#110964=CARTESIAN_POINT('Ctrl Pts',(8.54755771953123,6.61716872587381,-14.6071385438774)) ;
#110965=CARTESIAN_POINT('Ctrl Pts',(8.53352383957156,6.54998388968237,-14.5870066149148)) ;
#110966=CARTESIAN_POINT('Ctrl Pts',(8.49480263348501,6.55000000257396,-14.5267172762992)) ;
#110967=CARTESIAN_POINT('Ctrl Pts',(8.55524400651032,6.59355301617583,-14.5864805698954)) ;
#110968=CARTESIAN_POINT('Ctrl Pts',(8.53873552501328,6.54999036710749,-14.5612948588094)) ;
#110969=CARTESIAN_POINT('Ctrl Pts',(8.51008526949052,6.55000000166752,-14.5167757494185)) ;
#110970=CARTESIAN_POINT('Ctrl Pts',(8.55791451833573,6.58083494429022,-14.5784270674639)) ;
#110971=CARTESIAN_POINT('Ctrl Pts',(8.54027978136636,6.54999344602542,-14.5515790288343)) ;
#110972=CARTESIAN_POINT('Ctrl Pts',(8.51542462880457,6.55000000118004,-14.5138063443386)) ;
#110973=CARTESIAN_POINT('Ctrl Pts',(8.56122429319342,6.56135755929237,-14.5354165389634)) ;
#110974=CARTESIAN_POINT('Ctrl Pts',(8.54270214007071,6.54999771321876,-14.5220999056442)) ;
#110975=CARTESIAN_POINT('Ctrl Pts',(8.52194436340203,6.55000000043437,-14.5072674436739)) ;
#110976=CARTESIAN_POINT('Ctrl Pts',(8.56215003896757,6.55689889598544,-14.5125513447562)) ;
#110977=CARTESIAN_POINT('Ctrl Pts',(8.54355112280985,6.54999862629018,-14.5085854140215)) ;
#110978=CARTESIAN_POINT('Ctrl Pts',(8.52363168464777,6.55000000026381,-14.5041937607945)) ;
#110979=CARTESIAN_POINT('Ctrl Pts',(8.56153943432818,6.55906352913393,-14.4772061237909)) ;
#110980=CARTESIAN_POINT('Ctrl Pts',(8.54309854033144,6.5499981870035,-14.4871631682685)) ;
#110981=CARTESIAN_POINT('Ctrl Pts',(8.52276767133745,6.5500000003466,-14.49816751318)) ;
#110982=CARTESIAN_POINT('Ctrl Pts',(8.56059123720043,6.56303220640812,-14.4654869464625)) ;
#110983=CARTESIAN_POINT('Ctrl Pts',(8.54200379397878,6.54999736403672,-14.4794720470657)) ;
#110984=CARTESIAN_POINT('Ctrl Pts',(8.52069177703238,6.55000000049844,-14.4955213437361)) ;
#110985=CARTESIAN_POINT('Ctrl Pts',(8.55750819780173,6.57321782814892,-14.4388078145325)) ;
#110986=CARTESIAN_POINT('Ctrl Pts',(8.53873610184734,6.54999517041881,-14.4605268596429)) ;
#110987=CARTESIAN_POINT('Ctrl Pts',(8.51454797734041,6.55000000088831,-14.4886566308241)) ;
#110988=CARTESIAN_POINT('Ctrl Pts',(8.55505442469283,6.5799017379831,-14.4292926744612)) ;
#110989=CARTESIAN_POINT('Ctrl Pts',(8.53621107118182,6.54999365791211,-14.4521766604066)) ;
#110990=CARTESIAN_POINT('Ctrl Pts',(8.50963525726155,6.5500000011443,-14.4848261829157)) ;
#110991=CARTESIAN_POINT('Ctrl Pts',(8.55022399280474,6.59153973477788,-14.4129352059185)) ;
#110992=CARTESIAN_POINT('Ctrl Pts',(8.53156015545169,6.54999086985382,-14.4366211671793)) ;
#110993=CARTESIAN_POINT('Ctrl Pts',(8.49999539447557,6.55000000159032,-14.4771278236794)) ;
#110994=CARTESIAN_POINT('Ctrl Pts',(8.54779538881609,6.59665349532942,-14.4069161916983)) ;
#110995=CARTESIAN_POINT('Ctrl Pts',(8.5293657515114,6.54998957391999,-14.4299955473559)) ;
#110996=CARTESIAN_POINT('Ctrl Pts',(8.49512741158075,6.55000000178643,-14.4733364158986)) ;
#110997=CARTESIAN_POINT('Ctrl Pts',(8.54538355337156,6.6012117118503,-14.4016751744842)) ;
#110998=CARTESIAN_POINT('Ctrl Pts',(8.52733415536173,6.54998837980797,-14.4238983572099)) ;
#110999=CARTESIAN_POINT('Ctrl Pts',(8.49033880598513,6.55000000196131,-14.4694485970987)) ;
#111000=CARTESIAN_POINT('',(8.54582344182381,6.6163536986167,-14.606063651573)) ;
#111001=CARTESIAN_POINT('Ctrl Pts',(8.54582344182381,6.6163536986167,-14.606063651573)) ;
#111002=CARTESIAN_POINT('Ctrl Pts',(8.54493595163518,6.61793460914655,-14.6073940762099)) ;
#111003=CARTESIAN_POINT('Ctrl Pts',(8.5439844817107,6.61948114927954,-14.6087173928307)) ;
#111004=CARTESIAN_POINT('Ctrl Pts',(8.54296332801272,6.6209780844369,-14.6100407367798)) ;
#111005=CARTESIAN_POINT('Ctrl Pts',(8.53827263106763,6.62785429629763,-14.6161195527619)) ;
#111006=CARTESIAN_POINT('Ctrl Pts',(8.53198779426187,6.63349037496299,-14.6226115685244)) ;
#111007=CARTESIAN_POINT('Ctrl Pts',(8.5259873730411,6.63731070037229,-14.6300705892422)) ;
#111008=CARTESIAN_POINT('Ctrl Pts',(8.52000560405467,6.64111915034781,-14.6375064236874)) ;
#111009=CARTESIAN_POINT('Ctrl Pts',(8.51430181273566,6.64349626850742,-14.6460376473014)) ;
#111010=CARTESIAN_POINT('Ctrl Pts',(8.50998586672548,6.64522349213896,-14.6552009869701)) ;
#111011=CARTESIAN_POINT('Ctrl Pts',(8.50534188065424,6.64708199603772,-14.6650608002501)) ;
#111012=CARTESIAN_POINT('Ctrl Pts',(8.50212992821339,6.64824261275105,-14.6758875436748)) ;
#111013=CARTESIAN_POINT('Ctrl Pts',(8.50077314609738,6.64911992656046,-14.6868249119168)) ;
#111014=CARTESIAN_POINT('Ctrl Pts',(8.50025986706873,6.64945181977648,-14.6909625856677)) ;
#111015=CARTESIAN_POINT('Ctrl Pts',(8.50000017127793,6.64974165917873,-14.6951432551012)) ;
#111016=CARTESIAN_POINT('Ctrl Pts',(8.5000000000847,6.64999974464545,-14.6993178674956)) ;
#111017=CARTESIAN_POINT('',(8.55242393572493,6.60106172182544,-14.5932420987161)) ;
#111018=CARTESIAN_POINT('Ctrl Pts',(8.55241775170034,6.60106807917178,-14.5932328161544)) ;
#111019=CARTESIAN_POINT('Ctrl Pts',(8.55072388788561,6.6061902674336,-14.5977214769524)) ;
#111020=CARTESIAN_POINT('Ctrl Pts',(8.5485829404857,6.61143812822775,-14.6019269241449)) ;
#111021=CARTESIAN_POINT('Ctrl Pts',(8.54582344182381,6.6163536986167,-14.606063651573)) ;
#111022=CARTESIAN_POINT('Ctrl Pts',(8.55635360773813,6.58637108369505,-14.5786323907338)) ;
#111023=CARTESIAN_POINT('Ctrl Pts',(8.55606387390182,6.58765239867387,-14.5801123828075)) ;
#111024=CARTESIAN_POINT('Ctrl Pts',(8.55575324501782,6.58896823902364,-14.5815659413336)) ;
#111025=CARTESIAN_POINT('Ctrl Pts',(8.55541196992766,6.59037241127512,-14.5830432049404)) ;
#111026=CARTESIAN_POINT('Ctrl Pts',(8.55524290008377,6.59106804711321,-14.5837750506995)) ;
#111027=CARTESIAN_POINT('Ctrl Pts',(8.55506631250718,6.59178496983026,-14.5845119588377)) ;
#111028=CARTESIAN_POINT('Ctrl Pts',(8.55488049708424,6.59252693597572,-14.585256277619)) ;
#111029=CARTESIAN_POINT('Ctrl Pts',(8.55445908016381,6.59420966544528,-14.586944342709)) ;
#111030=CARTESIAN_POINT('Ctrl Pts',(8.55403589309454,6.59584037906542,-14.5884883777225)) ;
#111031=CARTESIAN_POINT('Ctrl Pts',(8.55359592981642,6.59737680581864,-14.5899031562334)) ;
#111032=CARTESIAN_POINT('Ctrl Pts',(8.55324292160432,6.59860957066101,-14.591038315592)) ;
#111033=CARTESIAN_POINT('Ctrl Pts',(8.55287861047121,6.59978201473825,-14.5920910425072)) ;
#111034=CARTESIAN_POINT('Ctrl Pts',(8.55248933155914,6.60087815532547,-14.5930771269867)) ;
#111035=CARTESIAN_POINT('Ctrl Pts',(8.55246754857564,6.60093949235551,-14.5931323055779)) ;
#111036=CARTESIAN_POINT('Ctrl Pts',(8.55244574956029,6.60100068203154,-14.5931872962785)) ;
#111037=CARTESIAN_POINT('Ctrl Pts',(8.55242393572493,6.60106172182544,-14.5932420987161)) ;
#111038=CARTESIAN_POINT('Ctrl Pts',(8.5,6.66256607592813,-14.6997127088383)) ;
#111039=CARTESIAN_POINT('Ctrl Pts',(8.5,6.66256607592813,-14.615)) ;
#111040=CARTESIAN_POINT('Ctrl Pts',(8.58356010126947,6.66256607592813,-14.6010733164551)) ;
#111041=CARTESIAN_POINT('Ctrl Pts',(8.5,6.61011302719822,-14.6997127072628)) ;
#111042=CARTESIAN_POINT('Ctrl Pts',(8.50000000000005,6.63245216822976,-14.6185572365992)) ;
#111043=CARTESIAN_POINT('Ctrl Pts',(8.57941760042981,6.63563981885127,-14.6017637332617)) ;
#111044=CARTESIAN_POINT('Ctrl Pts',(8.5,6.55934573373326,-14.6788469099428)) ;
#111045=CARTESIAN_POINT('Ctrl Pts',(8.5,6.60054351783578,-14.6080813958278)) ;
#111046=CARTESIAN_POINT('Ctrl Pts',(8.57705842698407,6.60987578993433,-14.5917275280477)) ;
#111047=CARTESIAN_POINT('Ctrl Pts',(8.5,6.52274941072028,-14.6422505892797)) ;
#111048=CARTESIAN_POINT('Ctrl Pts',(8.5,6.57873105977929,-14.5862689402207)) ;
#111049=CARTESIAN_POINT('Ctrl Pts',(8.57705842661295,6.59157413088145,-14.5734258691185)) ;
#111050=CARTESIAN_POINT('Origin',(8.49172374697003,1.4,-17.78)) ;
#111051=CARTESIAN_POINT('Origin',(8.49172374697003,1.4,-13.2778583129651)) ;
#111052=CARTESIAN_POINT('Origin',(8.49172374697002,1.4,-13.2778583129651)) ;
#111053=CARTESIAN_POINT('Origin',(8.49172374697003,1.4,-13.2778583129651)) ;
#111054=CARTESIAN_POINT('Ctrl Pts',(8.50816364570057,1.49863939238321,-13.2778583129651)) ;
#111055=CARTESIAN_POINT('Ctrl Pts',(8.51019246767907,1.4983012553868,-13.312927584071)) ;
#111056=CARTESIAN_POINT('Ctrl Pts',(8.50816364570057,1.47636598119991,-13.3402920109583)) ;
#111057=CARTESIAN_POINT('Ctrl Pts',(8.97755831131125,1.42040694811477,-13.2499486511544)) ;
#111058=CARTESIAN_POINT('Ctrl Pts',(8.97879997398683,1.42020000433581,-13.2845666731845)) ;
#111059=CARTESIAN_POINT('Ctrl Pts',(8.97755831689146,1.39869563385688,-13.311694816952)) ;
#111060=CARTESIAN_POINT('Ctrl Pts',(9.44698496305968,1.34216917282337,-13.2226313706305)) ;
#111061=CARTESIAN_POINT('Ctrl Pts',(9.44827639615881,1.3419539339721,-13.2567775286129)) ;
#111062=CARTESIAN_POINT('Ctrl Pts',(9.44698496887879,1.32097764915795,-13.2837229847104)) ;
#111063=CARTESIAN_POINT('Ctrl Pts',(9.91643989873053,1.26392668354489,-13.1958381198218)) ;
#111064=CARTESIAN_POINT('Ctrl Pts',(9.91830968165731,1.2636150530571,-13.229509344197)) ;
#111065=CARTESIAN_POINT('Ctrl Pts',(9.91643989873053,1.24322097942674,-13.256303564194)) ;
#111066=CARTESIAN_POINT('Origin',(9.9,1.16528729116168,-13.1958381198218)) ;
#111067=CARTESIAN_POINT('Origin',(9.9,1.16528729116168,-13.1958381198218)) ;
#111068=CARTESIAN_POINT('Origin',(-0.4,-3.36847777691809,-15.64)) ;
#111069=CARTESIAN_POINT('Origin',(-0.400000000000001,-3.36847777691809,
-15.64)) ;
#111070=CARTESIAN_POINT('Origin',(-0.4,-3.36847777691809,-15.64)) ;
#111071=CARTESIAN_POINT('Origin',(-0.400000000000001,-3.36847777691809,
-14.74)) ;
#111072=CARTESIAN_POINT('Origin',(-0.4,-3.36847777691809,-14.84)) ;
#111073=CARTESIAN_POINT('Origin',(-1.11032778078669,-3.36847777691809,-15.64)) ;
#111074=CARTESIAN_POINT('Origin',(0.4,-3.36847777691809,-15.64)) ;
#111075=CARTESIAN_POINT('Origin',(-0.400000000000001,-3.36847777691809,
-14.84)) ;
#111076=CARTESIAN_POINT('Origin',(-0.4,-3.36847777691809,-14.84)) ;
#111077=CARTESIAN_POINT('Origin',(0.400000000000001,-3.36847777691809,-15.64)) ;
#111078=CARTESIAN_POINT('Origin',(0.400000000000001,-3.36847777691809,-15.64)) ;
#111079=CARTESIAN_POINT('Origin',(1.5,-3.36847777691809,-14.84)) ;
#111080=CARTESIAN_POINT('Origin',(0.4,-3.36847777691809,-14.84)) ;
#111081=CARTESIAN_POINT('Origin',(0.4,-3.36847777691809,-14.74)) ;
#111082=CARTESIAN_POINT('Origin',(0.4,-3.36847777691809,-14.84)) ;
#111083=CARTESIAN_POINT('Origin',(0.4,-3.36847777691809,-14.84)) ;
#111084=CARTESIAN_POINT('Origin',(7.96847777691809,3.4,-15.64)) ;
#111085=CARTESIAN_POINT('Origin',(7.96847777691809,3.4,-15.64)) ;
#111086=CARTESIAN_POINT('Origin',(7.96847777691809,3.4,-15.64)) ;
#111087=CARTESIAN_POINT('Origin',(7.96847777691809,3.4,-14.74)) ;
#111088=CARTESIAN_POINT('Origin',(7.96847777691809,3.4,-14.84)) ;
#111089=CARTESIAN_POINT('Origin',(7.96847777691809,2.68967221921331,-15.64)) ;
#111090=CARTESIAN_POINT('Origin',(7.96847777691809,4.2,-15.64)) ;
#111091=CARTESIAN_POINT('Origin',(7.96847777691809,3.4,-14.84)) ;
#111092=CARTESIAN_POINT('Origin',(7.96847777691809,3.4,-14.84)) ;
#111093=CARTESIAN_POINT('Origin',(7.96847777691809,4.2,-15.64)) ;
#111094=CARTESIAN_POINT('Origin',(7.96847777691809,4.2,-15.64)) ;
#111095=CARTESIAN_POINT('Origin',(7.96847777691809,2.3,-14.84)) ;
#111096=CARTESIAN_POINT('Origin',(7.96847777691809,4.2,-14.84)) ;
#111097=CARTESIAN_POINT('Origin',(7.96847777691809,4.2,-14.74)) ;
#111098=CARTESIAN_POINT('Origin',(7.96847777691809,4.2,-14.84)) ;
#111099=CARTESIAN_POINT('Origin',(7.96847777691809,4.2,-14.84)) ;
#111100=CARTESIAN_POINT('Origin',(8.49172374697003,1.4,-17.78)) ;
#111101=CARTESIAN_POINT('Origin',(8.49172374697003,1.4,-17.2021416870349)) ;
#111102=CARTESIAN_POINT('Origin',(8.49172374697002,1.4,-17.2021416870349)) ;
#111103=CARTESIAN_POINT('Origin',(8.49172374697003,1.39999999999989,-17.2021416870347)) ;
#111104=CARTESIAN_POINT('Ctrl Pts',(8.50816364570058,1.47636598119991,-17.1397079890417)) ;
#111105=CARTESIAN_POINT('Ctrl Pts',(8.51019246767908,1.4983012553868,-17.167072415929)) ;
#111106=CARTESIAN_POINT('Ctrl Pts',(8.50816364570058,1.49863939238321,-17.2021416870349)) ;
#111107=CARTESIAN_POINT('Ctrl Pts',(8.9775583168915,1.39869563385713,-17.1683051830483)) ;
#111108=CARTESIAN_POINT('Ctrl Pts',(8.97879997398667,1.42020000433563,-17.1954333268176)) ;
#111109=CARTESIAN_POINT('Ctrl Pts',(8.97755831131135,1.42040694811475,-17.2300513488443)) ;
#111110=CARTESIAN_POINT('Ctrl Pts',(9.44698496887878,1.32097764915799,-17.1962770152897)) ;
#111111=CARTESIAN_POINT('Ctrl Pts',(9.4482763961588,1.34195393397339,-17.2232224713911)) ;
#111112=CARTESIAN_POINT('Ctrl Pts',(9.44698496305964,1.34216917282337,-17.2573686293698)) ;
#111113=CARTESIAN_POINT('Ctrl Pts',(9.91643989873053,1.24322097942674,-17.223696435806)) ;
#111114=CARTESIAN_POINT('Ctrl Pts',(9.91830968165732,1.26361505305709,-17.250490655803)) ;
#111115=CARTESIAN_POINT('Ctrl Pts',(9.91643989873053,1.26392668354489,-17.2841618801782)) ;
#111116=CARTESIAN_POINT('Origin',(9.9,1.16528729116168,-17.2841618801782)) ;
#111117=CARTESIAN_POINT('Origin',(9.9,1.16528729116168,-17.2841618801782)) ;
#111118=CARTESIAN_POINT('Origin',(8.48377223398316,8.2,-17.78)) ;
#111119=CARTESIAN_POINT('Origin',(8.48238055012102,8.20007134086553,-14.4931789299182)) ;
#111120=CARTESIAN_POINT('Ctrl Pts',(8.40201662970149,8.3,-14.7259759779213)) ;
#111121=CARTESIAN_POINT('Ctrl Pts',(8.50299337454948,8.3,-14.7126748112635)) ;
#111122=CARTESIAN_POINT('Ctrl Pts',(8.50100123624931,8.19773961376461,-14.7126888461177)) ;
#111123=CARTESIAN_POINT('Ctrl Pts',(8.3945412979896,8.3,-14.6744981813506)) ;
#111124=CARTESIAN_POINT('Ctrl Pts',(8.4969787523768,8.3,-14.6853741113346)) ;
#111125=CARTESIAN_POINT('Ctrl Pts',(8.49727262260755,8.20135231978531,-14.6850670639623)) ;
#111126=CARTESIAN_POINT('Ctrl Pts',(8.40820218948345,8.3,-14.6220253635242)) ;
#111127=CARTESIAN_POINT('Ctrl Pts',(8.49818669687003,8.3,-14.6624717278012)) ;
#111128=CARTESIAN_POINT('Ctrl Pts',(8.50412619268405,8.20300739730713,-14.6603884100247)) ;
#111129=CARTESIAN_POINT('Ctrl Pts',(8.44304134766321,8.3,-14.5709969330871)) ;
#111130=CARTESIAN_POINT('Ctrl Pts',(8.50894174387209,8.3,-14.6208550553806)) ;
#111131=CARTESIAN_POINT('Ctrl Pts',(8.52157716465941,8.21896555381605,-14.6301661266503)) ;
#111132=CARTESIAN_POINT('Ctrl Pts',(8.44963266995283,8.3,-14.5626678319782)) ;
#111133=CARTESIAN_POINT('Ctrl Pts',(8.51095981317517,8.3,-14.6137494404835)) ;
#111134=CARTESIAN_POINT('Ctrl Pts',(8.52487915500777,8.22226238914488,-14.6249516180519)) ;
#111135=CARTESIAN_POINT('Ctrl Pts',(8.46372306360151,8.3,-14.5469547263199)) ;
#111136=CARTESIAN_POINT('Ctrl Pts',(8.51547368264944,8.3,-14.5976327910559)) ;
#111137=CARTESIAN_POINT('Ctrl Pts',(8.53193863144478,8.23129792829965,-14.6133174783855)) ;
#111138=CARTESIAN_POINT('Ctrl Pts',(8.47128983770084,8.3,-14.5395586271464)) ;
#111139=CARTESIAN_POINT('Ctrl Pts',(8.5179623704237,8.3,-14.5892464949127)) ;
#111140=CARTESIAN_POINT('Ctrl Pts',(8.53572833262715,8.2367734386236,-14.6074295885077)) ;
#111141=CARTESIAN_POINT('Ctrl Pts',(8.48287565264706,8.3,-14.5287307948332)) ;
#111142=CARTESIAN_POINT('Ctrl Pts',(8.52168214469875,8.3,-14.57074351943)) ;
#111143=CARTESIAN_POINT('Ctrl Pts',(8.54153766811345,8.25077321967987,-14.5920449871074)) ;
#111144=CARTESIAN_POINT('Ctrl Pts',(8.48680760428677,8.3,-14.525187297402)) ;
#111145=CARTESIAN_POINT('Ctrl Pts',(8.52287759291297,8.3,-14.5641435049317)) ;
#111146=CARTESIAN_POINT('Ctrl Pts',(8.54350322705384,8.2564691763754,-14.5862622666034)) ;
#111147=CARTESIAN_POINT('Ctrl Pts',(8.49230810302881,8.3,-14.5194953499955)) ;
#111148=CARTESIAN_POINT('Ctrl Pts',(8.52426411271138,8.3,-14.5485665246336)) ;
#111149=CARTESIAN_POINT('Ctrl Pts',(8.54627296401923,8.26866384868898,-14.5685525693616)) ;
#111150=CARTESIAN_POINT('Ctrl Pts',(8.49410170711667,8.3,-14.517526518934)) ;
#111151=CARTESIAN_POINT('Ctrl Pts',(8.52463604790914,8.3,-14.5424055253652)) ;
#111152=CARTESIAN_POINT('Ctrl Pts',(8.54716490137964,8.27360757863439,-14.5607959594826)) ;
#111153=CARTESIAN_POINT('Ctrl Pts',(8.49698869685298,8.3,-14.5130732788095)) ;
#111154=CARTESIAN_POINT('Ctrl Pts',(8.52523118911551,8.3,-14.5265929344383)) ;
#111155=CARTESIAN_POINT('Ctrl Pts',(8.54862931231184,8.28262305001771,-14.5378413492704)) ;
#111156=CARTESIAN_POINT('Ctrl Pts',(8.4979868777125,8.3,-14.5105165211566)) ;
#111157=CARTESIAN_POINT('Ctrl Pts',(8.52551930315386,8.3,-14.5169062760438)) ;
#111158=CARTESIAN_POINT('Ctrl Pts',(8.54912969489065,8.28574379441723,-14.5223818974932)) ;
#111159=CARTESIAN_POINT('Ctrl Pts',(8.49821791151748,8.3,-14.5025795709374)) ;
#111160=CARTESIAN_POINT('Ctrl Pts',(8.52559423327562,8.3,-14.4921891247049)) ;
#111161=CARTESIAN_POINT('Ctrl Pts',(8.54922875625408,8.28635135062007,-14.4832386700469)) ;
#111162=CARTESIAN_POINT('Ctrl Pts',(8.49537847603514,8.3,-14.4976469108458)) ;
#111163=CARTESIAN_POINT('Ctrl Pts',(8.5243933105344,8.3,-14.4814732749821)) ;
#111164=CARTESIAN_POINT('Ctrl Pts',(8.54781890418529,8.2804054867288,-14.468471793372)) ;
#111165=CARTESIAN_POINT('Ctrl Pts',(8.48955273785442,8.3,-14.4889114034569)) ;
#111166=CARTESIAN_POINT('Ctrl Pts',(8.52168703568126,8.29999999999999,-14.4640525851282)) ;
#111167=CARTESIAN_POINT('Ctrl Pts',(8.54489815533715,8.27194212599122,-14.4461670077071)) ;
#111168=CARTESIAN_POINT('Ctrl Pts',(8.48620077197361,8.3,-14.4848263075048)) ;
#111169=CARTESIAN_POINT('Ctrl Pts',(8.52012703453236,8.30000000000001,-14.4571073328933)) ;
#111170=CARTESIAN_POINT('Ctrl Pts',(8.54324008387895,8.26788967346963,-14.4383142356384)) ;
#111171=CARTESIAN_POINT('Ctrl Pts',(8.48280151347419,8.3,-14.4807911096407)) ;
#111172=CARTESIAN_POINT('Ctrl Pts',(8.51858761497412,8.3,-14.4506520257852)) ;
#111173=CARTESIAN_POINT('Ctrl Pts',(8.54152015125555,8.26408224232382,-14.4313382250347)) ;
#111174=CARTESIAN_POINT('Origin',(8.4,8.2,-14.697927110149)) ;
#111175=CARTESIAN_POINT('Origin',(8.4,8.2,-15.865)) ;
#111176=CARTESIAN_POINT('Origin',(8.4,8.2,-15.782072889851)) ;
#111177=CARTESIAN_POINT('Ctrl Pts',(8.50101530037395,8.19768718256762,-15.7672017745814)) ;
#111178=CARTESIAN_POINT('Ctrl Pts',(8.50305639000873,8.3,-15.7672198113572)) ;
#111179=CARTESIAN_POINT('Ctrl Pts',(8.40204633857705,8.3,-15.7538202021254)) ;
#111180=CARTESIAN_POINT('Ctrl Pts',(8.49725464441632,8.20131038948436,-15.7948679119096)) ;
#111181=CARTESIAN_POINT('Ctrl Pts',(8.49701391805272,8.3,-15.7945609423404)) ;
#111182=CARTESIAN_POINT('Ctrl Pts',(8.39450526457597,8.3,-15.8053632910712)) ;
#111183=CARTESIAN_POINT('Ctrl Pts',(8.5041093504131,8.20295267265881,-15.8195792968114)) ;
#111184=CARTESIAN_POINT('Ctrl Pts',(8.498207495215,8.3,-15.8174643378906)) ;
#111185=CARTESIAN_POINT('Ctrl Pts',(8.40816401923481,8.3,-15.8579187290434)) ;
#111186=CARTESIAN_POINT('Ctrl Pts',(8.52158236570989,8.21893216789649,-15.8498300407758)) ;
#111187=CARTESIAN_POINT('Ctrl Pts',(8.50896456566521,8.3,-15.8591276783841)) ;
#111188=CARTESIAN_POINT('Ctrl Pts',(8.44304134766321,8.3,-15.9090030669129)) ;
#111189=CARTESIAN_POINT('Ctrl Pts',(8.5248849650705,8.22222991631201,-15.8550437061782)) ;
#111190=CARTESIAN_POINT('Ctrl Pts',(8.51098076140206,8.3,-15.8662331109763)) ;
#111191=CARTESIAN_POINT('Ctrl Pts',(8.44963266995282,8.3,-15.9173321680218)) ;
#111192=CARTESIAN_POINT('Ctrl Pts',(8.53194575580938,8.23126818558572,-15.8666757349666)) ;
#111193=CARTESIAN_POINT('Ctrl Pts',(8.51549074202138,8.3,-15.8823505031351)) ;
#111194=CARTESIAN_POINT('Ctrl Pts',(8.46372306360152,8.3,-15.9330452736801)) ;
#111195=CARTESIAN_POINT('Ctrl Pts',(8.53573618291037,8.23674548871788,-15.8725623770273)) ;
#111196=CARTESIAN_POINT('Ctrl Pts',(8.51797743940283,8.3,-15.8907374625586)) ;
#111197=CARTESIAN_POINT('Ctrl Pts',(8.47128983770083,8.3,-15.9404413728536)) ;
#111198=CARTESIAN_POINT('Ctrl Pts',(8.54154687836688,8.25075037830458,-15.8879451319455)) ;
#111199=CARTESIAN_POINT('Ctrl Pts',(8.52169408444524,8.3,-15.9092435543493)) ;
#111200=CARTESIAN_POINT('Ctrl Pts',(8.48287565264706,8.3,-15.9512692051668)) ;
#111201=CARTESIAN_POINT('Ctrl Pts',(8.54351297666181,8.25644859419422,-15.8937272780162)) ;
#111202=CARTESIAN_POINT('Ctrl Pts',(8.52288848488736,8.3,-15.9158447315488)) ;
#111203=CARTESIAN_POINT('Ctrl Pts',(8.48680760428676,8.3,-15.954812702598)) ;
#111204=CARTESIAN_POINT('Ctrl Pts',(8.54628376412584,8.26864846827403,-15.9114376231601)) ;
#111205=CARTESIAN_POINT('Ctrl Pts',(8.52427341038692,8.3,-15.9314250170403)) ;
#111206=CARTESIAN_POINT('Ctrl Pts',(8.4923081030288,8.3,-15.9605046500045)) ;
#111207=CARTESIAN_POINT('Ctrl Pts',(8.54717611873857,8.27359443500938,-15.9191948837187)) ;
#111208=CARTESIAN_POINT('Ctrl Pts',(8.52464480444821,8.3,-15.9375873399142)) ;
#111209=CARTESIAN_POINT('Ctrl Pts',(8.49410170711667,8.3,-15.962473481066)) ;
#111210=CARTESIAN_POINT('Ctrl Pts',(8.54864126180654,8.28261417405722,-15.9421529061248)) ;
#111211=CARTESIAN_POINT('Ctrl Pts',(8.52523908688552,8.3,-15.9534032849063)) ;
#111212=CARTESIAN_POINT('Ctrl Pts',(8.49698869685298,8.3,-15.9669267211905)) ;
#111213=CARTESIAN_POINT('Ctrl Pts',(8.5491418548716,8.28573645090425,-15.9576152824162)) ;
#111214=CARTESIAN_POINT('Ctrl Pts',(8.52552693815802,8.3,-15.9630919520163)) ;
#111215=CARTESIAN_POINT('Ctrl Pts',(8.49798687771249,8.3,-15.9694834788434)) ;
#111216=CARTESIAN_POINT('Ctrl Pts',(8.54924094958847,8.28634430798885,-15.9967659475983)) ;
#111217=CARTESIAN_POINT('Ctrl Pts',(8.52560181204939,8.3,-15.9878137517531)) ;
#111218=CARTESIAN_POINT('Ctrl Pts',(8.49821791151747,8.3,-15.9774204290626)) ;
#111219=CARTESIAN_POINT('Ctrl Pts',(8.54783079466743,8.28039553911293,-16.0115348059813)) ;
#111220=CARTESIAN_POINT('Ctrl Pts',(8.52440147378976,8.3,-15.9985312754323)) ;
#111221=CARTESIAN_POINT('Ctrl Pts',(8.49537847603514,8.3,-15.9823530891542)) ;
#111222=CARTESIAN_POINT('Ctrl Pts',(8.54465883986931,8.27120119512637,-16.0357571947032)) ;
#111223=CARTESIAN_POINT('Ctrl Pts',(8.52145785975945,8.3,-16.0174902783301)) ;
#111224=CARTESIAN_POINT('Ctrl Pts',(8.48905244827038,8.3,-15.9918387647145)) ;
#111225=CARTESIAN_POINT('Ctrl Pts',(8.54267599402786,8.26648669506697,-16.0442949904305)) ;
#111226=CARTESIAN_POINT('Ctrl Pts',(8.51958784692425,8.3,-16.0252641321447)) ;
#111227=CARTESIAN_POINT('Ctrl Pts',(8.48503640902804,8.3,-15.9965685970659)) ;
#111228=CARTESIAN_POINT('Ctrl Pts',(8.54064021294342,8.26212437554839,-16.0522000298239)) ;
#111229=CARTESIAN_POINT('Ctrl Pts',(8.51779796763698,8.3,-16.0326895170151)) ;
#111230=CARTESIAN_POINT('Ctrl Pts',(8.48104783026775,8.3,-16.0012848074951)) ;
#111231=CARTESIAN_POINT('Origin',(8.4823805486149,8.20007133319196,-15.9868210687046)) ;
#111232=CARTESIAN_POINT('Origin',(8.48377223398316,8.2,-17.78)) ;
#111233=CARTESIAN_POINT('Ctrl Pts',(8.55305389383868,6.58518362856711,-19.6598163714329)) ;
#111234=CARTESIAN_POINT('Ctrl Pts',(8.56447181517253,6.58947636230805,-19.6555236376919)) ;
#111235=CARTESIAN_POINT('Ctrl Pts',(8.57705842661295,6.59157413088145,-19.6534258691185)) ;
#111236=CARTESIAN_POINT('Ctrl Pts',(8.55305102515203,6.55898702014122,-19.6336204597774)) ;
#111237=CARTESIAN_POINT('Ctrl Pts',(8.56446969712857,6.56479854221787,-19.6308465230911)) ;
#111238=CARTESIAN_POINT('Ctrl Pts',(8.57705842709774,6.56766897765924,-19.6295207157347)) ;
#111239=CARTESIAN_POINT('Ctrl Pts',(8.55608440539073,6.54967077654141,-19.5934724260347)) ;
#111240=CARTESIAN_POINT('Ctrl Pts',(8.56803673427362,6.55578248257734,-19.5931311242349)) ;
#111241=CARTESIAN_POINT('Ctrl Pts',(8.58110225049762,6.55837193275,-19.5932648466505)) ;
#111242=CARTESIAN_POINT('Ctrl Pts',(8.56106007075016,6.56033186051354,-19.5569784615962)) ;
#111243=CARTESIAN_POINT('Ctrl Pts',(8.57385418571952,6.56560017282096,-19.5582038837617)) ;
#111244=CARTESIAN_POINT('Ctrl Pts',(8.58763814880121,6.56727264871055,-19.5585929056925)) ;
#111245=CARTESIAN_POINT('',(8.56104219912065,6.56017369985344,-19.5576338509444)) ;
#111246=CARTESIAN_POINT('',(8.55704445183397,6.58320973295693,-19.6548316411919)) ;
#111247=CARTESIAN_POINT('Ctrl Pts',(8.56104219912065,6.56017369985344,-19.5576338509444)) ;
#111248=CARTESIAN_POINT('Ctrl Pts',(8.56172006948825,6.55755272988493,-19.5705099834262)) ;
#111249=CARTESIAN_POINT('Ctrl Pts',(8.56178854742204,6.55691761311389,-19.5840188634591)) ;
#111250=CARTESIAN_POINT('Ctrl Pts',(8.56147572200372,6.55855061087387,-19.5970710371545)) ;
#111251=CARTESIAN_POINT('Ctrl Pts',(8.56116227470662,6.56018685493862,-19.6101491578135)) ;
#111252=CARTESIAN_POINT('Ctrl Pts',(8.5604843297899,6.56417103596015,-19.6231290791339)) ;
#111253=CARTESIAN_POINT('Ctrl Pts',(8.55945615587251,6.57017322470283,-19.6348222126965)) ;
#111254=CARTESIAN_POINT('Ctrl Pts',(8.55883284154062,6.57381195760855,-19.6419109917552)) ;
#111255=CARTESIAN_POINT('Ctrl Pts',(8.55807185541711,6.57823677723133,-19.6486350483951)) ;
#111256=CARTESIAN_POINT('Ctrl Pts',(8.55704487707431,6.58320791316478,-19.6548324621192)) ;
#111257=CARTESIAN_POINT('',(8.55635403291171,6.58636921675995,-19.6586302321744)) ;
#111258=CARTESIAN_POINT('Origin',(8.54420290085246,6.6281733092357,-19.6219411204917)) ;
#111259=CARTESIAN_POINT('',(8.57705842661295,6.59157413088145,-19.6534258691185)) ;
#111260=CARTESIAN_POINT('Origin',(8.6,6.52274941072028,-19.7222505892797)) ;
#111261=CARTESIAN_POINT('',(8.58355189313841,6.56397635572684,-19.582433776426)) ;
#111262=CARTESIAN_POINT('Origin',(8.59777129281795,6.65641294722127,-19.5808822359315)) ;
#111263=CARTESIAN_POINT('Ctrl Pts',(8.56104311409705,6.56017375480329,-19.5576348093723)) ;
#111264=CARTESIAN_POINT('Ctrl Pts',(8.56569547918965,6.56094902085081,-19.5631223861694)) ;
#111265=CARTESIAN_POINT('Ctrl Pts',(8.57049938306333,6.56176641478979,-19.5685092513474)) ;
#111266=CARTESIAN_POINT('Ctrl Pts',(8.57538893105716,6.56259599225628,-19.5737862661385)) ;
#111267=CARTESIAN_POINT('Ctrl Pts',(8.57808773793835,6.56305388107911,-19.576698936972)) ;
#111268=CARTESIAN_POINT('Ctrl Pts',(8.58081254036867,6.56351521010419,-19.5795793793677)) ;
#111269=CARTESIAN_POINT('Ctrl Pts',(8.58355195315297,6.56397636517831,-19.5824336197205)) ;
#111270=CARTESIAN_POINT('Ctrl Pts',(8.5,8.3521616921714,-19.6724060982502)) ;
#111271=CARTESIAN_POINT('Ctrl Pts',(8.5,8.2900428850829,-19.641346694706)) ;
#111272=CARTESIAN_POINT('Ctrl Pts',(8.56507848521152,8.26835005667905,-19.630500280504)) ;
#111273=CARTESIAN_POINT('Ctrl Pts',(8.5,8.31945293993537,-19.7378235972687)) ;
#111274=CARTESIAN_POINT('Ctrl Pts',(8.5,8.26922013491147,-19.6829921887968)) ;
#111275=CARTESIAN_POINT('Ctrl Pts',(8.56507848600994,8.25199117628908,-19.6632180406186)) ;
#111276=CARTESIAN_POINT('Ctrl Pts',(8.5,8.24922766844392,-19.7797127068513)) ;
#111277=CARTESIAN_POINT('Ctrl Pts',(8.5,8.21777561643124,-19.7044773698221)) ;
#111278=CARTESIAN_POINT('Ctrl Pts',(8.57228151929428,8.2145120273235,-19.6829530801176)) ;
#111279=CARTESIAN_POINT('Ctrl Pts',(8.5,8.17221734381475,-19.7797127088383)) ;
#111280=CARTESIAN_POINT('Ctrl Pts',(8.5,8.17221734381475,-19.695)) ;
#111281=CARTESIAN_POINT('Ctrl Pts',(8.58356010126947,8.17221734381475,-19.6810733164551)) ;
#111282=CARTESIAN_POINT('',(8.50000000249538,8.20000280433619,-19.7779047436384)) ;
#111283=CARTESIAN_POINT('',(8.54742025481395,8.27608084305204,-19.6343656619559)) ;
#111284=CARTESIAN_POINT('Ctrl Pts',(8.50000000249538,8.20000280433619,-19.7779047436384)) ;
#111285=CARTESIAN_POINT('Ctrl Pts',(8.50000274011724,8.2015414376578,-19.7656354484511)) ;
#111286=CARTESIAN_POINT('Ctrl Pts',(8.50225788919789,8.20358050335012,-19.7532664749796)) ;
#111287=CARTESIAN_POINT('Ctrl Pts',(8.50614710304112,8.20657022673326,-19.7419159810139)) ;
#111288=CARTESIAN_POINT('Ctrl Pts',(8.51002595055128,8.20955198129041,-19.7305957407205)) ;
#111289=CARTESIAN_POINT('Ctrl Pts',(8.51564213392183,8.21362262975068,-19.7200461335207)) ;
#111290=CARTESIAN_POINT('Ctrl Pts',(8.52129493663065,8.21921832196825,-19.710621792234)) ;
#111291=CARTESIAN_POINT('Ctrl Pts',(8.52933132065201,8.22717351408127,-19.6972235489855)) ;
#111292=CARTESIAN_POINT('Ctrl Pts',(8.53683691159804,8.23885362788864,-19.6856624434434)) ;
#111293=CARTESIAN_POINT('Ctrl Pts',(8.54097226482464,8.25011947738646,-19.6728811696171)) ;
#111294=CARTESIAN_POINT('Ctrl Pts',(8.54447125915462,8.25965170869904,-19.6620667114082)) ;
#111295=CARTESIAN_POINT('Ctrl Pts',(8.54617119150717,8.26873789958222,-19.6499396101897)) ;
#111296=CARTESIAN_POINT('Ctrl Pts',(8.54724932284106,8.27506683274844,-19.6365664602513)) ;
#111297=CARTESIAN_POINT('Ctrl Pts',(8.54730817192851,8.27541229338911,-19.6358364956863)) ;
#111298=CARTESIAN_POINT('Ctrl Pts',(8.54736510616621,8.27575037116516,-19.635102832606)) ;
#111299=CARTESIAN_POINT('Ctrl Pts',(8.54742024083733,8.27608084608571,-19.6343656752073)) ;
#111300=CARTESIAN_POINT('',(8.56507848521152,8.26835005667905,-19.630500280504)) ;
#111301=CARTESIAN_POINT('Origin',(8.6,8.3521616921714,-19.6724060982502)) ;
#111302=CARTESIAN_POINT('',(8.58356010126947,8.17221734381475,-19.6810733164551)) ;
#111303=CARTESIAN_POINT('Origin',(8.59670327708558,8.16883734299673,-19.5870689695193)) ;
#111304=CARTESIAN_POINT('',(8.5,8.17221734381475,-19.7797127088383)) ;
#111305=CARTESIAN_POINT('Origin',(8.6,8.17221734381475,-19.7797127088383)) ;
#111306=CARTESIAN_POINT('Origin',(8.5,8.1664264877272,-19.5571077523216)) ;
#111307=CARTESIAN_POINT('Origin',(2.9,3.8,-20.32)) ;
#111308=CARTESIAN_POINT('',(3.,2.4,-20.32)) ;
#111309=CARTESIAN_POINT('Origin',(3.,3.8,-20.32)) ;
#111310=CARTESIAN_POINT('',(2.9,2.3,-20.32)) ;
#111311=CARTESIAN_POINT('Origin',(2.9,2.4,-20.32)) ;
#111312=CARTESIAN_POINT('Origin',(2.9,3.8,-20.32)) ;
#111313=CARTESIAN_POINT('Origin',(1.35,3.8,-20.32)) ;
#111314=CARTESIAN_POINT('',(1.35,2.3,-20.32)) ;
#111315=CARTESIAN_POINT('Origin',(1.35,3.8,-20.32)) ;
#111316=CARTESIAN_POINT('',(1.25,2.2,-20.32)) ;
#111317=CARTESIAN_POINT('Origin',(1.35,2.2,-20.32)) ;
#111318=CARTESIAN_POINT('Origin',(1.25,3.8,-20.32)) ;
#111319=CARTESIAN_POINT('Origin',(13.9153543900904,1.02736587339764,-19.47)) ;
#111320=CARTESIAN_POINT('',(1.15,1.02736587339764,-19.57)) ;
#111321=CARTESIAN_POINT('',(1.15,0.931757800066529,-19.4406896551724)) ;
#111322=CARTESIAN_POINT('Origin',(1.15,1.02736587339764,-19.47)) ;
#111323=CARTESIAN_POINT('',(-0.900000000000002,1.02736587339765,-19.57)) ;
#111324=CARTESIAN_POINT('',(-1.,1.02736587339765,-19.57)) ;
#111325=CARTESIAN_POINT('',(-0.900000000000002,0.982644513847654,-19.5594427191)) ;
#111326=CARTESIAN_POINT('Origin',(-0.900000000000002,1.02736587339765,-19.47)) ;
#111327=CARTESIAN_POINT('',(-0.900000000000002,0.93175780006653,-19.4406896551724)) ;
#111328=CARTESIAN_POINT('Origin',(-0.900000000000002,1.02736587339765,-19.47)) ;
#111329=CARTESIAN_POINT('',(13.9153543900904,0.931757800066525,-19.4406896551724)) ;
#111330=CARTESIAN_POINT('Origin',(13.9153543900904,1.02736587339764,-21.17)) ;
#111331=CARTESIAN_POINT('',(1.15,0.93175780006653,-21.1993103448276)) ;
#111332=CARTESIAN_POINT('',(1.15,1.02736587339765,-21.07)) ;
#111333=CARTESIAN_POINT('Origin',(1.15,1.02736587339765,-21.17)) ;
#111334=CARTESIAN_POINT('',(-0.900000000000002,0.931757800066531,-21.1993103448276)) ;
#111335=CARTESIAN_POINT('',(13.9153543900904,0.931757800066525,-21.1993103448276)) ;
#111336=CARTESIAN_POINT('',(-0.900000000000002,1.02736587339765,-21.07)) ;
#111337=CARTESIAN_POINT('Origin',(-0.900000000000002,1.02736587339765,-21.17)) ;
#111338=CARTESIAN_POINT('',(-1.,1.02736587339765,-21.07)) ;
#111339=CARTESIAN_POINT('Origin',(8.49172374697003,3.8,-20.32)) ;
#111340=CARTESIAN_POINT('',(8.49172374697003,1.47741935483871,-18.4211532060953)) ;
#111341=CARTESIAN_POINT('',(8.49172374697003,1.47741935483871,-22.2188467939047)) ;
#111342=CARTESIAN_POINT('Origin',(8.49172374697003,3.8,-20.32)) ;
#111343=CARTESIAN_POINT('',(8.50816364570057,1.47636598119991,-18.4202920109583)) ;
#111344=CARTESIAN_POINT('Origin',(8.49172374697003,1.4,-18.3578583129651)) ;
#111345=CARTESIAN_POINT('',(8.50816364570057,1.47636598119991,-22.2197079890417)) ;
#111346=CARTESIAN_POINT('Origin',(8.50816364570057,3.8,-20.32)) ;
#111347=CARTESIAN_POINT('Origin',(8.49172374697003,1.4,-22.2821416870349)) ;
#111348=CARTESIAN_POINT('Origin',(1.25,3.8,-20.32)) ;
#111349=CARTESIAN_POINT('',(1.25,2.3,-20.32)) ;
#111350=CARTESIAN_POINT('Origin',(13.9153543900904,3.8,-20.32)) ;
#111351=CARTESIAN_POINT('',(-0.900000000000002,1.47741935483872,-22.2188467939047)) ;
#111352=CARTESIAN_POINT('',(13.9153543900904,1.47741935483871,-22.2188467939047)) ;
#111353=CARTESIAN_POINT('Origin',(-0.900000000000001,3.8,-20.32)) ;
#111354=CARTESIAN_POINT('',(1.35,0.876327704607742,-20.9924137931035)) ;
#111355=CARTESIAN_POINT('Ctrl Pts',(1.35,0.876327704607742,-20.9924137931035)) ;
#111356=CARTESIAN_POINT('Ctrl Pts',(1.35,0.888571289407569,-21.0456492115953)) ;
#111357=CARTESIAN_POINT('Ctrl Pts',(1.32969623836296,0.902340613578954,
-21.0979295970213)) ;
#111358=CARTESIAN_POINT('Ctrl Pts',(1.25741074236298,0.924142973728496,
-21.1750150537158)) ;
#111359=CARTESIAN_POINT('Ctrl Pts',(1.20472523187106,0.93175780006653,-21.1993103448276)) ;
#111360=CARTESIAN_POINT('Ctrl Pts',(1.15,0.93175780006653,-21.1993103448276)) ;
#111361=CARTESIAN_POINT('',(1.35,0.876327704607742,-19.6475862068966)) ;
#111362=CARTESIAN_POINT('Origin',(1.35,3.8,-20.32)) ;
#111363=CARTESIAN_POINT('Ctrl Pts',(1.15,0.931757800066529,-19.4406896551724)) ;
#111364=CARTESIAN_POINT('Ctrl Pts',(1.20475877631964,0.931757800066529,
-19.4406896551724)) ;
#111365=CARTESIAN_POINT('Ctrl Pts',(1.2574100247738,0.924155896380523,-19.4649343608884)) ;
#111366=CARTESIAN_POINT('Ctrl Pts',(1.32987646938161,0.9022735155524,-19.5423125455279)) ;
#111367=CARTESIAN_POINT('Ctrl Pts',(1.35,0.888577265820266,-19.5943248028101)) ;
#111368=CARTESIAN_POINT('Ctrl Pts',(1.35,0.876327704607742,-19.6475862068966)) ;
#111369=CARTESIAN_POINT('',(-0.900000000000002,1.47741935483872,-18.4211532060953)) ;
#111370=CARTESIAN_POINT('Origin',(-0.900000000000001,3.8,-20.32)) ;
#111371=CARTESIAN_POINT('',(13.9153543900904,1.47741935483871,-18.4211532060953)) ;
#111372=CARTESIAN_POINT('Origin',(0.55,3.09772049281573E-17,-20.32)) ;
#111373=CARTESIAN_POINT('',(0.549999999999999,4.4,-19.87)) ;
#111374=CARTESIAN_POINT('',(0.549999999999999,4.4,-20.77)) ;
#111375=CARTESIAN_POINT('',(0.549999999999999,4.4,-20.32)) ;
#111376=CARTESIAN_POINT('',(0.55,4.04473197180486,-20.77)) ;
#111377=CARTESIAN_POINT('',(0.55,1.39397422176708E-16,-20.77)) ;
#111378=CARTESIAN_POINT('',(0.55,4.05997159067981,-20.72)) ;
#111379=CARTESIAN_POINT('Ctrl Pts',(0.549999999999999,4.04473197180486,
-20.77)) ;
#111380=CARTESIAN_POINT('Ctrl Pts',(0.549999999999999,4.04764757798806,
-20.7655648611277)) ;
#111381=CARTESIAN_POINT('Ctrl Pts',(0.549999999999999,4.05014503921306,
-20.7609481448659)) ;
#111382=CARTESIAN_POINT('Ctrl Pts',(0.549999999999999,4.0569489863933,-20.7456814456903)) ;
#111383=CARTESIAN_POINT('Ctrl Pts',(0.549999999999999,4.0599715906798,-20.7318214564414)) ;
#111384=CARTESIAN_POINT('Ctrl Pts',(0.549999999999999,4.0599715906798,-20.72)) ;
#111385=CARTESIAN_POINT('',(0.55,4.05997159067981,-19.92)) ;
#111386=CARTESIAN_POINT('',(0.55,4.05997159067981,-19.82)) ;
#111387=CARTESIAN_POINT('',(0.55,4.04473197181449,-19.8700000000146)) ;
#111388=CARTESIAN_POINT('Origin',(0.550034503802634,3.93869457791706,-19.9224160296946)) ;
#111389=CARTESIAN_POINT('',(0.55,6.35032701027224E-17,-19.87)) ;
#111390=CARTESIAN_POINT('Origin',(10.,7.8,-22.86)) ;
#111391=CARTESIAN_POINT('',(9.93162277660169,7.82279240779944,-22.86)) ;
#111392=CARTESIAN_POINT('',(8.51539501058484,8.29486832980505,-22.86)) ;
#111393=CARTESIAN_POINT('',(10.,7.8,-22.86)) ;
#111394=CARTESIAN_POINT('',(8.51540095511711,8.29487265903615,-21.0890607599342)) ;
#111395=CARTESIAN_POINT('',(8.51539501058484,8.29486832980505,-22.86)) ;
#111396=CARTESIAN_POINT('',(8.54856023413467,8.2839858620311,-21.0760080665656)) ;
#111397=CARTESIAN_POINT('Ctrl Pts',(8.51540095511711,8.29487265903615,-21.0890607599342)) ;
#111398=CARTESIAN_POINT('Ctrl Pts',(8.51716444659961,8.29428466923188,-21.0896424828188)) ;
#111399=CARTESIAN_POINT('Ctrl Pts',(8.5190195486817,8.29366521079574,-21.0899704508582)) ;
#111400=CARTESIAN_POINT('Ctrl Pts',(8.52087614409674,8.29304501946167,-21.0900725025784)) ;
#111401=CARTESIAN_POINT('Ctrl Pts',(8.52171779595222,8.29276386763783,-21.0901187657647)) ;
#111402=CARTESIAN_POINT('Ctrl Pts',(8.52256005861366,8.29248252453827,-21.090119087778)) ;
#111403=CARTESIAN_POINT('Ctrl Pts',(8.52339613191994,8.29220315552769,-21.0900794460141)) ;
#111404=CARTESIAN_POINT('Ctrl Pts',(8.52456316579569,8.29181319797645,-21.0900241120128)) ;
#111405=CARTESIAN_POINT('Ctrl Pts',(8.52573147766847,8.29142195356397,-21.0898930049957)) ;
#111406=CARTESIAN_POINT('Ctrl Pts',(8.52689074379087,8.29103442649366,-21.089691327086)) ;
#111407=CARTESIAN_POINT('Ctrl Pts',(8.52858695132689,8.2904674071317,-21.0893962373015)) ;
#111408=CARTESIAN_POINT('Ctrl Pts',(8.53026630212623,8.2899212363328,-21.0889439218143)) ;
#111409=CARTESIAN_POINT('Ctrl Pts',(8.53190117913114,8.28939883282068,-21.0883683729163)) ;
#111410=CARTESIAN_POINT('Ctrl Pts',(8.53241671440272,8.28923410028381,-21.0881868817358)) ;
#111411=CARTESIAN_POINT('Ctrl Pts',(8.53292790037785,8.28907155799427,-21.0879933975174)) ;
#111412=CARTESIAN_POINT('Ctrl Pts',(8.53343404910735,8.28891083250767,-21.0877898379553)) ;
#111413=CARTESIAN_POINT('Ctrl Pts',(8.53529681408171,8.28831931900685,-21.0870406834076)) ;
#111414=CARTESIAN_POINT('Ctrl Pts',(8.53711612169875,8.28774836357889,-21.0861310088335)) ;
#111415=CARTESIAN_POINT('Ctrl Pts',(8.53885192161983,8.28720494689875,-21.085061264748)) ;
#111416=CARTESIAN_POINT('Ctrl Pts',(8.54015925159109,8.28679566878772,-21.0842555794339)) ;
#111417=CARTESIAN_POINT('Ctrl Pts',(8.54141951580282,8.28640152775899,-21.0833597461918)) ;
#111418=CARTESIAN_POINT('Ctrl Pts',(8.54261761299017,8.2860217121528,-21.0823927107854)) ;
#111419=CARTESIAN_POINT('Ctrl Pts',(8.54427390694791,8.28549664098141,-21.0810558451977)) ;
#111420=CARTESIAN_POINT('Ctrl Pts',(8.54582756795261,8.28499592220789,-21.0795574336962)) ;
#111421=CARTESIAN_POINT('Ctrl Pts',(8.54719190273359,8.28456181678109,-21.0779139760522)) ;
#111422=CARTESIAN_POINT('Ctrl Pts',(8.54768505754697,8.28440490428151,-21.0773199290052)) ;
#111423=CARTESIAN_POINT('Ctrl Pts',(8.54815358395156,8.28425671205374,-21.0767074323075)) ;
#111424=CARTESIAN_POINT('Ctrl Pts',(8.54859369700691,8.28411936587097,-21.0760788545618)) ;
#111425=CARTESIAN_POINT('',(8.56837597005374,8.27720399148448,-21.0525054212669)) ;
#111426=CARTESIAN_POINT('Ctrl Pts',(8.5485198670553,8.28382649282421,-21.0760140527758)) ;
#111427=CARTESIAN_POINT('Ctrl Pts',(8.55267891820627,8.28243778061541,-21.0705631273053)) ;
#111428=CARTESIAN_POINT('Ctrl Pts',(8.5570174719567,8.2809693370826,-21.0652590577817)) ;
#111429=CARTESIAN_POINT('Ctrl Pts',(8.56150853123423,8.27945301063663,-21.0601132102137)) ;
#111430=CARTESIAN_POINT('Ctrl Pts',(8.56331520072572,8.27884302075234,-21.0580431315899)) ;
#111431=CARTESIAN_POINT('Ctrl Pts',(8.56514663435523,8.27822544298235,-21.0559980022296)) ;
#111432=CARTESIAN_POINT('Ctrl Pts',(8.56700126712394,8.27760232477898,-21.0539757856585)) ;
#111433=CARTESIAN_POINT('Ctrl Pts',(8.56745273479657,8.27745064099025,-21.0534835235653)) ;
#111434=CARTESIAN_POINT('Ctrl Pts',(8.56790562999349,8.27729861980367,-21.0529951953627)) ;
#111435=CARTESIAN_POINT('Ctrl Pts',(8.56835731300612,8.27714712982918,-21.0525055965825)) ;
#111436=CARTESIAN_POINT('',(9.93162277660169,7.82279240779944,-21.2797127088383)) ;
#111437=CARTESIAN_POINT('',(9.98593528106273,7.80468823964576,-21.2887647929151)) ;
#111438=CARTESIAN_POINT('',(9.93162277660169,7.82279240779944,-22.86)) ;
#111439=CARTESIAN_POINT('Origin',(10.,6.8,-22.86)) ;
#111440=CARTESIAN_POINT('',(10.,6.8847127088383,-22.86)) ;
#111441=CARTESIAN_POINT('',(10.,7.72792407799439,-22.86)) ;
#111442=CARTESIAN_POINT('',(10.,6.8,-22.86)) ;
#111443=CARTESIAN_POINT('',(10.,7.72792407799439,-21.2797127088383)) ;
#111444=CARTESIAN_POINT('',(10.,7.72792407799439,-22.86)) ;
#111445=CARTESIAN_POINT('',(10.,6.8847127088383,-21.2797127088383)) ;
#111446=CARTESIAN_POINT('',(10.,6.8,-21.2797127088383)) ;
#111447=CARTESIAN_POINT('',(10.,6.8847127088383,-22.86)) ;
#111448=CARTESIAN_POINT('Origin',(8.5,6.55,-22.86)) ;
#111449=CARTESIAN_POINT('',(9.91643989873054,6.78607331645509,-21.2797127088383)) ;
#111450=CARTESIAN_POINT('',(8.58355805979354,6.56393854759965,-21.0575665415707)) ;
#111451=CARTESIAN_POINT('',(8.48442535909739,6.54740422651623,-21.0410436188994)) ;
#111452=CARTESIAN_POINT('',(8.56107669735261,6.56009388000089,-21.0823838472224)) ;
#111453=CARTESIAN_POINT('Ctrl Pts',(8.58354728038625,6.56400494118525,-21.0575667486351)) ;
#111454=CARTESIAN_POINT('Ctrl Pts',(8.57838853885694,6.56313097816977,-21.0629365696477)) ;
#111455=CARTESIAN_POINT('Ctrl Pts',(8.5733012794655,6.56225500583438,-21.0683881686567)) ;
#111456=CARTESIAN_POINT('Ctrl Pts',(8.56834297134802,6.56140899842962,-21.0739607837897)) ;
#111457=CARTESIAN_POINT('Ctrl Pts',(8.5658758707987,6.56098805134777,-21.0767335444834)) ;
#111458=CARTESIAN_POINT('Ctrl Pts',(8.56344049907312,6.56057499921404,-21.0795353033204)) ;
#111459=CARTESIAN_POINT('Ctrl Pts',(8.56104288133098,6.56017406260212,-21.0823650362459)) ;
#111460=CARTESIAN_POINT('',(8.50816305748501,6.55136011924236,-21.0973726221052)) ;
#111461=CARTESIAN_POINT('Ctrl Pts',(8.56125813732196,6.56020968955366,-21.0825506353537)) ;
#111462=CARTESIAN_POINT('Ctrl Pts',(8.5573713991649,6.55956189986082,-21.0872085994735)) ;
#111463=CARTESIAN_POINT('Ctrl Pts',(8.55306335190238,6.55884389198373,-21.0899674660873)) ;
#111464=CARTESIAN_POINT('Ctrl Pts',(8.54121332232612,6.55686888705435,-21.0965237407842)) ;
#111465=CARTESIAN_POINT('Ctrl Pts',(8.53496267038448,6.55582711173075,-21.0979613606691)) ;
#111466=CARTESIAN_POINT('Ctrl Pts',(8.5288866518513,6.55481444197522,-21.0992795539314)) ;
#111467=CARTESIAN_POINT('Ctrl Pts',(8.52471102104674,6.55411850350779,-21.0995977494013)) ;
#111468=CARTESIAN_POINT('Ctrl Pts',(8.52011475164502,6.5533524586075,-21.0997029599352)) ;
#111469=CARTESIAN_POINT('Ctrl Pts',(8.51754797133869,6.55292466188978,-21.0997186459429)) ;
#111470=CARTESIAN_POINT('Ctrl Pts',(8.51248317870076,6.55208052978346,-21.0989638228622)) ;
#111471=CARTESIAN_POINT('Ctrl Pts',(8.51021540604917,6.55170256767486,-21.0983708961115)) ;
#111472=CARTESIAN_POINT('Ctrl Pts',(8.50816120922225,6.55136020153704,-21.097376411526)) ;
#111473=CARTESIAN_POINT('',(8.50816364570071,6.55136060761679,-22.86)) ;
#111474=CARTESIAN_POINT('',(8.50816364570071,6.55136060761679,-22.86)) ;
#111475=CARTESIAN_POINT('',(9.91643989873054,6.78607331645509,-22.86)) ;
#111476=CARTESIAN_POINT('',(8.5,6.55,-22.86)) ;
#111477=CARTESIAN_POINT('',(9.91643989873054,6.78607331645509,-22.86)) ;
#111478=CARTESIAN_POINT('Origin',(10.,1.5,-22.86)) ;
#111479=CARTESIAN_POINT('',(-0.900000000000002,1.5,-22.2821416870349)) ;
#111480=CARTESIAN_POINT('',(8.49172374697003,1.5,-22.2821416870349)) ;
#111481=CARTESIAN_POINT('',(10.,1.5,-22.2821416870349)) ;
#111482=CARTESIAN_POINT('',(8.49172374697003,1.5,-22.86)) ;
#111483=CARTESIAN_POINT('',(8.49172374697003,1.5,-22.86)) ;
#111484=CARTESIAN_POINT('',(-0.900000000000001,1.5,-22.86)) ;
#111485=CARTESIAN_POINT('',(10.,1.5,-22.86)) ;
#111486=CARTESIAN_POINT('',(-0.900000000000002,1.5,-22.2461360284258)) ;
#111487=CARTESIAN_POINT('Origin',(10.,1.5,-22.86)) ;
#111488=CARTESIAN_POINT('',(8.49172374697003,1.5,-17.78)) ;
#111489=CARTESIAN_POINT('',(-0.900000000000001,1.5,-17.78)) ;
#111490=CARTESIAN_POINT('',(10.,1.5,-17.78)) ;
#111491=CARTESIAN_POINT('',(8.49172374697003,1.5,-18.3578583129651)) ;
#111492=CARTESIAN_POINT('',(8.49172374697003,1.5,-22.86)) ;
#111493=CARTESIAN_POINT('',(-0.900000000000002,1.5,-18.3578583129651)) ;
#111494=CARTESIAN_POINT('',(10.,1.5,-18.3578583129651)) ;
#111495=CARTESIAN_POINT('',(-0.900000000000001,1.5,-22.86)) ;
#111496=CARTESIAN_POINT('Origin',(10.,0.,-22.86)) ;
#111497=CARTESIAN_POINT('',(10.,0.1,-17.78)) ;
#111498=CARTESIAN_POINT('',(10.,1.16528729116168,-17.78)) ;
#111499=CARTESIAN_POINT('',(10.,0.,-17.78)) ;
#111500=CARTESIAN_POINT('',(10.,0.1,-22.86)) ;
#111501=CARTESIAN_POINT('',(10.,0.1,-22.86)) ;
#111502=CARTESIAN_POINT('',(10.,1.16528729116168,-22.86)) ;
#111503=CARTESIAN_POINT('',(10.,0.,-22.86)) ;
#111504=CARTESIAN_POINT('',(10.,1.16528729116168,-22.3641618801782)) ;
#111505=CARTESIAN_POINT('',(10.,1.16528729116168,-22.86)) ;
#111506=CARTESIAN_POINT('',(10.,1.16528729116168,-18.2758381198218)) ;
#111507=CARTESIAN_POINT('Origin',(10.,3.8,-20.32)) ;
#111508=CARTESIAN_POINT('',(10.,1.16528729116168,-22.86)) ;
#111509=CARTESIAN_POINT('Origin',(0.,0.,-22.86)) ;
#111510=CARTESIAN_POINT('',(8.48377223398316,8.3,-22.86)) ;
#111511=CARTESIAN_POINT('',(7.1,8.3,-22.86)) ;
#111512=CARTESIAN_POINT('',(8.5,8.3,-22.86)) ;
#111513=CARTESIAN_POINT('Origin',(8.48377223398316,8.2,-22.86)) ;
#111514=CARTESIAN_POINT('Origin',(9.9,7.72792407799439,-22.86)) ;
#111515=CARTESIAN_POINT('Origin',(9.9,6.8847127088383,-22.86)) ;
#111516=CARTESIAN_POINT('',(8.49172374697018,6.55,-22.86)) ;
#111517=CARTESIAN_POINT('Origin',(8.49172374697018,6.65,-22.86)) ;
#111518=CARTESIAN_POINT('',(-0.900000000000001,6.55,-22.86)) ;
#111519=CARTESIAN_POINT('',(1.25,6.55,-22.86)) ;
#111520=CARTESIAN_POINT('',(-1.,6.45,-22.86)) ;
#111521=CARTESIAN_POINT('Origin',(-0.9,6.45,-22.86)) ;
#111522=CARTESIAN_POINT('',(-1.,4.65,-22.86)) ;
#111523=CARTESIAN_POINT('',(-1.,3.46944695195362E-16,-22.86)) ;
#111524=CARTESIAN_POINT('',(-0.900000000000001,4.55,-22.86)) ;
#111525=CARTESIAN_POINT('Origin',(-0.900000000000001,4.65,-22.86)) ;
#111526=CARTESIAN_POINT('',(1.15,4.55,-22.86)) ;
#111527=CARTESIAN_POINT('',(1.57859836313889E-15,4.55,-22.86)) ;
#111528=CARTESIAN_POINT('',(1.25,4.45,-22.86)) ;
#111529=CARTESIAN_POINT('Origin',(1.15,4.45,-22.86)) ;
#111530=CARTESIAN_POINT('',(1.25,3.15,-22.86)) ;
#111531=CARTESIAN_POINT('',(1.25,1.5,-22.86)) ;
#111532=CARTESIAN_POINT('',(1.15,3.05,-22.86)) ;
#111533=CARTESIAN_POINT('Origin',(1.15,3.15,-22.86)) ;
#111534=CARTESIAN_POINT('',(-0.900000000000002,3.05,-22.86)) ;
#111535=CARTESIAN_POINT('',(1.05818132034585E-15,3.05,-22.86)) ;
#111536=CARTESIAN_POINT('',(-1.,2.95,-22.86)) ;
#111537=CARTESIAN_POINT('Origin',(-0.900000000000002,2.95,-22.86)) ;
#111538=CARTESIAN_POINT('',(-1.,1.6,-22.86)) ;
#111539=CARTESIAN_POINT('',(-1.,3.46944695195362E-16,-22.86)) ;
#111540=CARTESIAN_POINT('Origin',(-0.900000000000002,1.6,-22.86)) ;
#111541=CARTESIAN_POINT('',(8.50816364570057,1.49863939238321,-22.86)) ;
#111542=CARTESIAN_POINT('Origin',(8.49172374697003,1.4,-22.86)) ;
#111543=CARTESIAN_POINT('',(9.91643989873054,1.26392668354489,-22.86)) ;
#111544=CARTESIAN_POINT('',(10.,1.24999999999998,-22.86)) ;
#111545=CARTESIAN_POINT('Origin',(9.9,1.16528729116168,-22.86)) ;
#111546=CARTESIAN_POINT('',(9.9,0.,-22.86)) ;
#111547=CARTESIAN_POINT('Origin',(9.9,0.1,-22.86)) ;
#111548=CARTESIAN_POINT('',(-2.,0.,-22.86)) ;
#111549=CARTESIAN_POINT('',(-2.,0.,-22.86)) ;
#111550=CARTESIAN_POINT('',(-2.,7.55,-22.86)) ;
#111551=CARTESIAN_POINT('',(-2.,7.65,-22.86)) ;
#111552=CARTESIAN_POINT('',(-1.9,7.65,-22.86)) ;
#111553=CARTESIAN_POINT('Origin',(-1.9,7.55,-22.86)) ;
#111554=CARTESIAN_POINT('',(6.9,7.65,-22.86)) ;
#111555=CARTESIAN_POINT('',(7.,7.65,-22.86)) ;
#111556=CARTESIAN_POINT('',(7.,7.75,-22.86)) ;
#111557=CARTESIAN_POINT('Origin',(6.9,7.75,-22.86)) ;
#111558=CARTESIAN_POINT('',(7.,8.2,-22.86)) ;
#111559=CARTESIAN_POINT('',(7.,8.3,-22.86)) ;
#111560=CARTESIAN_POINT('Origin',(7.1,8.2,-22.86)) ;
#111561=CARTESIAN_POINT('Origin',(0.,0.,-17.78)) ;
#111562=CARTESIAN_POINT('',(9.93162277660169,7.82279240779944,-17.78)) ;
#111563=CARTESIAN_POINT('',(8.51539501058484,8.29486832980505,-17.78)) ;
#111564=CARTESIAN_POINT('',(10.,7.8,-17.78)) ;
#111565=CARTESIAN_POINT('',(8.48377223398316,8.3,-17.78)) ;
#111566=CARTESIAN_POINT('Origin',(8.48377223398316,8.2,-17.78)) ;
#111567=CARTESIAN_POINT('',(7.1,8.3,-17.78)) ;
#111568=CARTESIAN_POINT('',(8.5,8.3,-17.78)) ;
#111569=CARTESIAN_POINT('',(7.,8.2,-17.78)) ;
#111570=CARTESIAN_POINT('Origin',(7.1,8.2,-17.78)) ;
#111571=CARTESIAN_POINT('',(7.,7.75,-17.78)) ;
#111572=CARTESIAN_POINT('',(7.,8.3,-17.78)) ;
#111573=CARTESIAN_POINT('',(6.9,7.65,-17.78)) ;
#111574=CARTESIAN_POINT('Origin',(6.9,7.75,-17.78)) ;
#111575=CARTESIAN_POINT('',(-1.9,7.65,-17.78)) ;
#111576=CARTESIAN_POINT('',(7.,7.65,-17.78)) ;
#111577=CARTESIAN_POINT('',(-2.,7.55,-17.78)) ;
#111578=CARTESIAN_POINT('Origin',(-1.9,7.55,-17.78)) ;
#111579=CARTESIAN_POINT('',(-2.,0.,-17.78)) ;
#111580=CARTESIAN_POINT('',(-2.,7.65,-17.78)) ;
#111581=CARTESIAN_POINT('',(9.9,0.,-17.78)) ;
#111582=CARTESIAN_POINT('',(-2.,0.,-17.78)) ;
#111583=CARTESIAN_POINT('Origin',(9.9,0.1,-17.78)) ;
#111584=CARTESIAN_POINT('',(9.91643989873054,1.26392668354489,-17.78)) ;
#111585=CARTESIAN_POINT('Origin',(9.9,1.16528729116168,-17.78)) ;
#111586=CARTESIAN_POINT('',(8.50816364570057,1.49863939238321,-17.78)) ;
#111587=CARTESIAN_POINT('',(0.472972972972955,2.83783783783779,-17.78)) ;
#111588=CARTESIAN_POINT('Origin',(8.49172374697003,1.4,-17.78)) ;
#111589=CARTESIAN_POINT('',(-1.,1.6,-17.78)) ;
#111590=CARTESIAN_POINT('Origin',(-0.900000000000002,1.6,-17.78)) ;
#111591=CARTESIAN_POINT('',(-1.,2.95,-17.78)) ;
#111592=CARTESIAN_POINT('',(-1.,3.46944695195362E-16,-17.78)) ;
#111593=CARTESIAN_POINT('',(-0.900000000000002,3.05,-17.78)) ;
#111594=CARTESIAN_POINT('Origin',(-0.900000000000002,2.95,-17.78)) ;
#111595=CARTESIAN_POINT('',(1.15,3.05,-17.78)) ;
#111596=CARTESIAN_POINT('',(1.05818132034585E-15,3.05,-17.78)) ;
#111597=CARTESIAN_POINT('',(1.25,3.15,-17.78)) ;
#111598=CARTESIAN_POINT('Origin',(1.15,3.15,-17.78)) ;
#111599=CARTESIAN_POINT('',(1.25,4.45,-17.78)) ;
#111600=CARTESIAN_POINT('',(1.25,5.3,-17.78)) ;
#111601=CARTESIAN_POINT('',(1.15,4.55,-17.78)) ;
#111602=CARTESIAN_POINT('Origin',(1.15,4.45,-17.78)) ;
#111603=CARTESIAN_POINT('',(-0.900000000000001,4.55,-17.78)) ;
#111604=CARTESIAN_POINT('',(1.57859836313889E-15,4.55,-17.78)) ;
#111605=CARTESIAN_POINT('',(-1.,4.65,-17.78)) ;
#111606=CARTESIAN_POINT('Origin',(-0.900000000000001,4.65,-17.78)) ;
#111607=CARTESIAN_POINT('',(-1.,6.45,-17.78)) ;
#111608=CARTESIAN_POINT('',(-1.,3.46944695195362E-16,-17.78)) ;
#111609=CARTESIAN_POINT('',(-0.900000000000001,6.55,-17.78)) ;
#111610=CARTESIAN_POINT('Origin',(-0.9,6.45,-17.78)) ;
#111611=CARTESIAN_POINT('',(8.49172374697018,6.55,-17.78)) ;
#111612=CARTESIAN_POINT('',(1.25,6.55,-17.78)) ;
#111613=CARTESIAN_POINT('',(8.50816364570071,6.55136060761679,-17.78)) ;
#111614=CARTESIAN_POINT('Origin',(8.49172374697018,6.65,-17.78)) ;
#111615=CARTESIAN_POINT('',(9.91643989873054,6.78607331645509,-17.78)) ;
#111616=CARTESIAN_POINT('',(8.5,6.55,-17.78)) ;
#111617=CARTESIAN_POINT('',(10.,6.8847127088383,-17.78)) ;
#111618=CARTESIAN_POINT('Origin',(9.9,6.8847127088383,-17.78)) ;
#111619=CARTESIAN_POINT('',(10.,7.72792407799439,-17.78)) ;
#111620=CARTESIAN_POINT('',(10.,6.8,-17.78)) ;
#111621=CARTESIAN_POINT('Origin',(9.9,7.72792407799439,-17.78)) ;
#111622=CARTESIAN_POINT('Origin',(7.,7.65,-22.86)) ;
#111623=CARTESIAN_POINT('',(-1.9,7.65,-22.86)) ;
#111624=CARTESIAN_POINT('',(6.9,7.65,-22.86)) ;
#111625=CARTESIAN_POINT('Origin',(7.,8.3,-22.86)) ;
#111626=CARTESIAN_POINT('',(7.,7.75,-17.78)) ;
#111627=CARTESIAN_POINT('',(7.,8.2,-22.86)) ;
#111628=CARTESIAN_POINT('Origin',(8.5,8.3,-22.86)) ;
#111629=CARTESIAN_POINT('',(8.4,8.3,-20.862072889851)) ;
#111630=CARTESIAN_POINT('',(8.48377267093844,8.29999999999968,-21.0780525450042)) ;
#111631=CARTESIAN_POINT('Ctrl Pts',(8.40000000000001,8.3,-20.862072889851)) ;
#111632=CARTESIAN_POINT('Ctrl Pts',(8.40000007660114,8.3,-20.8792296501961)) ;
#111633=CARTESIAN_POINT('Ctrl Pts',(8.40222537906653,8.3,-20.8961962391188)) ;
#111634=CARTESIAN_POINT('Ctrl Pts',(8.40642689896248,8.3,-20.9126162565066)) ;
#111635=CARTESIAN_POINT('Ctrl Pts',(8.4108423802459,8.3,-20.92987245932)) ;
#111636=CARTESIAN_POINT('Ctrl Pts',(8.41744096861416,8.3,-20.946526744374)) ;
#111637=CARTESIAN_POINT('Ctrl Pts',(8.42598957610854,8.3,-20.9621622007355)) ;
#111638=CARTESIAN_POINT('Ctrl Pts',(8.42927578126155,8.3,-20.9681726904321)) ;
#111639=CARTESIAN_POINT('Ctrl Pts',(8.43285067318742,8.3,-20.9740324469635)) ;
#111640=CARTESIAN_POINT('Ctrl Pts',(8.43670279785319,8.3,-20.9797167867854)) ;
#111641=CARTESIAN_POINT('Ctrl Pts',(8.43684245837179,8.3,-20.9799228750916)) ;
#111642=CARTESIAN_POINT('Ctrl Pts',(8.43698247939113,8.3,-20.9801287268225)) ;
#111643=CARTESIAN_POINT('Ctrl Pts',(8.43712286024715,8.3,-20.9803343406941)) ;
#111644=CARTESIAN_POINT('Ctrl Pts',(8.44304092798571,8.3,-20.9890024515356)) ;
#111645=CARTESIAN_POINT('Ctrl Pts',(8.44963232699549,8.300000000002,-20.9973317313645)) ;
#111646=CARTESIAN_POINT('Ctrl Pts',(8.45667836512367,8.29999999999776,-21.0051882739642)) ;
#111647=CARTESIAN_POINT('Ctrl Pts',(8.46347186896914,8.29999999999368,-21.0127632333091)) ;
#111648=CARTESIAN_POINT('Ctrl Pts',(8.47075094334181,8.29999999998296,-21.0199098655154)) ;
#111649=CARTESIAN_POINT('Ctrl Pts',(8.47818849074308,8.29999999991001,-21.0268816128285)) ;
#111650=CARTESIAN_POINT('Ctrl Pts',(8.47846436286148,8.2999999999073,-21.0271402075771)) ;
#111651=CARTESIAN_POINT('Ctrl Pts',(8.47874045306876,8.29999999990447,-21.0273985605991)) ;
#111652=CARTESIAN_POINT('Ctrl Pts',(8.47901674447045,8.29999999990152,-21.0276566852)) ;
#111653=CARTESIAN_POINT('Ctrl Pts',(8.48287938578321,8.29999999986032,-21.0312653488833)) ;
#111654=CARTESIAN_POINT('Ctrl Pts',(8.48681205529409,8.29999999978803,-21.0348079367278)) ;
#111655=CARTESIAN_POINT('Ctrl Pts',(8.49047938959116,8.29999999977836,-21.0386027060218)) ;
#111656=CARTESIAN_POINT('Ctrl Pts',(8.49231307405274,8.29999999977353,-21.0405001085834)) ;
#111657=CARTESIAN_POINT('Ctrl Pts',(8.49410676862313,8.29999999978935,-21.042469327125)) ;
#111658=CARTESIAN_POINT('Ctrl Pts',(8.49555027122445,8.29999999981726,-21.0446968070099)) ;
#111659=CARTESIAN_POINT('Ctrl Pts',(8.49675259850851,8.2999999998405,-21.0465521274215)) ;
#111660=CARTESIAN_POINT('Ctrl Pts',(8.49764594203226,8.29999999986456,-21.0486368157432)) ;
#111661=CARTESIAN_POINT('Ctrl Pts',(8.49795530287013,8.29999999987615,-21.0508110374494)) ;
#111662=CARTESIAN_POINT('Ctrl Pts',(8.49801735255452,8.29999999987847,-21.0512471293982)) ;
#111663=CARTESIAN_POINT('Ctrl Pts',(8.49805590844334,8.29999999988033,-21.051686822978)) ;
#111664=CARTESIAN_POINT('Ctrl Pts',(8.49806875158486,8.29999999988168,-21.0521289896614)) ;
#111665=CARTESIAN_POINT('Ctrl Pts',(8.49822249685463,8.2999999998978,-21.0574221678068)) ;
#111666=CARTESIAN_POINT('Ctrl Pts',(8.49538250015676,8.29999999989889,-21.0623553442684)) ;
#111667=CARTESIAN_POINT('Ctrl Pts',(8.49246863081133,8.29999999993393,-21.066722860551)) ;
#111668=CARTESIAN_POINT('Ctrl Pts',(8.48983292606215,8.29999999996562,-21.0706734437939)) ;
#111669=CARTESIAN_POINT('Ctrl Pts',(8.48683766317129,8.3,-21.0743922110698)) ;
#111670=CARTESIAN_POINT('Ctrl Pts',(8.48377316486175,8.3,-21.0780519562975)) ;
#111671=CARTESIAN_POINT('',(8.48377223398316,8.3,-22.86)) ;
#111672=CARTESIAN_POINT('',(7.1,8.3,-22.86)) ;
#111673=CARTESIAN_POINT('',(8.48377267093845,8.29999999999968,-19.5619474549958)) ;
#111674=CARTESIAN_POINT('',(8.48377223398316,8.3,-22.86)) ;
#111675=CARTESIAN_POINT('',(8.4,8.3,-19.777927110149)) ;
#111676=CARTESIAN_POINT('Ctrl Pts',(8.48377316486178,8.3,-19.5619480437025)) ;
#111677=CARTESIAN_POINT('Ctrl Pts',(8.48683766317132,8.3,-19.5656077889302)) ;
#111678=CARTESIAN_POINT('Ctrl Pts',(8.48983292606215,8.29999999996562,-19.5693265562061)) ;
#111679=CARTESIAN_POINT('Ctrl Pts',(8.49246863081132,8.29999999993393,-19.573277139449)) ;
#111680=CARTESIAN_POINT('Ctrl Pts',(8.49538250015675,8.29999999989889,-19.5776446557316)) ;
#111681=CARTESIAN_POINT('Ctrl Pts',(8.49822249685464,8.2999999998978,-19.5825778321932)) ;
#111682=CARTESIAN_POINT('Ctrl Pts',(8.49806875158487,8.29999999988168,-19.5878710103386)) ;
#111683=CARTESIAN_POINT('Ctrl Pts',(8.49805590844335,8.29999999988033,-19.588313177022)) ;
#111684=CARTESIAN_POINT('Ctrl Pts',(8.49801735255452,8.29999999987847,-19.5887528706018)) ;
#111685=CARTESIAN_POINT('Ctrl Pts',(8.49795530287013,8.29999999987615,-19.5891889625506)) ;
#111686=CARTESIAN_POINT('Ctrl Pts',(8.49764594190814,8.29999999986456,-19.5913631851291)) ;
#111687=CARTESIAN_POINT('Ctrl Pts',(8.49675259754384,8.2999999998405,-19.5934478740673)) ;
#111688=CARTESIAN_POINT('Ctrl Pts',(8.49555027122431,8.29999999981726,-19.59530319299)) ;
#111689=CARTESIAN_POINT('Ctrl Pts',(8.4941067657021,8.29999999978935,-19.5975306773816)) ;
#111690=CARTESIAN_POINT('Ctrl Pts',(8.49231306928119,8.29999999977353,-19.599499896352)) ;
#111691=CARTESIAN_POINT('Ctrl Pts',(8.49047938958767,8.29999999977837,-19.6013972939748)) ;
#111692=CARTESIAN_POINT('Ctrl Pts',(8.48681202348066,8.29999999978803,-19.6051920961739)) ;
#111693=CARTESIAN_POINT('Ctrl Pts',(8.48287934332709,8.29999999986032,-19.6087346907302)) ;
#111694=CARTESIAN_POINT('Ctrl Pts',(8.47901674443309,8.29999999990152,-19.6123433147599)) ;
#111695=CARTESIAN_POINT('Ctrl Pts',(8.47874052296043,8.29999999990447,-19.6126013740281)) ;
#111696=CARTESIAN_POINT('Ctrl Pts',(8.47846450284309,8.2999999999073,-19.6128596613565)) ;
#111697=CARTESIAN_POINT('Ctrl Pts',(8.47818870097127,8.29999999991001,-19.6131181900299)) ;
#111698=CARTESIAN_POINT('Ctrl Pts',(8.4707518532558,8.29999999998296,-19.620089275328)) ;
#111699=CARTESIAN_POINT('Ctrl Pts',(8.46347271757077,8.29999999998104,-19.627236821007)) ;
#111700=CARTESIAN_POINT('Ctrl Pts',(8.45667934899943,8.29999999998018,-19.6348126083154)) ;
#111701=CARTESIAN_POINT('Ctrl Pts',(8.44963335392747,8.29999999997929,-19.6426701181032)) ;
#111702=CARTESIAN_POINT('Ctrl Pts',(8.44304226791566,8.29999999996634,-19.651000256345)) ;
#111703=CARTESIAN_POINT('Ctrl Pts',(8.43712466127423,8.29999999997622,-19.659666888942)) ;
#111704=CARTESIAN_POINT('Ctrl Pts',(8.43698358608699,8.29999999997646,-19.6598735006502)) ;
#111705=CARTESIAN_POINT('Ctrl Pts',(8.43684287437576,8.2999999999767,-19.6600803512793)) ;
#111706=CARTESIAN_POINT('Ctrl Pts',(8.43670252680328,8.29999999997696,-19.6602874394955)) ;
#111707=CARTESIAN_POINT('Ctrl Pts',(8.42665365624043,8.29999999999548,-19.6751149327167)) ;
#111708=CARTESIAN_POINT('Ctrl Pts',(8.41848789916046,8.29999999999779,-19.6911348631973)) ;
#111709=CARTESIAN_POINT('Ctrl Pts',(8.41242260582095,8.29999999999911,-19.7079180514057)) ;
#111710=CARTESIAN_POINT('Ctrl Pts',(8.40662497273872,8.30000000000037,-19.7239606006668)) ;
#111711=CARTESIAN_POINT('Ctrl Pts',(8.40274598945664,8.3,-19.7407021939303)) ;
#111712=CARTESIAN_POINT('Ctrl Pts',(8.40101973895557,8.3,-19.757779788354)) ;
#111713=CARTESIAN_POINT('Ctrl Pts',(8.4003453349776,8.3,-19.7644515880762)) ;
#111714=CARTESIAN_POINT('Ctrl Pts',(8.40000003014814,8.3,-19.7711746730442)) ;
#111715=CARTESIAN_POINT('Ctrl Pts',(8.4,8.3,-19.777927110149)) ;
#111716=CARTESIAN_POINT('',(8.4,8.3,-20.9036545563009)) ;
#111717=CARTESIAN_POINT('Origin',(10.,7.8,-22.86)) ;
#111718=CARTESIAN_POINT('',(8.56837722373804,8.27720759208727,-19.5874948832496)) ;
#111719=CARTESIAN_POINT('',(8.54843785958922,8.2838540468036,-19.5639803122607)) ;
#111720=CARTESIAN_POINT('Ctrl Pts',(8.56837722339832,8.27720759220056,-19.5874948833623)) ;
#111721=CARTESIAN_POINT('Ctrl Pts',(8.56792584473107,8.27735805175631,-19.5870046902277)) ;
#111722=CARTESIAN_POINT('Ctrl Pts',(8.56747319573485,8.27750893475505,-19.5865157932638)) ;
#111723=CARTESIAN_POINT('Ctrl Pts',(8.56702308739659,8.2776589708678,-19.5860243039587)) ;
#111724=CARTESIAN_POINT('Ctrl Pts',(8.56055949575605,8.27981350141465,-19.5789664783343)) ;
#111725=CARTESIAN_POINT('Ctrl Pts',(8.55435459773969,8.28188180075344,-19.5716283954692)) ;
#111726=CARTESIAN_POINT('Ctrl Pts',(8.54852002808959,8.28382665730347,-19.5639858663514)) ;
#111727=CARTESIAN_POINT('',(8.51539953939803,8.29486682020066,-19.550940330123)) ;
#111728=CARTESIAN_POINT('Origin',(8.52916905055879,8.29027698314707,-19.5707344704815)) ;
#111729=CARTESIAN_POINT('',(8.51539501058484,8.29486832980505,-22.86)) ;
#111730=CARTESIAN_POINT('',(9.93162277660169,7.82279240779944,-19.3602872911617)) ;
#111731=CARTESIAN_POINT('',(9.93162277660169,7.82279240779944,-22.86)) ;
#111732=CARTESIAN_POINT('',(8.48593528106273,8.30468823964576,-19.6012352070849)) ;
#111733=CARTESIAN_POINT('Origin',(10.,6.8,-22.86)) ;
#111734=CARTESIAN_POINT('',(10.,6.8847127088383,-19.3602872911617)) ;
#111735=CARTESIAN_POINT('',(10.,7.72792407799439,-19.3602872911617)) ;
#111736=CARTESIAN_POINT('',(10.,7.8,-19.3602872911617)) ;
#111737=CARTESIAN_POINT('',(10.,7.72792407799439,-22.86)) ;
#111738=CARTESIAN_POINT('',(10.,6.8847127088383,-22.86)) ;
#111739=CARTESIAN_POINT('Origin',(8.5,6.55,-22.86)) ;
#111740=CARTESIAN_POINT('',(8.50816305748852,6.55136011924294,-19.5426273778919)) ;
#111741=CARTESIAN_POINT('Ctrl Pts',(8.50816120922619,6.5513602015377,-19.542623588472)) ;
#111742=CARTESIAN_POINT('Ctrl Pts',(8.50982330775214,6.55163721795869,-19.5418189278179)) ;
#111743=CARTESIAN_POINT('Ctrl Pts',(8.51162127657743,6.55193687942957,-19.541279028441)) ;
#111744=CARTESIAN_POINT('Ctrl Pts',(8.51523682141501,6.55253947023584,-19.5405710923351)) ;
#111745=CARTESIAN_POINT('Ctrl Pts',(8.51710259142463,6.5528504319041,-19.5403934679392)) ;
#111746=CARTESIAN_POINT('Ctrl Pts',(8.52217030373324,6.55369505062221,-19.5402356911266)) ;
#111747=CARTESIAN_POINT('Ctrl Pts',(8.52587381750002,6.55431230291667,-19.5404838833945)) ;
#111748=CARTESIAN_POINT('Ctrl Pts',(8.53482421528023,6.55580403588004,-19.5417298501843)) ;
#111749=CARTESIAN_POINT('Ctrl Pts',(8.53952102462709,6.55658683673489,-19.5432204474238)) ;
#111750=CARTESIAN_POINT('Ctrl Pts',(8.54640674065863,6.55773445607348,-19.5463682122463)) ;
#111751=CARTESIAN_POINT('Ctrl Pts',(8.55013419152287,6.55835569858715,-19.548236730231)) ;
#111752=CARTESIAN_POINT('Ctrl Pts',(8.55581906875195,6.55930317812533,-19.55204337543)) ;
#111753=CARTESIAN_POINT('Ctrl Pts',(8.5586115073215,6.55976858455358,-19.5542775555632)) ;
#111754=CARTESIAN_POINT('Ctrl Pts',(8.56125821409731,6.56020970234955,-19.5574494566561)) ;
#111755=CARTESIAN_POINT('',(9.91643989873054,6.78607331645509,-19.3602872911617)) ;
#111756=CARTESIAN_POINT('',(9.98442535909739,6.79740422651623,-19.3489563811006)) ;
#111757=CARTESIAN_POINT('',(9.91643989873054,6.78607331645509,-22.86)) ;
#111758=CARTESIAN_POINT('',(8.50816364570071,6.55136060761679,-22.86)) ;
#111759=CARTESIAN_POINT('Origin',(1.25,6.55,-22.86)) ;
#111760=CARTESIAN_POINT('',(8.49172372711481,6.55000000000007,-21.0894558427306)) ;
#111761=CARTESIAN_POINT('',(8.49172374697018,6.55,-22.86)) ;
#111762=CARTESIAN_POINT('',(8.4,6.55,-20.8606780018997)) ;
#111763=CARTESIAN_POINT('Ctrl Pts',(8.49172374697018,6.55000000000105,-21.0894557456557)) ;
#111764=CARTESIAN_POINT('Ctrl Pts',(8.4960680367363,6.55000000001052,-21.0859505863269)) ;
#111765=CARTESIAN_POINT('Ctrl Pts',(8.50046735944504,6.54999999990302,-21.0825119042492)) ;
#111766=CARTESIAN_POINT('Ctrl Pts',(8.5092028047519,6.55000000136502,-21.075516026702)) ;
#111767=CARTESIAN_POINT('Ctrl Pts',(8.51365366733359,6.55000000372466,-21.0720189182924)) ;
#111768=CARTESIAN_POINT('Ctrl Pts',(8.51786969589101,6.55000000840872,-21.0675740514918)) ;
#111769=CARTESIAN_POINT('Ctrl Pts',(8.51824835575336,6.5500000088438,-21.0671628343558)) ;
#111770=CARTESIAN_POINT('Ctrl Pts',(8.51893753951069,6.55000000964297,-21.0663894122641)) ;
#111771=CARTESIAN_POINT('Ctrl Pts',(8.51925555226624,6.55000001000021,-21.0660246830609)) ;
#111772=CARTESIAN_POINT('Ctrl Pts',(8.52125362518915,6.55000001218547,-21.0636369664008)) ;
#111773=CARTESIAN_POINT('Ctrl Pts',(8.52280131776514,6.55000000862054,-21.0613625215737)) ;
#111774=CARTESIAN_POINT('Ctrl Pts',(8.52354796988915,6.55000000490364,-21.0562172682012)) ;
#111775=CARTESIAN_POINT('Ctrl Pts',(8.52233587755859,6.5500000056078,-21.0535629178234)) ;
#111776=CARTESIAN_POINT('Ctrl Pts',(8.52032554216559,6.55000000470579,-21.0511610105705)) ;
#111777=CARTESIAN_POINT('Ctrl Pts',(8.52004618744962,6.55000000456892,-21.0508554672246)) ;
#111778=CARTESIAN_POINT('Ctrl Pts',(8.51943244221704,6.55000000425258,-21.0502375575506)) ;
#111779=CARTESIAN_POINT('Ctrl Pts',(8.51910103101854,6.55000000405877,-21.0499172773213)) ;
#111780=CARTESIAN_POINT('Ctrl Pts',(8.51460799223803,6.5500000014124,-21.0457349310042)) ;
#111781=CARTESIAN_POINT('Ctrl Pts',(8.50969722522557,6.55000000036127,-21.042960241153)) ;
#111782=CARTESIAN_POINT('Ctrl Pts',(8.50463600502756,6.55000000021577,-21.0396634748388)) ;
#111783=CARTESIAN_POINT('Ctrl Pts',(8.50427412871943,6.55000000020764,-21.0394272801265)) ;
#111784=CARTESIAN_POINT('Ctrl Pts',(8.49410349041849,6.55000000002642,-21.0327743312814)) ;
#111785=CARTESIAN_POINT('Ctrl Pts',(8.48448997361522,6.54999999999179,-21.0260809389623)) ;
#111786=CARTESIAN_POINT('Ctrl Pts',(8.46629237463078,6.55000000001684,-21.0109770243886)) ;
#111787=CARTESIAN_POINT('Ctrl Pts',(8.45766562693774,6.55000000000152,-21.0025939316619)) ;
#111788=CARTESIAN_POINT('Ctrl Pts',(8.44955830666692,6.55,-20.9932123342682)) ;
#111789=CARTESIAN_POINT('Ctrl Pts',(8.44937081015217,6.55,-20.9929944283117)) ;
#111790=CARTESIAN_POINT('Ctrl Pts',(8.43720071044388,6.5500000000026,-20.9787892740214)) ;
#111791=CARTESIAN_POINT('Ctrl Pts',(8.42721384365712,6.55000000009149,-20.963256668189)) ;
#111792=CARTESIAN_POINT('Ctrl Pts',(8.4118490364227,6.55000000007035,-20.9305950553166)) ;
#111793=CARTESIAN_POINT('Ctrl Pts',(8.40635547808238,6.5500000000232,-20.9135173325265)) ;
#111794=CARTESIAN_POINT('Ctrl Pts',(8.40108598764556,6.5499999999995,-20.8843588087523)) ;
#111795=CARTESIAN_POINT('Ctrl Pts',(8.4,6.55,-20.8725595279368)) ;
#111796=CARTESIAN_POINT('Ctrl Pts',(8.4,6.55,-20.8606780018997)) ;
#111797=CARTESIAN_POINT('',(8.4,6.55,-19.7793219981003)) ;
#111798=CARTESIAN_POINT('',(8.4,6.55,-19.5963606076168)) ;
#111799=CARTESIAN_POINT('',(8.4917237271148,6.5500000000004,-19.5505441572684)) ;
#111800=CARTESIAN_POINT('Ctrl Pts',(8.4,6.55000000000001,-19.7793219981003)) ;
#111801=CARTESIAN_POINT('Ctrl Pts',(8.4,6.55,-19.7614603515919)) ;
#111802=CARTESIAN_POINT('Ctrl Pts',(8.4024517784973,6.55000000000111,-19.7437850580849)) ;
#111803=CARTESIAN_POINT('Ctrl Pts',(8.40709634751727,6.55000000003439,-19.7267518487488)) ;
#111804=CARTESIAN_POINT('Ctrl Pts',(8.41193897064973,6.55000000006908,-19.708992307832)) ;
#111805=CARTESIAN_POINT('Ctrl Pts',(8.41916594308737,6.55000000013771,-19.6919288881297)) ;
#111806=CARTESIAN_POINT('Ctrl Pts',(8.42853896334544,6.55000000013582,-19.676081267302)) ;
#111807=CARTESIAN_POINT('Ctrl Pts',(8.43455058706601,6.55000000013461,-19.6659169946706)) ;
#111808=CARTESIAN_POINT('Ctrl Pts',(8.4414461105567,6.55000000009671,-19.6562530007178)) ;
#111809=CARTESIAN_POINT('Ctrl Pts',(8.44917210140209,6.55000000005186,-19.6472326831015)) ;
#111810=CARTESIAN_POINT('Ctrl Pts',(8.44936219523642,6.55000000005075,-19.6470107430557)) ;
#111811=CARTESIAN_POINT('Ctrl Pts',(8.44955278293318,6.55000000004968,-19.6467892022862)) ;
#111812=CARTESIAN_POINT('Ctrl Pts',(8.44974386351698,6.55000000004864,-19.6465680630167)) ;
#111813=CARTESIAN_POINT('Ctrl Pts',(8.45766118910687,6.55000000000559,-19.6374052712633)) ;
#111814=CARTESIAN_POINT('Ctrl Pts',(8.46628870646482,6.54999999999864,-19.6290215515032)) ;
#111815=CARTESIAN_POINT('Ctrl Pts',(8.47555348469889,6.55000000000007,-19.621335275949)) ;
#111816=CARTESIAN_POINT('Ctrl Pts',(8.48448851770308,6.55000000000144,-19.6139225647086)) ;
#111817=CARTESIAN_POINT('Ctrl Pts',(8.4941027369538,6.5500000000304,-19.6072346929705)) ;
#111818=CARTESIAN_POINT('Ctrl Pts',(8.50391213313786,6.55000000016212,-19.6008238957712)) ;
#111819=CARTESIAN_POINT('Ctrl Pts',(8.50409415224113,6.55000000016456,-19.6007049396667)) ;
#111820=CARTESIAN_POINT('Ctrl Pts',(8.50427622716239,6.55000000016576,-19.6005860597931)) ;
#111821=CARTESIAN_POINT('Ctrl Pts',(8.504458355799,6.55000000016576,-19.600467254632)) ;
#111822=CARTESIAN_POINT('Ctrl Pts',(8.50464048443561,6.55000000016577,-19.6003484494708)) ;
#111823=CARTESIAN_POINT('Ctrl Pts',(8.50482266678758,6.55000000016458,-19.6002297190221)) ;
#111824=CARTESIAN_POINT('Ctrl Pts',(8.50500490075226,6.55000000016234,-19.6001110617675)) ;
#111825=CARTESIAN_POINT('Ctrl Pts',(8.50970297364428,6.55000000010443,-19.5970520248173)) ;
#111826=CARTESIAN_POINT('Ctrl Pts',(8.51460443926445,6.55000000028677,-19.5942756540706)) ;
#111827=CARTESIAN_POINT('Ctrl Pts',(8.51874830926338,6.55000000038295,-19.5904369847284)) ;
#111828=CARTESIAN_POINT('Ctrl Pts',(8.51909542442965,6.550000000391,-19.5901154349821)) ;
#111829=CARTESIAN_POINT('Ctrl Pts',(8.51943721516341,6.55000000039357,-19.5897864145015)) ;
#111830=CARTESIAN_POINT('Ctrl Pts',(8.5197731018719,6.55000000039098,-19.5894491161473)) ;
#111831=CARTESIAN_POINT('Ctrl Pts',(8.52085916897642,6.5500000003826,-19.5883584845811)) ;
#111832=CARTESIAN_POINT('Ctrl Pts',(8.52182399801745,6.55000000033868,-19.5870446208819)) ;
#111833=CARTESIAN_POINT('Ctrl Pts',(8.52246334063467,6.55000000029842,-19.5856267666595)) ;
#111834=CARTESIAN_POINT('Ctrl Pts',(8.52278301194328,6.55000000027829,-19.5849178395483)) ;
#111835=CARTESIAN_POINT('Ctrl Pts',(8.52302131164593,6.55000000025926,-19.5841829148064)) ;
#111836=CARTESIAN_POINT('Ctrl Pts',(8.52315270869759,6.55000000024662,-19.5834368976348)) ;
#111837=CARTESIAN_POINT('Ctrl Pts',(8.52328410574924,6.55000000023398,-19.5826908804633)) ;
#111838=CARTESIAN_POINT('Ctrl Pts',(8.52330860014991,6.55000000022778,-19.5819337708622)) ;
#111839=CARTESIAN_POINT('Ctrl Pts',(8.52320066085453,6.55000000023233,-19.5811804740327)) ;
#111840=CARTESIAN_POINT('Ctrl Pts',(8.52284031330747,6.55000000024754,-19.5786656469369)) ;
#111841=CARTESIAN_POINT('Ctrl Pts',(8.52133564423349,6.55000000029586,-19.5764067380131)) ;
#111842=CARTESIAN_POINT('Ctrl Pts',(8.51965878991878,6.55000000031744,-19.5743986514954)) ;
#111843=CARTESIAN_POINT('Ctrl Pts',(8.51932554032811,6.55000000032172,-19.573999574483)) ;
#111844=CARTESIAN_POINT('Ctrl Pts',(8.51898545723477,6.55000000032522,-19.5736103757648)) ;
#111845=CARTESIAN_POINT('Ctrl Pts',(8.5186461503849,6.55000000032769,-19.5732310123193)) ;
#111846=CARTESIAN_POINT('Ctrl Pts',(8.51455081658658,6.55000000035749,-19.5686522072032)) ;
#111847=CARTESIAN_POINT('Ctrl Pts',(8.50963987409776,6.55000000028078,-19.5648202086186)) ;
#111848=CARTESIAN_POINT('Ctrl Pts',(8.50482177382259,6.55000000018959,-19.5609688701254)) ;
#111849=CARTESIAN_POINT('Ctrl Pts',(8.5004640292375,6.5500000001071,-19.5574855160012)) ;
#111850=CARTESIAN_POINT('Ctrl Pts',(8.49606692679174,6.55000000001227,-19.5540490105462)) ;
#111851=CARTESIAN_POINT('Ctrl Pts',(8.49172374697017,6.55000000000105,-19.5505442543438)) ;
#111852=CARTESIAN_POINT('',(8.49172374697018,6.55,-22.86)) ;
#111853=CARTESIAN_POINT('',(-0.9,6.55,-19.47)) ;
#111854=CARTESIAN_POINT('',(-0.900000000000001,6.55,-22.86)) ;
#111855=CARTESIAN_POINT('',(1.15,6.55,-19.47)) ;
#111856=CARTESIAN_POINT('',(1.25,6.55,-19.47)) ;
#111857=CARTESIAN_POINT('',(1.35,6.55,-19.67)) ;
#111858=CARTESIAN_POINT('Origin',(1.15,6.55,-19.67)) ;
#111859=CARTESIAN_POINT('',(1.35,6.55,-20.97)) ;
#111860=CARTESIAN_POINT('',(1.35,6.55,-21.07)) ;
#111861=CARTESIAN_POINT('',(1.15,6.55,-21.17)) ;
#111862=CARTESIAN_POINT('Origin',(1.15,6.55,-20.97)) ;
#111863=CARTESIAN_POINT('',(-0.9,6.55,-21.17)) ;
#111864=CARTESIAN_POINT('',(1.25,6.55,-21.17)) ;
#111865=CARTESIAN_POINT('',(-0.9,6.55,-22.86)) ;
#111866=CARTESIAN_POINT('Origin',(1.25,5.3,-22.86)) ;
#111867=CARTESIAN_POINT('',(1.25,3.15,-21.9631676725155)) ;
#111868=CARTESIAN_POINT('',(1.25,3.04189189189189,-21.7855279241354)) ;
#111869=CARTESIAN_POINT('Origin',(1.25,2.95,-21.9631676725155)) ;
#111870=CARTESIAN_POINT('',(1.25,3.15,-22.86)) ;
#111871=CARTESIAN_POINT('',(1.25,4.45,-21.9631676725155)) ;
#111872=CARTESIAN_POINT('',(1.25,4.45,-21.9011388300842)) ;
#111873=CARTESIAN_POINT('',(1.25,4.55810810810811,-21.7855279241354)) ;
#111874=CARTESIAN_POINT('Origin',(1.25,4.65,-21.9631676725155)) ;
#111875=CARTESIAN_POINT('',(1.25,5.26552792413544,-21.0781081081081)) ;
#111876=CARTESIAN_POINT('Origin',(1.25,3.8,-20.32)) ;
#111877=CARTESIAN_POINT('',(1.25,5.4431676725155,-20.97)) ;
#111878=CARTESIAN_POINT('Origin',(1.25,5.4431676725155,-21.17)) ;
#111879=CARTESIAN_POINT('',(1.25,6.45,-20.97)) ;
#111880=CARTESIAN_POINT('',(1.25,6.55,-20.97)) ;
#111881=CARTESIAN_POINT('',(1.25,6.45,-19.67)) ;
#111882=CARTESIAN_POINT('',(1.25,6.45,-19.57)) ;
#111883=CARTESIAN_POINT('',(1.25,5.4431676725155,-19.67)) ;
#111884=CARTESIAN_POINT('',(1.25,5.38113883008419,-19.67)) ;
#111885=CARTESIAN_POINT('',(1.25,5.26552792413544,-19.5618918918919)) ;
#111886=CARTESIAN_POINT('Origin',(1.25,5.4431676725155,-19.47)) ;
#111887=CARTESIAN_POINT('',(1.25,4.55810810810811,-18.8544720758646)) ;
#111888=CARTESIAN_POINT('Origin',(1.25,3.8,-20.32)) ;
#111889=CARTESIAN_POINT('',(1.25,4.45,-18.6768323274845)) ;
#111890=CARTESIAN_POINT('Origin',(1.25,4.65,-18.6768323274845)) ;
#111891=CARTESIAN_POINT('',(1.25,4.45,-17.78)) ;
#111892=CARTESIAN_POINT('',(1.25,3.15,-18.6768323274845)) ;
#111893=CARTESIAN_POINT('',(1.25,3.15,-18.7388611699158)) ;
#111894=CARTESIAN_POINT('',(1.25,3.04189189189189,-18.8544720758646)) ;
#111895=CARTESIAN_POINT('Origin',(1.25,2.95,-18.6768323274845)) ;
#111896=CARTESIAN_POINT('',(1.25,2.33447207586456,-19.5618918918919)) ;
#111897=CARTESIAN_POINT('Origin',(1.25,3.8,-20.32)) ;
#111898=CARTESIAN_POINT('',(1.25,2.1568323274845,-19.67)) ;
#111899=CARTESIAN_POINT('Origin',(1.25,2.1568323274845,-19.47)) ;
#111900=CARTESIAN_POINT('',(1.25,0.973783447787483,-19.67)) ;
#111901=CARTESIAN_POINT('',(1.25,0.895262490344437,-19.67)) ;
#111902=CARTESIAN_POINT('',(1.25,0.973783447787483,-20.97)) ;
#111903=CARTESIAN_POINT('Origin',(1.25,3.8,-20.32)) ;
#111904=CARTESIAN_POINT('',(1.25,2.1568323274845,-20.97)) ;
#111905=CARTESIAN_POINT('',(1.25,2.21886116991581,-20.97)) ;
#111906=CARTESIAN_POINT('',(1.25,2.33447207586456,-21.0781081081081)) ;
#111907=CARTESIAN_POINT('Origin',(1.25,2.1568323274845,-21.17)) ;
#111908=CARTESIAN_POINT('Origin',(1.25,3.8,-20.32)) ;
#111909=CARTESIAN_POINT('Origin',(-2.,0.,-22.86)) ;
#111910=CARTESIAN_POINT('',(0.899999999999999,0.,-21.92)) ;
#111911=CARTESIAN_POINT('',(1.1,0.,-21.72)) ;
#111912=CARTESIAN_POINT('Origin',(0.899999999999999,0.,-21.72)) ;
#111913=CARTESIAN_POINT('',(-2.,0.,-21.92)) ;
#111914=CARTESIAN_POINT('',(-2.,0.,-21.92)) ;
#111915=CARTESIAN_POINT('',(-2.,0.,-22.86)) ;
#111916=CARTESIAN_POINT('',(9.9,0.,-22.86)) ;
#111917=CARTESIAN_POINT('',(-2.,0.,-18.72)) ;
#111918=CARTESIAN_POINT('',(-2.,0.,-22.86)) ;
#111919=CARTESIAN_POINT('',(0.899999999999999,0.,-18.72)) ;
#111920=CARTESIAN_POINT('',(0.999999999999999,0.,-18.72)) ;
#111921=CARTESIAN_POINT('',(1.1,0.,-18.92)) ;
#111922=CARTESIAN_POINT('Origin',(0.899999999999999,0.,-18.92)) ;
#111923=CARTESIAN_POINT('',(1.1,0.,-21.82)) ;
#111924=CARTESIAN_POINT('Origin',(-2.,7.65,-22.86)) ;
#111925=CARTESIAN_POINT('',(-2.,6.9,-18.72)) ;
#111926=CARTESIAN_POINT('',(-2.,7.1,-18.92)) ;
#111927=CARTESIAN_POINT('Origin',(-2.,6.9,-18.92)) ;
#111928=CARTESIAN_POINT('',(-2.,-1.13380619344889E-17,-18.72)) ;
#111929=CARTESIAN_POINT('',(-2.,7.55,-22.86)) ;
#111930=CARTESIAN_POINT('',(-2.,6.9,-21.92)) ;
#111931=CARTESIAN_POINT('',(-2.,7.,-21.92)) ;
#111932=CARTESIAN_POINT('',(-2.,7.1,-21.72)) ;
#111933=CARTESIAN_POINT('Origin',(-2.,6.9,-21.72)) ;
#111934=CARTESIAN_POINT('',(-2.,7.1,-18.82)) ;
#111935=CARTESIAN_POINT('Origin',(-1.8,7.,-18.82)) ;
#111936=CARTESIAN_POINT('',(-1.7,0.1,-18.82)) ;
#111937=CARTESIAN_POINT('',(-1.9,0.1,-18.82)) ;
#111938=CARTESIAN_POINT('',(-2.,0.1,-18.82)) ;
#111939=CARTESIAN_POINT('',(-1.9,0.3,-18.82)) ;
#111940=CARTESIAN_POINT('',(-1.9,7.,-18.82)) ;
#111941=CARTESIAN_POINT('Origin',(-1.7,0.3,-18.82)) ;
#111942=CARTESIAN_POINT('Origin',(-1.8,7.,-21.82)) ;
#111943=CARTESIAN_POINT('',(-1.9,0.3,-21.82)) ;
#111944=CARTESIAN_POINT('',(-1.7,0.1,-21.82)) ;
#111945=CARTESIAN_POINT('Origin',(-1.7,0.3,-21.82)) ;
#111946=CARTESIAN_POINT('',(-1.9,0.1,-21.82)) ;
#111947=CARTESIAN_POINT('',(-1.9,1.23908819712629E-17,-21.82)) ;
#111948=CARTESIAN_POINT('',(0.999999999999999,0.1,-21.82)) ;
#111949=CARTESIAN_POINT('Origin',(-1.8,-2.2514151555628E-16,-20.32)) ;
#111950=CARTESIAN_POINT('',(-1.8,4.6,-20.97)) ;
#111951=CARTESIAN_POINT('',(-1.8,4.6,-19.67)) ;
#111952=CARTESIAN_POINT('',(-1.8,4.6,-19.77)) ;
#111953=CARTESIAN_POINT('',(-1.8,0.3,-19.67)) ;
#111954=CARTESIAN_POINT('',(-1.8,0.2,-19.67)) ;
#111955=CARTESIAN_POINT('',(-1.8,0.3,-18.92)) ;
#111956=CARTESIAN_POINT('',(-1.8,0.3,-18.82)) ;
#111957=CARTESIAN_POINT('',(-1.8,6.9,-18.92)) ;
#111958=CARTESIAN_POINT('',(-1.8,-5.16691679585995E-17,-18.92)) ;
#111959=CARTESIAN_POINT('',(-1.8,6.9,-21.72)) ;
#111960=CARTESIAN_POINT('',(-1.8,6.9,-20.32)) ;
#111961=CARTESIAN_POINT('',(-1.8,0.3,-21.72)) ;
#111962=CARTESIAN_POINT('',(-1.8,-3.98613863153961E-16,-21.72)) ;
#111963=CARTESIAN_POINT('',(-1.8,0.3,-20.97)) ;
#111964=CARTESIAN_POINT('',(-1.8,0.3,-20.87)) ;
#111965=CARTESIAN_POINT('',(-1.8,4.5,-20.97)) ;
#111966=CARTESIAN_POINT('Origin',(0.549999999999999,4.5,-19.77)) ;
#111967=CARTESIAN_POINT('',(-1.7,0.3,-19.77)) ;
#111968=CARTESIAN_POINT('',(-1.7,4.4,-19.77)) ;
#111969=CARTESIAN_POINT('',(-1.7,4.5,-19.77)) ;
#111970=CARTESIAN_POINT('',(0.45,4.4,-19.77)) ;
#111971=CARTESIAN_POINT('',(0.45,4.4,-19.77)) ;
#111972=CARTESIAN_POINT('',(0.45,0.3,-19.77)) ;
#111973=CARTESIAN_POINT('',(0.45,4.5,-19.77)) ;
#111974=CARTESIAN_POINT('',(0.549999999999999,0.3,-19.77)) ;
#111975=CARTESIAN_POINT('Origin',(0.549999999999999,4.5,-20.87)) ;
#111976=CARTESIAN_POINT('',(0.45,0.3,-20.87)) ;
#111977=CARTESIAN_POINT('',(0.45,4.4,-20.87)) ;
#111978=CARTESIAN_POINT('',(0.45,4.5,-20.87)) ;
#111979=CARTESIAN_POINT('',(-1.7,4.4,-20.87)) ;
#111980=CARTESIAN_POINT('',(-1.7,4.4,-20.87)) ;
#111981=CARTESIAN_POINT('',(-1.7,0.3,-20.87)) ;
#111982=CARTESIAN_POINT('',(-1.7,0.2,-20.87)) ;
#111983=CARTESIAN_POINT('',(0.549999999999999,0.3,-20.87)) ;
#111984=CARTESIAN_POINT('Origin',(0.549999999999999,4.5,-20.87)) ;
#111985=CARTESIAN_POINT('',(-1.7,4.5,-19.87)) ;
#111986=CARTESIAN_POINT('',(-1.7,4.5,-20.77)) ;
#111987=CARTESIAN_POINT('',(-1.7,4.5,-20.87)) ;
#111988=CARTESIAN_POINT('',(0.45,4.5,-20.77)) ;
#111989=CARTESIAN_POINT('',(0.45,4.5,-20.77)) ;
#111990=CARTESIAN_POINT('',(0.45,4.5,-19.87)) ;
#111991=CARTESIAN_POINT('',(0.45,4.5,-20.87)) ;
#111992=CARTESIAN_POINT('',(-1.7,4.5,-19.87)) ;
#111993=CARTESIAN_POINT('Origin',(0.55,3.09772049281573E-17,-20.32)) ;
#111994=CARTESIAN_POINT('',(0.55,2.61224989991992,-20.72)) ;
#111995=CARTESIAN_POINT('',(0.55,2.65280931275608,-20.77)) ;
#111996=CARTESIAN_POINT('Ctrl Pts',(0.55,2.61224989991992,-20.72)) ;
#111997=CARTESIAN_POINT('Ctrl Pts',(0.55,2.61224989991992,-20.723869744162)) ;
#111998=CARTESIAN_POINT('Ctrl Pts',(0.55,2.61317624258758,-20.7284201039157)) ;
#111999=CARTESIAN_POINT('Ctrl Pts',(0.55,2.61634258087509,-20.7366330008589)) ;
#112000=CARTESIAN_POINT('Ctrl Pts',(0.55,2.61951410407877,-20.7416304286453)) ;
#112001=CARTESIAN_POINT('Ctrl Pts',(0.55,2.63040394024853,-20.7549387190702)) ;
#112002=CARTESIAN_POINT('Ctrl Pts',(0.55,2.64148366881061,-20.7631705809674)) ;
#112003=CARTESIAN_POINT('Ctrl Pts',(0.55,2.65280931275608,-20.77)) ;
#112004=CARTESIAN_POINT('',(0.55,0.3,-20.77)) ;
#112005=CARTESIAN_POINT('',(0.55,1.39397422176708E-16,-20.77)) ;
#112006=CARTESIAN_POINT('',(0.55,0.3,-19.87)) ;
#112007=CARTESIAN_POINT('',(0.55,0.3,-19.77)) ;
#112008=CARTESIAN_POINT('',(0.55,2.65280931275594,-19.8700000000001)) ;
#112009=CARTESIAN_POINT('',(0.55,6.35032701027224E-17,-19.87)) ;
#112010=CARTESIAN_POINT('',(0.55,2.61224989991992,-19.92)) ;
#112011=CARTESIAN_POINT('Ctrl Pts',(0.55,2.65280931275593,-19.8700000000001)) ;
#112012=CARTESIAN_POINT('Ctrl Pts',(0.55,2.64148366881051,-19.8768294190327)) ;
#112013=CARTESIAN_POINT('Ctrl Pts',(0.55,2.63040394024849,-19.8850612809299)) ;
#112014=CARTESIAN_POINT('Ctrl Pts',(0.55,2.61951410407877,-19.8983695713547)) ;
#112015=CARTESIAN_POINT('Ctrl Pts',(0.55,2.61634258087509,-19.9033669991411)) ;
#112016=CARTESIAN_POINT('Ctrl Pts',(0.55,2.61317624258758,-19.9115798960843)) ;
#112017=CARTESIAN_POINT('Ctrl Pts',(0.55,2.61224989991992,-19.916130255838)) ;
#112018=CARTESIAN_POINT('Ctrl Pts',(0.55,2.61224989991992,-19.92)) ;
#112019=CARTESIAN_POINT('',(0.55,2.61224989991992,-19.82)) ;
#112020=CARTESIAN_POINT('Origin',(0.,0.2,-20.32)) ;
#112021=CARTESIAN_POINT('',(-1.7,0.2,-20.97)) ;
#112022=CARTESIAN_POINT('',(-1.7,0.2,-21.72)) ;
#112023=CARTESIAN_POINT('',(-1.7,0.2,-21.82)) ;
#112024=CARTESIAN_POINT('',(0.899999999999999,0.2,-21.72)) ;
#112025=CARTESIAN_POINT('',(0.999999999999999,0.2,-21.72)) ;
#112026=CARTESIAN_POINT('',(0.899999999999999,0.2,-18.92)) ;
#112027=CARTESIAN_POINT('',(0.899999999999999,0.2,-18.82)) ;
#112028=CARTESIAN_POINT('',(-1.7,0.2,-18.92)) ;
#112029=CARTESIAN_POINT('',(-1.8,0.2,-18.92)) ;
#112030=CARTESIAN_POINT('',(-1.7,0.2,-19.67)) ;
#112031=CARTESIAN_POINT('',(-1.7,0.2,-19.77)) ;
#112032=CARTESIAN_POINT('',(0.65,0.2,-19.67)) ;
#112033=CARTESIAN_POINT('',(-1.16429916652874E-32,0.2,-19.67)) ;
#112034=CARTESIAN_POINT('',(0.65,0.2,-20.97)) ;
#112035=CARTESIAN_POINT('',(0.65,0.2,-20.87)) ;
#112036=CARTESIAN_POINT('',(-1.35834902761687E-32,0.2,-20.97)) ;
#112037=CARTESIAN_POINT('Origin',(3.,2.3,-22.86)) ;
#112038=CARTESIAN_POINT('',(3.,4.2,-19.82)) ;
#112039=CARTESIAN_POINT('',(3.,3.4,-19.82)) ;
#112040=CARTESIAN_POINT('',(3.,2.3,-19.82)) ;
#112041=CARTESIAN_POINT('',(3.,4.3,-19.92)) ;
#112042=CARTESIAN_POINT('Origin',(3.,4.2,-19.92)) ;
#112043=CARTESIAN_POINT('',(3.,4.3,-20.72)) ;
#112044=CARTESIAN_POINT('',(3.,4.3,-22.86)) ;
#112045=CARTESIAN_POINT('',(3.,4.2,-20.82)) ;
#112046=CARTESIAN_POINT('Origin',(3.,4.2,-20.72)) ;
#112047=CARTESIAN_POINT('',(3.,3.4,-20.82)) ;
#112048=CARTESIAN_POINT('',(3.,2.3,-20.82)) ;
#112049=CARTESIAN_POINT('',(3.,3.3,-20.72)) ;
#112050=CARTESIAN_POINT('Origin',(3.,3.4,-20.72)) ;
#112051=CARTESIAN_POINT('',(3.,3.3,-19.92)) ;
#112052=CARTESIAN_POINT('',(3.,3.3,-22.86)) ;
#112053=CARTESIAN_POINT('Origin',(3.,3.4,-19.92)) ;
#112054=CARTESIAN_POINT('Origin',(-1.,3.8,-20.32)) ;
#112055=CARTESIAN_POINT('',(-1.,1.6,-22.2821416870349)) ;
#112056=CARTESIAN_POINT('',(-1.,1.55483870967742,-22.1555519007746)) ;
#112057=CARTESIAN_POINT('Origin',(-1.,1.40000000000001,-22.2821416870349)) ;
#112058=CARTESIAN_POINT('',(-1.,1.6,-22.86)) ;
#112059=CARTESIAN_POINT('',(-1.,2.95,-21.9631676725155)) ;
#112060=CARTESIAN_POINT('',(-1.,2.95,-20.32)) ;
#112061=CARTESIAN_POINT('',(-1.,2.1568323274845,-21.17)) ;
#112062=CARTESIAN_POINT('Origin',(-1.,3.8,-20.32)) ;
#112063=CARTESIAN_POINT('',(-1.,1.02736587339765,-21.17)) ;
#112064=CARTESIAN_POINT('',(-1.,3.8,-21.17)) ;
#112065=CARTESIAN_POINT('Origin',(-1.,3.8,-20.32)) ;
#112066=CARTESIAN_POINT('Origin',(-1.,3.05,-22.87)) ;
#112067=CARTESIAN_POINT('',(1.15,3.05,-21.9631676725155)) ;
#112068=CARTESIAN_POINT('',(1.15,3.05,-21.9011388300842)) ;
#112069=CARTESIAN_POINT('',(-0.900000000000002,3.05,-21.9631676725155)) ;
#112070=CARTESIAN_POINT('',(-1.,3.05,-21.9631676725155)) ;
#112071=CARTESIAN_POINT('',(-0.900000000000002,3.05,-22.87)) ;
#112072=CARTESIAN_POINT('Origin',(-1.,2.21886116991581,-21.07)) ;
#112073=CARTESIAN_POINT('',(-0.900000000000002,2.1568323274845,-21.07)) ;
#112074=CARTESIAN_POINT('',(1.15,2.1568323274845,-21.07)) ;
#112075=CARTESIAN_POINT('',(1.25,2.1568323274845,-21.07)) ;
#112076=CARTESIAN_POINT('',(1.15,0.895262490344437,-21.07)) ;
#112077=CARTESIAN_POINT('',(-0.900000000000002,2.21886116991581,-21.07)) ;
#112078=CARTESIAN_POINT('Origin',(-1.,3.8,-20.32)) ;
#112079=CARTESIAN_POINT('',(-0.900000000000002,2.24565220167453,-21.1240540540541)) ;
#112080=CARTESIAN_POINT('',(-0.900000000000001,2.99594594594595,-21.8743477983255)) ;
#112081=CARTESIAN_POINT('Origin',(-0.900000000000001,3.8,-20.32)) ;
#112082=CARTESIAN_POINT('',(1.15,2.99594594594595,-21.8743477983255)) ;
#112083=CARTESIAN_POINT('',(-1.,2.99594594594595,-21.8743477983255)) ;
#112084=CARTESIAN_POINT('',(1.15,2.24565220167453,-21.1240540540541)) ;
#112085=CARTESIAN_POINT('Origin',(1.15,3.8,-20.32)) ;
#112086=CARTESIAN_POINT('',(-1.,2.24565220167453,-21.1240540540541)) ;
#112087=CARTESIAN_POINT('Origin',(-1.,3.8,-20.32)) ;
#112088=CARTESIAN_POINT('',(-0.900000000000002,2.99594594594594,-18.7656522016745)) ;
#112089=CARTESIAN_POINT('',(-0.900000000000002,2.24565220167453,-19.515945945946)) ;
#112090=CARTESIAN_POINT('Origin',(-0.900000000000001,3.8,-20.32)) ;
#112091=CARTESIAN_POINT('',(1.15,2.24565220167453,-19.515945945946)) ;
#112092=CARTESIAN_POINT('',(-1.,2.24565220167453,-19.515945945946)) ;
#112093=CARTESIAN_POINT('',(1.15,2.99594594594594,-18.7656522016745)) ;
#112094=CARTESIAN_POINT('Origin',(1.15,3.8,-20.32)) ;
#112095=CARTESIAN_POINT('',(-1.,2.99594594594594,-18.7656522016745)) ;
#112096=CARTESIAN_POINT('Origin',(-1.,2.21886116991581,-19.57)) ;
#112097=CARTESIAN_POINT('',(1.15,2.1568323274845,-19.57)) ;
#112098=CARTESIAN_POINT('',(1.15,2.21886116991581,-19.57)) ;
#112099=CARTESIAN_POINT('',(-0.900000000000002,2.1568323274845,-19.57)) ;
#112100=CARTESIAN_POINT('',(-1.,2.1568323274845,-19.57)) ;
#112101=CARTESIAN_POINT('',(-0.900000000000002,0.895262490344437,-19.57)) ;
#112102=CARTESIAN_POINT('Origin',(-1.,3.05,-17.77)) ;
#112103=CARTESIAN_POINT('',(-0.900000000000002,3.05,-18.6768323274845)) ;
#112104=CARTESIAN_POINT('',(1.15,3.05,-18.6768323274845)) ;
#112105=CARTESIAN_POINT('',(1.25,3.05,-18.6768323274845)) ;
#112106=CARTESIAN_POINT('',(1.15,3.05,-17.78)) ;
#112107=CARTESIAN_POINT('',(-0.900000000000002,3.05,-18.7388611699158)) ;
#112108=CARTESIAN_POINT('Origin',(-1.,3.8,-20.32)) ;
#112109=CARTESIAN_POINT('',(-1.,2.1568323274845,-19.47)) ;
#112110=CARTESIAN_POINT('',(-1.,2.95,-18.6768323274845)) ;
#112111=CARTESIAN_POINT('Origin',(-1.,3.8,-20.32)) ;
#112112=CARTESIAN_POINT('',(-1.,2.95,-17.78)) ;
#112113=CARTESIAN_POINT('',(-1.,1.6,-18.3578583129651)) ;
#112114=CARTESIAN_POINT('',(-1.,1.6,-20.32)) ;
#112115=CARTESIAN_POINT('',(-1.,1.55483870967743,-18.4844480992254)) ;
#112116=CARTESIAN_POINT('Origin',(-1.,1.40000000000001,-18.3578583129651)) ;
#112117=CARTESIAN_POINT('',(-1.,1.02736587339765,-19.47)) ;
#112118=CARTESIAN_POINT('Origin',(-1.,3.8,-20.32)) ;
#112119=CARTESIAN_POINT('',(-1.,2.21886116991581,-19.47)) ;
#112120=CARTESIAN_POINT('Origin',(-1.,3.8,-20.32)) ;
#112121=CARTESIAN_POINT('',(-1.,5.4431676725155,-21.17)) ;
#112122=CARTESIAN_POINT('',(-1.,4.65,-21.9631676725155)) ;
#112123=CARTESIAN_POINT('Origin',(-1.,3.8,-20.32)) ;
#112124=CARTESIAN_POINT('',(-1.,4.65,-20.32)) ;
#112125=CARTESIAN_POINT('',(-1.,6.45,-21.17)) ;
#112126=CARTESIAN_POINT('',(-1.,6.45,-21.07)) ;
#112127=CARTESIAN_POINT('',(-1.,3.8,-21.17)) ;
#112128=CARTESIAN_POINT('Origin',(-1.,4.55,-21.9011388300842)) ;
#112129=CARTESIAN_POINT('',(-0.900000000000001,4.55,-21.9631676725155)) ;
#112130=CARTESIAN_POINT('',(1.15,4.55,-21.9631676725155)) ;
#112131=CARTESIAN_POINT('',(1.25,4.55,-21.9631676725155)) ;
#112132=CARTESIAN_POINT('',(1.15,4.55,-22.86)) ;
#112133=CARTESIAN_POINT('',(-0.900000000000001,4.55,-21.9011388300842)) ;
#112134=CARTESIAN_POINT('Origin',(-1.,3.8,-20.32)) ;
#112135=CARTESIAN_POINT('',(-0.900000000000001,4.60405405405406,-21.8743477983255)) ;
#112136=CARTESIAN_POINT('',(-0.900000000000001,5.35434779832547,-21.1240540540541)) ;
#112137=CARTESIAN_POINT('Origin',(-0.900000000000001,3.8,-20.32)) ;
#112138=CARTESIAN_POINT('',(1.15,5.35434779832547,-21.1240540540541)) ;
#112139=CARTESIAN_POINT('',(-1.,5.35434779832547,-21.1240540540541)) ;
#112140=CARTESIAN_POINT('',(1.15,4.60405405405405,-21.8743477983255)) ;
#112141=CARTESIAN_POINT('Origin',(1.15,3.8,-20.32)) ;
#112142=CARTESIAN_POINT('',(-1.,4.60405405405406,-21.8743477983255)) ;
#112143=CARTESIAN_POINT('Origin',(-1.,6.55,-21.07)) ;
#112144=CARTESIAN_POINT('',(-0.900000000000001,5.4431676725155,-21.07)) ;
#112145=CARTESIAN_POINT('',(-0.9,6.45,-21.07)) ;
#112146=CARTESIAN_POINT('',(-0.9,6.55,-21.07)) ;
#112147=CARTESIAN_POINT('',(1.15,6.45,-21.07)) ;
#112148=CARTESIAN_POINT('',(-1.,6.45,-21.07)) ;
#112149=CARTESIAN_POINT('',(1.15,5.4431676725155,-21.07)) ;
#112150=CARTESIAN_POINT('',(1.15,5.38113883008419,-21.07)) ;
#112151=CARTESIAN_POINT('',(-1.,5.4431676725155,-21.07)) ;
#112152=CARTESIAN_POINT('Origin',(-1.,3.8,-20.32)) ;
#112153=CARTESIAN_POINT('',(-0.900000000000001,5.35434779832547,-19.515945945946)) ;
#112154=CARTESIAN_POINT('',(-0.900000000000001,4.60405405405405,-18.7656522016745)) ;
#112155=CARTESIAN_POINT('Origin',(-0.900000000000001,3.8,-20.32)) ;
#112156=CARTESIAN_POINT('',(1.15,4.60405405405405,-18.7656522016745)) ;
#112157=CARTESIAN_POINT('',(-1.,4.60405405405405,-18.7656522016745)) ;
#112158=CARTESIAN_POINT('',(1.15,5.35434779832547,-19.515945945946)) ;
#112159=CARTESIAN_POINT('Origin',(1.15,3.8,-20.32)) ;
#112160=CARTESIAN_POINT('',(-1.,5.35434779832547,-19.515945945946)) ;
#112161=CARTESIAN_POINT('Origin',(-1.,4.55,-18.7388611699158)) ;
#112162=CARTESIAN_POINT('',(1.15,4.55,-18.6768323274845)) ;
#112163=CARTESIAN_POINT('',(1.15,4.55,-18.7388611699158)) ;
#112164=CARTESIAN_POINT('',(-0.900000000000001,4.55,-18.6768323274845)) ;
#112165=CARTESIAN_POINT('',(-1.,4.55,-18.6768323274845)) ;
#112166=CARTESIAN_POINT('',(-0.900000000000001,4.55,-17.78)) ;
#112167=CARTESIAN_POINT('Origin',(-1.,6.55,-19.57)) ;
#112168=CARTESIAN_POINT('',(1.15,5.4431676725155,-19.57)) ;
#112169=CARTESIAN_POINT('',(1.15,6.45,-19.57)) ;
#112170=CARTESIAN_POINT('',(1.15,6.55,-19.57)) ;
#112171=CARTESIAN_POINT('',(-0.9,6.45,-19.57)) ;
#112172=CARTESIAN_POINT('',(-1.,6.45,-19.57)) ;
#112173=CARTESIAN_POINT('',(-0.900000000000001,5.4431676725155,-19.57)) ;
#112174=CARTESIAN_POINT('',(-0.900000000000001,5.38113883008419,-19.57)) ;
#112175=CARTESIAN_POINT('',(1.25,5.4431676725155,-19.57)) ;
#112176=CARTESIAN_POINT('Origin',(-1.,3.8,-20.32)) ;
#112177=CARTESIAN_POINT('',(-1.,5.4431676725155,-19.47)) ;
#112178=CARTESIAN_POINT('',(-1.,6.45,-19.47)) ;
#112179=CARTESIAN_POINT('',(-1.,6.55,-19.47)) ;
#112180=CARTESIAN_POINT('',(-1.,6.45,-20.32)) ;
#112181=CARTESIAN_POINT('',(-1.,4.65,-18.6768323274845)) ;
#112182=CARTESIAN_POINT('',(-1.,4.65,-18.7388611699158)) ;
#112183=CARTESIAN_POINT('Origin',(-1.,3.8,-20.32)) ;
#112184=CARTESIAN_POINT('Origin',(10.,4.35421736843756,-21.195)) ;
#112185=CARTESIAN_POINT('',(9.91643989873054,7.72792407799439,-21.1810733164551)) ;
#112186=CARTESIAN_POINT('',(8.58356010126947,8.17221734381475,-20.9589266835449)) ;
#112187=CARTESIAN_POINT('',(8.47075240319158,8.20981990984071,-20.9401254005319)) ;
#112188=CARTESIAN_POINT('',(8.58356010126947,6.66256607592813,-20.9589266835449)) ;
#112189=CARTESIAN_POINT('',(8.58356010126947,6.64863939238321,-20.9589266835449)) ;
#112190=CARTESIAN_POINT('',(9.91643989873054,6.8847127088383,-21.1810733164551)) ;
#112191=CARTESIAN_POINT('',(9.98442535909739,6.89604361889945,-21.1924042265162)) ;
#112192=CARTESIAN_POINT('',(9.91643989873054,7.8,-21.1810733164551)) ;
#112193=CARTESIAN_POINT('Origin',(8.5,4.35421736843756,-20.945)) ;
#112194=CARTESIAN_POINT('',(8.5,8.17221734381475,-20.8602872911617)) ;
#112195=CARTESIAN_POINT('',(8.50000000129681,8.20000000266559,-20.862105625353)) ;
#112196=CARTESIAN_POINT('Origin',(8.5,8.1787077453077,-21.0490376414923)) ;
#112197=CARTESIAN_POINT('',(8.5,8.2,-19.7363454436991)) ;
#112198=CARTESIAN_POINT('',(8.5,6.66256607592813,-19.7797127088383)) ;
#112199=CARTESIAN_POINT('',(8.5,6.64863939238321,-19.7797127088383)) ;
#112200=CARTESIAN_POINT('',(8.50000000002143,6.64999999935441,-19.7793178443263)) ;
#112201=CARTESIAN_POINT('Origin',(8.5,6.65811550064505,-19.5831885106307)) ;
#112202=CARTESIAN_POINT('',(8.49999999999933,6.65000073218972,-20.8606896909637)) ;
#112203=CARTESIAN_POINT('',(8.5,6.65,-21.0436393923832)) ;
#112204=CARTESIAN_POINT('',(8.5,6.66256607592813,-20.8602872911617)) ;
#112205=CARTESIAN_POINT('Origin',(8.5,6.65133313842863,-21.0570100177546)) ;
#112206=CARTESIAN_POINT('',(8.5,8.20007071090457,-20.8602872911617)) ;
#112207=CARTESIAN_POINT('Origin',(8.5,4.35421736843756,-19.695)) ;
#112208=CARTESIAN_POINT('',(9.91643989873054,6.8847127088383,-19.4589266835449)) ;
#112209=CARTESIAN_POINT('',(8.58356010126947,6.66256607592813,-19.6810733164551)) ;
#112210=CARTESIAN_POINT('',(8.48442535909739,6.64604361889945,-19.6975957734838)) ;
#112211=CARTESIAN_POINT('',(8.58356010126947,8.20007071090456,-19.6810733164551)) ;
#112212=CARTESIAN_POINT('',(9.91643989873054,7.72792407799439,-19.4589266835449)) ;
#112213=CARTESIAN_POINT('',(9.97075240319158,7.70981990984071,-19.4498745994681)) ;
#112214=CARTESIAN_POINT('',(9.91643989873054,6.8,-19.4589266835449)) ;
#112215=CARTESIAN_POINT('Origin',(8.5,3.65,-19.82)) ;
#112216=CARTESIAN_POINT('',(8.45734623443633,3.62014236410543,-20.2220655561573)) ;
#112217=CARTESIAN_POINT('',(8.02582401135442,3.3180768079481,-19.92)) ;
#112218=CARTESIAN_POINT('',(8.34729988159781,3.54310991711847,-20.1450331091704)) ;
#112219=CARTESIAN_POINT('',(8.02582401135442,3.31807680794809,-20.72)) ;
#112220=CARTESIAN_POINT('',(8.02582401135442,3.3180768079481,-19.82)) ;
#112221=CARTESIAN_POINT('',(8.45734623443633,3.62014236410543,-20.4179344438427)) ;
#112222=CARTESIAN_POINT('',(8.70083523513316,3.79058466459322,-20.2474921433549)) ;
#112223=CARTESIAN_POINT('',(8.45734623443633,3.62014236410543,-19.82)) ;
#112224=CARTESIAN_POINT('Origin',(8.5,3.95,-19.82)) ;
#112225=CARTESIAN_POINT('',(8.5,3.89793444384266,-20.4179344438427)) ;
#112226=CARTESIAN_POINT('',(8.5,3.89793444384266,-20.2220655561573)) ;
#112227=CARTESIAN_POINT('',(8.5,3.89793444384266,-19.82)) ;
#112228=CARTESIAN_POINT('',(8.5,3.70206555615734,-20.2220655561573)) ;
#112229=CARTESIAN_POINT('',(8.5,3.95,-20.2220655561573)) ;
#112230=CARTESIAN_POINT('',(8.5,3.70206555615734,-20.4179344438427)) ;
#112231=CARTESIAN_POINT('',(8.5,3.70206555615734,-19.82)) ;
#112232=CARTESIAN_POINT('',(8.5,3.95,-20.4179344438427)) ;
#112233=CARTESIAN_POINT('Origin',(8.,4.3,-19.82)) ;
#112234=CARTESIAN_POINT('',(8.45734623443633,3.97985763589457,-20.4179344438427)) ;
#112235=CARTESIAN_POINT('',(8.02582401135442,4.2819231920519,-20.72)) ;
#112236=CARTESIAN_POINT('',(8.32457260887054,4.07279917379062,-20.5108759817387)) ;
#112237=CARTESIAN_POINT('',(8.02582401135442,4.2819231920519,-19.92)) ;
#112238=CARTESIAN_POINT('',(8.02582401135442,4.2819231920519,-19.82)) ;
#112239=CARTESIAN_POINT('',(8.45734623443633,3.97985763589457,-20.2220655561573)) ;
#112240=CARTESIAN_POINT('',(7.97103725533518,4.32027392126537,-19.8816492707865)) ;
#112241=CARTESIAN_POINT('',(8.45734623443633,3.97985763589457,-19.82)) ;
#112242=CARTESIAN_POINT('Origin',(1.5,2.3,-19.82)) ;
#112243=CARTESIAN_POINT('',(7.96847777691809,3.4,-19.82)) ;
#112244=CARTESIAN_POINT('',(8.,3.4,-19.82)) ;
#112245=CARTESIAN_POINT('',(7.96847777691809,4.2,-19.82)) ;
#112246=CARTESIAN_POINT('',(7.96847777691809,4.2,-19.82)) ;
#112247=CARTESIAN_POINT('',(3.,4.2,-19.82)) ;
#112248=CARTESIAN_POINT('Origin',(1.5,2.3,-20.82)) ;
#112249=CARTESIAN_POINT('',(7.96847777691809,4.2,-20.82)) ;
#112250=CARTESIAN_POINT('',(1.5,4.2,-20.82)) ;
#112251=CARTESIAN_POINT('',(7.96847777691809,3.4,-20.82)) ;
#112252=CARTESIAN_POINT('',(7.96847777691809,2.3,-20.82)) ;
#112253=CARTESIAN_POINT('',(1.5,3.4,-20.82)) ;
#112254=CARTESIAN_POINT('Origin',(8.,3.3,-19.82)) ;
#112255=CARTESIAN_POINT('',(7.96847777691809,3.3,-20.72)) ;
#112256=CARTESIAN_POINT('',(8.,3.3,-20.72)) ;
#112257=CARTESIAN_POINT('',(7.96847777691809,3.3,-19.92)) ;
#112258=CARTESIAN_POINT('',(7.96847777691809,3.3,-19.82)) ;
#112259=CARTESIAN_POINT('',(3.,3.3,-19.92)) ;
#112260=CARTESIAN_POINT('Origin',(1.5,4.3,-19.82)) ;
#112261=CARTESIAN_POINT('',(7.96847777691809,4.3,-19.92)) ;
#112262=CARTESIAN_POINT('',(8.,4.3,-19.92)) ;
#112263=CARTESIAN_POINT('',(7.96847777691809,4.3,-20.72)) ;
#112264=CARTESIAN_POINT('',(7.96847777691809,4.3,-19.82)) ;
#112265=CARTESIAN_POINT('',(1.5,4.3,-20.72)) ;
#112266=CARTESIAN_POINT('Origin',(1.5,2.3,-19.82)) ;
#112267=CARTESIAN_POINT('',(-0.4,2.3,-19.82)) ;
#112268=CARTESIAN_POINT('',(-0.4,-3.36847777691809,-19.82)) ;
#112269=CARTESIAN_POINT('',(-0.4,-3.4,-19.82)) ;
#112270=CARTESIAN_POINT('',(0.4,-3.36847777691809,-19.82)) ;
#112271=CARTESIAN_POINT('',(0.4,-3.36847777691809,-19.82)) ;
#112272=CARTESIAN_POINT('',(0.4,2.29999999999999,-19.82)) ;
#112273=CARTESIAN_POINT('',(0.4,2.29999999999999,-19.82)) ;
#112274=CARTESIAN_POINT('',(0.536602540378444,2.83090991212703,-19.82)) ;
#112275=CARTESIAN_POINT('Origin',(1.5,2.3,-19.82)) ;
#112276=CARTESIAN_POINT('',(0.536602540378444,3.93764017256378,-19.82)) ;
#112277=CARTESIAN_POINT('',(0.536602540378444,2.83090991212703,-19.82)) ;
#112278=CARTESIAN_POINT('Origin',(1.5,2.3,-19.82)) ;
#112279=CARTESIAN_POINT('Origin',(1.5,2.3,-20.82)) ;
#112280=CARTESIAN_POINT('',(0.4,2.29999999999999,-20.82)) ;
#112281=CARTESIAN_POINT('',(0.4,-3.36847777691809,-20.82)) ;
#112282=CARTESIAN_POINT('',(0.4,2.3,-20.82)) ;
#112283=CARTESIAN_POINT('',(-0.4,-3.36847777691809,-20.82)) ;
#112284=CARTESIAN_POINT('',(1.5,-3.36847777691809,-20.82)) ;
#112285=CARTESIAN_POINT('',(-0.4,2.3,-20.82)) ;
#112286=CARTESIAN_POINT('',(-0.4,2.3,-20.82)) ;
#112287=CARTESIAN_POINT('',(0.536602540378444,3.93764017256378,-20.82)) ;
#112288=CARTESIAN_POINT('Origin',(1.5,2.3,-20.82)) ;
#112289=CARTESIAN_POINT('',(0.536602540378444,2.83090991212703,-20.82)) ;
#112290=CARTESIAN_POINT('',(0.536602540378444,3.93764017256378,-20.82)) ;
#112291=CARTESIAN_POINT('Origin',(1.5,2.3,-20.82)) ;
#112292=CARTESIAN_POINT('Origin',(1.5,2.3,-19.82)) ;
#112293=CARTESIAN_POINT('',(-0.5,2.3,-19.92)) ;
#112294=CARTESIAN_POINT('',(-0.5,2.3,-20.72)) ;
#112295=CARTESIAN_POINT('',(-0.5,2.3,-19.82)) ;
#112296=CARTESIAN_POINT('Origin',(1.5,2.3,-19.92)) ;
#112297=CARTESIAN_POINT('Origin',(1.5,2.3,-20.72)) ;
#112298=CARTESIAN_POINT('Origin',(-0.5,-3.4,-19.82)) ;
#112299=CARTESIAN_POINT('',(-0.5,-3.36847777691809,-20.72)) ;
#112300=CARTESIAN_POINT('',(-0.5,-3.4,-20.72)) ;
#112301=CARTESIAN_POINT('',(-0.5,-3.36847777691809,-19.92)) ;
#112302=CARTESIAN_POINT('',(-0.5,-3.36847777691809,-19.82)) ;
#112303=CARTESIAN_POINT('',(-0.5,2.3,-19.92)) ;
#112304=CARTESIAN_POINT('Origin',(-0.15,-3.9,-19.82)) ;
#112305=CARTESIAN_POINT('',(-0.179857635894567,-3.85734623443633,-20.2220655561573)) ;
#112306=CARTESIAN_POINT('',(-0.481923192051905,-3.42582401135442,-19.92)) ;
#112307=CARTESIAN_POINT('',(-0.256890082881532,-3.74729988159781,-20.1450331091704)) ;
#112308=CARTESIAN_POINT('',(-0.481923192051905,-3.42582401135442,-20.72)) ;
#112309=CARTESIAN_POINT('',(-0.481923192051905,-3.42582401135442,-19.82)) ;
#112310=CARTESIAN_POINT('',(-0.179857635894567,-3.85734623443633,-20.4179344438427)) ;
#112311=CARTESIAN_POINT('',(-0.00941533540678435,-4.10083523513317,-20.2474921433549)) ;
#112312=CARTESIAN_POINT('',(-0.179857635894567,-3.85734623443633,-19.82)) ;
#112313=CARTESIAN_POINT('Origin',(0.15,-3.9,-19.82)) ;
#112314=CARTESIAN_POINT('',(0.0979344438426627,-3.9,-20.4179344438427)) ;
#112315=CARTESIAN_POINT('',(0.0979344438426627,-3.9,-20.2220655561573)) ;
#112316=CARTESIAN_POINT('',(0.0979344438426627,-3.9,-19.82)) ;
#112317=CARTESIAN_POINT('',(-0.0979344438426628,-3.9,-20.2220655561573)) ;
#112318=CARTESIAN_POINT('',(0.15,-3.9,-20.2220655561573)) ;
#112319=CARTESIAN_POINT('',(-0.0979344438426628,-3.9,-20.4179344438427)) ;
#112320=CARTESIAN_POINT('',(-0.0979344438426628,-3.9,-19.82)) ;
#112321=CARTESIAN_POINT('',(0.15,-3.9,-20.4179344438427)) ;
#112322=CARTESIAN_POINT('Origin',(0.5,-3.4,-19.82)) ;
#112323=CARTESIAN_POINT('',(0.179857635894567,-3.85734623443633,-20.4179344438427)) ;
#112324=CARTESIAN_POINT('',(0.481923192051904,-3.42582401135442,-20.72)) ;
#112325=CARTESIAN_POINT('',(0.272799173790623,-3.72457260887054,-20.5108759817387)) ;
#112326=CARTESIAN_POINT('',(0.481923192051904,-3.42582401135442,-19.92)) ;
#112327=CARTESIAN_POINT('',(0.481923192051904,-3.42582401135442,-19.82)) ;
#112328=CARTESIAN_POINT('',(0.179857635894567,-3.85734623443633,-20.2220655561573)) ;
#112329=CARTESIAN_POINT('',(0.520273921265371,-3.37103725533519,-19.8816492707865)) ;
#112330=CARTESIAN_POINT('',(0.179857635894567,-3.85734623443633,-19.82)) ;
#112331=CARTESIAN_POINT('Origin',(0.5,2.29999999999999,-19.82)) ;
#112332=CARTESIAN_POINT('',(0.500000000000001,2.29999999999999,-19.92)) ;
#112333=CARTESIAN_POINT('',(0.5,-3.36847777691809,-19.92)) ;
#112334=CARTESIAN_POINT('',(0.5,-3.4,-19.92)) ;
#112335=CARTESIAN_POINT('',(0.5,-3.36847777691809,-20.72)) ;
#112336=CARTESIAN_POINT('',(0.5,-3.36847777691809,-19.82)) ;
#112337=CARTESIAN_POINT('',(0.500000000000001,2.29999999999999,-20.72)) ;
#112338=CARTESIAN_POINT('',(0.5,2.29999999999999,-20.72)) ;
#112339=CARTESIAN_POINT('',(0.500000000000001,2.29999999999999,-19.82)) ;
#112340=CARTESIAN_POINT('Origin',(1.5,2.3,-19.82)) ;
#112341=CARTESIAN_POINT('Origin',(1.5,2.3,-19.92)) ;
#112342=CARTESIAN_POINT('Origin',(1.5,2.3,-20.72)) ;
#112343=CARTESIAN_POINT('Origin',(8.,2.68967221921331,-20.82)) ;
#112344=CARTESIAN_POINT('',(8.45734623443633,3.70206555615734,-20.4998576358946)) ;
#112345=CARTESIAN_POINT('',(8.02582401135442,3.4,-20.8019231920519)) ;
#112346=CARTESIAN_POINT('',(7.75526480758232,3.21060855735952,-20.9913146346924)) ;
#112347=CARTESIAN_POINT('',(8.02582401135442,4.2,-20.8019231920519)) ;
#112348=CARTESIAN_POINT('',(8.02582401135442,2.68967221921331,-20.8019231920519)) ;
#112349=CARTESIAN_POINT('',(8.45734623443633,3.89793444384266,-20.4998576358946)) ;
#112350=CARTESIAN_POINT('',(8.54034505662341,3.83983526831171,-20.4417584603636)) ;
#112351=CARTESIAN_POINT('',(8.45734623443633,2.68967221921331,-20.4998576358946)) ;
#112352=CARTESIAN_POINT('Origin',(8.,2.68967221921331,-19.82)) ;
#112353=CARTESIAN_POINT('',(8.45734623443633,3.89793444384266,-20.1401423641054)) ;
#112354=CARTESIAN_POINT('',(8.02582401135442,4.2,-19.8380768079481)) ;
#112355=CARTESIAN_POINT('',(8.54034505662341,3.83983526831171,-20.1982415396364)) ;
#112356=CARTESIAN_POINT('',(8.02582401135442,3.4,-19.8380768079481)) ;
#112357=CARTESIAN_POINT('',(8.02582401135442,3.4,-19.8380768079481)) ;
#112358=CARTESIAN_POINT('',(8.45734623443633,3.70206555615734,-20.1401423641054)) ;
#112359=CARTESIAN_POINT('',(7.75526480758232,3.21060855735952,-19.6486853653076)) ;
#112360=CARTESIAN_POINT('',(8.45734623443633,2.68967221921331,-20.1401423641054)) ;
#112361=CARTESIAN_POINT('Origin',(-1.11032778078669,-3.9,-20.17)) ;
#112362=CARTESIAN_POINT('',(0.0979344438426626,-3.85734623443633,-20.1401423641054)) ;
#112363=CARTESIAN_POINT('',(0.4,-3.42582401135442,-19.8380768079481)) ;
#112364=CARTESIAN_POINT('',(-0.223548570072128,-4.31660768288603,-20.4616253780202)) ;
#112365=CARTESIAN_POINT('',(-0.400000000000001,-3.42582401135442,-19.8380768079481)) ;
#112366=CARTESIAN_POINT('',(-0.400000000000001,-3.42582401135442,-19.8380768079481)) ;
#112367=CARTESIAN_POINT('',(-0.0979344438426627,-3.85734623443633,-20.1401423641054)) ;
#112368=CARTESIAN_POINT('',(-0.326007604256636,-3.53152743384494,-19.9120692036915)) ;
#112369=CARTESIAN_POINT('',(-1.11032778078669,-3.85734623443633,-20.1401423641054)) ;
#112370=CARTESIAN_POINT('Origin',(-1.11032778078669,-3.4,-20.82)) ;
#112371=CARTESIAN_POINT('',(-0.0979344438426627,-3.85734623443633,-20.4998576358946)) ;
#112372=CARTESIAN_POINT('',(-0.4,-3.42582401135442,-20.8019231920519)) ;
#112373=CARTESIAN_POINT('',(-0.589391442640475,-3.15526480758232,-20.9913146346924)) ;
#112374=CARTESIAN_POINT('',(0.400000000000001,-3.42582401135442,-20.8019231920519)) ;
#112375=CARTESIAN_POINT('',(-1.11032778078669,-3.42582401135442,-20.8019231920519)) ;
#112376=CARTESIAN_POINT('',(0.0979344438426626,-3.85734623443633,-20.4998576358946)) ;
#112377=CARTESIAN_POINT('',(0.0398352683117103,-3.94034505662341,-20.4417584603636)) ;
#112378=CARTESIAN_POINT('',(-1.11032778078669,-3.85734623443633,-20.4998576358946)) ;
#112379=CARTESIAN_POINT('Origin',(10.,1.24999999999998,-22.86)) ;
#112380=CARTESIAN_POINT('',(9.91643989873054,1.26392668354489,-18.2758381198218)) ;
#112381=CARTESIAN_POINT('',(9.91643989873054,1.26392668354489,-22.86)) ;
#112382=CARTESIAN_POINT('',(8.50816364570057,1.49863939238321,-18.3578583129651)) ;
#112383=CARTESIAN_POINT('Origin',(43.7052916441365,-4.36754860694379,-627.008201735632)) ;
#112384=CARTESIAN_POINT('',(8.50816364570057,1.49863939238321,-22.86)) ;
#112385=CARTESIAN_POINT('Origin',(8.49999999999985,3.8,-20.32)) ;
#112386=CARTESIAN_POINT('',(9.91643989873053,1.24322097942674,-18.3363035641941)) ;
#112387=CARTESIAN_POINT('',(9.91643989873053,1.24322097942648,-22.3036964358056)) ;
#112388=CARTESIAN_POINT('Origin',(9.91643989873053,3.8,-20.32)) ;
#112389=CARTESIAN_POINT('Origin',(36.5480653420491,-40.3802616895407,551.957655191746)) ;
#112390=CARTESIAN_POINT('Origin',(36.5480652367772,-40.3802620727359,-592.59765448914)) ;
#112391=CARTESIAN_POINT('Origin',(10.,1.24999999999998,-22.86)) ;
#112392=CARTESIAN_POINT('',(8.50816364570059,1.49863939238321,-22.2821416870347)) ;
#112393=CARTESIAN_POINT('',(8.50816364570057,1.49863939238321,-22.86)) ;
#112394=CARTESIAN_POINT('',(9.91643989873054,1.26392668354489,-22.3641618801782)) ;
#112395=CARTESIAN_POINT('Origin',(43.705291720328,-4.36754862033938,586.368203082216)) ;
#112396=CARTESIAN_POINT('',(9.91643989873054,1.26392668354489,-22.86)) ;
#112397=CARTESIAN_POINT('Origin',(-0.900000000000001,4.65,-20.32)) ;
#112398=CARTESIAN_POINT('Origin',(-0.900000000000001,4.65,-18.6768323274845)) ;
#112399=CARTESIAN_POINT('Origin',(-0.900000000000001,4.65,-18.6768323274845)) ;
#112400=CARTESIAN_POINT('Origin',(-0.900000000000001,4.65,-18.6768323274845)) ;
#112401=CARTESIAN_POINT('Origin',(-0.900000000000001,4.65,-18.6768323274845)) ;
#112402=CARTESIAN_POINT('Origin',(1.15,4.45,-18.7388611699158)) ;
#112403=CARTESIAN_POINT('Origin',(1.15,4.45,-18.6768323274845)) ;
#112404=CARTESIAN_POINT('Origin',(-1.,4.65,-18.6768323274845)) ;
#112405=CARTESIAN_POINT('Origin',(1.15,4.65,-18.6768323274845)) ;
#112406=CARTESIAN_POINT('Origin',(-0.900000000000001,3.8,-20.32)) ;
#112407=CARTESIAN_POINT('Origin',(-0.900000000000001,5.4431676725155,-19.47)) ;
#112408=CARTESIAN_POINT('Origin',(1.15,4.65,-18.6768323274845)) ;
#112409=CARTESIAN_POINT('Origin',(1.15,4.55810810810811,-18.8544720758646)) ;
#112410=CARTESIAN_POINT('Origin',(-0.900000000000001,5.4431676725155,-19.47)) ;
#112411=CARTESIAN_POINT('Origin',(-0.900000000000001,5.4431676725155,-19.47)) ;
#112412=CARTESIAN_POINT('Origin',(-0.900000000000001,5.4431676725155,-19.47)) ;
#112413=CARTESIAN_POINT('Origin',(-0.900000000000001,4.65,-20.32)) ;
#112414=CARTESIAN_POINT('Origin',(-0.900000000000001,4.65,-21.9631676725155)) ;
#112415=CARTESIAN_POINT('Origin',(-1.,4.65,-21.9631676725155)) ;
#112416=CARTESIAN_POINT('Origin',(1.15,4.65,-21.9631676725155)) ;
#112417=CARTESIAN_POINT('Origin',(-0.900000000000001,4.65,-21.9631676725155)) ;
#112418=CARTESIAN_POINT('Origin',(1.15,4.45,-21.9011388300842)) ;
#112419=CARTESIAN_POINT('Origin',(1.15,4.45,-21.9631676725155)) ;
#112420=CARTESIAN_POINT('Origin',(1.15,3.8,-20.32)) ;
#112421=CARTESIAN_POINT('Origin',(1.15,5.26552792413544,-19.5618918918919)) ;
#112422=CARTESIAN_POINT('Origin',(-1.,5.4431676725155,-19.47)) ;
#112423=CARTESIAN_POINT('Origin',(1.15,5.4431676725155,-19.47)) ;
#112424=CARTESIAN_POINT('Origin',(-0.900000000000001,3.8,-19.47)) ;
#112425=CARTESIAN_POINT('Origin',(-0.9,6.45,-19.47)) ;
#112426=CARTESIAN_POINT('Origin',(-0.9,6.45,-20.32)) ;
#112427=CARTESIAN_POINT('Origin',(-0.9,6.45,-19.47)) ;
#112428=CARTESIAN_POINT('Origin',(-0.900000000000001,4.65,-21.9631676725155)) ;
#112429=CARTESIAN_POINT('Origin',(-0.900000000000001,4.65,-21.9631676725155)) ;
#112430=CARTESIAN_POINT('Origin',(1.15,4.65,-21.9631676725155)) ;
#112431=CARTESIAN_POINT('Origin',(1.15,4.55810810810811,-21.7855279241354)) ;
#112432=CARTESIAN_POINT('Origin',(1.15,5.4431676725155,-19.47)) ;
#112433=CARTESIAN_POINT('Origin',(1.15,5.4431676725155,-19.67)) ;
#112434=CARTESIAN_POINT('Origin',(-0.9,6.45,-19.47)) ;
#112435=CARTESIAN_POINT('Origin',(-0.9,6.45,-19.47)) ;
#112436=CARTESIAN_POINT('Origin',(-0.900000000000001,3.8,-20.32)) ;
#112437=CARTESIAN_POINT('Origin',(-0.900000000000001,5.4431676725155,-21.17)) ;
#112438=CARTESIAN_POINT('Origin',(-1.,5.4431676725155,-21.17)) ;
#112439=CARTESIAN_POINT('Origin',(1.15,5.4431676725155,-21.17)) ;
#112440=CARTESIAN_POINT('Origin',(-0.900000000000001,5.4431676725155,-21.17)) ;
#112441=CARTESIAN_POINT('Origin',(1.15,3.8,-20.32)) ;
#112442=CARTESIAN_POINT('Origin',(1.15,5.26552792413544,-21.0781081081081)) ;
#112443=CARTESIAN_POINT('Origin',(1.15,6.55,-19.67)) ;
#112444=CARTESIAN_POINT('Origin',(1.15,6.45,-19.67)) ;
#112445=CARTESIAN_POINT('Origin',(1.25,6.45,-19.47)) ;
#112446=CARTESIAN_POINT('Origin',(1.15,6.45,-19.47)) ;
#112447=CARTESIAN_POINT('Origin',(-0.900000000000001,5.4431676725155,-21.17)) ;
#112448=CARTESIAN_POINT('Origin',(-0.900000000000001,5.4431676725155,-21.17)) ;
#112449=CARTESIAN_POINT('Origin',(1.15,5.4431676725155,-21.17)) ;
#112450=CARTESIAN_POINT('Origin',(1.15,5.4431676725155,-20.97)) ;
#112451=CARTESIAN_POINT('Origin',(1.15,6.45,-19.67)) ;
#112452=CARTESIAN_POINT('Origin',(1.35,6.45,-19.67)) ;
#112453=CARTESIAN_POINT('Origin',(-0.9,6.45,-20.32)) ;
#112454=CARTESIAN_POINT('Origin',(-0.9,6.45,-21.17)) ;
#112455=CARTESIAN_POINT('Origin',(-0.900000000000001,3.8,-21.17)) ;
#112456=CARTESIAN_POINT('Origin',(-0.9,6.45,-21.17)) ;
#112457=CARTESIAN_POINT('Origin',(1.15,6.55,-20.97)) ;
#112458=CARTESIAN_POINT('Origin',(1.15,6.45,-20.97)) ;
#112459=CARTESIAN_POINT('Origin',(1.35,6.45,-22.86)) ;
#112460=CARTESIAN_POINT('Origin',(1.35,6.45,-20.97)) ;
#112461=CARTESIAN_POINT('Origin',(-0.9,6.45,-21.17)) ;
#112462=CARTESIAN_POINT('Origin',(-0.9,6.45,-21.17)) ;
#112463=CARTESIAN_POINT('Origin',(1.15,6.45,-20.97)) ;
#112464=CARTESIAN_POINT('Origin',(1.15,6.45,-21.17)) ;
#112465=CARTESIAN_POINT('Origin',(-1.,6.45,-21.17)) ;
#112466=CARTESIAN_POINT('Origin',(-1.7,0.3,-20.97)) ;
#112467=CARTESIAN_POINT('Origin',(-1.7,0.3,-20.97)) ;
#112468=CARTESIAN_POINT('Origin',(-1.7,0.3,-20.97)) ;
#112469=CARTESIAN_POINT('Origin',(-1.7,0.3,-20.97)) ;
#112470=CARTESIAN_POINT('Origin',(0.549999999999999,0.3,-20.97)) ;
#112471=CARTESIAN_POINT('',(0.508578643762789,0.229289321881395,-20.8992893218813)) ;
#112472=CARTESIAN_POINT('Ctrl Pts',(0.65,0.200000000000001,-20.97)) ;
#112473=CARTESIAN_POINT('Ctrl Pts',(0.639834283464219,0.200000000000001,
-20.9649171417321)) ;
#112474=CARTESIAN_POINT('Ctrl Pts',(0.629316849080676,0.200389688120421,
-20.959657683858)) ;
#112475=CARTESIAN_POINT('Ctrl Pts',(0.606957334720003,0.202165884217635,
-20.9484679497194)) ;
#112476=CARTESIAN_POINT('Ctrl Pts',(0.595086727401555,0.203647820493405,
-20.9425227617951)) ;
#112477=CARTESIAN_POINT('Ctrl Pts',(0.572283837383469,0.207685608830753,
-20.9311067603974)) ;
#112478=CARTESIAN_POINT('Ctrl Pts',(0.561337481655848,0.210178193247152,
-20.9256298613106)) ;
#112479=CARTESIAN_POINT('Ctrl Pts',(0.549549942890579,0.213544620664103,
-20.9197406960418)) ;
#112480=CARTESIAN_POINT('Ctrl Pts',(0.548290718948528,0.213913346521202,
-20.9191116827674)) ;
#112481=CARTESIAN_POINT('Ctrl Pts',(0.536119229733184,0.217566912232432,
-20.9130327513519)) ;
#112482=CARTESIAN_POINT('Ctrl Pts',(0.52570691736286,0.221400308602526,
-20.9078422384292)) ;
#112483=CARTESIAN_POINT('Ctrl Pts',(0.513545110027472,0.226871185484663,
-20.9017711869643)) ;
#112484=CARTESIAN_POINT('Ctrl Pts',(0.511029334128475,0.228063976698571,
-20.9005146670641)) ;
#112485=CARTESIAN_POINT('Ctrl Pts',(0.508578643762789,0.229289321881392,
-20.8992893218813)) ;
#112486=CARTESIAN_POINT('Origin',(0.664280054302503,0.302990743361758,-20.9771421042501)) ;
#112487=CARTESIAN_POINT('Origin',(-1.7,4.5,-20.97)) ;
#112488=CARTESIAN_POINT('',(-1.77071067811866,4.45857864376269,-20.8992893218813)) ;
#112489=CARTESIAN_POINT('Origin',(-1.69703459697577,4.61417009504575,-20.977086685377)) ;
#112490=CARTESIAN_POINT('Ctrl Pts',(-1.77071067811863,4.45857864376269,
-20.8992893218813)) ;
#112491=CARTESIAN_POINT('Ctrl Pts',(-1.77521675558369,4.46759079869273,
-20.9037953993464)) ;
#112492=CARTESIAN_POINT('Ctrl Pts',(-1.77928079264421,4.47748625817284,
-20.9087264816716)) ;
#112493=CARTESIAN_POINT('Ctrl Pts',(-1.78624680748594,4.49811277056781,
-20.9190208825473)) ;
#112494=CARTESIAN_POINT('Ctrl Pts',(-1.78918030781741,4.50880509433286,
-20.9243639841482)) ;
#112495=CARTESIAN_POINT('Ctrl Pts',(-1.79185985500252,4.52101859321837,
-20.9304747545319)) ;
#112496=CARTESIAN_POINT('Ctrl Pts',(-1.79213045061208,4.522287517226,-20.9311097099085)) ;
#112497=CARTESIAN_POINT('Ctrl Pts',(-1.7947746790983,4.53504937002851,-20.937496289134)) ;
#112498=CARTESIAN_POINT('Ctrl Pts',(-1.79657370273652,4.54677936428193,
-20.9433715724062)) ;
#112499=CARTESIAN_POINT('Ctrl Pts',(-1.79896007643135,4.56920025888385,
-20.9545957747611)) ;
#112500=CARTESIAN_POINT('Ctrl Pts',(-1.79963010255188,4.57990192168147,
-20.959950075945)) ;
#112501=CARTESIAN_POINT('Ctrl Pts',(-1.79996164986962,4.59357116034293,
-20.966785573817)) ;
#112502=CARTESIAN_POINT('Ctrl Pts',(-1.8,4.59680282631913,-20.9684014131596)) ;
#112503=CARTESIAN_POINT('Ctrl Pts',(-1.8,4.6,-20.97)) ;
#112504=CARTESIAN_POINT('Origin',(-1.7,0.3,-20.32)) ;
#112505=CARTESIAN_POINT('Origin',(-1.7,0.3,-21.72)) ;
#112506=CARTESIAN_POINT('Origin',(0.65,0.3,-20.32)) ;
#112507=CARTESIAN_POINT('',(0.579289321881345,0.229289321881346,-20.8285786437627)) ;
#112508=CARTESIAN_POINT('Origin',(0.657086685361009,0.302965403016329,-20.9841700950131)) ;
#112509=CARTESIAN_POINT('Ctrl Pts',(0.579289321881345,0.229289321881345,
-20.8285786437627)) ;
#112510=CARTESIAN_POINT('Ctrl Pts',(0.583795399346365,0.224783244416326,
-20.8375907986927)) ;
#112511=CARTESIAN_POINT('Ctrl Pts',(0.588726481671636,0.220719207355781,
-20.8474862581728)) ;
#112512=CARTESIAN_POINT('Ctrl Pts',(0.599020882547777,0.213753192513749,
-20.8681127705687)) ;
#112513=CARTESIAN_POINT('Ctrl Pts',(0.604363984149085,0.210819692182088,
-20.8788050943346)) ;
#112514=CARTESIAN_POINT('Ctrl Pts',(0.610474754532814,0.208140144997089,
-20.8910185932202)) ;
#112515=CARTESIAN_POINT('Ctrl Pts',(0.611109709908936,0.207869549387731,
-20.8922875172269)) ;
#112516=CARTESIAN_POINT('Ctrl Pts',(0.617496289133951,0.205225320901704,
-20.9050493700285)) ;
#112517=CARTESIAN_POINT('Ctrl Pts',(0.623371572406202,0.203426297263468,
-20.916779364282)) ;
#112518=CARTESIAN_POINT('Ctrl Pts',(0.634595774761219,0.201039923568638,
-20.9392002588839)) ;
#112519=CARTESIAN_POINT('Ctrl Pts',(0.639950075945042,0.200369897448119,
-20.9499019216816)) ;
#112520=CARTESIAN_POINT('Ctrl Pts',(0.646785573817055,0.200038350130375,
-20.963571160343)) ;
#112521=CARTESIAN_POINT('Ctrl Pts',(0.648401413159587,0.2,-20.9668028263192)) ;
#112522=CARTESIAN_POINT('Ctrl Pts',(0.65,0.2,-20.97)) ;
#112523=CARTESIAN_POINT('',(0.579289321881345,0.229289321881345,-19.8114213562373)) ;
#112524=CARTESIAN_POINT('Ctrl Pts',(0.65,0.2,-19.67)) ;
#112525=CARTESIAN_POINT('Ctrl Pts',(0.64491714173209,0.2,-19.6801657165358)) ;
#112526=CARTESIAN_POINT('Ctrl Pts',(0.639657683858026,0.200389688120421,
-19.6906831509195)) ;
#112527=CARTESIAN_POINT('Ctrl Pts',(0.628467949719372,0.20216588421764,
-19.7130426652803)) ;
#112528=CARTESIAN_POINT('Ctrl Pts',(0.622522761794955,0.203647820493434,
-19.7249132725989)) ;
#112529=CARTESIAN_POINT('Ctrl Pts',(0.611106760396054,0.207685608831243,
-19.7477161626195)) ;
#112530=CARTESIAN_POINT('Ctrl Pts',(0.605629861308111,0.210178193248298,
-19.7586625183495)) ;
#112531=CARTESIAN_POINT('Ctrl Pts',(0.599740696039384,0.213544620665521,
-19.7704500571145)) ;
#112532=CARTESIAN_POINT('Ctrl Pts',(0.599111682766073,0.213913346521975,
-19.7717092810543)) ;
#112533=CARTESIAN_POINT('Ctrl Pts',(0.593032751351765,0.21756691223254,
-19.7838807702673)) ;
#112534=CARTESIAN_POINT('Ctrl Pts',(0.587842238429117,0.221400308602601,
-19.7942930826376)) ;
#112535=CARTESIAN_POINT('Ctrl Pts',(0.581771186964304,0.226871185484679,
-19.8064548899728)) ;
#112536=CARTESIAN_POINT('Ctrl Pts',(0.580514667064145,0.228063976698545,
-19.8089706658717)) ;
#112537=CARTESIAN_POINT('Ctrl Pts',(0.579289321881345,0.229289321881345,
-19.8114213562373)) ;
#112538=CARTESIAN_POINT('Origin',(0.657142104237265,0.302990743356481,-19.6557199457236)) ;
#112539=CARTESIAN_POINT('Origin',(-1.7,4.6,-20.87)) ;
#112540=CARTESIAN_POINT('',(-1.77071067811866,4.52928932188135,-20.8285786437627)) ;
#112541=CARTESIAN_POINT('Ctrl Pts',(-1.8,4.6,-20.97)) ;
#112542=CARTESIAN_POINT('Ctrl Pts',(-1.8,4.5949171417321,-20.9598342834642)) ;
#112543=CARTESIAN_POINT('Ctrl Pts',(-1.79961031187958,4.58965768385804,
-20.9493168490806)) ;
#112544=CARTESIAN_POINT('Ctrl Pts',(-1.79783411578236,4.57846794971939,
-20.9269573347197)) ;
#112545=CARTESIAN_POINT('Ctrl Pts',(-1.79635217950657,4.57252276179498,
-20.9150867274011)) ;
#112546=CARTESIAN_POINT('Ctrl Pts',(-1.79231439116883,4.56110676039624,
-20.8922838373809)) ;
#112547=CARTESIAN_POINT('Ctrl Pts',(-1.78982180675186,4.55562986130845,
-20.8813374816513)) ;
#112548=CARTESIAN_POINT('Ctrl Pts',(-1.78645537933467,4.54974069603971,
-20.8695499428861)) ;
#112549=CARTESIAN_POINT('Ctrl Pts',(-1.78608665347813,4.54911168276625,
-20.8682907189461)) ;
#112550=CARTESIAN_POINT('Ctrl Pts',(-1.78243308776747,4.54303275135178,
-20.8561192297327)) ;
#112551=CARTESIAN_POINT('Ctrl Pts',(-1.77859969139741,4.53784223842912,
-20.8457069173624)) ;
#112552=CARTESIAN_POINT('Ctrl Pts',(-1.77312881451532,4.53177118696431,
-20.8335451100272)) ;
#112553=CARTESIAN_POINT('Ctrl Pts',(-1.77193602330146,4.53051466706415,
-20.8310293341283)) ;
#112554=CARTESIAN_POINT('Ctrl Pts',(-1.77071067811866,4.52928932188135,
-20.8285786437627)) ;
#112555=CARTESIAN_POINT('Origin',(-1.69700925664257,4.60714210423891,-20.9842800542796)) ;
#112556=CARTESIAN_POINT('',(-1.77071067811866,4.52928932188135,-19.8114213562373)) ;
#112557=CARTESIAN_POINT('Origin',(-1.69703459698473,4.60708668535819,-19.6558299049927)) ;
#112558=CARTESIAN_POINT('Ctrl Pts',(-1.77071067811866,4.52928932188135,
-19.8114213562373)) ;
#112559=CARTESIAN_POINT('Ctrl Pts',(-1.77521675558368,4.53379539934637,
-19.8024092013073)) ;
#112560=CARTESIAN_POINT('Ctrl Pts',(-1.77928079264423,4.53872648167165,
-19.7925137418271)) ;
#112561=CARTESIAN_POINT('Ctrl Pts',(-1.78624680748614,4.54902088254762,
-19.7718872294317)) ;
#112562=CARTESIAN_POINT('Ctrl Pts',(-1.78918030781772,4.55436398414873,
-19.7611949056661)) ;
#112563=CARTESIAN_POINT('Ctrl Pts',(-1.79185985500276,4.56047475453246,
-19.7489814067805)) ;
#112564=CARTESIAN_POINT('Ctrl Pts',(-1.7921304506122,4.56110970990877,-19.7477124827734)) ;
#112565=CARTESIAN_POINT('Ctrl Pts',(-1.7947746790983,4.56749628913397,-19.7349506299714)) ;
#112566=CARTESIAN_POINT('Ctrl Pts',(-1.79657370273654,4.57337157240623,
-19.723220635718)) ;
#112567=CARTESIAN_POINT('Ctrl Pts',(-1.79896007643136,4.58459577476124,
-19.7007997411161)) ;
#112568=CARTESIAN_POINT('Ctrl Pts',(-1.79963010255188,4.58995007594506,
-19.6900980783184)) ;
#112569=CARTESIAN_POINT('Ctrl Pts',(-1.79996164986962,4.59678557381705,
-19.676428839657)) ;
#112570=CARTESIAN_POINT('Ctrl Pts',(-1.8,4.59840141315959,-19.6731971736808)) ;
#112571=CARTESIAN_POINT('Ctrl Pts',(-1.8,4.6,-19.67)) ;
#112572=CARTESIAN_POINT('Origin',(-1.7,0.3,-21.72)) ;
#112573=CARTESIAN_POINT('Origin',(-1.7,0.1,-21.72)) ;
#112574=CARTESIAN_POINT('Origin',(-1.9,0.3,-21.72)) ;
#112575=CARTESIAN_POINT('Origin',(1.9668402209837E-32,0.1,-21.72)) ;
#112576=CARTESIAN_POINT('',(0.899999999999999,0.1,-21.82)) ;
#112577=CARTESIAN_POINT('',(-1.8,0.1,-21.82)) ;
#112578=CARTESIAN_POINT('Origin',(0.899999999999999,0.1,-21.72)) ;
#112579=CARTESIAN_POINT('Origin',(0.899999999999999,0.1,-21.72)) ;
#112580=CARTESIAN_POINT('',(0.999999999999999,0.1,-21.72)) ;
#112581=CARTESIAN_POINT('Origin',(0.899999999999999,0.1,-21.72)) ;
#112582=CARTESIAN_POINT('Origin',(0.899999999999999,0.1,-21.72)) ;
#112583=CARTESIAN_POINT('Origin',(0.549999999999999,0.3,-19.67)) ;
#112584=CARTESIAN_POINT('',(0.508578643762786,0.229289321881393,-19.7407106781187)) ;
#112585=CARTESIAN_POINT('Origin',(0.664170095050064,0.302965403024492,-19.6629133146209)) ;
#112586=CARTESIAN_POINT('Ctrl Pts',(0.508578643762786,0.229289321881391,
-19.7407106781187)) ;
#112587=CARTESIAN_POINT('Ctrl Pts',(0.517590798692864,0.224783244416372,
-19.7362046006537)) ;
#112588=CARTESIAN_POINT('Ctrl Pts',(0.527486258173022,0.220719207355799,
-19.7312735183284)) ;
#112589=CARTESIAN_POINT('Ctrl Pts',(0.548112770567078,0.213753192514375,
-19.7209791174532)) ;
#112590=CARTESIAN_POINT('Ctrl Pts',(0.558805094331059,0.210819692183137,
-19.7156360158528)) ;
#112591=CARTESIAN_POINT('Ctrl Pts',(0.571018593216485,0.208140144997932,
-19.7095252454692)) ;
#112592=CARTESIAN_POINT('Ctrl Pts',(0.572287517225128,0.207869549388149,
-19.7088902900921)) ;
#112593=CARTESIAN_POINT('Ctrl Pts',(0.585049370028565,0.20522532090174,
-19.7025037108661)) ;
#112594=CARTESIAN_POINT('Ctrl Pts',(0.596779364281885,0.203426297263527,
-19.696628427594)) ;
#112595=CARTESIAN_POINT('Ctrl Pts',(0.619200258883654,0.201039923568666,
-19.685404225239)) ;
#112596=CARTESIAN_POINT('Ctrl Pts',(0.629901921681228,0.20036989744814,
-19.6800499240552)) ;
#112597=CARTESIAN_POINT('Ctrl Pts',(0.64357116034274,0.200038350130378,
-19.6732144261831)) ;
#112598=CARTESIAN_POINT('Ctrl Pts',(0.646802826319035,0.200000000000001,
-19.6715985868405)) ;
#112599=CARTESIAN_POINT('Ctrl Pts',(0.65,0.200000000000001,-19.67)) ;
#112600=CARTESIAN_POINT('Origin',(-1.7,0.3,-19.67)) ;
#112601=CARTESIAN_POINT('Origin',(-1.7,4.5,-19.67)) ;
#112602=CARTESIAN_POINT('',(-1.77071067811866,4.45857864376269,-19.7407106781187)) ;
#112603=CARTESIAN_POINT('Ctrl Pts',(-1.8,4.6,-19.67)) ;
#112604=CARTESIAN_POINT('Ctrl Pts',(-1.8,4.58983428346418,-19.6750828582679)) ;
#112605=CARTESIAN_POINT('Ctrl Pts',(-1.79961031187958,4.57931684908058,
-19.680342316142)) ;
#112606=CARTESIAN_POINT('Ctrl Pts',(-1.79783411578237,4.55695733471976,
-19.6915320502806)) ;
#112607=CARTESIAN_POINT('Ctrl Pts',(-1.79635217950657,4.54508672740122,
-19.697477238205)) ;
#112608=CARTESIAN_POINT('Ctrl Pts',(-1.79231439116924,4.52228383738322,
-19.7088932396026)) ;
#112609=CARTESIAN_POINT('Ctrl Pts',(-1.78982180675289,4.51133748165579,
-19.7143701386893)) ;
#112610=CARTESIAN_POINT('Ctrl Pts',(-1.78645537933594,4.49954994289049,
-19.7202593039581)) ;
#112611=CARTESIAN_POINT('Ctrl Pts',(-1.78608665347879,4.49829071894825,
-19.7208883172327)) ;
#112612=CARTESIAN_POINT('Ctrl Pts',(-1.7824330877675,4.48611922973279,-19.7269672486482)) ;
#112613=CARTESIAN_POINT('Ctrl Pts',(-1.77859969139746,4.47570691736254,
-19.7321577615708)) ;
#112614=CARTESIAN_POINT('Ctrl Pts',(-1.77312881451533,4.46354511002727,
-19.7382288130357)) ;
#112615=CARTESIAN_POINT('Ctrl Pts',(-1.77193602330149,4.46102933412832,
-19.7394853329358)) ;
#112616=CARTESIAN_POINT('Ctrl Pts',(-1.77071067811864,4.45857864376269,
-19.7407106781187)) ;
#112617=CARTESIAN_POINT('Origin',(-1.69700925663949,4.61428005429195,-19.6628578957552)) ;
#112618=CARTESIAN_POINT('Origin',(-1.7,0.3,-19.67)) ;
#112619=CARTESIAN_POINT('Origin',(-1.9,-4.11004745125224E-16,-21.72)) ;
#112620=CARTESIAN_POINT('',(-1.9,6.9,-21.82)) ;
#112621=CARTESIAN_POINT('Origin',(-1.9,6.9,-21.72)) ;
#112622=CARTESIAN_POINT('',(-1.9,7.,-21.82)) ;
#112623=CARTESIAN_POINT('Origin',(-2.,0.1,-21.92)) ;
#112624=CARTESIAN_POINT('Origin',(-1.89999999999986,0.100000000000145,-21.9200000000001)) ;
#112625=CARTESIAN_POINT('Origin',(0.899999999999999,0.1,-21.92)) ;
#112626=CARTESIAN_POINT('Origin',(0.899999999999999,0.1,-21.72)) ;
#112627=CARTESIAN_POINT('Origin',(1.1,0.1,-21.72)) ;
#112628=CARTESIAN_POINT('Origin',(0.899999999999999,0.1,-20.32)) ;
#112629=CARTESIAN_POINT('',(0.999999999999999,0.1,-18.92)) ;
#112630=CARTESIAN_POINT('',(0.999999999999999,0.1,-21.82)) ;
#112631=CARTESIAN_POINT('Origin',(0.899999999999999,0.1,-18.92)) ;
#112632=CARTESIAN_POINT('Origin',(-1.7,0.3,-19.67)) ;
#112633=CARTESIAN_POINT('Origin',(-1.7,0.3,-19.67)) ;
#112634=CARTESIAN_POINT('Origin',(-1.9,6.9,-21.72)) ;
#112635=CARTESIAN_POINT('',(-1.9,7.,-21.72)) ;
#112636=CARTESIAN_POINT('Origin',(-1.9,6.9,-21.72)) ;
#112637=CARTESIAN_POINT('Origin',(-1.9,6.9,-21.72)) ;
#112638=CARTESIAN_POINT('Origin',(-1.9,7.,-21.92)) ;
#112639=CARTESIAN_POINT('Origin',(-1.9,6.9,-21.92)) ;
#112640=CARTESIAN_POINT('Origin',(1.1,0.1,-18.82)) ;
#112641=CARTESIAN_POINT('Origin',(1.1,0.1,-18.92)) ;
#112642=CARTESIAN_POINT('Origin',(0.899999999999999,0.1,-18.92)) ;
#112643=CARTESIAN_POINT('',(0.899999999999999,0.1,-18.82)) ;
#112644=CARTESIAN_POINT('Origin',(0.899999999999999,0.1,-18.92)) ;
#112645=CARTESIAN_POINT('Origin',(0.899999999999999,0.1,-18.92)) ;
#112646=CARTESIAN_POINT('Origin',(-1.7,0.3,-20.32)) ;
#112647=CARTESIAN_POINT('Origin',(-1.7,0.3,-18.92)) ;
#112648=CARTESIAN_POINT('Origin',(-1.9,6.9,-20.32)) ;
#112649=CARTESIAN_POINT('',(-1.9,7.,-18.92)) ;
#112650=CARTESIAN_POINT('Origin',(-1.9,6.9,-18.92)) ;
#112651=CARTESIAN_POINT('',(-1.9,7.,-21.82)) ;
#112652=CARTESIAN_POINT('Origin',(-1.9,6.9,-21.72)) ;
#112653=CARTESIAN_POINT('Origin',(-1.9,7.1,-21.72)) ;
#112654=CARTESIAN_POINT('Origin',(0.899999999999999,0.1,-18.92)) ;
#112655=CARTESIAN_POINT('Origin',(0.899999999999999,0.1,-18.72)) ;
#112656=CARTESIAN_POINT('Origin',(-1.9668402209837E-32,0.1,-18.92)) ;
#112657=CARTESIAN_POINT('',(0.999999999999999,0.1,-18.82)) ;
#112658=CARTESIAN_POINT('Origin',(-1.7,0.1,-18.92)) ;
#112659=CARTESIAN_POINT('Origin',(-1.7,0.3,-18.92)) ;
#112660=CARTESIAN_POINT('Origin',(-1.9,0.3,-18.92)) ;
#112661=CARTESIAN_POINT('Origin',(-1.9,6.9,-18.92)) ;
#112662=CARTESIAN_POINT('',(-1.9,6.9,-18.82)) ;
#112663=CARTESIAN_POINT('Origin',(-1.9,6.9,-18.92)) ;
#112664=CARTESIAN_POINT('Origin',(-1.9,6.9,-18.92)) ;
#112665=CARTESIAN_POINT('Origin',(-1.9,7.1,-21.82)) ;
#112666=CARTESIAN_POINT('Origin',(-1.9,7.1,-18.92)) ;
#112667=CARTESIAN_POINT('Origin',(-1.8,0.1,-18.72)) ;
#112668=CARTESIAN_POINT('Origin',(-1.90000000000013,0.0999999999998694,
-18.7200000000001)) ;
#112669=CARTESIAN_POINT('Origin',(-1.9,-6.40600499298624E-17,-18.92)) ;
#112670=CARTESIAN_POINT('',(-1.9,7.,-18.82)) ;
#112671=CARTESIAN_POINT('Origin',(-1.9,6.9,-18.92)) ;
#112672=CARTESIAN_POINT('Origin',(-1.9,6.9,-18.72)) ;
#112673=CARTESIAN_POINT('Origin',(-1.9,7.,-18.72)) ;
#112674=CARTESIAN_POINT('Origin',(-0.900000000000002,2.95,-20.32)) ;
#112675=CARTESIAN_POINT('Origin',(-0.900000000000001,2.95,-21.9631676725155)) ;
#112676=CARTESIAN_POINT('Origin',(-0.900000000000002,2.95,-21.9631676725155)) ;
#112677=CARTESIAN_POINT('Origin',(-0.900000000000001,2.95,-21.9631676725155)) ;
#112678=CARTESIAN_POINT('Origin',(-0.900000000000002,2.95,-21.9631676725155)) ;
#112679=CARTESIAN_POINT('Origin',(1.15,3.15,-22.87)) ;
#112680=CARTESIAN_POINT('Origin',(1.15,3.15,-21.9631676725155)) ;
#112681=CARTESIAN_POINT('Origin',(-1.,2.95,-21.9631676725155)) ;
#112682=CARTESIAN_POINT('Origin',(1.15,2.95,-21.9631676725155)) ;
#112683=CARTESIAN_POINT('Origin',(-0.900000000000001,3.8,-20.32)) ;
#112684=CARTESIAN_POINT('Origin',(-0.900000000000002,2.1568323274845,-21.17)) ;
#112685=CARTESIAN_POINT('Origin',(-0.900000000000002,1.6,-20.32)) ;
#112686=CARTESIAN_POINT('Origin',(-0.900000000000002,1.6,-22.2821416870349)) ;
#112687=CARTESIAN_POINT('Origin',(13.9153543900904,1.4,-22.2821416870349)) ;
#112688=CARTESIAN_POINT('Origin',(8.49172374697002,1.4,-22.2821416870349)) ;
#112689=CARTESIAN_POINT('Origin',(-0.900000000000001,1.40000000000001,-22.2821416870349)) ;
#112690=CARTESIAN_POINT('Origin',(1.15,2.95,-21.9631676725155)) ;
#112691=CARTESIAN_POINT('Origin',(1.15,3.04189189189189,-21.7855279241354)) ;
#112692=CARTESIAN_POINT('Origin',(-0.900000000000002,2.1568323274845,-21.17)) ;
#112693=CARTESIAN_POINT('Origin',(-0.900000000000002,2.1568323274845,-21.17)) ;
#112694=CARTESIAN_POINT('Origin',(-0.900000000000002,2.1568323274845,-21.17)) ;
#112695=CARTESIAN_POINT('Origin',(-0.900000000000001,1.40000000000001,-22.2821416870349)) ;
#112696=CARTESIAN_POINT('Origin',(-0.900000000000002,1.55483870967742,-22.1555519007746)) ;
#112697=CARTESIAN_POINT('Origin',(1.15,3.8,-20.32)) ;
#112698=CARTESIAN_POINT('Origin',(1.15,2.33447207586456,-21.0781081081081)) ;
#112699=CARTESIAN_POINT('Origin',(-1.,2.1568323274845,-21.17)) ;
#112700=CARTESIAN_POINT('Origin',(1.15,2.1568323274845,-21.17)) ;
#112701=CARTESIAN_POINT('Origin',(-0.900000000000001,3.8,-21.17)) ;
#112702=CARTESIAN_POINT('Origin',(-0.900000000000002,1.02736587339765,-21.17)) ;
#112703=CARTESIAN_POINT('Origin',(-0.900000000000001,3.8,-20.32)) ;
#112704=CARTESIAN_POINT('Origin',(-0.900000000000002,1.02736587339765,-21.17)) ;
#112705=CARTESIAN_POINT('Origin',(13.9153543900904,1.4,-18.3578583129651)) ;
#112706=CARTESIAN_POINT('Origin',(8.49172374697002,1.4,-18.3578583129651)) ;
#112707=CARTESIAN_POINT('Origin',(-0.900000000000001,1.40000000000001,-18.3578583129651)) ;
#112708=CARTESIAN_POINT('Origin',(-0.900000000000002,1.6,-20.32)) ;
#112709=CARTESIAN_POINT('Origin',(-0.900000000000002,1.6,-18.3578583129651)) ;
#112710=CARTESIAN_POINT('Origin',(-0.900000000000002,2.95,-20.32)) ;
#112711=CARTESIAN_POINT('Origin',(-0.900000000000002,2.95,-18.6768323274845)) ;
#112712=CARTESIAN_POINT('Origin',(1.15,2.1568323274845,-21.17)) ;
#112713=CARTESIAN_POINT('Origin',(1.15,2.1568323274845,-20.97)) ;
#112714=CARTESIAN_POINT('Origin',(-0.900000000000002,1.02736587339765,-21.17)) ;
#112715=CARTESIAN_POINT('Origin',(-0.900000000000001,1.40000000000001,-18.3578583129651)) ;
#112716=CARTESIAN_POINT('Origin',(-0.900000000000002,1.55483870967743,-18.4844480992254)) ;
#112717=CARTESIAN_POINT('Origin',(-0.900000000000002,2.95,-18.6768323274845)) ;
#112718=CARTESIAN_POINT('Origin',(-0.900000000000002,2.95,-18.6768323274845)) ;
#112719=CARTESIAN_POINT('Origin',(-0.900000000000001,2.95,-18.6768323274845)) ;
#112720=CARTESIAN_POINT('Origin',(1.15,2.21886116991581,-20.97)) ;
#112721=CARTESIAN_POINT('Ctrl Pts',(1.15,1.02736587339765,-21.07)) ;
#112722=CARTESIAN_POINT('Ctrl Pts',(1.1608920328805,1.02736587339765,-21.07)) ;
#112723=CARTESIAN_POINT('Ctrl Pts',(1.17195716626105,1.02622125393927,-21.068143843926)) ;
#112724=CARTESIAN_POINT('Ctrl Pts',(1.1820844490224,1.02414637334385,-21.0647131887908)) ;
#112725=CARTESIAN_POINT('Ctrl Pts',(1.19245005921088,1.02202266415684,-21.0612017993431)) ;
#112726=CARTESIAN_POINT('Ctrl Pts',(1.20216743701154,1.01888103823701,-21.0559601980703)) ;
#112727=CARTESIAN_POINT('Ctrl Pts',(1.21053792402812,1.01518120925307,-21.0495937168021)) ;
#112728=CARTESIAN_POINT('Ctrl Pts',(1.219343173684,1.01128921135341,-21.0428965608439)) ;
#112729=CARTESIAN_POINT('Ctrl Pts',(1.22692289939014,1.00668521903338,-21.0347851615315)) ;
#112730=CARTESIAN_POINT('Ctrl Pts',(1.23290049538659,1.00186003905466,-21.0259241259624)) ;
#112731=CARTESIAN_POINT('Ctrl Pts',(1.23922345568944,0.9967560772818,-21.01655113117)) ;
#112732=CARTESIAN_POINT('Ctrl Pts',(1.24392209779927,0.991279542094837,
-21.0061045599897)) ;
#112733=CARTESIAN_POINT('Ctrl Pts',(1.24674870216524,0.985895902333124,
-20.9952920665297)) ;
#112734=CARTESIAN_POINT('Ctrl Pts',(1.24889292215336,0.981811953364218,
-20.9870898699727)) ;
#112735=CARTESIAN_POINT('Ctrl Pts',(1.25,0.977715885027402,-20.9785491686292)) ;
#112736=CARTESIAN_POINT('Ctrl Pts',(1.25,0.973783447787483,-20.97)) ;
#112737=CARTESIAN_POINT('Origin',(-0.900000000000001,3.8,-20.32)) ;
#112738=CARTESIAN_POINT('Origin',(-0.900000000000002,1.02736587339765,-19.47)) ;
#112739=CARTESIAN_POINT('Origin',(-0.900000000000001,3.8,-19.47)) ;
#112740=CARTESIAN_POINT('Origin',(-0.900000000000002,2.1568323274845,-19.47)) ;
#112741=CARTESIAN_POINT('Origin',(-0.900000000000002,1.02736587339765,-19.47)) ;
#112742=CARTESIAN_POINT('Origin',(-0.900000000000001,3.8,-20.32)) ;
#112743=CARTESIAN_POINT('Origin',(-0.900000000000002,2.1568323274845,-19.47)) ;
#112744=CARTESIAN_POINT('Origin',(-1.,2.95,-18.6768323274845)) ;
#112745=CARTESIAN_POINT('Origin',(1.15,2.95,-18.6768323274845)) ;
#112746=CARTESIAN_POINT('Origin',(1.15,3.15,-17.77)) ;
#112747=CARTESIAN_POINT('Origin',(1.15,3.15,-18.6768323274845)) ;
#112748=CARTESIAN_POINT('Ctrl Pts',(1.11028558574902,0.930383836951476,
-21.1949942836581)) ;
#112749=CARTESIAN_POINT('Ctrl Pts',(1.14039000477524,0.892136466138335,
-21.0699697185941)) ;
#112750=CARTESIAN_POINT('Ctrl Pts',(1.13015013463564,1.02610337426265,-21.0678511248828)) ;
#112751=CARTESIAN_POINT('Ctrl Pts',(1.17639690652712,0.935225109827649,
-21.2101257399467)) ;
#112752=CARTESIAN_POINT('Ctrl Pts',(1.15491086542929,0.891146666106391,
-21.0692760504014)) ;
#112753=CARTESIAN_POINT('Ctrl Pts',(1.16319405445819,1.03078047702076,-21.0751648742452)) ;
#112754=CARTESIAN_POINT('Ctrl Pts',(1.24701363206612,0.927145283841802,
-21.1855522038251)) ;
#112755=CARTESIAN_POINT('Ctrl Pts',(1.1775998083145,0.893467326853946,-21.0726373120314)) ;
#112756=CARTESIAN_POINT('Ctrl Pts',(1.19848758201044,1.02297467453099,-21.063287122555)) ;
#112757=CARTESIAN_POINT('Ctrl Pts',(1.33816236560056,0.900022463714237,
-21.0898088506149)) ;
#112758=CARTESIAN_POINT('Ctrl Pts',(1.22862786282608,0.888037626604027,
-21.043153964324)) ;
#112759=CARTESIAN_POINT('Ctrl Pts',(1.24403288504499,0.996768276947721,
-21.0170266594133)) ;
#112760=CARTESIAN_POINT('Ctrl Pts',(1.35959492575595,0.881455895025368,
-21.018532341229)) ;
#112761=CARTESIAN_POINT('Ctrl Pts',(1.25320519750646,0.880428099081736,
-21.0110649378273)) ;
#112762=CARTESIAN_POINT('Ctrl Pts',(1.25473603279823,0.978811277328825,
-20.982557487151)) ;
#112763=CARTESIAN_POINT('Ctrl Pts',(1.34615355831623,0.867571605181219,
-20.9527925825335)) ;
#112764=CARTESIAN_POINT('Ctrl Pts',(1.25176090202828,0.870950130624649,
-20.9694490170578)) ;
#112765=CARTESIAN_POINT('Ctrl Pts',(1.24801589497573,0.965423101361819,
-20.9508695481641)) ;
#112766=CARTESIAN_POINT('Origin',(1.35,0.973783447787483,-20.97)) ;
#112767=CARTESIAN_POINT('Origin',(-0.900000000000002,1.02736587339765,-19.47)) ;
#112768=CARTESIAN_POINT('',(-0.957735026918965,0.969630846478687,-19.527735026919)) ;
#112769=CARTESIAN_POINT('Origin',(-0.900000000000002,1.02736587339765,-19.47)) ;
#112770=CARTESIAN_POINT('Origin',(-0.900000000000002,2.1568323274845,-19.47)) ;
#112771=CARTESIAN_POINT('Origin',(-0.900000000000002,2.1568323274845,-19.47)) ;
#112772=CARTESIAN_POINT('Origin',(1.15,2.95,-18.6768323274845)) ;
#112773=CARTESIAN_POINT('Origin',(1.15,3.04189189189189,-18.8544720758646)) ;
#112774=CARTESIAN_POINT('Origin',(1.35,3.8,-20.32)) ;
#112775=CARTESIAN_POINT('Origin',(1.35,0.973783447787484,-19.67)) ;
#112776=CARTESIAN_POINT('Origin',(-1.,2.1568323274845,-19.47)) ;
#112777=CARTESIAN_POINT('Origin',(1.15,2.1568323274845,-19.47)) ;
#112778=CARTESIAN_POINT('Origin',(1.15,3.8,-20.32)) ;
#112779=CARTESIAN_POINT('Origin',(1.15,2.33447207586456,-19.5618918918919)) ;
#112780=CARTESIAN_POINT('Ctrl Pts',(1.34754079198595,0.869159571293143,
-19.6797485347856)) ;
#112781=CARTESIAN_POINT('Ctrl Pts',(1.25183398383322,0.871999770424367,
-19.6659986517603)) ;
#112782=CARTESIAN_POINT('Ctrl Pts',(1.24871534599026,0.966951450593966,
-19.6855357130736)) ;
#112783=CARTESIAN_POINT('Ctrl Pts',(1.35788971301869,0.882932151572375,
-19.615777428268)) ;
#112784=CARTESIAN_POINT('Ctrl Pts',(1.25138796519091,0.881019151005352,
-19.6264872814237)) ;
#112785=CARTESIAN_POINT('Ctrl Pts',(1.25389076424431,0.980237216252235,
-19.6546886342593)) ;
#112786=CARTESIAN_POINT('Ctrl Pts',(1.33642796493172,0.900551643074762,
-19.5483167189689)) ;
#112787=CARTESIAN_POINT('Ctrl Pts',(1.22773025960896,0.888154519889412,
-19.5963023541524)) ;
#112788=CARTESIAN_POINT('Ctrl Pts',(1.2431720339903,0.997278352451067,-19.6220644582831)) ;
#112789=CARTESIAN_POINT('Ctrl Pts',(1.24851212064762,0.926675670999774,
-19.4561118541865)) ;
#112790=CARTESIAN_POINT('Ctrl Pts',(1.17855408504649,0.893378082604311,
-19.5679358454001)) ;
#112791=CARTESIAN_POINT('Ctrl Pts',(1.1992394771088,1.02252144543593,-19.5775111840606)) ;
#112792=CARTESIAN_POINT('Ctrl Pts',(1.18212686068544,0.934567888698279,
-19.4318922599007)) ;
#112793=CARTESIAN_POINT('Ctrl Pts',(1.15690947476174,0.891342319658717,
-19.5705013022393)) ;
#112794=CARTESIAN_POINT('Ctrl Pts',(1.16605892368793,1.03014681530421,-19.5658041235204)) ;
#112795=CARTESIAN_POINT('Ctrl Pts',(1.11776263740947,0.930888708579155,
-19.4434235819161)) ;
#112796=CARTESIAN_POINT('Ctrl Pts',(1.1419771056359,0.892059806627037,-19.5700822996553)) ;
#112797=CARTESIAN_POINT('Ctrl Pts',(1.13388624958142,1.02659206201251,-19.5713778561013)) ;
#112798=CARTESIAN_POINT('Ctrl Pts',(1.15,1.02736587339764,-19.57)) ;
#112799=CARTESIAN_POINT('Ctrl Pts',(1.15623005440502,1.02736587339759,-19.5699999999999)) ;
#112800=CARTESIAN_POINT('Ctrl Pts',(1.16249579431471,1.02700282517053,-19.570590866069)) ;
#112801=CARTESIAN_POINT('Ctrl Pts',(1.16857840195431,1.02630083270769,-19.5717409394467)) ;
#112802=CARTESIAN_POINT('Ctrl Pts',(1.1798885498395,1.02499553092934,-19.5738794137247)) ;
#112803=CARTESIAN_POINT('Ctrl Pts',(1.19084787809767,1.02245621903271,-19.5780506966152)) ;
#112804=CARTESIAN_POINT('Ctrl Pts',(1.20043335385463,1.01914369852331,-19.5836491064379)) ;
#112805=CARTESIAN_POINT('Ctrl Pts',(1.21063893018497,1.01561688548223,-19.5896096868225)) ;
#112806=CARTESIAN_POINT('Ctrl Pts',(1.21965078109605,1.01112191387731,-19.5973548511019)) ;
#112807=CARTESIAN_POINT('Ctrl Pts',(1.226898722009,1.00626683908294,-19.6060735848543)) ;
#112808=CARTESIAN_POINT('Ctrl Pts',(1.23435386869391,1.0012729663137,-19.6150415717366)) ;
#112809=CARTESIAN_POINT('Ctrl Pts',(1.24017476602864,0.995763540409855,
-19.6252870264069)) ;
#112810=CARTESIAN_POINT('Ctrl Pts',(1.24405759382605,0.990267693778535,
-19.6360416572305)) ;
#112811=CARTESIAN_POINT('Ctrl Pts',(1.24795610732226,0.9847496452368,-19.6468397341991)) ;
#112812=CARTESIAN_POINT('Ctrl Pts',(1.25,0.97910634898267,-19.658427945028)) ;
#112813=CARTESIAN_POINT('Ctrl Pts',(1.25,0.973783447787483,-19.67)) ;
#112814=CARTESIAN_POINT('Origin',(1.15,2.1568323274845,-19.47)) ;
#112815=CARTESIAN_POINT('Origin',(1.15,2.1568323274845,-19.67)) ;
#112816=CARTESIAN_POINT('Origin',(1.15,2.21886116991581,-19.67)) ;
#112817=CARTESIAN_POINT('Origin',(1.5,2.3,-20.72)) ;
#112818=CARTESIAN_POINT('Ctrl Pts',(0.549999999999999,4.04473197180487,
-20.77)) ;
#112819=CARTESIAN_POINT('Ctrl Pts',(0.549999999999999,4.04340510574359,
-20.7720183916746)) ;
#112820=CARTESIAN_POINT('Ctrl Pts',(0.549938912488049,4.04197482121862,
-20.7739799093559)) ;
#112821=CARTESIAN_POINT('Ctrl Pts',(0.549362579613713,4.03414945156058,
-20.783763201697)) ;
#112822=CARTESIAN_POINT('Ctrl Pts',(0.548040652125092,4.02633974827551,
-20.7905458262272)) ;
#112823=CARTESIAN_POINT('Ctrl Pts',(0.544205267183616,4.00519499286846,
-20.8046839427888)) ;
#112824=CARTESIAN_POINT('Ctrl Pts',(0.541221332378481,3.99011995637977,
-20.8112251154482)) ;
#112825=CARTESIAN_POINT('Ctrl Pts',(0.537814556431532,3.96385893187633,
-20.81793059224)) ;
#112826=CARTESIAN_POINT('Ctrl Pts',(0.53660254037844,3.95132390702842,-20.82)) ;
#112827=CARTESIAN_POINT('Ctrl Pts',(0.53660254037844,3.93764017256378,-20.82)) ;
#112828=CARTESIAN_POINT('Origin',(-0.4,2.3,-20.72)) ;
#112829=CARTESIAN_POINT('Origin',(-0.4,-3.4,-20.72)) ;
#112830=CARTESIAN_POINT('Origin',(-0.4,-3.36847777691809,-20.72)) ;
#112831=CARTESIAN_POINT('Origin',(1.5,2.3,-20.72)) ;
#112832=CARTESIAN_POINT('Ctrl Pts',(0.536602540378443,2.83090991212703,
-20.82)) ;
#112833=CARTESIAN_POINT('Ctrl Pts',(0.536602540378443,2.80627146475521,
-20.82)) ;
#112834=CARTESIAN_POINT('Ctrl Pts',(0.538106903229136,2.77742679387696,
-20.8179527908127)) ;
#112835=CARTESIAN_POINT('Ctrl Pts',(0.54518697656879,2.71156844363407,-20.8020839809802)) ;
#112836=CARTESIAN_POINT('Ctrl Pts',(0.55,2.68282906082737,-20.7881020558141)) ;
#112837=CARTESIAN_POINT('Ctrl Pts',(0.549999999999999,2.65280931275608,
-20.77)) ;
#112838=CARTESIAN_POINT('Origin',(0.400000000000001,2.29999999999999,-20.72)) ;
#112839=CARTESIAN_POINT('Origin',(0.0725078566451197,-4.04348900069683,
-20.2474921433549)) ;
#112840=CARTESIAN_POINT('Origin',(-0.4,-3.36847777691809,-20.72)) ;
#112841=CARTESIAN_POINT('Origin',(-0.0979344438426628,-3.8,-20.4179344438427)) ;
#112842=CARTESIAN_POINT('Origin',(1.5,2.3,-19.92)) ;
#112843=CARTESIAN_POINT('Ctrl Pts',(0.536602540378444,3.93764017256378,
-19.82)) ;
#112844=CARTESIAN_POINT('Ctrl Pts',(0.536602540378444,3.93925361219679,
-19.82)) ;
#112845=CARTESIAN_POINT('Ctrl Pts',(0.536619300889441,3.94087098264046,
-19.8200289972578)) ;
#112846=CARTESIAN_POINT('Ctrl Pts',(0.536997639747773,3.95938954612139,
-19.8206858128959)) ;
#112847=CARTESIAN_POINT('Ctrl Pts',(0.539142315171152,3.97567120869963,
-19.8243120615618)) ;
#112848=CARTESIAN_POINT('Ctrl Pts',(0.544035197036784,4.00535605098148,
-19.8353993916663)) ;
#112849=CARTESIAN_POINT('Ctrl Pts',(0.546989816174504,4.01946236900651,
-19.8435699446353)) ;
#112850=CARTESIAN_POINT('Ctrl Pts',(0.549463062495712,4.03595536007421,
-19.8585473816974)) ;
#112851=CARTESIAN_POINT('Ctrl Pts',(0.550000000000877,4.04078397701442,
-19.8639944203465)) ;
#112852=CARTESIAN_POINT('Ctrl Pts',(0.549999999999999,4.04473197181447,
-19.8700000000146)) ;
#112853=CARTESIAN_POINT('Origin',(-0.4,2.3,-19.92)) ;
#112854=CARTESIAN_POINT('Origin',(0.4,2.29999999999999,-20.72)) ;
#112855=CARTESIAN_POINT('Origin',(0.4,-3.36847777691809,-20.72)) ;
#112856=CARTESIAN_POINT('Origin',(-0.0979344438426628,-3.8,-20.4179344438427)) ;
#112857=CARTESIAN_POINT('Origin',(-0.0979344438426628,-3.8,-20.4179344438427)) ;
#112858=CARTESIAN_POINT('Origin',(-0.0979344438426627,-3.8,-20.4179344438427)) ;
#112859=CARTESIAN_POINT('Origin',(-0.4,2.3,-19.92)) ;
#112860=CARTESIAN_POINT('Origin',(-0.4,-3.36847777691809,-19.92)) ;
#112861=CARTESIAN_POINT('Origin',(0.190875981738719,-3.6672263744342,-20.5108759817387)) ;
#112862=CARTESIAN_POINT('Origin',(0.400000000000001,-3.36847777691809,-20.72)) ;
#112863=CARTESIAN_POINT('Origin',(0.0979344438426626,-3.8,-20.4179344438427)) ;
#112864=CARTESIAN_POINT('Origin',(0.15,-3.8,-20.4179344438427)) ;
#112865=CARTESIAN_POINT('Origin',(0.0979344438426627,-3.8,-20.4179344438427)) ;
#112866=CARTESIAN_POINT('Origin',(-0.0979344438426628,-3.8,-19.82)) ;
#112867=CARTESIAN_POINT('Origin',(-0.0979344438426628,-3.8,-20.2220655561573)) ;
#112868=CARTESIAN_POINT('Origin',(-0.174966890829628,-3.68995364716148,
-20.1450331091704)) ;
#112869=CARTESIAN_POINT('Origin',(-0.400000000000001,-3.36847777691809,
-19.92)) ;
#112870=CARTESIAN_POINT('Origin',(-0.0979344438426627,-3.8,-20.2220655561573)) ;
#112871=CARTESIAN_POINT('Origin',(0.0979344438426627,-3.8,-20.4179344438427)) ;
#112872=CARTESIAN_POINT('Origin',(0.0979344438426628,-3.8,-20.4179344438427)) ;
#112873=CARTESIAN_POINT('Origin',(-0.0979344438426628,-3.8,-20.2220655561573)) ;
#112874=CARTESIAN_POINT('Origin',(-0.0979344438426628,-3.8,-20.2220655561573)) ;
#112875=CARTESIAN_POINT('Origin',(0.0979344438426627,-3.8,-19.82)) ;
#112876=CARTESIAN_POINT('Origin',(0.0979344438426627,-3.8,-20.2220655561573)) ;
#112877=CARTESIAN_POINT('Origin',(-1.11032778078669,-3.8,-20.2220655561573)) ;
#112878=CARTESIAN_POINT('Origin',(0.0979344438426626,-3.8,-20.2220655561573)) ;
#112879=CARTESIAN_POINT('Origin',(0.0979344438426627,-3.8,-20.2220655561573)) ;
#112880=CARTESIAN_POINT('Origin',(0.0979344438426627,-3.8,-20.2220655561573)) ;
#112881=CARTESIAN_POINT('Origin',(0.438350729213467,-3.31369102089885,-19.8816492707865)) ;
#112882=CARTESIAN_POINT('Origin',(0.399999999999999,-3.36847777691809,-19.92)) ;
#112883=CARTESIAN_POINT('Origin',(0.4,2.3,-19.92)) ;
#112884=CARTESIAN_POINT('Origin',(0.4,-3.36847777691809,-19.92)) ;
#112885=CARTESIAN_POINT('Origin',(0.4,2.29999999999999,-19.92)) ;
#112886=CARTESIAN_POINT('Origin',(1.5,2.3,-19.92)) ;
#112887=CARTESIAN_POINT('Ctrl Pts',(0.55,2.65280931275593,-19.8700000000001)) ;
#112888=CARTESIAN_POINT('Ctrl Pts',(0.550000000000013,2.67648433237897,
-19.8557238466627)) ;
#112889=CARTESIAN_POINT('Ctrl Pts',(0.546908864252789,2.69988533923261,
-19.8435257008476)) ;
#112890=CARTESIAN_POINT('Ctrl Pts',(0.539540151921447,2.76165254733706,
-19.8240915981901)) ;
#112891=CARTESIAN_POINT('Ctrl Pts',(0.536602540378444,2.79600904778111,
-19.82)) ;
#112892=CARTESIAN_POINT('Ctrl Pts',(0.536602540378444,2.83090991212703,
-19.82)) ;
#112893=CARTESIAN_POINT('Origin',(8.,3.4,-20.72)) ;
#112894=CARTESIAN_POINT('Origin',(7.96847777691809,3.4,-20.72)) ;
#112895=CARTESIAN_POINT('Origin',(1.5,4.2,-20.72)) ;
#112896=CARTESIAN_POINT('Origin',(7.96847777691809,4.2,-20.72)) ;
#112897=CARTESIAN_POINT('Origin',(8.64348900069683,3.87250785664512,-20.2474921433549)) ;
#112898=CARTESIAN_POINT('Origin',(7.96847777691809,3.4,-20.72)) ;
#112899=CARTESIAN_POINT('Origin',(8.4,3.70206555615734,-20.4179344438427)) ;
#112900=CARTESIAN_POINT('Origin',(8.26722637443421,3.99087598173872,-20.5108759817387)) ;
#112901=CARTESIAN_POINT('Origin',(7.96847777691809,4.2,-20.72)) ;
#112902=CARTESIAN_POINT('Origin',(8.4,3.89793444384266,-20.4179344438427)) ;
#112903=CARTESIAN_POINT('Origin',(8.4,3.95,-20.4179344438427)) ;
#112904=CARTESIAN_POINT('Origin',(8.4,3.70206555615734,-20.4179344438427)) ;
#112905=CARTESIAN_POINT('Origin',(8.4,3.89793444384266,-20.4179344438427)) ;
#112906=CARTESIAN_POINT('Origin',(8.4,3.70206555615734,-20.4179344438427)) ;
#112907=CARTESIAN_POINT('Origin',(8.4,3.70206555615734,-20.4179344438427)) ;
#112908=CARTESIAN_POINT('Origin',(1.5,3.4,-19.92)) ;
#112909=CARTESIAN_POINT('Origin',(7.96847777691809,3.4,-19.92)) ;
#112910=CARTESIAN_POINT('Origin',(1.5,4.2,-19.92)) ;
#112911=CARTESIAN_POINT('Origin',(7.96847777691809,4.2,-19.92)) ;
#112912=CARTESIAN_POINT('Origin',(8.4,3.89793444384266,-20.4179344438427)) ;
#112913=CARTESIAN_POINT('Origin',(8.4,3.89793444384266,-20.4179344438427)) ;
#112914=CARTESIAN_POINT('Origin',(8.4,3.70206555615734,-19.82)) ;
#112915=CARTESIAN_POINT('Origin',(8.4,3.70206555615734,-20.2220655561573)) ;
#112916=CARTESIAN_POINT('Origin',(8.28995364716148,3.62503310917037,-20.1450331091704)) ;
#112917=CARTESIAN_POINT('Origin',(7.96847777691809,3.4,-19.92)) ;
#112918=CARTESIAN_POINT('Origin',(8.4,3.70206555615734,-20.2220655561573)) ;
#112919=CARTESIAN_POINT('Origin',(7.91369102089885,4.23835072921347,-19.8816492707865)) ;
#112920=CARTESIAN_POINT('Origin',(7.96847777691809,4.2,-19.92)) ;
#112921=CARTESIAN_POINT('Origin',(8.4,3.89793444384266,-20.2220655561573)) ;
#112922=CARTESIAN_POINT('Origin',(8.4,3.89793444384266,-19.82)) ;
#112923=CARTESIAN_POINT('Origin',(8.4,3.89793444384266,-20.2220655561573)) ;
#112924=CARTESIAN_POINT('Origin',(8.4,3.70206555615734,-20.2220655561573)) ;
#112925=CARTESIAN_POINT('Origin',(8.4,3.70206555615734,-20.2220655561573)) ;
#112926=CARTESIAN_POINT('Origin',(8.4,3.89793444384266,-20.2220655561573)) ;
#112927=CARTESIAN_POINT('Origin',(8.4,3.89793444384266,-20.2220655561573)) ;
#112928=CARTESIAN_POINT('Origin',(8.4,2.68967221921331,-20.2220655561573)) ;
#112929=CARTESIAN_POINT('Origin',(9.9,6.8847127088383,-22.86)) ;
#112930=CARTESIAN_POINT('Origin',(9.9,6.8847127088383,-21.2797127088383)) ;
#112931=CARTESIAN_POINT('Origin',(8.77035388141948,6.69643835574155,-21.0914383557416)) ;
#112932=CARTESIAN_POINT('Ctrl Pts',(8.58356010126946,6.66256607592812,-20.958926683545)) ;
#112933=CARTESIAN_POINT('Ctrl Pts',(8.58266714977878,6.65676189123867,-20.9587778582965)) ;
#112934=CARTESIAN_POINT('Ctrl Pts',(8.58182526931893,6.6507714222091,-20.9591141714741)) ;
#112935=CARTESIAN_POINT('Ctrl Pts',(8.58032528754329,6.63886560514773,-20.9609127350998)) ;
#112936=CARTESIAN_POINT('Ctrl Pts',(8.57966270906097,6.63295370212089,-20.9623448243331)) ;
#112937=CARTESIAN_POINT('Ctrl Pts',(8.57906641006211,6.62681909302424,-20.9644771744941)) ;
#112938=CARTESIAN_POINT('Ctrl Pts',(8.57903375157323,6.62647998752457,-20.9645971697287)) ;
#112939=CARTESIAN_POINT('Ctrl Pts',(8.57846569624192,6.6205258217488,-20.966741731681)) ;
#112940=CARTESIAN_POINT('Ctrl Pts',(8.57802501793965,6.61503168015257,-20.9693142858557)) ;
#112941=CARTESIAN_POINT('Ctrl Pts',(8.57766199200569,6.60925146760312,-20.9727462133234)) ;
#112942=CARTESIAN_POINT('Ctrl Pts',(8.57762821177172,6.60869602779103,-20.9730838351647)) ;
#112943=CARTESIAN_POINT('Ctrl Pts',(8.57728522755447,6.60286036001468,-20.9767147989572)) ;
#112944=CARTESIAN_POINT('Ctrl Pts',(8.57709550103272,6.59788070192354,-20.9805482210562)) ;
#112945=CARTESIAN_POINT('Ctrl Pts',(8.57703980289278,6.59299711069415,-20.9851723373547)) ;
#112946=CARTESIAN_POINT('Ctrl Pts',(8.57703670271021,6.5926595243005,-20.985496892542)) ;
#112947=CARTESIAN_POINT('Ctrl Pts',(8.57701334129169,6.58927432516128,-20.9888013815953)) ;
#112948=CARTESIAN_POINT('Ctrl Pts',(8.57705699426434,6.5864297120155,-20.9919917444088)) ;
#112949=CARTESIAN_POINT('Ctrl Pts',(8.57735031225521,6.57961409340222,-21.0007954417554)) ;
#112950=CARTESIAN_POINT('Ctrl Pts',(8.57770856513437,6.57604383182914,-21.0066682455399)) ;
#112951=CARTESIAN_POINT('Ctrl Pts',(8.57865704971091,6.57055741297635,-21.0183322193388)) ;
#112952=CARTESIAN_POINT('Ctrl Pts',(8.57922107378969,6.56851476050446,-21.0240736349077)) ;
#112953=CARTESIAN_POINT('Ctrl Pts',(8.57993695782543,6.56687610193753,-21.0304559348163)) ;
#112954=CARTESIAN_POINT('Ctrl Pts',(8.58000419042984,6.56673001682056,-21.0310478351839)) ;
#112955=CARTESIAN_POINT('Ctrl Pts',(8.58074399738015,6.56520526212529,-21.037481251735)) ;
#112956=CARTESIAN_POINT('Ctrl Pts',(8.58149993293339,6.56438134785785,-21.0433541800929)) ;
#112957=CARTESIAN_POINT('Ctrl Pts',(8.58236768178469,6.56403389662205,-21.0494987578227)) ;
#112958=CARTESIAN_POINT('Ctrl Pts',(8.58242358604544,6.56401394107887,-21.0498921736313)) ;
#112959=CARTESIAN_POINT('Ctrl Pts',(8.58283067264383,6.56388592662946,-21.0527394234264)) ;
#112960=CARTESIAN_POINT('Ctrl Pts',(8.58319156240649,6.56386525642005,-21.0551699505828)) ;
#112961=CARTESIAN_POINT('Ctrl Pts',(8.58356019967707,6.56392669994633,-21.0575662650647)) ;
#112962=CARTESIAN_POINT('Origin',(9.9,6.8847127088383,-21.2797127088383)) ;
#112963=CARTESIAN_POINT('Origin',(9.9,6.8847127088383,-21.2797127088383)) ;
#112964=CARTESIAN_POINT('Origin',(9.9,6.8847127088383,-21.2797127088383)) ;
#112965=CARTESIAN_POINT('Origin',(9.9,7.72792407799439,-22.86)) ;
#112966=CARTESIAN_POINT('Origin',(9.9,7.72792407799439,-21.2797127088383)) ;
#112967=CARTESIAN_POINT('Origin',(9.90000000000001,4.35421736843756,-21.2797127088383)) ;
#112968=CARTESIAN_POINT('Origin',(9.9,7.72792407799439,-21.2797127088383)) ;
#112969=CARTESIAN_POINT('Origin',(9.9,7.72792407799439,-21.2797127088383)) ;
#112970=CARTESIAN_POINT('Origin',(9.9,7.72792407799439,-21.2797127088383)) ;
#112971=CARTESIAN_POINT('Origin',(10.9628342502842,7.37364599456632,-21.4568517505523)) ;
#112972=CARTESIAN_POINT('Ctrl Pts',(8.56837732530586,8.2772075582313,-21.0525052537977)) ;
#112973=CARTESIAN_POINT('Ctrl Pts',(8.56753565030797,8.2774881236726,-21.0466129921974)) ;
#112974=CARTESIAN_POINT('Ctrl Pts',(8.56682045541689,8.2772118066791,-21.0405412944396)) ;
#112975=CARTESIAN_POINT('Ctrl Pts',(8.56575413148015,8.27538624160209,-21.0287284721177)) ;
#112976=CARTESIAN_POINT('Ctrl Pts',(8.56538426077852,8.27391165896476,-21.0229905624278)) ;
#112977=CARTESIAN_POINT('Ctrl Pts',(8.56517777855932,8.27166501362512,-21.0170147754472)) ;
#112978=CARTESIAN_POINT('Ctrl Pts',(8.56516523451682,8.27151619608598,-21.0166276382838)) ;
#112979=CARTESIAN_POINT('Ctrl Pts',(8.56497390811214,8.26902793125451,-21.0102953359912)) ;
#112980=CARTESIAN_POINT('Ctrl Pts',(8.56499903025534,8.2659763012945,-21.0045357784659)) ;
#112981=CARTESIAN_POINT('Ctrl Pts',(8.56538588200257,8.26046191593055,-20.9965906723681)) ;
#112982=CARTESIAN_POINT('Ctrl Pts',(8.56556309332507,8.25853771611458,-20.9941212364558)) ;
#112983=CARTESIAN_POINT('Ctrl Pts',(8.56628156514548,8.25214511987158,-20.9868017566891)) ;
#112984=CARTESIAN_POINT('Ctrl Pts',(8.56700742874793,8.2472021625627,-20.982305445231)) ;
#112985=CARTESIAN_POINT('Ctrl Pts',(8.56880713798126,8.23661566152161,-20.97462449488)) ;
#112986=CARTESIAN_POINT('Ctrl Pts',(8.5698603939132,8.23102391526957,-20.9713848807255)) ;
#112987=CARTESIAN_POINT('Ctrl Pts',(8.57116255171755,8.22459552194118,-20.9684467745269)) ;
#112988=CARTESIAN_POINT('Ctrl Pts',(8.57127495810218,8.22404408343782,-20.9682006607901)) ;
#112989=CARTESIAN_POINT('Ctrl Pts',(8.57260511146312,8.21755901312581,-20.9653749153055)) ;
#112990=CARTESIAN_POINT('Ctrl Pts',(8.5739562967284,8.21135759730909,-20.9633463864276)) ;
#112991=CARTESIAN_POINT('Ctrl Pts',(8.57552311082417,8.20452945286284,-20.9617495443173)) ;
#112992=CARTESIAN_POINT('Ctrl Pts',(8.57564505123012,8.20400026307089,-20.961629826956)) ;
#112993=CARTESIAN_POINT('Ctrl Pts',(8.57731301559524,8.1967919362264,-20.960053462537)) ;
#112994=CARTESIAN_POINT('Ctrl Pts',(8.57896065127869,8.19002168485366,-20.959210969344)) ;
#112995=CARTESIAN_POINT('Ctrl Pts',(8.58161366784366,8.17959769015482,-20.9587553172771)) ;
#112996=CARTESIAN_POINT('Ctrl Pts',(8.58258362864269,8.17587911616515,-20.9587639381071)) ;
#112997=CARTESIAN_POINT('Ctrl Pts',(8.58356010126947,8.17221734381475,-20.9589266835449)) ;
#112998=CARTESIAN_POINT('Origin',(7.96824861826159,6.56275414521524,-19.6822458547848)) ;
#112999=CARTESIAN_POINT('Origin',(8.5968837020256,6.66156024040156,-19.5912434752671)) ;
#113000=CARTESIAN_POINT('Origin',(9.9,6.8847127088383,-19.3602872911617)) ;
#113001=CARTESIAN_POINT('Origin',(9.9,6.8847127088383,-22.86)) ;
#113002=CARTESIAN_POINT('Origin',(9.9,6.8847127088383,-19.3602872911617)) ;
#113003=CARTESIAN_POINT('Origin',(9.9,6.8847127088383,-19.3602872911617)) ;
#113004=CARTESIAN_POINT('Origin',(9.9,6.8847127088383,-19.3602872911617)) ;
#113005=CARTESIAN_POINT('Origin',(9.9,6.8,-19.3602872911617)) ;
#113006=CARTESIAN_POINT('Origin',(9.9,7.72792407799439,-19.3602872911617)) ;
#113007=CARTESIAN_POINT('Origin',(9.9,7.72792407799439,-22.86)) ;
#113008=CARTESIAN_POINT('Origin',(9.9,7.72792407799439,-19.3602872911617)) ;
#113009=CARTESIAN_POINT('Origin',(9.9,7.72792407799439,-19.3602872911617)) ;
#113010=CARTESIAN_POINT('Origin',(9.9,7.72792407799439,-19.3602872911617)) ;
#113011=CARTESIAN_POINT('Origin',(9.60917571369883,7.82486550676144,-19.4087580055452)) ;
#113012=CARTESIAN_POINT('Origin',(8.59099001845867,8.18966234087289,-19.5851609739002)) ;
#113013=CARTESIAN_POINT('Origin',(0.45,4.4,-20.32)) ;
#113014=CARTESIAN_POINT('Origin',(0.45,4.4,-20.77)) ;
#113015=CARTESIAN_POINT('Origin',(0.45,4.4,-19.87)) ;
#113016=CARTESIAN_POINT('Origin',(-1.9,7.55,-22.86)) ;
#113017=CARTESIAN_POINT('Origin',(6.9,7.75,-22.86)) ;
#113018=CARTESIAN_POINT('Origin',(7.1,8.2,-22.86)) ;
#113019=CARTESIAN_POINT('Origin',(9.9,0.1,-22.86)) ;
#113020=CARTESIAN_POINT('Origin',(9.9,1.16528729116168,-22.86)) ;
#113021=CARTESIAN_POINT('Origin',(9.9,1.16528729116168,-22.3641618801782)) ;
#113022=CARTESIAN_POINT('Origin',(9.9,3.8,-20.32)) ;
#113023=CARTESIAN_POINT('Origin',(9.9,1.16528729116168,-18.2758381198218)) ;
#113024=CARTESIAN_POINT('Origin',(9.9,1.16528729116168,-22.3641618801782)) ;
#113025=CARTESIAN_POINT('Origin',(9.9,1.16528729116168,-22.86)) ;
#113026=CARTESIAN_POINT('Origin',(9.9,1.16528729116168,-18.2758381198218)) ;
#113027=CARTESIAN_POINT('Ctrl Pts',(0.55,0.3,-20.77)) ;
#113028=CARTESIAN_POINT('Ctrl Pts',(0.55,0.3,-20.87)) ;
#113029=CARTESIAN_POINT('Ctrl Pts',(0.45,0.3,-20.87)) ;
#113030=CARTESIAN_POINT('Ctrl Pts',(0.55,0.28690770353672,-20.7700000008182)) ;
#113031=CARTESIAN_POINT('Ctrl Pts',(0.549992696056738,0.300543498484345,
-20.8699926960962)) ;
#113032=CARTESIAN_POINT('Ctrl Pts',(0.450000000818259,0.286907703536713,
-20.87)) ;
#113033=CARTESIAN_POINT('Ctrl Pts',(0.552602750539093,0.273825167611082,
-20.7752055010782)) ;
#113034=CARTESIAN_POINT('Ctrl Pts',(0.546703256435903,0.299059401315785,
-20.8667032564359)) ;
#113035=CARTESIAN_POINT('Ctrl Pts',(0.455205501078185,0.273825167611091,
-20.8726027505391)) ;
#113036=CARTESIAN_POINT('Ctrl Pts',(0.56262134295865,0.249638145915901,
-20.7952426859173)) ;
#113037=CARTESIAN_POINT('Ctrl Pts',(0.544986924117065,0.28207277643954,
-20.8649869241171)) ;
#113038=CARTESIAN_POINT('Ctrl Pts',(0.4752426859173,0.249638145915891,-20.8826213429587)) ;
#113039=CARTESIAN_POINT('Ctrl Pts',(0.570033341471288,0.238545302291403,
-20.8100666829426)) ;
#113040=CARTESIAN_POINT('Ctrl Pts',(0.54711619685839,0.267914459835251,
-20.8671161968584)) ;
#113041=CARTESIAN_POINT('Ctrl Pts',(0.490066682942577,0.238545302291388,
-20.8900333414713)) ;
#113042=CARTESIAN_POINT('Ctrl Pts',(0.597801282701459,0.210777361061231,
-20.8656025654029)) ;
#113043=CARTESIAN_POINT('Ctrl Pts',(0.570853448890191,0.226374713859272,
-20.8908534488901)) ;
#113044=CARTESIAN_POINT('Ctrl Pts',(0.545602565402917,0.21077736106126,
-20.9178012827014)) ;
#113045=CARTESIAN_POINT('Ctrl Pts',(0.623746567173686,0.2,-20.9174931343473)) ;
#113046=CARTESIAN_POINT('Ctrl Pts',(0.610458667315294,0.2,-20.930458667316)) ;
#113047=CARTESIAN_POINT('Ctrl Pts',(0.597493134347343,0.2,-20.9437465671735)) ;
#113048=CARTESIAN_POINT('Ctrl Pts',(0.65,0.2,-20.97)) ;
#113049=CARTESIAN_POINT('Ctrl Pts',(0.65,0.2,-20.97)) ;
#113050=CARTESIAN_POINT('Ctrl Pts',(0.65,0.2,-20.97)) ;
#113051=CARTESIAN_POINT('Origin',(0.45,0.3,-20.77)) ;
#113052=CARTESIAN_POINT('Origin',(0.45,1.24941393210234E-16,-20.77)) ;
#113053=CARTESIAN_POINT('Origin',(0.45,4.4,-20.77)) ;
#113054=CARTESIAN_POINT('Origin',(0.45,4.4,-20.77)) ;
#113055=CARTESIAN_POINT('Origin',(0.45,4.4,-20.77)) ;
#113056=CARTESIAN_POINT('Origin',(0.549999999999999,4.4,-20.77)) ;
#113057=CARTESIAN_POINT('Origin',(-1.7,4.4,-20.77)) ;
#113058=CARTESIAN_POINT('Ctrl Pts',(-1.8,4.6,-20.97)) ;
#113059=CARTESIAN_POINT('Ctrl Pts',(-1.8,4.6,-20.97)) ;
#113060=CARTESIAN_POINT('Ctrl Pts',(-1.8,4.6,-20.97)) ;
#113061=CARTESIAN_POINT('Ctrl Pts',(-1.8,4.57374656717372,-20.9174931343473)) ;
#113062=CARTESIAN_POINT('Ctrl Pts',(-1.8,4.56045866731641,-20.930458667317)) ;
#113063=CARTESIAN_POINT('Ctrl Pts',(-1.8,4.54749313434728,-20.9437465671737)) ;
#113064=CARTESIAN_POINT('Ctrl Pts',(-1.78922263893876,4.54780128270145,
-20.8656025654029)) ;
#113065=CARTESIAN_POINT('Ctrl Pts',(-1.77362528614074,4.52085344889015,
-20.8908534488901)) ;
#113066=CARTESIAN_POINT('Ctrl Pts',(-1.78922263893874,4.49560256540291,
-20.9178012827014)) ;
#113067=CARTESIAN_POINT('Ctrl Pts',(-1.7614546977086,4.5200333414713,-20.8100666829426)) ;
#113068=CARTESIAN_POINT('Ctrl Pts',(-1.73208554016474,4.49711619685842,
-20.8671161968584)) ;
#113069=CARTESIAN_POINT('Ctrl Pts',(-1.76145469770861,4.44006668294258,
-20.8900333414713)) ;
#113070=CARTESIAN_POINT('Ctrl Pts',(-1.7503618540841,4.51262134295865,-20.7952426859173)) ;
#113071=CARTESIAN_POINT('Ctrl Pts',(-1.71792722356046,4.49498692411707,
-20.8649869241171)) ;
#113072=CARTESIAN_POINT('Ctrl Pts',(-1.75036185408411,4.42524268591729,
-20.8826213429587)) ;
#113073=CARTESIAN_POINT('Ctrl Pts',(-1.72617483238892,4.50260275053909,
-20.7752055010782)) ;
#113074=CARTESIAN_POINT('Ctrl Pts',(-1.70094059868422,4.4967032564359,-20.8667032564359)) ;
#113075=CARTESIAN_POINT('Ctrl Pts',(-1.72617483238891,4.4052055010782,-20.8726027505391)) ;
#113076=CARTESIAN_POINT('Ctrl Pts',(-1.71309229646328,4.5,-20.7700000008182)) ;
#113077=CARTESIAN_POINT('Ctrl Pts',(-1.69945650152272,4.49999269603968,
-20.8699926960963)) ;
#113078=CARTESIAN_POINT('Ctrl Pts',(-1.71309229646328,4.40000000081823,
-20.87)) ;
#113079=CARTESIAN_POINT('Ctrl Pts',(-1.7,4.5,-20.77)) ;
#113080=CARTESIAN_POINT('Ctrl Pts',(-1.7,4.5,-20.87)) ;
#113081=CARTESIAN_POINT('Ctrl Pts',(-1.7,4.4,-20.87)) ;
#113082=CARTESIAN_POINT('Ctrl Pts',(-1.8,4.6,-19.67)) ;
#113083=CARTESIAN_POINT('Ctrl Pts',(-1.8,4.6,-19.67)) ;
#113084=CARTESIAN_POINT('Ctrl Pts',(-1.8,4.6,-19.67)) ;
#113085=CARTESIAN_POINT('Ctrl Pts',(-1.8,4.54749313434728,-19.6962534328263)) ;
#113086=CARTESIAN_POINT('Ctrl Pts',(-1.8,4.5604586673143,-19.7095413326856)) ;
#113087=CARTESIAN_POINT('Ctrl Pts',(-1.8,4.57374656717372,-19.7225068656528)) ;
#113088=CARTESIAN_POINT('Ctrl Pts',(-1.78922263893874,4.49560256540291,
-19.7221987172986)) ;
#113089=CARTESIAN_POINT('Ctrl Pts',(-1.77362528614074,4.52085344889015,
-19.7491465511099)) ;
#113090=CARTESIAN_POINT('Ctrl Pts',(-1.78922263893876,4.54780128270145,
-19.7743974345971)) ;
#113091=CARTESIAN_POINT('Ctrl Pts',(-1.76145469770861,4.44006668294258,
-19.7499666585287)) ;
#113092=CARTESIAN_POINT('Ctrl Pts',(-1.73208554016474,4.49711619685842,
-19.7728838031416)) ;
#113093=CARTESIAN_POINT('Ctrl Pts',(-1.7614546977086,4.5200333414713,-19.8299333170574)) ;
#113094=CARTESIAN_POINT('Ctrl Pts',(-1.75036185408411,4.42524268591729,
-19.7573786570413)) ;
#113095=CARTESIAN_POINT('Ctrl Pts',(-1.71792722356045,4.49498692411707,
-19.7750130758829)) ;
#113096=CARTESIAN_POINT('Ctrl Pts',(-1.7503618540841,4.51262134295865,-19.8447573140827)) ;
#113097=CARTESIAN_POINT('Ctrl Pts',(-1.72617483238891,4.4052055010782,-19.7673972494609)) ;
#113098=CARTESIAN_POINT('Ctrl Pts',(-1.70094059868422,4.4967032564359,-19.7732967435641)) ;
#113099=CARTESIAN_POINT('Ctrl Pts',(-1.72617483238892,4.50260275053909,
-19.8647944989218)) ;
#113100=CARTESIAN_POINT('Ctrl Pts',(-1.71309229646329,4.40000000081823,
-19.77)) ;
#113101=CARTESIAN_POINT('Ctrl Pts',(-1.69945650152272,4.49999269603968,
-19.7700073039037)) ;
#113102=CARTESIAN_POINT('Ctrl Pts',(-1.71309229646328,4.5,-19.8699999991818)) ;
#113103=CARTESIAN_POINT('Ctrl Pts',(-1.7,4.4,-19.77)) ;
#113104=CARTESIAN_POINT('Ctrl Pts',(-1.7,4.5,-19.77)) ;
#113105=CARTESIAN_POINT('Ctrl Pts',(-1.7,4.5,-19.87)) ;
#113106=CARTESIAN_POINT('Origin',(-1.7,4.4,-19.87)) ;
#113107=CARTESIAN_POINT('Origin',(0.549999999999999,4.4,-19.87)) ;
#113108=CARTESIAN_POINT('Origin',(0.45,4.4,-19.87)) ;
#113109=CARTESIAN_POINT('Origin',(0.45,4.4,-19.87)) ;
#113110=CARTESIAN_POINT('Origin',(0.45,4.4,-19.87)) ;
#113111=CARTESIAN_POINT('Origin',(0.45,4.9047241136249E-17,-19.87)) ;
#113112=CARTESIAN_POINT('Origin',(0.45,0.3,-19.87)) ;
#113113=CARTESIAN_POINT('Ctrl Pts',(0.45,0.3,-19.77)) ;
#113114=CARTESIAN_POINT('Ctrl Pts',(0.55,0.3,-19.77)) ;
#113115=CARTESIAN_POINT('Ctrl Pts',(0.55,0.3,-19.87)) ;
#113116=CARTESIAN_POINT('Ctrl Pts',(0.450000000818259,0.286907703536713,
-19.77)) ;
#113117=CARTESIAN_POINT('Ctrl Pts',(0.549992696056738,0.300543498484345,
-19.7700073039038)) ;
#113118=CARTESIAN_POINT('Ctrl Pts',(0.55,0.28690770353672,-19.8699999991818)) ;
#113119=CARTESIAN_POINT('Ctrl Pts',(0.455205501078185,0.273825167611091,
-19.7673972494609)) ;
#113120=CARTESIAN_POINT('Ctrl Pts',(0.546703256435901,0.299059401315784,
-19.7732967435641)) ;
#113121=CARTESIAN_POINT('Ctrl Pts',(0.552602750539093,0.273825167611082,
-19.8647944989218)) ;
#113122=CARTESIAN_POINT('Ctrl Pts',(0.4752426859173,0.249638145915891,-19.7573786570413)) ;
#113123=CARTESIAN_POINT('Ctrl Pts',(0.544986924117067,0.282072776439541,
-19.7750130758829)) ;
#113124=CARTESIAN_POINT('Ctrl Pts',(0.56262134295865,0.249638145915901,
-19.8447573140827)) ;
#113125=CARTESIAN_POINT('Ctrl Pts',(0.490066682942577,0.238545302291388,
-19.7499666585287)) ;
#113126=CARTESIAN_POINT('Ctrl Pts',(0.54711619685839,0.267914459835252,
-19.7728838031416)) ;
#113127=CARTESIAN_POINT('Ctrl Pts',(0.570033341471288,0.238545302291403,
-19.8299333170574)) ;
#113128=CARTESIAN_POINT('Ctrl Pts',(0.545602565402917,0.21077736106126,
-19.7221987172986)) ;
#113129=CARTESIAN_POINT('Ctrl Pts',(0.570853448890191,0.22637471385927,
-19.7491465511099)) ;
#113130=CARTESIAN_POINT('Ctrl Pts',(0.597801282701459,0.210777361061231,
-19.7743974345971)) ;
#113131=CARTESIAN_POINT('Ctrl Pts',(0.597493134347346,0.2,-19.6962534328265)) ;
#113132=CARTESIAN_POINT('Ctrl Pts',(0.610458667316253,0.2,-19.7095413326839)) ;
#113133=CARTESIAN_POINT('Ctrl Pts',(0.623746567173686,0.2,-19.7225068656527)) ;
#113134=CARTESIAN_POINT('Ctrl Pts',(0.65,0.2,-19.67)) ;
#113135=CARTESIAN_POINT('Ctrl Pts',(0.65,0.2,-19.67)) ;
#113136=CARTESIAN_POINT('Ctrl Pts',(0.65,0.2,-19.67)) ;
#113137=CARTESIAN_POINT('Ctrl Pts',(8.5,8.17221734381475,-20.8602872911617)) ;
#113138=CARTESIAN_POINT('Ctrl Pts',(8.5,8.17221734381475,-20.945)) ;
#113139=CARTESIAN_POINT('Ctrl Pts',(8.58356010126947,8.17221734381475,-20.9589266835449)) ;
#113140=CARTESIAN_POINT('Ctrl Pts',(8.5,8.23335379241385,-20.8602872927391)) ;
#113141=CARTESIAN_POINT('Ctrl Pts',(8.5,8.2084742596066,-20.9374575674223)) ;
#113142=CARTESIAN_POINT('Ctrl Pts',(8.57460439031233,8.20580126077889,-20.9574340650521)) ;
#113143=CARTESIAN_POINT('Ctrl Pts',(8.5,8.29192178062155,-20.8871741150785)) ;
#113144=CARTESIAN_POINT('Ctrl Pts',(8.49999999999995,8.25010493984403,-20.9492546083116)) ;
#113145=CARTESIAN_POINT('Ctrl Pts',(8.56800970738924,8.23725302684489,-20.9697783631899)) ;
#113146=CARTESIAN_POINT('Ctrl Pts',(8.5,8.36583651094027,-20.9765506232914)) ;
#113147=CARTESIAN_POINT('Ctrl Pts',(8.50000000000005,8.29925403146166,-21.0033614370367)) ;
#113148=CARTESIAN_POINT('Ctrl Pts',(8.56373266208983,8.27563607377072,-21.0137537764131)) ;
#113149=CARTESIAN_POINT('Ctrl Pts',(8.5,8.38029241321759,-21.0379552056996)) ;
#113150=CARTESIAN_POINT('Ctrl Pts',(8.50000000000015,8.30669116589111,-21.044808849941)) ;
#113151=CARTESIAN_POINT('Ctrl Pts',(8.56610123859376,8.28208399509955,-21.044808702407)) ;
#113152=CARTESIAN_POINT('Ctrl Pts',(8.5,8.36719795478508,-21.0960547234799)) ;
#113153=CARTESIAN_POINT('Ctrl Pts',(8.5,8.29381262650623,-21.0795151496718)) ;
#113154=CARTESIAN_POINT('Ctrl Pts',(8.57227762885807,8.27346847343705,-21.0749299876354)) ;
#113155=CARTESIAN_POINT('Ctrl Pts',(8.5485213309235,8.28383177029354,-21.0759865327337)) ;
#113156=CARTESIAN_POINT('Ctrl Pts',(8.54913757890789,8.28625057716299,-21.062921659184)) ;
#113157=CARTESIAN_POINT('Ctrl Pts',(8.549146361399,8.28675781111762,-21.0492647894026)) ;
#113158=CARTESIAN_POINT('Ctrl Pts',(8.54883414737369,8.28489376483071,-21.036098869425)) ;
#113159=CARTESIAN_POINT('Ctrl Pts',(8.54852072231757,8.28302248819127,-21.0228818808428)) ;
#113160=CARTESIAN_POINT('Ctrl Pts',(8.54791723678494,8.27865742078997,-21.0098312958117)) ;
#113161=CARTESIAN_POINT('Ctrl Pts',(8.54677696932927,8.27237937104781,-20.9981020767297)) ;
#113162=CARTESIAN_POINT('Ctrl Pts',(8.5454465495755,8.26505438658866,-20.9844168797302)) ;
#113163=CARTESIAN_POINT('Ctrl Pts',(8.54324462275112,8.25487237915563,-20.9722537533388)) ;
#113164=CARTESIAN_POINT('Ctrl Pts',(8.53884071267076,8.24480815719263,-20.9612071681992)) ;
#113165=CARTESIAN_POINT('Ctrl Pts',(8.5342440055524,8.23430333763594,-20.9496769789768)) ;
#113166=CARTESIAN_POINT('Ctrl Pts',(8.52670159721618,8.22420330618022,-20.938704260243)) ;
#113167=CARTESIAN_POINT('Ctrl Pts',(8.51928858688475,8.21729138318396,-20.9259881754653)) ;
#113168=CARTESIAN_POINT('Ctrl Pts',(8.51327528614099,8.21168455548023,-20.915673116045)) ;
#113169=CARTESIAN_POINT('Ctrl Pts',(8.50759525524367,8.20778929846109,-20.9039849430828)) ;
#113170=CARTESIAN_POINT('Ctrl Pts',(8.50412058850191,8.20498026622232,-20.8915739486628)) ;
#113171=CARTESIAN_POINT('Ctrl Pts',(8.50147164778345,8.20283877743224,-20.8821123251694)) ;
#113172=CARTESIAN_POINT('Ctrl Pts',(8.50000317248551,8.2012555848359,-20.872083357655)) ;
#113173=CARTESIAN_POINT('Ctrl Pts',(8.50000000513446,8.20000405629318,-20.8621052387284)) ;
#113174=CARTESIAN_POINT('Origin',(8.6,8.17221734381475,-20.8602872911617)) ;
#113175=CARTESIAN_POINT('Origin',(8.6,4.35421736843756,-20.8602872911617)) ;
#113176=CARTESIAN_POINT('Origin',(8.6,6.66256607592813,-20.8602872911617)) ;
#113177=CARTESIAN_POINT('Ctrl Pts',(8.5,6.47083593368087,-21.1048081099244)) ;
#113178=CARTESIAN_POINT('Ctrl Pts',(8.5,6.55684090505321,-21.0843877386952)) ;
#113179=CARTESIAN_POINT('Ctrl Pts',(8.58772778625753,6.56739561896918,-21.081881707091)) ;
#113180=CARTESIAN_POINT('Ctrl Pts',(8.5,6.45680686388577,-21.0457215297177)) ;
#113181=CARTESIAN_POINT('Ctrl Pts',(8.50000000000015,6.54406229478603,-21.0525101654037)) ;
#113182=CARTESIAN_POINT('Ctrl Pts',(8.58195196310359,6.55941415012443,-21.0513576868779)) ;
#113183=CARTESIAN_POINT('Ctrl Pts',(8.5,6.47061556584392,-20.9819524568048)) ;
#113184=CARTESIAN_POINT('Ctrl Pts',(8.5,6.54836369988892,-21.0123987274072)) ;
#113185=CARTESIAN_POINT('Ctrl Pts',(8.57801125828727,6.5656660137223,-21.0188344592028)) ;
#113186=CARTESIAN_POINT('Ctrl Pts',(8.5,6.54379299301794,-20.8886264716581)) ;
#113187=CARTESIAN_POINT('Ctrl Pts',(8.5,6.5907178951622,-20.9562265152921)) ;
#113188=CARTESIAN_POINT('Ctrl Pts',(8.57642058265785,6.60198961470446,-20.9719063540245)) ;
#113189=CARTESIAN_POINT('Ctrl Pts',(8.5,6.60220518075382,-20.8602872929745)) ;
#113190=CARTESIAN_POINT('Ctrl Pts',(8.5,6.62800697860328,-20.9409176707628)) ;
#113191=CARTESIAN_POINT('Ctrl Pts',(8.57879135173924,6.63156920211803,-20.9581318919565)) ;
#113192=CARTESIAN_POINT('Ctrl Pts',(8.5,6.66256607592813,-20.8602872911617)) ;
#113193=CARTESIAN_POINT('Ctrl Pts',(8.5,6.66256607592813,-20.945)) ;
#113194=CARTESIAN_POINT('Ctrl Pts',(8.58356010126947,6.66256607592813,-20.9589266835449)) ;
#113195=CARTESIAN_POINT('',(8.54565366748552,6.61650711946997,-20.9539653182917)) ;
#113196=CARTESIAN_POINT('Ctrl Pts',(8.54565366716102,6.61650712004131,-20.9539653178135)) ;
#113197=CARTESIAN_POINT('Ctrl Pts',(8.54527684775567,6.61717057264361,-20.9534100008637)) ;
#113198=CARTESIAN_POINT('Ctrl Pts',(8.54488909344006,6.61782772231432,-20.9528554298997)) ;
#113199=CARTESIAN_POINT('Ctrl Pts',(8.54449064961563,6.61847724592616,-20.9523008713851)) ;
#113200=CARTESIAN_POINT('Ctrl Pts',(8.54445329550709,6.61853813876477,-20.9522488815244)) ;
#113201=CARTESIAN_POINT('Ctrl Pts',(8.54441584757976,6.61859896452229,-20.9521968917916)) ;
#113202=CARTESIAN_POINT('Ctrl Pts',(8.54437830610599,6.61865972207467,-20.9521449015859)) ;
#113203=CARTESIAN_POINT('Ctrl Pts',(8.54363538409152,6.61986207559656,-20.9511160483068)) ;
#113204=CARTESIAN_POINT('Ctrl Pts',(8.54285495000596,6.62104203503525,-20.9500848621747)) ;
#113205=CARTESIAN_POINT('Ctrl Pts',(8.54204093171159,6.62218056960115,-20.9490511151673)) ;
#113206=CARTESIAN_POINT('Ctrl Pts',(8.54157979215443,6.62282554690592,-20.9484654997818)) ;
#113207=CARTESIAN_POINT('Ctrl Pts',(8.54110770812191,6.62345780120142,-20.9478786499067)) ;
#113208=CARTESIAN_POINT('Ctrl Pts',(8.54062344907117,6.62407892448169,-20.9472869541396)) ;
#113209=CARTESIAN_POINT('Ctrl Pts',(8.54011932596481,6.62472552591744,-20.9466709873185)) ;
#113210=CARTESIAN_POINT('Ctrl Pts',(8.53960207832256,6.62535666566135,-20.946050990589)) ;
#113211=CARTESIAN_POINT('Ctrl Pts',(8.53907286520408,6.62597244099096,-20.9454252288111)) ;
#113212=CARTESIAN_POINT('Ctrl Pts',(8.53887441028465,6.62620335673957,-20.9451905681443)) ;
#113213=CARTESIAN_POINT('Ctrl Pts',(8.53867427664143,6.6264321129994,-20.9449550998211)) ;
#113214=CARTESIAN_POINT('Ctrl Pts',(8.53847256319998,6.62665871795109,-20.9447187642184)) ;
#113215=CARTESIAN_POINT('Ctrl Pts',(8.53842843838466,6.62670828778427,-20.9446670658053)) ;
#113216=CARTESIAN_POINT('Ctrl Pts',(8.53838423811749,6.62675775467668,-20.9446153260174)) ;
#113217=CARTESIAN_POINT('Ctrl Pts',(8.53833996369345,6.62680711871687,-20.9445635444601)) ;
#113218=CARTESIAN_POINT('Ctrl Pts',(8.53829707284515,6.62685494013081,-20.9445133810765)) ;
#113219=CARTESIAN_POINT('Ctrl Pts',(8.53825411240225,6.62690266502018,-20.9444631784931)) ;
#113220=CARTESIAN_POINT('Ctrl Pts',(8.53821108363806,6.62695029346532,-20.9444129364377)) ;
#113221=CARTESIAN_POINT('Ctrl Pts',(8.53803571435332,6.62714440934376,-20.9442081684534)) ;
#113222=CARTESIAN_POINT('Ctrl Pts',(8.53785876035507,6.62733753498028,-20.9440021836648)) ;
#113223=CARTESIAN_POINT('Ctrl Pts',(8.53767995296704,6.62753033615257,-20.9437944665652)) ;
#113224=CARTESIAN_POINT('Ctrl Pts',(8.53649871780654,6.62880401687797,-20.942422248425)) ;
#113225=CARTESIAN_POINT('Ctrl Pts',(8.53528300832265,6.62998038079526,-20.9410380760596)) ;
#113226=CARTESIAN_POINT('Ctrl Pts',(8.53403203676338,6.63110281535143,-20.9396044865649)) ;
#113227=CARTESIAN_POINT('Ctrl Pts',(8.53346870389682,6.63160826591214,-20.9389589178679)) ;
#113228=CARTESIAN_POINT('Ctrl Pts',(8.53289959536922,6.63209979040222,-20.9383054256595)) ;
#113229=CARTESIAN_POINT('Ctrl Pts',(8.53232661340321,6.6325773534403,-20.9376437014439)) ;
#113230=CARTESIAN_POINT('Ctrl Pts',(8.53206474273906,6.63279561467254,-20.9373412727985)) ;
#113231=CARTESIAN_POINT('Ctrl Pts',(8.53180206199566,6.63301096017661,-20.9370371260807)) ;
#113232=CARTESIAN_POINT('Ctrl Pts',(8.53153874718658,6.63322338883723,-20.9367312388807)) ;
#113233=CARTESIAN_POINT('Ctrl Pts',(8.5300736365822,6.63440536369243,-20.9350292511271)) ;
#113234=CARTESIAN_POINT('Ctrl Pts',(8.52858926277509,6.63549697414122,-20.9332730839131)) ;
#113235=CARTESIAN_POINT('Ctrl Pts',(8.52711342564668,6.63649856635108,-20.9314611393064)) ;
#113236=CARTESIAN_POINT('Ctrl Pts',(8.5263431695412,6.63702130866457,-20.9305154649028)) ;
#113237=CARTESIAN_POINT('Ctrl Pts',(8.52557615349971,6.63751985710294,-20.9295557193112)) ;
#113238=CARTESIAN_POINT('Ctrl Pts',(8.52481401823433,6.63799287689813,-20.9285803261613)) ;
#113239=CARTESIAN_POINT('Ctrl Pts',(8.52460710835824,6.63812129566006,-20.9283155195253)) ;
#113240=CARTESIAN_POINT('Ctrl Pts',(8.52440075574007,6.63824801482191,-20.9280497539023)) ;
#113241=CARTESIAN_POINT('Ctrl Pts',(8.52419502810874,6.63837284070829,-20.9277830860811)) ;
#113242=CARTESIAN_POINT('Ctrl Pts',(8.52404824365687,6.63846190263541,-20.9275928214593)) ;
#113243=CARTESIAN_POINT('Ctrl Pts',(8.52390173612806,6.63855002749204,-20.9274020437347)) ;
#113244=CARTESIAN_POINT('Ctrl Pts',(8.52375553261477,6.63863721305423,-20.9272107628049)) ;
#113245=CARTESIAN_POINT('Ctrl Pts',(8.52294204127161,6.63912232246438,-20.9261464560924)) ;
#113246=CARTESIAN_POINT('Ctrl Pts',(8.52213801365707,6.63957834748689,-20.9250665375564)) ;
#113247=CARTESIAN_POINT('Ctrl Pts',(8.52134774490512,6.64000494097979,-20.9239729614464)) ;
#113248=CARTESIAN_POINT('Ctrl Pts',(8.51876608595599,6.64139854145543,-20.9204004545695)) ;
#113249=CARTESIAN_POINT('Ctrl Pts',(8.51630176076719,6.64256282842068,-20.9166245667844)) ;
#113250=CARTESIAN_POINT('Ctrl Pts',(8.51404737801022,6.64354662431173,-20.9126687582286)) ;
#113251=CARTESIAN_POINT('Ctrl Pts',(8.51174271377019,6.64455236266853,-20.9086247197926)) ;
#113252=CARTESIAN_POINT('Ctrl Pts',(8.50965863261302,6.64536892721963,-20.9043937780696)) ;
#113253=CARTESIAN_POINT('Ctrl Pts',(8.50786496313903,6.64606338785379,-20.9000441654859)) ;
#113254=CARTESIAN_POINT('Ctrl Pts',(8.50767015284864,6.64613881316473,-20.8995717544299)) ;
#113255=CARTESIAN_POINT('Ctrl Pts',(8.50747873128293,6.64621281334902,-20.8990979736875)) ;
#113256=CARTESIAN_POINT('Ctrl Pts',(8.50729076020856,6.64628549377757,-20.8986229301938)) ;
#113257=CARTESIAN_POINT('Ctrl Pts',(8.50722027105568,6.64631274893828,-20.8984447888837)) ;
#113258=CARTESIAN_POINT('Ctrl Pts',(8.50715026706477,6.64633981850992,-20.8982664700192)) ;
#113259=CARTESIAN_POINT('Ctrl Pts',(8.50708075128541,6.64636670806329,-20.8980879793594)) ;
#113260=CARTESIAN_POINT('Ctrl Pts',(8.50659414082988,6.6465549349369,-20.896838544741)) ;
#113261=CARTESIAN_POINT('Ctrl Pts',(8.50613147592892,6.64673434010345,-20.895580683755)) ;
#113262=CARTESIAN_POINT('Ctrl Pts',(8.50569363751095,6.64690683932497,-20.8943164275023)) ;
#113263=CARTESIAN_POINT('Ctrl Pts',(8.50395436040173,6.64759207829676,-20.8892942735061)) ;
#113264=CARTESIAN_POINT('Ctrl Pts',(8.50258205288248,6.64816393978949,-20.8840915596128)) ;
#113265=CARTESIAN_POINT('Ctrl Pts',(8.50162662717083,6.64864720987532,-20.8788041247401)) ;
#113266=CARTESIAN_POINT('Ctrl Pts',(8.50156399248179,6.64867889153427,-20.8784574972263)) ;
#113267=CARTESIAN_POINT('Ctrl Pts',(8.50150313499559,6.64871019935933,-20.8781105075148)) ;
#113268=CARTESIAN_POINT('Ctrl Pts',(8.50144406283924,6.64874114271687,-20.8777631835019)) ;
#113269=CARTESIAN_POINT('Ctrl Pts',(8.50057491246564,6.64919642372279,-20.8726528774933)) ;
#113270=CARTESIAN_POINT('Ctrl Pts',(8.50009537300571,6.64957062705854,-20.8674713290504)) ;
#113271=CARTESIAN_POINT('Ctrl Pts',(8.50001293997568,6.64989933182553,-20.8623144435395)) ;
#113272=CARTESIAN_POINT('Ctrl Pts',(8.50000430878269,6.64993374902796,-20.861774489178)) ;
#113273=CARTESIAN_POINT('Ctrl Pts',(8.5,6.64996765698299,-20.8612348144278)) ;
#113274=CARTESIAN_POINT('Ctrl Pts',(8.5,6.65000108682384,-20.8606955361059)) ;
#113275=CARTESIAN_POINT('',(8.55245136877619,6.60097994372616,-20.9667801193795)) ;
#113276=CARTESIAN_POINT('Ctrl Pts',(8.55238056475491,6.60105295171781,-20.9668886154986)) ;
#113277=CARTESIAN_POINT('Ctrl Pts',(8.55170523171908,6.60308542368566,-20.9651022656148)) ;
#113278=CARTESIAN_POINT('Ctrl Pts',(8.5509582952036,6.60513808680132,-20.9633627348221)) ;
#113279=CARTESIAN_POINT('Ctrl Pts',(8.55012599030524,6.60719152980376,-20.9616544441814)) ;
#113280=CARTESIAN_POINT('Ctrl Pts',(8.5496832294788,6.60828389886539,-20.9607456856515)) ;
#113281=CARTESIAN_POINT('Ctrl Pts',(8.54921644930866,6.60937569995271,-20.9598462491234)) ;
#113282=CARTESIAN_POINT('Ctrl Pts',(8.54872481267393,6.61045954913299,-20.9589557465494)) ;
#113283=CARTESIAN_POINT('Ctrl Pts',(8.54779539897816,6.61250851009546,-20.9572722973719)) ;
#113284=CARTESIAN_POINT('Ctrl Pts',(8.54677348694554,6.61453549290064,-20.9556155908862)) ;
#113285=CARTESIAN_POINT('Ctrl Pts',(8.54565366748551,6.61650711946996,-20.9539653182917)) ;
#113286=CARTESIAN_POINT('',(8.55735473176745,6.58264207262453,-20.9849557973616)) ;
#113287=CARTESIAN_POINT('Ctrl Pts',(8.557354731687,6.58264207302788,-20.9849557968441)) ;
#113288=CARTESIAN_POINT('Ctrl Pts',(8.55706916598053,6.58397660851271,-20.9832296933714)) ;
#113289=CARTESIAN_POINT('Ctrl Pts',(8.55678088122702,6.58528501693261,-20.9816621009603)) ;
#113290=CARTESIAN_POINT('Ctrl Pts',(8.55647408091819,6.58661569125895,-20.9801718232515)) ;
#113291=CARTESIAN_POINT('Ctrl Pts',(8.55614409617576,6.58804692262413,-20.9785689275185)) ;
#113292=CARTESIAN_POINT('Ctrl Pts',(8.55579261555185,6.58950524590121,-20.9770567950172)) ;
#113293=CARTESIAN_POINT('Ctrl Pts',(8.55539993844501,6.59102291080546,-20.9755875677792)) ;
#113294=CARTESIAN_POINT('Ctrl Pts',(8.55517214917304,6.59190329771267,-20.974735279227)) ;
#113295=CARTESIAN_POINT('Ctrl Pts',(8.55493049881961,6.59280308289159,-20.9738983977538)) ;
#113296=CARTESIAN_POINT('Ctrl Pts',(8.55467134659048,6.59372113732148,-20.9730707946419)) ;
#113297=CARTESIAN_POINT('Ctrl Pts',(8.5543480523717,6.59486641664517,-20.9720383539702)) ;
#113298=CARTESIAN_POINT('Ctrl Pts',(8.55400737519029,6.59602723165037,-20.9710361981957)) ;
#113299=CARTESIAN_POINT('Ctrl Pts',(8.55365328858766,6.59718920061514,-20.9700452155133)) ;
#113300=CARTESIAN_POINT('Ctrl Pts',(8.55328167888691,6.59840867329803,-20.969005190911)) ;
#113301=CARTESIAN_POINT('Ctrl Pts',(8.55289390107695,6.59963546460028,-20.9679736796763)) ;
#113302=CARTESIAN_POINT('Ctrl Pts',(8.55249886556662,6.60083562835459,-20.9669081494348)) ;
#113303=CARTESIAN_POINT('Ctrl Pts',(8.55248304763317,6.60088368507325,-20.9668654836845)) ;
#113304=CARTESIAN_POINT('Ctrl Pts',(8.5524672152281,6.60093179017222,-20.966822806733)) ;
#113305=CARTESIAN_POINT('Ctrl Pts',(8.55245136877619,6.60097994372615,-20.9667801193796)) ;
#113306=CARTESIAN_POINT('Ctrl Pts',(8.56107669735261,6.56009388000089,-21.0823838472224)) ;
#113307=CARTESIAN_POINT('Ctrl Pts',(8.56115635543005,6.55978170524809,-21.0808207343832)) ;
#113308=CARTESIAN_POINT('Ctrl Pts',(8.56122592915387,6.55950119162287,-21.0792507129806)) ;
#113309=CARTESIAN_POINT('Ctrl Pts',(8.56128584055879,6.55925348717442,-21.0776933919486)) ;
#113310=CARTESIAN_POINT('Ctrl Pts',(8.56142626445294,6.55867290283844,-21.074043250811)) ;
#113311=CARTESIAN_POINT('Ctrl Pts',(8.56152217534693,6.55825854507369,-21.0703756338773)) ;
#113312=CARTESIAN_POINT('Ctrl Pts',(8.56158081746989,6.55798577878937,-21.0666701354258)) ;
#113313=CARTESIAN_POINT('Ctrl Pts',(8.56158917845351,6.55794688875062,-21.0661418187435)) ;
#113314=CARTESIAN_POINT('Ctrl Pts',(8.56159677639836,6.55791088241229,-21.0656126452596)) ;
#113315=CARTESIAN_POINT('Ctrl Pts',(8.56160362608008,6.55787769947531,-21.0650824674717)) ;
#113316=CARTESIAN_POINT('Ctrl Pts',(8.56164117305277,6.55769580506315,-21.0621762636859)) ;
#113317=CARTESIAN_POINT('Ctrl Pts',(8.56164095204358,6.55766773657216,-21.0592640119965)) ;
#113318=CARTESIAN_POINT('Ctrl Pts',(8.56161306230089,6.55774920537473,-21.0563655672582)) ;
#113319=CARTESIAN_POINT('Ctrl Pts',(8.56157759693122,6.55785280336173,-21.0526798246077)) ;
#113320=CARTESIAN_POINT('Ctrl Pts',(8.56150275624659,6.55813669070955,-21.0490049280206)) ;
#113321=CARTESIAN_POINT('Ctrl Pts',(8.56141108129143,6.55856506509346,-21.0453632925476)) ;
#113322=CARTESIAN_POINT('Ctrl Pts',(8.56136615997218,6.5587749713042,-21.0435788676806)) ;
#113323=CARTESIAN_POINT('Ctrl Pts',(8.56131707129296,6.55902016312288,-21.0418016709682)) ;
#113324=CARTESIAN_POINT('Ctrl Pts',(8.56126585691691,6.55929956116447,-21.0400315254682)) ;
#113325=CARTESIAN_POINT('Ctrl Pts',(8.56116752027492,6.55983603289969,-21.0366326719095)) ;
#113326=CARTESIAN_POINT('Ctrl Pts',(8.56104954130216,6.56049109659205,-21.0332540075755)) ;
#113327=CARTESIAN_POINT('Ctrl Pts',(8.56091150449775,6.56129147625804,-21.0298304710248)) ;
#113328=CARTESIAN_POINT('Ctrl Pts',(8.56080235670743,6.56192434857304,-21.0271234288616)) ;
#113329=CARTESIAN_POINT('Ctrl Pts',(8.56068045333715,6.56264902401852,-21.0243872666894)) ;
#113330=CARTESIAN_POINT('Ctrl Pts',(8.56054379825319,6.56349285586897,-21.0216234877213)) ;
#113331=CARTESIAN_POINT('Ctrl Pts',(8.56050762866484,6.56371619955867,-21.0208919763521)) ;
#113332=CARTESIAN_POINT('Ctrl Pts',(8.56047042218818,6.56394794674722,-21.0201587916983)) ;
#113333=CARTESIAN_POINT('Ctrl Pts',(8.5604321390176,6.56418871538696,-21.0194246234709)) ;
#113334=CARTESIAN_POINT('Ctrl Pts',(8.56026887460239,6.56521550994376,-21.0162936511792)) ;
#113335=CARTESIAN_POINT('Ctrl Pts',(8.56008532870544,6.56636514336274,-21.0132612149346)) ;
#113336=CARTESIAN_POINT('Ctrl Pts',(8.5598891591871,6.56762686151826,-21.0104713276669)) ;
#113337=CARTESIAN_POINT('Ctrl Pts',(8.55964574654527,6.56919243680269,-21.0070095572757)) ;
#113338=CARTESIAN_POINT('Ctrl Pts',(8.55938661160132,6.57080906160864,-21.003732634051)) ;
#113339=CARTESIAN_POINT('Ctrl Pts',(8.55911582090257,6.57246439798288,-21.000667212428)) ;
#113340=CARTESIAN_POINT('Ctrl Pts',(8.55888928658553,6.57384919626708,-20.9981027846356)) ;
#113341=CARTESIAN_POINT('Ctrl Pts',(8.55863813502894,6.57544444689303,-20.9953653454317)) ;
#113342=CARTESIAN_POINT('Ctrl Pts',(8.55834707044214,6.57718152485352,-20.9926681258236)) ;
#113343=CARTESIAN_POINT('Ctrl Pts',(8.55828762047116,6.57753632320078,-20.9921172184488)) ;
#113344=CARTESIAN_POINT('Ctrl Pts',(8.55822651695173,6.57789694345767,-20.9915678465794)) ;
#113345=CARTESIAN_POINT('Ctrl Pts',(8.55816364958867,6.57826264684155,-20.9910215710793)) ;
#113346=CARTESIAN_POINT('Ctrl Pts',(8.55792499569721,6.57965091145837,-20.9889478277641)) ;
#113347=CARTESIAN_POINT('Ctrl Pts',(8.5576603261423,6.58110993502786,-20.9869213132877)) ;
#113348=CARTESIAN_POINT('Ctrl Pts',(8.55735473176745,6.58264207262453,-20.9849557973616)) ;
#113349=CARTESIAN_POINT('Origin',(8.49172374697018,6.65,-22.86)) ;
#113350=CARTESIAN_POINT('Origin',(8.49226931262625,6.63793757533841,-21.0929882716362)) ;
#113351=CARTESIAN_POINT('Ctrl Pts',(8.40188506081761,6.5500005341705,-20.8315458308153)) ;
#113352=CARTESIAN_POINT('Ctrl Pts',(8.50280744587441,6.54966497091121,-20.8451950407541)) ;
#113353=CARTESIAN_POINT('Ctrl Pts',(8.50109204799972,6.65199687180765,-20.8456804549399)) ;
#113354=CARTESIAN_POINT('Ctrl Pts',(8.3929693293079,6.55000052027914,-20.889675802422)) ;
#113355=CARTESIAN_POINT('Ctrl Pts',(8.49725036372775,6.54968051003366,-20.8769136026832)) ;
#113356=CARTESIAN_POINT('Ctrl Pts',(8.49665296516362,6.64935672317805,-20.8760247114635)) ;
#113357=CARTESIAN_POINT('Ctrl Pts',(8.41146079558545,6.55000052635931,-20.949608884646)) ;
#113358=CARTESIAN_POINT('Ctrl Pts',(8.50278789772743,6.54967384197881,-20.9010143519806)) ;
#113359=CARTESIAN_POINT('Ctrl Pts',(8.50590954255545,6.65051247736748,-20.9044272120935)) ;
#113360=CARTESIAN_POINT('Ctrl Pts',(8.45744515914171,6.55000045243509,-21.0028021918823)) ;
#113361=CARTESIAN_POINT('Ctrl Pts',(8.5202381168081,6.54973725194854,-20.941633015821)) ;
#113362=CARTESIAN_POINT('Ctrl Pts',(8.52891723073132,6.63643009777379,-20.9334751630783)) ;
#113363=CARTESIAN_POINT('Ctrl Pts',(8.46608867121678,6.55000043643008,-21.0111950991748)) ;
#113364=CARTESIAN_POINT('Ctrl Pts',(8.52334270167615,6.54974993059823,-20.948470240079)) ;
#113365=CARTESIAN_POINT('Ctrl Pts',(8.53324349789231,6.63337968978884,-20.9382208913)) ;
#113366=CARTESIAN_POINT('Ctrl Pts',(8.48465388181683,6.55000038323734,-21.0265763138745)) ;
#113367=CARTESIAN_POINT('Ctrl Pts',(8.53001210036428,6.54978938646811,-20.9651245951232)) ;
#113368=CARTESIAN_POINT('Ctrl Pts',(8.54253954944034,6.62323710347997,-20.948863146269)) ;
#113369=CARTESIAN_POINT('Ctrl Pts',(8.49467048074911,6.55000035131511,-21.0334884944614)) ;
#113370=CARTESIAN_POINT('Ctrl Pts',(8.53347884787438,6.54981166882491,-20.97305903115)) ;
#113371=CARTESIAN_POINT('Ctrl Pts',(8.5475533753473,6.6171479354886,-20.9528676881263)) ;
#113372=CARTESIAN_POINT('Ctrl Pts',(8.50997930894002,6.55000022766094,-21.0433889027859)) ;
#113373=CARTESIAN_POINT('Ctrl Pts',(8.53869035159218,6.54988741100163,-20.9987742327549)) ;
#113374=CARTESIAN_POINT('Ctrl Pts',(8.55523846583762,6.59353839814627,-20.9735278831083)) ;
#113375=CARTESIAN_POINT('Ctrl Pts',(8.51532901080101,6.55000016113069,-21.0463389673193)) ;
#113376=CARTESIAN_POINT('Ctrl Pts',(8.54023459682686,6.54992340374042,-21.0084897483873)) ;
#113377=CARTESIAN_POINT('Ctrl Pts',(8.55790835982309,6.58082417519535,-20.9815823085729)) ;
#113378=CARTESIAN_POINT('Ctrl Pts',(8.52186010906342,6.55000005932357,-21.0527927598773)) ;
#113379=CARTESIAN_POINT('Ctrl Pts',(8.54265823247976,6.5499732773141,-21.0379316441152)) ;
#113380=CARTESIAN_POINT('Ctrl Pts',(8.56121746518602,6.56135337205753,-21.0245883700754)) ;
#113381=CARTESIAN_POINT('Ctrl Pts',(8.52354993939967,6.55000003603139,-21.0558242622279)) ;
#113382=CARTESIAN_POINT('Ctrl Pts',(8.54350769968238,6.54998394755847,-21.0514238732007)) ;
#113383=CARTESIAN_POINT('Ctrl Pts',(8.5621431061544,6.55689632415131,-21.0474501335625)) ;
#113384=CARTESIAN_POINT('Ctrl Pts',(8.52268461318107,6.55000004733862,-21.0617875304157)) ;
#113385=CARTESIAN_POINT('Ctrl Pts',(8.54305517585922,6.54997881410036,-21.07281341214)) ;
#113386=CARTESIAN_POINT('Ctrl Pts',(8.56153259171391,6.55906016573919,-21.0827901815805)) ;
#113387=CARTESIAN_POINT('Ctrl Pts',(8.52060566253923,6.55000006807331,-21.0644138065496)) ;
#113388=CARTESIAN_POINT('Ctrl Pts',(8.54195943530536,6.54996919659462,-21.0804945748859)) ;
#113389=CARTESIAN_POINT('Ctrl Pts',(8.560584416286,6.56302742363386,-21.0945079215137)) ;
#113390=CARTESIAN_POINT('Ctrl Pts',(8.51445291480382,6.55000012130567,-21.0712328149552)) ;
#113391=CARTESIAN_POINT('Ctrl Pts',(8.53868948987836,6.54994355920607,-21.0994191817675)) ;
#113392=CARTESIAN_POINT('Ctrl Pts',(8.55750149922674,6.57320954252655,-21.1211844353069)) ;
#113393=CARTESIAN_POINT('Ctrl Pts',(8.50953280296012,6.55000015625149,-21.0750479464372)) ;
#113394=CARTESIAN_POINT('Ctrl Pts',(8.53616288920967,6.54992588038503,-21.1077647485266)) ;
#113395=CARTESIAN_POINT('Ctrl Pts',(8.55504783006516,6.57989127253965,-21.1306993167928)) ;
#113396=CARTESIAN_POINT('Ctrl Pts',(8.49261655785707,6.55000026291039,-21.0884926065688)) ;
#113397=CARTESIAN_POINT('Ctrl Pts',(8.52778251455086,6.54986718408743,-21.1357691608947)) ;
#113398=CARTESIAN_POINT('Ctrl Pts',(8.54658667616929,6.60027178071327,-21.1593533757438)) ;
#113399=CARTESIAN_POINT('Ctrl Pts',(8.48022165824516,6.55000031608561,-21.0977685341604)) ;
#113400=CARTESIAN_POINT('Ctrl Pts',(8.52288681814163,6.54983437262026,-21.1474559489292)) ;
#113401=CARTESIAN_POINT('Ctrl Pts',(8.5404533945046,6.61042388759305,-21.1663019909607)) ;
#113402=CARTESIAN_POINT('Ctrl Pts',(8.46952991654743,6.55000035836673,-21.1090954462182)) ;
#113403=CARTESIAN_POINT('Ctrl Pts',(8.51900842894227,6.54980714069579,-21.1633676846765)) ;
#113404=CARTESIAN_POINT('Ctrl Pts',(8.53471369258705,6.61849392543623,-21.1813833684422)) ;
#113405=CARTESIAN_POINT('Origin',(8.4,6.65,-20.8606780018997)) ;
#113406=CARTESIAN_POINT('Ctrl Pts',(8.54848814460235,8.28374914930622,-19.5635371747799)) ;
#113407=CARTESIAN_POINT('Ctrl Pts',(8.55964225199693,8.27720012980425,-19.5649679483223)) ;
#113408=CARTESIAN_POINT('Ctrl Pts',(8.572140519951,8.27365818248462,-19.5657417625569)) ;
#113409=CARTESIAN_POINT('Ctrl Pts',(8.54519582228988,8.29111303851998,-19.5879603788076)) ;
#113410=CARTESIAN_POINT('Ctrl Pts',(8.5556995989114,8.28406912459882,-19.5880376174409)) ;
#113411=CARTESIAN_POINT('Ctrl Pts',(8.56757951573632,8.2799170974937,-19.5881916339118)) ;
#113412=CARTESIAN_POINT('Ctrl Pts',(8.54340782920287,8.28927570119136,-19.6138229931233)) ;
#113413=CARTESIAN_POINT('Ctrl Pts',(8.5535505383751,8.28232618564301,-19.6121546442898)) ;
#113414=CARTESIAN_POINT('Ctrl Pts',(8.56507848568419,8.27803412520748,-19.6111321430533)) ;
#113415=CARTESIAN_POINT('Ctrl Pts',(8.54340835145922,8.27841951799441,-19.6355350111617)) ;
#113416=CARTESIAN_POINT('Ctrl Pts',(8.55355093564017,8.27219257320284,-19.6324215387659)) ;
#113417=CARTESIAN_POINT('Ctrl Pts',(8.56507848521152,8.26835005667905,-19.630500280504)) ;
#113418=CARTESIAN_POINT('Ctrl Pts',(8.54742026180265,8.27608084857563,-19.6343656412486)) ;
#113419=CARTESIAN_POINT('Ctrl Pts',(8.54754672558908,8.27683897030432,-19.6326745730365)) ;
#113420=CARTESIAN_POINT('Ctrl Pts',(8.54766225486891,8.27755642830994,-19.6309654973084)) ;
#113421=CARTESIAN_POINT('Ctrl Pts',(8.54776713596767,8.27823455672261,-19.6292350167776)) ;
#113422=CARTESIAN_POINT('Ctrl Pts',(8.54791712013337,8.27920430747289,-19.626760360412)) ;
#113423=CARTESIAN_POINT('Ctrl Pts',(8.54806168001141,8.28008011045343,-19.6242463372678)) ;
#113424=CARTESIAN_POINT('Ctrl Pts',(8.54818998754191,8.28086237513948,-19.6217186838591)) ;
#113425=CARTESIAN_POINT('Ctrl Pts',(8.54824194926749,8.28117917511831,-19.6206950398668)) ;
#113426=CARTESIAN_POINT('Ctrl Pts',(8.54829140719363,8.2814807826497,-19.6196686742903)) ;
#113427=CARTESIAN_POINT('Ctrl Pts',(8.54833813644416,8.28176759858577,-19.6186396299771)) ;
#113428=CARTESIAN_POINT('Ctrl Pts',(8.54850061324771,8.28276485268192,-19.615061660529)) ;
#113429=CARTESIAN_POINT('Ctrl Pts',(8.54863339756395,8.28360845633779,-19.6113501235291)) ;
#113430=CARTESIAN_POINT('Ctrl Pts',(8.54873421749656,8.28426438239338,-19.6076130867581)) ;
#113431=CARTESIAN_POINT('Ctrl Pts',(8.54878752953696,8.28461122607273,-19.6056369987943)) ;
#113432=CARTESIAN_POINT('Ctrl Pts',(8.54883168679926,8.28490640714041,-19.6036540820739)) ;
#113433=CARTESIAN_POINT('Ctrl Pts',(8.54886500248133,8.28515040605088,-19.6016818590293)) ;
#113434=CARTESIAN_POINT('Ctrl Pts',(8.54887385422351,8.2852152348436,-19.6011578532512)) ;
#113435=CARTESIAN_POINT('Ctrl Pts',(8.54888411330031,8.28527512151702,-19.6006350091921)) ;
#113436=CARTESIAN_POINT('Ctrl Pts',(8.54889386083024,8.28533143086091,-19.6001120867861)) ;
#113437=CARTESIAN_POINT('Ctrl Pts',(8.54894969070932,8.28565394783545,-19.5971170003468)) ;
#113438=CARTESIAN_POINT('Ctrl Pts',(8.54897935138211,8.28586680424121,-19.5940986363827)) ;
#113439=CARTESIAN_POINT('Ctrl Pts',(8.54899968230029,8.28595875954339,-19.5910675778011)) ;
#113440=CARTESIAN_POINT('Ctrl Pts',(8.54900356561227,8.28597632348831,-19.5904886297173)) ;
#113441=CARTESIAN_POINT('Ctrl Pts',(8.54900713937599,8.28598945835117,-19.5899093088041)) ;
#113442=CARTESIAN_POINT('Ctrl Pts',(8.5490105728891,8.2859980637762,-19.5893298402186)) ;
#113443=CARTESIAN_POINT('Ctrl Pts',(8.54902784271198,8.28604134718936,-19.5864152394759)) ;
#113444=CARTESIAN_POINT('Ctrl Pts',(8.54901619593281,8.28598556136224,-19.5835157757217)) ;
#113445=CARTESIAN_POINT('Ctrl Pts',(8.54898431260111,8.28582669412323,-19.5806064286754)) ;
#113446=CARTESIAN_POINT('Ctrl Pts',(8.54893914418924,8.28560163041434,-19.5764848209685)) ;
#113447=CARTESIAN_POINT('Ctrl Pts',(8.54884805310399,8.2851729064642,-19.5723770999644)) ;
#113448=CARTESIAN_POINT('Ctrl Pts',(8.54869940582901,8.28455561418372,-19.5683070774105)) ;
#113449=CARTESIAN_POINT('Ctrl Pts',(8.54864697316327,8.28433787538015,-19.5668714498003)) ;
#113450=CARTESIAN_POINT('Ctrl Pts',(8.5485873643535,8.28409676597397,-19.5654408395913)) ;
#113451=CARTESIAN_POINT('Ctrl Pts',(8.54851996240545,8.28383343043593,-19.5640172030853)) ;
#113452=CARTESIAN_POINT('Origin',(8.4,6.65,-22.86)) ;
#113453=CARTESIAN_POINT('Origin',(8.4,6.65,-19.7793219981003)) ;
#113454=CARTESIAN_POINT('Origin',(8.49172374697018,6.65,-22.86)) ;
#113455=CARTESIAN_POINT('Origin',(8.49225485641684,6.63809817973796,-19.5470086283537)) ;
#113456=CARTESIAN_POINT('Origin',(8.6,4.35421736843756,-19.7797127088383)) ;
#113457=CARTESIAN_POINT('Origin',(8.6,6.66256607592813,-19.7797127088383)) ;
#113458=CARTESIAN_POINT('Ctrl Pts',(8.50134874936238,6.65217253603381,-19.7959852560808)) ;
#113459=CARTESIAN_POINT('Ctrl Pts',(8.50315244876582,6.5499712757703,-19.7965863692586)) ;
#113460=CARTESIAN_POINT('Ctrl Pts',(8.40269444133667,6.55000000392137,-19.8115964965758)) ;
#113461=CARTESIAN_POINT('Ctrl Pts',(8.49631753783953,6.64933701877088,-19.7650156523955)) ;
#113462=CARTESIAN_POINT('Ctrl Pts',(8.49707874924866,6.54997270174429,-19.7639612234982)) ;
#113463=CARTESIAN_POINT('Ctrl Pts',(8.39261127161998,6.55000000381176,-19.7525550208105)) ;
#113464=CARTESIAN_POINT('Ctrl Pts',(8.50556246021202,6.6507523520896,-19.7360110455015)) ;
#113465=CARTESIAN_POINT('Ctrl Pts',(8.50253957946717,6.54997202229494,-19.7396441304546)) ;
#113466=CARTESIAN_POINT('Ctrl Pts',(8.41103525938995,6.55000000386643,-19.6913383496346)) ;
#113467=CARTESIAN_POINT('Ctrl Pts',(8.52891970071474,6.63645479210453,-19.7065271584827)) ;
#113468=CARTESIAN_POINT('Ctrl Pts',(8.52027792490146,6.54997752826675,-19.6984049399611)) ;
#113469=CARTESIAN_POINT('Ctrl Pts',(8.4576425585104,6.5500000033157,-19.637390101583)) ;
#113470=CARTESIAN_POINT('Ctrl Pts',(8.53324635448931,6.63340383613801,-19.7017820657382)) ;
#113471=CARTESIAN_POINT('Ctrl Pts',(8.52338394863782,6.5499786118932,-19.6915733138909)) ;
#113472=CARTESIAN_POINT('Ctrl Pts',(8.46627109069301,6.55000000319827,-19.6290047485327)) ;
#113473=CARTESIAN_POINT('Ctrl Pts',(8.54254332011243,6.62325922024827,-19.6911417482178)) ;
#113474=CARTESIAN_POINT('Ctrl Pts',(8.53005572430516,6.54998198465682,-19.674932642468)) ;
#113475=CARTESIAN_POINT('Ctrl Pts',(8.48480454940912,6.55000000280808,-19.6136278088231)) ;
#113476=CARTESIAN_POINT('Ctrl Pts',(8.54755771953125,6.61716872587347,-19.6871385438772)) ;
#113477=CARTESIAN_POINT('Ctrl Pts',(8.53352383957151,6.54998388968243,-19.6670066149145)) ;
#113478=CARTESIAN_POINT('Ctrl Pts',(8.49480263348509,6.55000000257396,-19.6067172762992)) ;
#113479=CARTESIAN_POINT('Ctrl Pts',(8.55524400651034,6.59355301617587,-19.6664805698954)) ;
#113480=CARTESIAN_POINT('Ctrl Pts',(8.53873552501335,6.54999036710752,-19.6412948588094)) ;
#113481=CARTESIAN_POINT('Ctrl Pts',(8.51008526949062,6.55000000166752,-19.5967757494185)) ;
#113482=CARTESIAN_POINT('Ctrl Pts',(8.55791451833572,6.5808349442897,-19.6584270674629)) ;
#113483=CARTESIAN_POINT('Ctrl Pts',(8.54027978136633,6.54999344602544,-19.6315790288336)) ;
#113484=CARTESIAN_POINT('Ctrl Pts',(8.51542462880467,6.55000000118004,-19.5938063443386)) ;
#113485=CARTESIAN_POINT('Ctrl Pts',(8.56122429319345,6.56135755929253,-19.6154165389637)) ;
#113486=CARTESIAN_POINT('Ctrl Pts',(8.54270214007079,6.54999771321877,-19.6020999056444)) ;
#113487=CARTESIAN_POINT('Ctrl Pts',(8.5219443634021,6.55000000043436,-19.5872674436738)) ;
#113488=CARTESIAN_POINT('Ctrl Pts',(8.56215003896757,6.55689889598542,-19.5925513447558)) ;
#113489=CARTESIAN_POINT('Ctrl Pts',(8.54355112280986,6.54999862629019,-19.5885854140212)) ;
#113490=CARTESIAN_POINT('Ctrl Pts',(8.52363168464781,6.55000000026381,-19.5841937607945)) ;
#113491=CARTESIAN_POINT('Ctrl Pts',(8.56153943432815,6.55906352913399,-19.5572061237906)) ;
#113492=CARTESIAN_POINT('Ctrl Pts',(8.54309854033143,6.54999818700351,-19.5671631682683)) ;
#113493=CARTESIAN_POINT('Ctrl Pts',(8.52276767133745,6.5500000003466,-19.5781675131799)) ;
#113494=CARTESIAN_POINT('Ctrl Pts',(8.5605912372004,6.56303220640817,-19.5454869464624)) ;
#113495=CARTESIAN_POINT('Ctrl Pts',(8.54200379397878,6.54999736403673,-19.5594720470655)) ;
#113496=CARTESIAN_POINT('Ctrl Pts',(8.52069177703237,6.55000000049843,-19.575521343736)) ;
#113497=CARTESIAN_POINT('Ctrl Pts',(8.5575081978017,6.57321782814896,-19.5188078145324)) ;
#113498=CARTESIAN_POINT('Ctrl Pts',(8.53873610184732,6.54999517041883,-19.5405268596428)) ;
#113499=CARTESIAN_POINT('Ctrl Pts',(8.5145479773404,6.55000000088831,-19.568656630824)) ;
#113500=CARTESIAN_POINT('Ctrl Pts',(8.55505442469281,6.57990173798312,-19.5092926744612)) ;
#113501=CARTESIAN_POINT('Ctrl Pts',(8.53621107118182,6.54999365791213,-19.5321766604066)) ;
#113502=CARTESIAN_POINT('Ctrl Pts',(8.50963525726155,6.55000000114429,-19.5648261829157)) ;
#113503=CARTESIAN_POINT('Ctrl Pts',(8.55022399280473,6.59153973477787,-19.4929352059185)) ;
#113504=CARTESIAN_POINT('Ctrl Pts',(8.5315601554517,6.54999086985385,-19.5166211671793)) ;
#113505=CARTESIAN_POINT('Ctrl Pts',(8.49999539447561,6.55000000159032,-19.5571278236793)) ;
#113506=CARTESIAN_POINT('Ctrl Pts',(8.54779538881607,6.5966534953294,-19.4869161916983)) ;
#113507=CARTESIAN_POINT('Ctrl Pts',(8.52936575151139,6.54998957392002,-19.5099955473559)) ;
#113508=CARTESIAN_POINT('Ctrl Pts',(8.49512741158077,6.55000000178643,-19.5533364158986)) ;
#113509=CARTESIAN_POINT('Ctrl Pts',(8.54538355337156,6.60121171185028,-19.4816751744843)) ;
#113510=CARTESIAN_POINT('Ctrl Pts',(8.52733415536173,6.54998837980801,-19.5038983572099)) ;
#113511=CARTESIAN_POINT('Ctrl Pts',(8.49033880598518,6.55000000196131,-19.5494485970987)) ;
#113512=CARTESIAN_POINT('',(8.5458234418239,6.61635369861655,-19.6860636515728)) ;
#113513=CARTESIAN_POINT('Ctrl Pts',(8.5458234418239,6.61635369861655,-19.6860636515728)) ;
#113514=CARTESIAN_POINT('Ctrl Pts',(8.54493595163524,6.61793460914645,-19.6873940762098)) ;
#113515=CARTESIAN_POINT('Ctrl Pts',(8.54398448171073,6.61948114927949,-19.6887173928307)) ;
#113516=CARTESIAN_POINT('Ctrl Pts',(8.54296332801272,6.6209780844369,-19.6900407367798)) ;
#113517=CARTESIAN_POINT('Ctrl Pts',(8.53827263106763,6.62785429629763,-19.6961195527619)) ;
#113518=CARTESIAN_POINT('Ctrl Pts',(8.53198779426187,6.63349037496299,-19.7026115685244)) ;
#113519=CARTESIAN_POINT('Ctrl Pts',(8.5259873730411,6.63731070037229,-19.7100705892422)) ;
#113520=CARTESIAN_POINT('Ctrl Pts',(8.52000560405467,6.64111915034781,-19.7175064236874)) ;
#113521=CARTESIAN_POINT('Ctrl Pts',(8.51430181273566,6.64349626850742,-19.7260376473014)) ;
#113522=CARTESIAN_POINT('Ctrl Pts',(8.50998586672548,6.64522349213896,-19.7352009869701)) ;
#113523=CARTESIAN_POINT('Ctrl Pts',(8.50534188065424,6.64708199603772,-19.7450608002501)) ;
#113524=CARTESIAN_POINT('Ctrl Pts',(8.50212992821339,6.64824261275105,-19.7558875436748)) ;
#113525=CARTESIAN_POINT('Ctrl Pts',(8.50077314609738,6.64911992656046,-19.7668249119168)) ;
#113526=CARTESIAN_POINT('Ctrl Pts',(8.50025986706873,6.64945181977648,-19.7709625856677)) ;
#113527=CARTESIAN_POINT('Ctrl Pts',(8.50000017127792,6.64974165917873,-19.7751432551012)) ;
#113528=CARTESIAN_POINT('Ctrl Pts',(8.5000000000847,6.64999974464545,-19.7793178674956)) ;
#113529=CARTESIAN_POINT('',(8.55242393572497,6.60106172182536,-19.673242098716)) ;
#113530=CARTESIAN_POINT('Ctrl Pts',(8.55241775170037,6.6010680791717,-19.6732328161544)) ;
#113531=CARTESIAN_POINT('Ctrl Pts',(8.55072388788565,6.60619026743349,-19.6777214769524)) ;
#113532=CARTESIAN_POINT('Ctrl Pts',(8.54858294048575,6.61143812822761,-19.6819269241448)) ;
#113533=CARTESIAN_POINT('Ctrl Pts',(8.5458234418239,6.61635369861655,-19.6860636515728)) ;
#113534=CARTESIAN_POINT('Ctrl Pts',(8.55635360773813,6.58637108369504,-19.6586323907337)) ;
#113535=CARTESIAN_POINT('Ctrl Pts',(8.55606387390184,6.58765239867375,-19.6601123828074)) ;
#113536=CARTESIAN_POINT('Ctrl Pts',(8.55575324501786,6.5889682390234,-19.6615659413334)) ;
#113537=CARTESIAN_POINT('Ctrl Pts',(8.55541196992778,6.5903724112747,-19.66304320494)) ;
#113538=CARTESIAN_POINT('Ctrl Pts',(8.55524290008387,6.59106804711291,-19.6637750506991)) ;
#113539=CARTESIAN_POINT('Ctrl Pts',(8.55506631250724,6.59178496983012,-19.6645119588375)) ;
#113540=CARTESIAN_POINT('Ctrl Pts',(8.55488049708426,6.59252693597574,-19.665256277619)) ;
#113541=CARTESIAN_POINT('Ctrl Pts',(8.55445908016383,6.59420966544526,-19.666944342709)) ;
#113542=CARTESIAN_POINT('Ctrl Pts',(8.55403589309453,6.59584037906545,-19.6684883777226)) ;
#113543=CARTESIAN_POINT('Ctrl Pts',(8.55359592981642,6.59737680581866,-19.6699031562334)) ;
#113544=CARTESIAN_POINT('Ctrl Pts',(8.55324292160432,6.598609570661,-19.671038315592)) ;
#113545=CARTESIAN_POINT('Ctrl Pts',(8.55287861047125,6.59978201473819,-19.6720910425071)) ;
#113546=CARTESIAN_POINT('Ctrl Pts',(8.55248933155918,6.60087815532536,-19.6730771269866)) ;
#113547=CARTESIAN_POINT('Ctrl Pts',(8.55246754857568,6.60093949235542,-19.6731323055778)) ;
#113548=CARTESIAN_POINT('Ctrl Pts',(8.55244574956032,6.60100068203144,-19.6731872962784)) ;
#113549=CARTESIAN_POINT('Ctrl Pts',(8.55242393572497,6.60106172182536,-19.673242098716)) ;
#113550=CARTESIAN_POINT('Ctrl Pts',(8.5,6.66256607592813,-19.7797127088383)) ;
#113551=CARTESIAN_POINT('Ctrl Pts',(8.5,6.66256607592813,-19.695)) ;
#113552=CARTESIAN_POINT('Ctrl Pts',(8.58356010126947,6.66256607592813,-19.6810733164551)) ;
#113553=CARTESIAN_POINT('Ctrl Pts',(8.5,6.61011302719839,-19.779712707263)) ;
#113554=CARTESIAN_POINT('Ctrl Pts',(8.5,6.63245216822994,-19.6985572365993)) ;
#113555=CARTESIAN_POINT('Ctrl Pts',(8.57941760042978,6.6356398188513,-19.6817637332617)) ;
#113556=CARTESIAN_POINT('Ctrl Pts',(8.5,6.55934573373302,-19.7588469099427)) ;
#113557=CARTESIAN_POINT('Ctrl Pts',(8.5,6.60054351783555,-19.6880813958278)) ;
#113558=CARTESIAN_POINT('Ctrl Pts',(8.57705842698403,6.6098757899343,-19.6717275280477)) ;
#113559=CARTESIAN_POINT('Ctrl Pts',(8.5,6.52274941072028,-19.7222505892797)) ;
#113560=CARTESIAN_POINT('Ctrl Pts',(8.5,6.57873105977929,-19.6662689402207)) ;
#113561=CARTESIAN_POINT('Ctrl Pts',(8.57705842661295,6.59157413088145,-19.6534258691185)) ;
#113562=CARTESIAN_POINT('Origin',(8.49172374697003,1.4,-22.86)) ;
#113563=CARTESIAN_POINT('Origin',(8.49172374697003,1.4,-18.3578583129651)) ;
#113564=CARTESIAN_POINT('Origin',(8.49172374697002,1.4,-18.3578583129651)) ;
#113565=CARTESIAN_POINT('Origin',(8.49172374697003,1.4,-18.3578583129651)) ;
#113566=CARTESIAN_POINT('Ctrl Pts',(8.50816364570057,1.49863939238321,-18.3578583129651)) ;
#113567=CARTESIAN_POINT('Ctrl Pts',(8.51019246767907,1.4983012553868,-18.392927584071)) ;
#113568=CARTESIAN_POINT('Ctrl Pts',(8.50816364570057,1.47636598119991,-18.4202920109583)) ;
#113569=CARTESIAN_POINT('Ctrl Pts',(8.97755831131121,1.42040694811478,-18.3299486511532)) ;
#113570=CARTESIAN_POINT('Ctrl Pts',(8.97879997398643,1.42020000433524,-18.3645666731799)) ;
#113571=CARTESIAN_POINT('Ctrl Pts',(8.97755831689156,1.39869563385813,-18.3916948169504)) ;
#113572=CARTESIAN_POINT('Ctrl Pts',(9.44698496305965,1.34216917282337,-18.3026313706301)) ;
#113573=CARTESIAN_POINT('Ctrl Pts',(9.44827639615879,1.34195393397322,-18.3367775286088)) ;
#113574=CARTESIAN_POINT('Ctrl Pts',(9.44698496887881,1.32097764915797,-18.3637229847104)) ;
#113575=CARTESIAN_POINT('Ctrl Pts',(9.91643989873053,1.26392668354489,-18.2758381198218)) ;
#113576=CARTESIAN_POINT('Ctrl Pts',(9.91830968165731,1.26361505305709,-18.309509344197)) ;
#113577=CARTESIAN_POINT('Ctrl Pts',(9.91643989873053,1.24322097942674,-18.336303564194)) ;
#113578=CARTESIAN_POINT('Origin',(9.9,1.16528729116168,-18.2758381198218)) ;
#113579=CARTESIAN_POINT('Origin',(9.9,1.16528729116168,-18.2758381198218)) ;
#113580=CARTESIAN_POINT('Origin',(-0.4,-3.36847777691809,-20.72)) ;
#113581=CARTESIAN_POINT('Origin',(-0.400000000000001,-3.36847777691809,
-20.72)) ;
#113582=CARTESIAN_POINT('Origin',(-0.4,-3.36847777691809,-20.72)) ;
#113583=CARTESIAN_POINT('Origin',(-0.400000000000001,-3.36847777691809,
-19.82)) ;
#113584=CARTESIAN_POINT('Origin',(-0.4,-3.36847777691809,-19.92)) ;
#113585=CARTESIAN_POINT('Origin',(-1.11032778078669,-3.36847777691809,-20.72)) ;
#113586=CARTESIAN_POINT('Origin',(0.4,-3.36847777691809,-20.72)) ;
#113587=CARTESIAN_POINT('Origin',(-0.400000000000001,-3.36847777691809,
-19.92)) ;
#113588=CARTESIAN_POINT('Origin',(-0.4,-3.36847777691809,-19.92)) ;
#113589=CARTESIAN_POINT('Origin',(0.400000000000001,-3.36847777691809,-20.72)) ;
#113590=CARTESIAN_POINT('Origin',(0.400000000000001,-3.36847777691809,-20.72)) ;
#113591=CARTESIAN_POINT('Origin',(1.5,-3.36847777691809,-19.92)) ;
#113592=CARTESIAN_POINT('Origin',(0.4,-3.36847777691809,-19.92)) ;
#113593=CARTESIAN_POINT('Origin',(0.4,-3.36847777691809,-19.82)) ;
#113594=CARTESIAN_POINT('Origin',(0.4,-3.36847777691809,-19.92)) ;
#113595=CARTESIAN_POINT('Origin',(0.4,-3.36847777691809,-19.92)) ;
#113596=CARTESIAN_POINT('Origin',(7.96847777691809,3.4,-20.72)) ;
#113597=CARTESIAN_POINT('Origin',(7.96847777691809,3.4,-20.72)) ;
#113598=CARTESIAN_POINT('Origin',(7.96847777691809,3.4,-20.72)) ;
#113599=CARTESIAN_POINT('Origin',(7.96847777691809,3.4,-19.82)) ;
#113600=CARTESIAN_POINT('Origin',(7.96847777691809,3.4,-19.92)) ;
#113601=CARTESIAN_POINT('Origin',(7.96847777691809,2.68967221921331,-20.72)) ;
#113602=CARTESIAN_POINT('Origin',(7.96847777691809,4.2,-20.72)) ;
#113603=CARTESIAN_POINT('Origin',(7.96847777691809,3.4,-19.92)) ;
#113604=CARTESIAN_POINT('Origin',(7.96847777691809,3.4,-19.92)) ;
#113605=CARTESIAN_POINT('Origin',(7.96847777691809,4.2,-20.72)) ;
#113606=CARTESIAN_POINT('Origin',(7.96847777691809,4.2,-20.72)) ;
#113607=CARTESIAN_POINT('Origin',(7.96847777691809,2.3,-19.92)) ;
#113608=CARTESIAN_POINT('Origin',(7.96847777691809,4.2,-19.92)) ;
#113609=CARTESIAN_POINT('Origin',(7.96847777691809,4.2,-19.82)) ;
#113610=CARTESIAN_POINT('Origin',(7.96847777691809,4.2,-19.92)) ;
#113611=CARTESIAN_POINT('Origin',(7.96847777691809,4.2,-19.92)) ;
#113612=CARTESIAN_POINT('Origin',(8.49172374697003,1.4,-22.86)) ;
#113613=CARTESIAN_POINT('Origin',(8.49172374697003,1.4,-22.2821416870349)) ;
#113614=CARTESIAN_POINT('Origin',(8.49172374697002,1.4,-22.2821416870349)) ;
#113615=CARTESIAN_POINT('Origin',(8.49172374697003,1.39999999999989,-22.2821416870347)) ;
#113616=CARTESIAN_POINT('Ctrl Pts',(8.50816364570058,1.47636598119991,-22.2197079890417)) ;
#113617=CARTESIAN_POINT('Ctrl Pts',(8.51019246767907,1.4983012553868,-22.247072415929)) ;
#113618=CARTESIAN_POINT('Ctrl Pts',(8.50816364570058,1.49863939238321,-22.2821416870349)) ;
#113619=CARTESIAN_POINT('Ctrl Pts',(8.97755831689149,1.39869563385714,-22.2483051830483)) ;
#113620=CARTESIAN_POINT('Ctrl Pts',(8.97879997398686,1.42020000433534,-22.2754333268135)) ;
#113621=CARTESIAN_POINT('Ctrl Pts',(8.97755831131135,1.42040694811475,-22.3100513488443)) ;
#113622=CARTESIAN_POINT('Ctrl Pts',(9.44698496887879,1.32097764915799,-22.2762770152897)) ;
#113623=CARTESIAN_POINT('Ctrl Pts',(9.4482763961588,1.34195393397339,-22.3032224713911)) ;
#113624=CARTESIAN_POINT('Ctrl Pts',(9.44698496305964,1.34216917282337,-22.3373686293698)) ;
#113625=CARTESIAN_POINT('Ctrl Pts',(9.91643989873053,1.24322097942674,-22.303696435806)) ;
#113626=CARTESIAN_POINT('Ctrl Pts',(9.91830968165732,1.26361505305709,-22.330490655803)) ;
#113627=CARTESIAN_POINT('Ctrl Pts',(9.91643989873053,1.26392668354489,-22.3641618801782)) ;
#113628=CARTESIAN_POINT('Origin',(9.9,1.16528729116168,-22.3641618801782)) ;
#113629=CARTESIAN_POINT('Origin',(9.9,1.16528729116168,-22.3641618801782)) ;
#113630=CARTESIAN_POINT('Origin',(8.48377223398316,8.2,-22.86)) ;
#113631=CARTESIAN_POINT('Origin',(8.48238054866943,8.20007133352095,-19.5731789312376)) ;
#113632=CARTESIAN_POINT('Ctrl Pts',(8.40201662970151,8.3,-19.8059759779215)) ;
#113633=CARTESIAN_POINT('Ctrl Pts',(8.50299337454958,8.3,-19.7926748112638)) ;
#113634=CARTESIAN_POINT('Ctrl Pts',(8.50100123624931,8.19773961376455,-19.7926888461178)) ;
#113635=CARTESIAN_POINT('Ctrl Pts',(8.39454129798956,8.3,-19.7544981813506)) ;
#113636=CARTESIAN_POINT('Ctrl Pts',(8.49697875237666,8.3,-19.7653741113344)) ;
#113637=CARTESIAN_POINT('Ctrl Pts',(8.49727262260757,8.20135231978541,-19.765067063962)) ;
#113638=CARTESIAN_POINT('Ctrl Pts',(8.40820218948347,8.3,-19.7020253635243)) ;
#113639=CARTESIAN_POINT('Ctrl Pts',(8.49818669687012,8.3,-19.7424717278015)) ;
#113640=CARTESIAN_POINT('Ctrl Pts',(8.50412619268399,8.20300739730705,-19.7403884100248)) ;
#113641=CARTESIAN_POINT('Ctrl Pts',(8.4430413476632,8.3,-19.6509969330871)) ;
#113642=CARTESIAN_POINT('Ctrl Pts',(8.50894174387208,8.3,-19.7008550553805)) ;
#113643=CARTESIAN_POINT('Ctrl Pts',(8.52157716465943,8.21896555381606,-19.7101661266503)) ;
#113644=CARTESIAN_POINT('Ctrl Pts',(8.44963266995283,8.3,-19.6426678319782)) ;
#113645=CARTESIAN_POINT('Ctrl Pts',(8.51095981317517,8.3,-19.6937494404835)) ;
#113646=CARTESIAN_POINT('Ctrl Pts',(8.52487915500779,8.22226238914488,-19.7049516180519)) ;
#113647=CARTESIAN_POINT('Ctrl Pts',(8.46372306360151,8.3,-19.6269547263199)) ;
#113648=CARTESIAN_POINT('Ctrl Pts',(8.51547368264944,8.3,-19.6776327910559)) ;
#113649=CARTESIAN_POINT('Ctrl Pts',(8.53193863144477,8.23129792829964,-19.6933174783855)) ;
#113650=CARTESIAN_POINT('Ctrl Pts',(8.47128983770082,8.3,-19.6195586271464)) ;
#113651=CARTESIAN_POINT('Ctrl Pts',(8.51796237042371,8.3,-19.6692464949128)) ;
#113652=CARTESIAN_POINT('Ctrl Pts',(8.53572833262714,8.23677343862355,-19.6874295885078)) ;
#113653=CARTESIAN_POINT('Ctrl Pts',(8.48287565264707,8.3,-19.6087307948332)) ;
#113654=CARTESIAN_POINT('Ctrl Pts',(8.52168214469875,8.3,-19.65074351943)) ;
#113655=CARTESIAN_POINT('Ctrl Pts',(8.54153766811345,8.25077321967989,-19.6720449871073)) ;
#113656=CARTESIAN_POINT('Ctrl Pts',(8.48680760428676,8.3,-19.605187297402)) ;
#113657=CARTESIAN_POINT('Ctrl Pts',(8.52287759291296,8.3,-19.6441435049317)) ;
#113658=CARTESIAN_POINT('Ctrl Pts',(8.54350322705384,8.2564691763754,-19.6662622666034)) ;
#113659=CARTESIAN_POINT('Ctrl Pts',(8.49230810302881,8.3,-19.5994953499955)) ;
#113660=CARTESIAN_POINT('Ctrl Pts',(8.52426411271138,8.3,-19.6285665246336)) ;
#113661=CARTESIAN_POINT('Ctrl Pts',(8.54627296401924,8.26866384868896,-19.6485525693616)) ;
#113662=CARTESIAN_POINT('Ctrl Pts',(8.49410170711667,8.3,-19.597526518934)) ;
#113663=CARTESIAN_POINT('Ctrl Pts',(8.52463604790914,8.3,-19.6224055253652)) ;
#113664=CARTESIAN_POINT('Ctrl Pts',(8.54716490137965,8.27360757863441,-19.6407959594825)) ;
#113665=CARTESIAN_POINT('Ctrl Pts',(8.49698869685298,8.3,-19.5930732788095)) ;
#113666=CARTESIAN_POINT('Ctrl Pts',(8.52523118911551,8.3,-19.6065929344384)) ;
#113667=CARTESIAN_POINT('Ctrl Pts',(8.54862931231183,8.28262305001768,-19.6178413492705)) ;
#113668=CARTESIAN_POINT('Ctrl Pts',(8.49798687771249,8.3,-19.5905165211566)) ;
#113669=CARTESIAN_POINT('Ctrl Pts',(8.52551930315386,8.3,-19.5969062760439)) ;
#113670=CARTESIAN_POINT('Ctrl Pts',(8.54912969489065,8.28574379441722,-19.6023818974934)) ;
#113671=CARTESIAN_POINT('Ctrl Pts',(8.49821791151749,8.3,-19.5825795709374)) ;
#113672=CARTESIAN_POINT('Ctrl Pts',(8.52559423327562,8.3,-19.5721891247048)) ;
#113673=CARTESIAN_POINT('Ctrl Pts',(8.54922875625409,8.28635135062008,-19.5632386700468)) ;
#113674=CARTESIAN_POINT('Ctrl Pts',(8.49537847603514,8.3,-19.5776469108458)) ;
#113675=CARTESIAN_POINT('Ctrl Pts',(8.5243933105344,8.3,-19.5614732749821)) ;
#113676=CARTESIAN_POINT('Ctrl Pts',(8.54781890418529,8.28040548672879,-19.548471793372)) ;
#113677=CARTESIAN_POINT('Ctrl Pts',(8.48955273785443,8.3,-19.5689114034569)) ;
#113678=CARTESIAN_POINT('Ctrl Pts',(8.52168703568127,8.3,-19.5440525851282)) ;
#113679=CARTESIAN_POINT('Ctrl Pts',(8.54489815533716,8.27194212599123,-19.5261670077071)) ;
#113680=CARTESIAN_POINT('Ctrl Pts',(8.48620077197361,8.3,-19.5648263075048)) ;
#113681=CARTESIAN_POINT('Ctrl Pts',(8.52012703453235,8.3,-19.5371073328932)) ;
#113682=CARTESIAN_POINT('Ctrl Pts',(8.54324008387894,8.26788967346962,-19.5183142356383)) ;
#113683=CARTESIAN_POINT('Ctrl Pts',(8.48280151347419,8.3,-19.5607911096407)) ;
#113684=CARTESIAN_POINT('Ctrl Pts',(8.51858761497412,8.3,-19.5306520257852)) ;
#113685=CARTESIAN_POINT('Ctrl Pts',(8.54152015125555,8.26408224232382,-19.5113382250347)) ;
#113686=CARTESIAN_POINT('Origin',(8.4,8.2,-19.777927110149)) ;
#113687=CARTESIAN_POINT('Origin',(8.4,8.2,-20.945)) ;
#113688=CARTESIAN_POINT('Origin',(8.4,8.2,-20.862072889851)) ;
#113689=CARTESIAN_POINT('Ctrl Pts',(8.50101530037396,8.19768718256762,-20.8472017745814)) ;
#113690=CARTESIAN_POINT('Ctrl Pts',(8.50305639000874,8.3,-20.8472198113571)) ;
#113691=CARTESIAN_POINT('Ctrl Pts',(8.40204633857706,8.3,-20.8338202021253)) ;
#113692=CARTESIAN_POINT('Ctrl Pts',(8.49725464441631,8.20131038948437,-20.8748679119096)) ;
#113693=CARTESIAN_POINT('Ctrl Pts',(8.4970139180527,8.29999999999998,-20.8745609423402)) ;
#113694=CARTESIAN_POINT('Ctrl Pts',(8.39450526457596,8.3,-20.8853632910711)) ;
#113695=CARTESIAN_POINT('Ctrl Pts',(8.50410935041309,8.20295267265882,-20.8995792968114)) ;
#113696=CARTESIAN_POINT('Ctrl Pts',(8.49820749521504,8.30000000000005,-20.8974643378906)) ;
#113697=CARTESIAN_POINT('Ctrl Pts',(8.40816401923479,8.3,-20.9379187290433)) ;
#113698=CARTESIAN_POINT('Ctrl Pts',(8.52158236570989,8.2189321678965,-20.9298300407758)) ;
#113699=CARTESIAN_POINT('Ctrl Pts',(8.5089645656652,8.29999999999999,-20.9391276783841)) ;
#113700=CARTESIAN_POINT('Ctrl Pts',(8.44304134766321,8.3,-20.9890030669129)) ;
#113701=CARTESIAN_POINT('Ctrl Pts',(8.52488496507049,8.22222991631201,-20.9350437061782)) ;
#113702=CARTESIAN_POINT('Ctrl Pts',(8.51098076140206,8.29999999999999,-20.9462331109763)) ;
#113703=CARTESIAN_POINT('Ctrl Pts',(8.44963266995282,8.3,-20.9973321680218)) ;
#113704=CARTESIAN_POINT('Ctrl Pts',(8.53194575580938,8.23126818558572,-20.9466757349666)) ;
#113705=CARTESIAN_POINT('Ctrl Pts',(8.51549074202138,8.30000000000001,-20.9623505031351)) ;
#113706=CARTESIAN_POINT('Ctrl Pts',(8.46372306360152,8.3,-21.0130452736801)) ;
#113707=CARTESIAN_POINT('Ctrl Pts',(8.53573618291037,8.23674548871788,-20.9525623770273)) ;
#113708=CARTESIAN_POINT('Ctrl Pts',(8.51797743940283,8.3,-20.9707374625586)) ;
#113709=CARTESIAN_POINT('Ctrl Pts',(8.47128983770083,8.3,-21.0204413728536)) ;
#113710=CARTESIAN_POINT('Ctrl Pts',(8.54154687836688,8.25075037830458,-20.9679451319455)) ;
#113711=CARTESIAN_POINT('Ctrl Pts',(8.52169408444524,8.3,-20.9892435543493)) ;
#113712=CARTESIAN_POINT('Ctrl Pts',(8.48287565264706,8.3,-21.0312692051668)) ;
#113713=CARTESIAN_POINT('Ctrl Pts',(8.54351297666181,8.25644859419422,-20.9737272780162)) ;
#113714=CARTESIAN_POINT('Ctrl Pts',(8.52288848488736,8.3,-20.9958447315488)) ;
#113715=CARTESIAN_POINT('Ctrl Pts',(8.48680760428676,8.3,-21.034812702598)) ;
#113716=CARTESIAN_POINT('Ctrl Pts',(8.54628376412584,8.26864846827403,-20.9914376231601)) ;
#113717=CARTESIAN_POINT('Ctrl Pts',(8.52427341038692,8.3,-21.0114250170403)) ;
#113718=CARTESIAN_POINT('Ctrl Pts',(8.4923081030288,8.3,-21.0405046500045)) ;
#113719=CARTESIAN_POINT('Ctrl Pts',(8.54717611873857,8.27359443500939,-20.9991948837187)) ;
#113720=CARTESIAN_POINT('Ctrl Pts',(8.52464480444821,8.3,-21.0175873399142)) ;
#113721=CARTESIAN_POINT('Ctrl Pts',(8.49410170711667,8.3,-21.042473481066)) ;
#113722=CARTESIAN_POINT('Ctrl Pts',(8.54864126180654,8.28261417405722,-21.0221529061248)) ;
#113723=CARTESIAN_POINT('Ctrl Pts',(8.52523908688552,8.3,-21.0334032849063)) ;
#113724=CARTESIAN_POINT('Ctrl Pts',(8.49698869685298,8.3,-21.0469267211905)) ;
#113725=CARTESIAN_POINT('Ctrl Pts',(8.5491418548716,8.28573645090425,-21.0376152824162)) ;
#113726=CARTESIAN_POINT('Ctrl Pts',(8.52552693815802,8.3,-21.0430919520163)) ;
#113727=CARTESIAN_POINT('Ctrl Pts',(8.49798687771249,8.3,-21.0494834788434)) ;
#113728=CARTESIAN_POINT('Ctrl Pts',(8.54924094958847,8.28634430798884,-21.0767659475983)) ;
#113729=CARTESIAN_POINT('Ctrl Pts',(8.52560181204939,8.3,-21.0678137517531)) ;
#113730=CARTESIAN_POINT('Ctrl Pts',(8.49821791151747,8.3,-21.0574204290626)) ;
#113731=CARTESIAN_POINT('Ctrl Pts',(8.54783079466743,8.28039553911293,-21.0915348059813)) ;
#113732=CARTESIAN_POINT('Ctrl Pts',(8.52440147378976,8.3,-21.0785312754323)) ;
#113733=CARTESIAN_POINT('Ctrl Pts',(8.49537847603514,8.3,-21.0623530891542)) ;
#113734=CARTESIAN_POINT('Ctrl Pts',(8.5446588398693,8.27120119512636,-21.1157571947032)) ;
#113735=CARTESIAN_POINT('Ctrl Pts',(8.52145785975945,8.3,-21.0974902783301)) ;
#113736=CARTESIAN_POINT('Ctrl Pts',(8.48905244827037,8.3,-21.0718387647145)) ;
#113737=CARTESIAN_POINT('Ctrl Pts',(8.54267599402785,8.26648669506698,-21.1242949904305)) ;
#113738=CARTESIAN_POINT('Ctrl Pts',(8.51958784692425,8.3,-21.1052641321446)) ;
#113739=CARTESIAN_POINT('Ctrl Pts',(8.48503640902804,8.3,-21.0765685970659)) ;
#113740=CARTESIAN_POINT('Ctrl Pts',(8.54064021294341,8.26212437554838,-21.1322000298239)) ;
#113741=CARTESIAN_POINT('Ctrl Pts',(8.51779796763698,8.3,-21.1126895170151)) ;
#113742=CARTESIAN_POINT('Ctrl Pts',(8.48104783026774,8.3,-21.0812848074951)) ;
#113743=CARTESIAN_POINT('Origin',(8.48238055011341,8.20007134081619,-21.0668210700733)) ;
#113744=CARTESIAN_POINT('Origin',(8.48377223398316,8.2,-22.86)) ;
#126558=UNCERTAINTY_MEASURE_WITH_UNIT(LENGTH_MEASURE(0.01),#126572,
'DISTANCE_ACCURACY_VALUE',
'Maximum model space distance between geometric entities at asserted c
onnectivities') ;
#126563=UNCERTAINTY_MEASURE_WITH_UNIT(LENGTH_MEASURE(0.01),#126572,
'DISTANCE_ACCURACY_VALUE',
'Maximum model space distance between geometric entities at asserted c
onnectivities') ;
#126566=(
GEOMETRIC_REPRESENTATION_CONTEXT(3)
GLOBAL_UNCERTAINTY_ASSIGNED_CONTEXT((#126558))
GLOBAL_UNIT_ASSIGNED_CONTEXT((#126572,#126574,#126575))
REPRESENTATION_CONTEXT('','3D')
) ;
#126571=(
GEOMETRIC_REPRESENTATION_CONTEXT(3)
GLOBAL_UNCERTAINTY_ASSIGNED_CONTEXT((#126563))
GLOBAL_UNIT_ASSIGNED_CONTEXT((#126572,#126574,#126575))
REPRESENTATION_CONTEXT('','3D')
) ;
#126572=(
LENGTH_UNIT()
NAMED_UNIT(*)
SI_UNIT(.MILLI.,.METRE.)
) ;
#126574=(
NAMED_UNIT(*)
PLANE_ANGLE_UNIT()
SI_UNIT($,.RADIAN.)
) ;
#126575=(
NAMED_UNIT(*)
SI_UNIT($,.STERADIAN.)
SOLID_ANGLE_UNIT()
) ;
#126578=SHAPE_DEFINITION_REPRESENTATION(#126585,#126600) ;
#126585=PRODUCT_DEFINITION_SHAPE('',$,#126608) ;
#126600=SHAPE_REPRESENTATION('',(#68778),#126566) ;
#126605=PRODUCT_DEFINITION_CONTEXT('part definition',#126628,'design') ;
#126608=PRODUCT_DEFINITION('Header_200mil_N5','Header_200mil_N5',#126615,
#126605) ;
#126615=PRODUCT_DEFINITION_FORMATION('',$,#126632) ;
#126628=APPLICATION_CONTEXT(
'Core Data for Automotive Mechanical Design Process') ;
#126629=PRODUCT_CONTEXT('part definition',#126628,'mechanical') ;
#126632=PRODUCT('Header_200mil_N5','Header_200mil_N5',$,(#126629)) ;
#126639=PRESENTATION_STYLE_ASSIGNMENT((#126648)) ;
#126640=PRESENTATION_STYLE_ASSIGNMENT((#126649)) ;
#126641=PRESENTATION_STYLE_ASSIGNMENT((#126650)) ;
#126648=SURFACE_STYLE_USAGE(.BOTH.,#126657) ;
#126649=SURFACE_STYLE_USAGE(.BOTH.,#126658) ;
#126650=SURFACE_STYLE_USAGE(.BOTH.,#126659) ;
#126657=SURFACE_SIDE_STYLE('',(#126666)) ;
#126658=SURFACE_SIDE_STYLE('',(#126667)) ;
#126659=SURFACE_SIDE_STYLE('',(#126668)) ;
#126666=SURFACE_STYLE_FILL_AREA(#126675) ;
#126667=SURFACE_STYLE_FILL_AREA(#126676) ;
#126668=SURFACE_STYLE_FILL_AREA(#126677) ;
#126675=FILL_AREA_STYLE('Opaque(202,209,238)',(#126684)) ;
#126676=FILL_AREA_STYLE('Opaque(128,255,128)',(#126685)) ;
#126677=FILL_AREA_STYLE('Opaque(204,207,204)',(#126686)) ;
#126684=FILL_AREA_STYLE_COLOUR('Opaque(202,209,238)',#126693) ;
#126685=FILL_AREA_STYLE_COLOUR('Opaque(128,255,128)',#126694) ;
#126686=FILL_AREA_STYLE_COLOUR('Opaque(204,207,204)',#126695) ;
#126693=COLOUR_RGB('Opaque(202,209,238)', 0.66274510, 0.83137255, 0.94901961) ;
#126694=COLOUR_RGB('Opaque(128,255,128)', 0.66274510, 0.83137255, 0.94901961) ;
#126695=COLOUR_RGB('Opaque(204,207,204)', 0.40784314, 0.44705882, 0.49803922) ;
ENDSEC;
END-ISO-10303-21;
